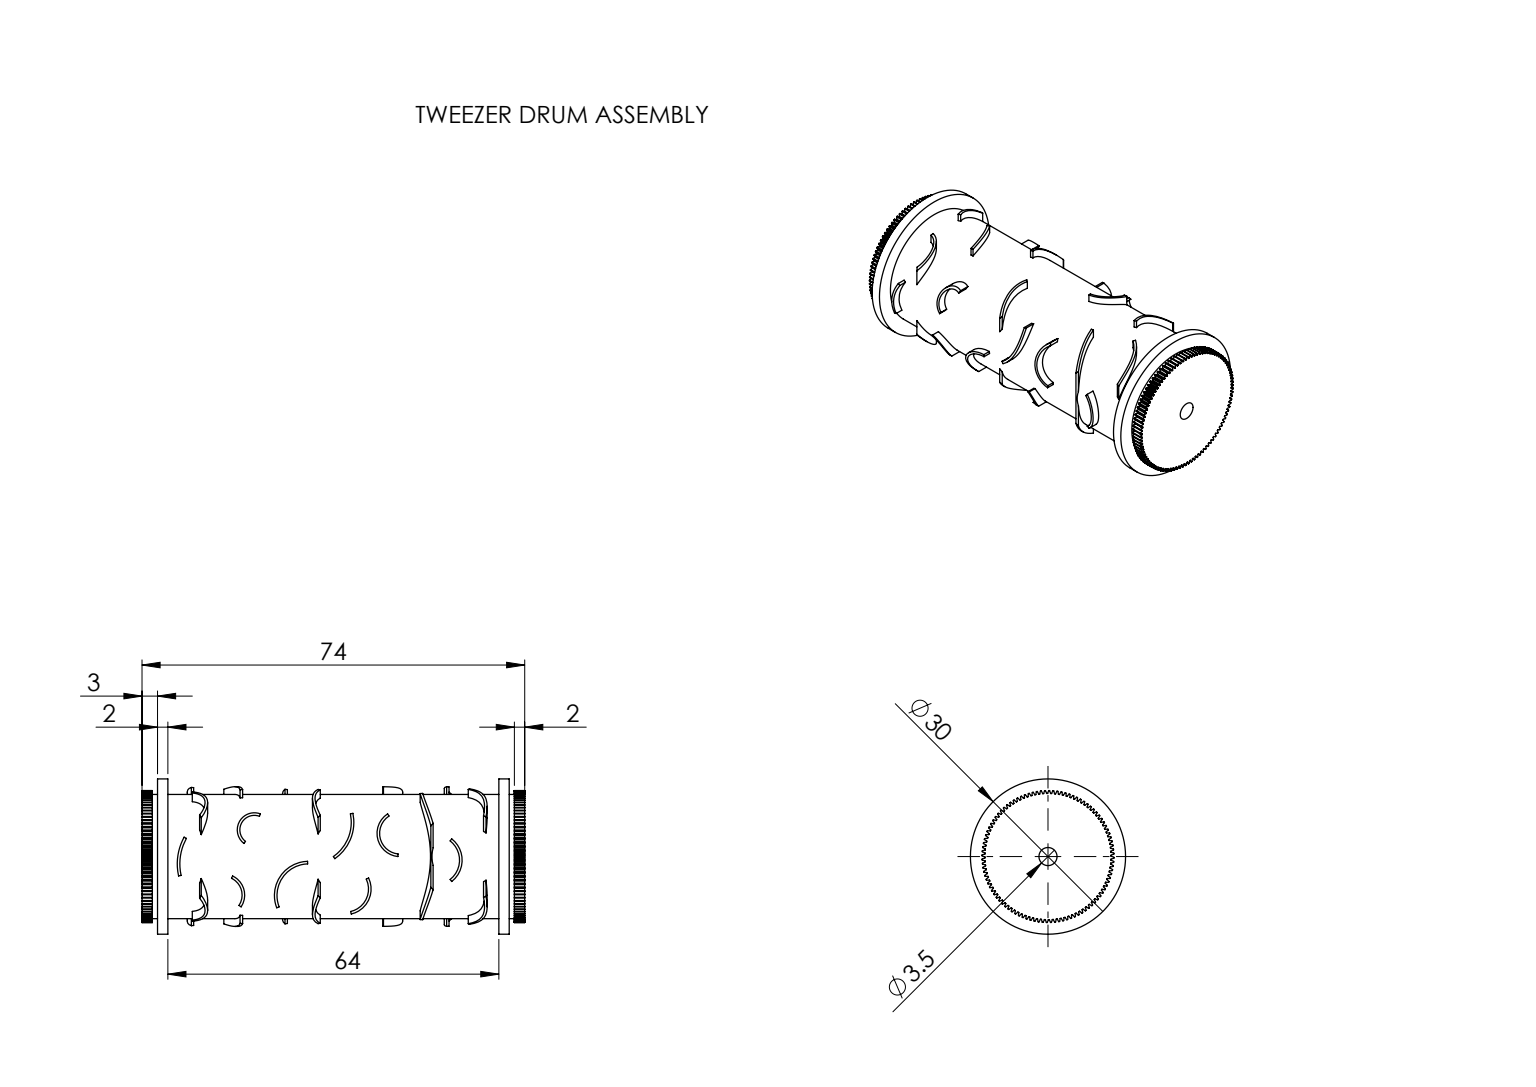
ISO-10303-21;
HEADER;
FILE_DESCRIPTION (('STEP AP214'),
    '1' );
FILE_NAME ('tweezer drum assembly.step',
    '2026-10-09T15:17:24',
    ( '' ),
    ( '' ),
    'SwSTEP 2.0',
    'SolidWorks 2026',
    '' );
FILE_SCHEMA (( 'AUTOMOTIVE_DESIGN' ));
ENDSEC;

DATA;
#1=ORIENTED_EDGE ( 'NONE', *, *, #54093, .F. ) ;
#2=( BOUNDED_CURVE ( )  B_SPLINE_CURVE ( 3, ( #3306, #62815, #58857, #63152 ),
 .UNSPECIFIED., .F., .T. ) 
 B_SPLINE_CURVE_WITH_KNOTS ( ( 4, 4 ),
 ( 1.289274629942206873, 1.307832622343243267 ),
 .UNSPECIFIED. ) 
 CURVE ( )  GEOMETRIC_REPRESENTATION_ITEM ( )  RATIONAL_B_SPLINE_CURVE ( ( 1.000000000000000000, 0.9999713002824244246, 0.9999713002824244246, 1.000000000000000000 ) ) 
 REPRESENTATION_ITEM ( '' )  );
#3=DIRECTION ( 'NONE',  ( 1.000000000000000000, 0.000000000000000000, -0.000000000000000000 ) ) ;
#4=CARTESIAN_POINT ( 'NONE',  ( 34.00000000000000000, 1.267509437117510519E-14, 0.000000000000000000 ) ) ;
#5=EDGE_CURVE ( 'NONE', #33980, #40116, #8200, .T. ) ;
#6=ORIENTED_EDGE ( 'NONE', *, *, #26203, .T. ) ;
#7=CARTESIAN_POINT ( 'NONE',  ( -27.64865282621882869, 11.88308961669896746, -6.412759754742364926 ) ) ;
#8=CARTESIAN_POINT ( 'NONE',  ( 29.22757921152195948, 7.948027597311009274, 9.002217460645077551 ) ) ;
#10=AXIS2_PLACEMENT_3D ( 'NONE', #51106, #21495, #16509 ) ;
#13=EDGE_CURVE ( 'NONE', #20288, #62523, #39030, .T. ) ;
#14=CIRCLE ( 'NONE', #45668, 4.999999999999999112 ) ;
#15=ORIENTED_EDGE ( 'NONE', *, *, #45352, .F. ) ;
#16=CARTESIAN_POINT ( 'NONE',  ( -2.532614230583026593, 25.00000000000000000, 10.89930238848911337 ) ) ;
#17=CARTESIAN_POINT ( 'NONE',  ( -20.31445708845316389, -13.09484702705360704, -3.338600914039887346 ) ) ;
#22=CARTESIAN_POINT ( 'NONE',  ( 37.00000000000000711, -6.303578524887017309, -10.42955799785317872 ) ) ;
#23=CARTESIAN_POINT ( 'NONE',  ( 3.459614771489464946, -11.09853614738469396, 25.00000000000000000 ) ) ;
#24=AXIS2_PLACEMENT_3D ( 'NONE', #425, #35953, #14688 ) ;
#26=CARTESIAN_POINT ( 'NONE',  ( 35.00000000000000000, 4.705694406421931860E-17, -3.469127814946512892E-15 ) ) ;
#27=CIRCLE ( 'NONE', #62657, 12.18649999999999878 ) ;
#29=CARTESIAN_POINT ( 'NONE',  ( 47.00000000000000711, 4.705694406421931860E-17, -3.469127814946512892E-15 ) ) ;
#30=DIRECTION ( 'NONE',  ( 1.000000000000000000, -0.000000000000000000, 0.000000000000000000 ) ) ;
#32=CARTESIAN_POINT ( 'NONE',  ( -36.00000000000000711, -2.527899948230555083, -12.49688848680887077 ) ) ;
#36=CIRCLE ( 'NONE', #39342, 5.000000000000000000 ) ;
#38=ORIENTED_EDGE ( 'NONE', *, *, #32481, .T. ) ;
#39=DIRECTION ( 'NONE',  ( 0.2227494284590502138, 0.000000000000000000, 0.9748757316300199482 ) ) ;
#41=DIRECTION ( 'NONE',  ( -1.000000000000000000, 0.000000000000000000, 0.000000000000000000 ) ) ;
#42=DIRECTION ( 'NONE',  ( -0.000000000000000000, -0.000000000000000000, -1.000000000000000000 ) ) ;
#43=ORIENTED_EDGE ( 'NONE', *, *, #16886, .F. ) ;
#44=VERTEX_POINT ( 'NONE', #43427 ) ;
#45=ORIENTED_EDGE ( 'NONE', *, *, #528, .T. ) ;
#47=AXIS2_PLACEMENT_3D ( 'NONE', #35700, #25750, #46038 ) ;
#48=CARTESIAN_POINT ( 'NONE',  ( -20.92008205012189848, -11.37744109147143590, -3.816568647652266222 ) ) ;
#49=EDGE_CURVE ( 'NONE', #39147, #50867, #8852, .T. ) ;
#52=CARTESIAN_POINT ( 'NONE',  ( 35.00000000000000000, 3.511814412392283646, 11.66953048682395355 ) ) ;
#54=ORIENTED_EDGE ( 'NONE', *, *, #43453, .T. ) ;
#56=EDGE_CURVE ( 'NONE', #31963, #46746, #12133, .T. ) ;
#58=DIRECTION ( 'NONE',  ( -0.000000000000000000, -0.000000000000000000, -1.000000000000000000 ) ) ;
#62=EDGE_LOOP ( 'NONE', ( #29288, #23107, #41719, #50661 ) ) ;
#64=VECTOR ( 'NONE', #37546, 1000.000000000000000 ) ;
#65=ORIENTED_EDGE ( 'NONE', *, *, #16176, .T. ) ;
#66=CARTESIAN_POINT ( 'NONE',  ( -28.82521652700830117, 2.770713649382011923, -11.70126355471820467 ) ) ;
#68=CARTESIAN_POINT ( 'NONE',  ( 37.00000000000000711, -11.24036214326524608, -6.018036132182126963 ) ) ;
#72=FACE_OUTER_BOUND ( 'NONE', #21763, .T. ) ;
#73=ADVANCED_FACE ( 'NONE', ( #28468 ), #28161, .T. ) ;
#76=CARTESIAN_POINT ( 'NONE',  ( -37.00000000000000711, 0.7536123767500182424, -11.72195762423409171 ) ) ;
#77=ORIENTED_EDGE ( 'NONE', *, *, #43041, .T. ) ;
#79=AXIS2_PLACEMENT_3D ( 'NONE', #49490, #64734, #28522 ) ;
#80=ORIENTED_EDGE ( 'NONE', *, *, #29710, .F. ) ;
#82=VERTEX_POINT ( 'NONE', #8514 ) ;
#83=EDGE_CURVE ( 'NONE', #13628, #12164, #48775, .T. ) ;
#85=VECTOR ( 'NONE', #37422, 1000.000000000000000 ) ;
#86=ORIENTED_EDGE ( 'NONE', *, *, #15250, .T. ) ;
#87=DIRECTION ( 'NONE',  ( 1.000000000000000000, -0.000000000000000000, -0.000000000000000000 ) ) ;
#88=LINE ( 'NONE', #34354, #47498 ) ;
#91=DIRECTION ( 'NONE',  ( 1.000000000000000000, 0.000000000000000000, 0.000000000000000000 ) ) ;
#92=CIRCLE ( 'NONE', #17079, 4.999999999999999112 ) ;
#93=AXIS2_PLACEMENT_3D ( 'NONE', #46470, #925, #21193 ) ;
#94=AXIS2_PLACEMENT_3D ( 'NONE', #16809, #31133, #22127 ) ;
#95=VERTEX_POINT ( 'NONE', #49115 ) ;
#96=CARTESIAN_POINT ( 'NONE',  ( -37.00000000000000711, 7.474872387601008583, 9.060822531526074641 ) ) ;
#97=EDGE_CURVE ( 'NONE', #10033, #43796, #33778, .T. ) ;
#98=AXIS2_PLACEMENT_3D ( 'NONE', #57341, #58008, #7118 ) ;
#99=ORIENTED_EDGE ( 'NONE', *, *, #2192, .T. ) ;
#102=FACE_OUTER_BOUND ( 'NONE', #65679, .T. ) ;
#105=CARTESIAN_POINT ( 'NONE',  ( -35.00000000000000000, 0.000000000000000000, 0.000000000000000000 ) ) ;
#107=AXIS2_PLACEMENT_3D ( 'NONE', #48295, #12020, #32299 ) ;
#108=CIRCLE ( 'NONE', #63839, 12.18649999999999700 ) ;
#109=AXIS2_PLACEMENT_3D ( 'NONE', #42573, #46294, #734 ) ;
#112=AXIS2_PLACEMENT_3D ( 'NONE', #43314, #33991, #53653 ) ;
#113=CARTESIAN_POINT ( 'NONE',  ( -10.71713000802667359, -9.043952695441483058, -10.03432938415238951 ) ) ;
#115=ORIENTED_EDGE ( 'NONE', *, *, #54584, .T. ) ;
#119=AXIS2_PLACEMENT_3D ( 'NONE', #1581, #5588, #900 ) ;
#120=ADVANCED_FACE ( 'NONE', ( #39097 ), #54424, .T. ) ;
#122=CARTESIAN_POINT ( 'NONE',  ( -37.00000000000000711, 12.02534193257726969, -4.237174932027097718 ) ) ;
#123=DIRECTION ( 'NONE',  ( 1.000000000000000000, -0.000000000000000000, 0.000000000000000000 ) ) ;
#124=CIRCLE ( 'NONE', #37284, 5.000000000000000000 ) ;
#127=CARTESIAN_POINT ( 'NONE',  ( 2.096166925314653984, 2.110369137379828786, -11.81794094722716260 ) ) ;
#129=EDGE_LOOP ( 'NONE', ( #26089, #45979, #28221, #53129 ) ) ;
#130=CARTESIAN_POINT ( 'NONE',  ( -35.00000000000000000, 11.56998259273177787, 3.827046518385122553 ) ) ;
#131=AXIS2_PLACEMENT_3D ( 'NONE', #9769, #50367, #4141 ) ;
#132=CARTESIAN_POINT ( 'NONE',  ( 37.00000000000000711, 4.705694406421931860E-17, -3.469127814946512892E-15 ) ) ;
#133=ORIENTED_EDGE ( 'NONE', *, *, #30675, .T. ) ;
#134=EDGE_CURVE ( 'NONE', #53943, #37151, #49390, .T. ) ;
#136=VERTEX_POINT ( 'NONE', #26116 ) ;
#137=AXIS2_PLACEMENT_3D ( 'NONE', #15886, #35532, #47176 ) ;
#139=VECTOR ( 'NONE', #13828, 1000.000000000000000 ) ;
#140=EDGE_CURVE ( 'NONE', #38995, #49368, #10066, .T. ) ;
#141=ORIENTED_EDGE ( 'NONE', *, *, #6255, .F. ) ;
#142=FACE_OUTER_BOUND ( 'NONE', #36024, .T. ) ;
#143=DIRECTION ( 'NONE',  ( 0.000000000000000000, -0.01356324068817999114, 0.9999080150203989437 ) ) ;
#144=DIRECTION ( 'NONE',  ( 1.000000000000000000, 0.000000000000000000, 0.000000000000000000 ) ) ;
#145=DIRECTION ( 'NONE',  ( 0.000000000000000000, -0.9796553971857763221, -0.2006870767258792099 ) ) ;
#148=CARTESIAN_POINT ( 'NONE',  ( -17.73782175230979874, 11.72754298194778677, 2.564785682591074867 ) ) ;
#149=CARTESIAN_POINT ( 'NONE',  ( 3.780834652287974773, 8.352030633203074927, 25.00000000000000000 ) ) ;
#150=ORIENTED_EDGE ( 'NONE', *, *, #41675, .F. ) ;
#151=DIRECTION ( 'NONE',  ( 0.1024315404614497965, 0.9947400562552481951, 0.000000000000000000 ) ) ;
#152=EDGE_CURVE ( 'NONE', #21897, #44042, #18588, .T. ) ;
#153=VERTEX_POINT ( 'NONE', #21105 ) ;
#154=CARTESIAN_POINT ( 'NONE',  ( 35.00000000000000000, 5.015831474386306610, -10.62137734850269943 ) ) ;
#155=EDGE_LOOP ( 'NONE', ( #12731, #28986, #56785, #59281 ) ) ;
#156=ORIENTED_EDGE ( 'NONE', *, *, #22157, .F. ) ;
#158=AXIS2_PLACEMENT_3D ( 'NONE', #49089, #24435, #29743 ) ;
#160=DIRECTION ( 'NONE',  ( 0.9318405276259970060, 0.3628680629012471237, 0.000000000000000000 ) ) ;
#161=AXIS2_PLACEMENT_3D ( 'NONE', #36598, #16644, #2007 ) ;
#163=CARTESIAN_POINT ( 'NONE',  ( 37.00000000000000711, -4.426194442447322075, -11.35427606708804937 ) ) ;
#167=VERTEX_POINT ( 'NONE', #45398 ) ;
#168=CARTESIAN_POINT ( 'NONE',  ( -36.00000000000000711, -10.59380114696474884, 7.094637218249319588 ) ) ;
#169=EDGE_LOOP ( 'NONE', ( #2246, #11811, #65657, #252 ) ) ;
#170=EDGE_CURVE ( 'NONE', #3983, #20113, #56362, .T. ) ;
#171=AXIS2_PLACEMENT_3D ( 'NONE', #20760, #45365, #40362 ) ;
#172=EDGE_CURVE ( 'NONE', #21730, #4780, #9821, .T. ) ;
#173=VERTEX_POINT ( 'NONE', #29764 ) ;
#174=FACE_OUTER_BOUND ( 'NONE', #28123, .T. ) ;
#176=DIRECTION ( 'NONE',  ( 0.000000000000000000, -0.4380125133594036657, 0.8989688749565127868 ) ) ;
#182=AXIS2_PLACEMENT_3D ( 'NONE', #6884, #41786, #7187 ) ;
#184=ORIENTED_EDGE ( 'NONE', *, *, #58820, .T. ) ;
#185=ADVANCED_FACE ( 'NONE', ( #61669 ), #5522, .T. ) ;
#187=VECTOR ( 'NONE', #61611, 1000.000000000000000 ) ;
#188=CARTESIAN_POINT ( 'NONE',  ( -19.47984447937493613, -3.750539801530005768, -12.96855624952674724 ) ) ;
#189=CARTESIAN_POINT ( 'NONE',  ( 36.00000000000000711, 4.983891302653744582, 11.73555825188270596 ) ) ;
#190=CARTESIAN_POINT ( 'NONE',  ( 6.361445718264521432, -4.355102044641763648, -12.77822703589027320 ) ) ;
#192=AXIS2_PLACEMENT_3D ( 'NONE', #53124, #17228, #57806 ) ;
#196=( BOUNDED_CURVE ( )  B_SPLINE_CURVE ( 3, ( #42557, #43227, #37603, #11661 ),
 .UNSPECIFIED., .F., .F. ) 
 B_SPLINE_CURVE_WITH_KNOTS ( ( 4, 4 ),
 ( 1.718692970945833176, 1.736025308729231442 ),
 .UNSPECIFIED. ) 
 CURVE ( )  GEOMETRIC_REPRESENTATION_ITEM ( )  RATIONAL_B_SPLINE_CURVE ( ( 1.000000000000000000, 0.9999749659955903258, 0.9999749659955903258, 1.000000000000000000 ) ) 
 REPRESENTATION_ITEM ( '' )  );
#197=CYLINDRICAL_SURFACE ( 'NONE', #36249, 12.18650000000000055 ) ;
#200=ORIENTED_EDGE ( 'NONE', *, *, #42042, .T. ) ;
#202=CARTESIAN_POINT ( 'NONE',  ( -35.00000000000000000, 10.14433819232434253, 6.753013023069750709 ) ) ;
#203=FACE_OUTER_BOUND ( 'NONE', #44719, .T. ) ;
#204=CIRCLE ( 'NONE', #54373, 12.74999999999999822 ) ;
#205=AXIS2_PLACEMENT_3D ( 'NONE', #46819, #52490, #27194 ) ;
#207=AXIS2_PLACEMENT_3D ( 'NONE', #6492, #31105, #57702 ) ;
#209=EDGE_CURVE ( 'NONE', #63155, #63467, #60591, .T. ) ;
#211=ORIENTED_EDGE ( 'NONE', *, *, #16595, .T. ) ;
#212=CARTESIAN_POINT ( 'NONE',  ( -37.00000000000000711, -12.18632975068353019, -0.06441628369849204672 ) ) ;
#217=VERTEX_POINT ( 'NONE', #15781 ) ;
#218=CARTESIAN_POINT ( 'NONE',  ( -35.00000000000000000, 8.839356091080043498, 8.389074212634319849 ) ) ;
#219=DIRECTION ( 'NONE',  ( -1.000000000000000000, 0.000000000000000000, 0.000000000000000000 ) ) ;
#221=AXIS2_PLACEMENT_3D ( 'NONE', #54414, #54070, #45388 ) ;
#222=EDGE_CURVE ( 'NONE', #29075, #15867, #7943, .T. ) ;
#229=CIRCLE ( 'NONE', #27843, 5.000000000000000888 ) ;
#230=CARTESIAN_POINT ( 'NONE',  ( -9.317410475120057711, 12.33400277018097313, -5.499978468384917996 ) ) ;
#231=CARTESIAN_POINT ( 'NONE',  ( -18.58686583997218378, 5.413436517372335111, -12.37033473226556701 ) ) ;
#232=DIRECTION ( 'NONE',  ( 0.000000000000000000, 0.9105187689795939399, -0.4134677391718545314 ) ) ;
#234=DIRECTION ( 'NONE',  ( 0.000000000000000000, -0.9718671068226485410, 0.2355298848897412756 ) ) ;
#237=ORIENTED_EDGE ( 'NONE', *, *, #59193, .T. ) ;
#238=DIRECTION ( 'NONE',  ( 0.000000000000000000, -0.01356324068817999114, 0.9999080150203989437 ) ) ;
#240=CIRCLE ( 'NONE', #37383, 5.000000000000000000 ) ;
#242=CARTESIAN_POINT ( 'NONE',  ( 35.00000000000000000, 1.771820996347156507, -11.61175578952786935 ) ) ;
#243=VECTOR ( 'NONE', #9924, 1000.000000000000000 ) ;
#245=AXIS2_PLACEMENT_3D ( 'NONE', #20192, #25505, #24868 ) ;
#246=AXIS2_PLACEMENT_3D ( 'NONE', #24663, #44940, #65220 ) ;
#250=CARTESIAN_POINT ( 'NONE',  ( 11.97679899998448683, 9.005363106165312104, -7.938319193498352355 ) ) ;
#252=ORIENTED_EDGE ( 'NONE', *, *, #20641, .T. ) ;
#253=ORIENTED_EDGE ( 'NONE', *, *, #48209, .T. ) ;
#254=FACE_OUTER_BOUND ( 'NONE', #27919, .T. ) ;
#255=ORIENTED_EDGE ( 'NONE', *, *, #44339, .F. ) ;
#256=CARTESIAN_POINT ( 'NONE',  ( 25.05309951391468459, -8.823569016628452388, -8.132934882857099979 ) ) ;
#259=ADVANCED_FACE ( 'NONE', ( #62326 ), #1174, .T. ) ;
#260=CARTESIAN_POINT ( 'NONE',  ( -35.00000000000000000, 9.752226076388895493, 6.547236723514054724 ) ) ;
#261=AXIS2_PLACEMENT_3D ( 'NONE', #65222, #29972, #35280 ) ;
#265=DIRECTION ( 'NONE',  ( -1.000000000000000000, -0.000000000000000000, 0.000000000000000000 ) ) ;
#266=VERTEX_POINT ( 'NONE', #11780 ) ;
#269=EDGE_CURVE ( 'NONE', #27971, #17610, #57880, .T. ) ;
#270=DIRECTION ( 'NONE',  ( 1.000000000000000000, 0.000000000000000000, 0.000000000000000000 ) ) ;
#271=DIRECTION ( 'NONE',  ( 0.000000000000000000, -0.01356324068817999114, 0.9999080150203989437 ) ) ;
#272=LINE ( 'NONE', #49512, #53068 ) ;
#273=LINE ( 'NONE', #15537, #61542 ) ;
#274=FACE_OUTER_BOUND ( 'NONE', #61383, .T. ) ;
#275=CARTESIAN_POINT ( 'NONE',  ( -37.00000000000000711, 1.591260454995410578, -12.08216339958899077 ) ) ;
#276=DIRECTION ( 'NONE',  ( 1.000000000000000000, 0.000000000000000000, 0.000000000000000000 ) ) ;
#278=CARTESIAN_POINT ( 'NONE',  ( 35.00000000000000000, -4.545979934229326780, 11.30684963584393543 ) ) ;
#279=EDGE_CURVE ( 'NONE', #31543, #49222, #7578, .T. ) ;
#280=AXIS2_PLACEMENT_3D ( 'NONE', #4610, #53838, #9548 ) ;
#282=CARTESIAN_POINT ( 'NONE',  ( -3.473816564737393087, -10.12352008167872164, 6.455743956261353667 ) ) ;
#283=CARTESIAN_POINT ( 'NONE',  ( -37.00000000000000711, 5.246972444134173408, -10.99909370905151995 ) ) ;
#286=CARTESIAN_POINT ( 'NONE',  ( 10.75853767213705225, 7.830989516993144051, 25.00000000000000000 ) ) ;
#287=ORIENTED_EDGE ( 'NONE', *, *, #23022, .F. ) ;
#288=AXIS2_PLACEMENT_3D ( 'NONE', #38389, #39045, #58707 ) ;
#301=CYLINDRICAL_SURFACE ( 'NONE', #23785, 4.999999999999999112 ) ;
#302=CARTESIAN_POINT ( 'NONE',  ( 36.00000000000000711, 1.457575200925544934, -12.66641127287626567 ) ) ;
#308=ORIENTED_EDGE ( 'NONE', *, *, #52732, .F. ) ;
#309=ORIENTED_EDGE ( 'NONE', *, *, #45374, .F. ) ;
#310=CARTESIAN_POINT ( 'NONE',  ( -30.12760453383368286, -0.2822123306220293837, 11.99877405949625242 ) ) ;
#311=VERTEX_POINT ( 'NONE', #11457 ) ;
#312=CARTESIAN_POINT ( 'NONE',  ( -27.45775109278351067, -10.51123867646838050, -8.471355351200609007 ) ) ;
#316=CARTESIAN_POINT ( 'NONE',  ( -11.40165637463000259, -7.955952249420155553, 10.91980268859785141 ) ) ;
#317=CARTESIAN_POINT ( 'NONE',  ( -11.37368538729251277, -6.793519583034608011, 9.901714675131643162 ) ) ;
#318=ORIENTED_EDGE ( 'NONE', *, *, #52044, .T. ) ;
#322=CARTESIAN_POINT ( 'NONE',  ( -35.00000000000000000, 1.039216533673073206, -11.70009620280410445 ) ) ;
#324=FACE_OUTER_BOUND ( 'NONE', #21670, .T. ) ;
#325=VERTEX_POINT ( 'NONE', #18102 ) ;
#327=ORIENTED_EDGE ( 'NONE', *, *, #30537, .F. ) ;
#329=CARTESIAN_POINT ( 'NONE',  ( -37.00000000000000711, -10.54834585426215732, -6.102719229070786788 ) ) ;
#330=CARTESIAN_POINT ( 'NONE',  ( 35.00000000000000000, 1.285879139104720949E-14, 0.000000000000000000 ) ) ;
#333=ORIENTED_EDGE ( 'NONE', *, *, #41127, .T. ) ;
#337=ORIENTED_EDGE ( 'NONE', *, *, #61367, .T. ) ;
#338=VECTOR ( 'NONE', #37910, 1000.000000000000000 ) ;
#339=AXIS2_PLACEMENT_3D ( 'NONE', #1310, #57489, #57162 ) ;
#341=EDGE_LOOP ( 'NONE', ( #2410, #23856, #26253, #58156 ) ) ;
#342=FACE_OUTER_BOUND ( 'NONE', #65268, .T. ) ;
#347=FACE_OUTER_BOUND ( 'NONE', #44647, .T. ) ;
#350=DIRECTION ( 'NONE',  ( 1.000000000000000000, 0.000000000000000000, 0.000000000000000000 ) ) ;
#351=ORIENTED_EDGE ( 'NONE', *, *, #15803, .T. ) ;
#352=CARTESIAN_POINT ( 'NONE',  ( -17.29244623348158783, 2.525873743887551814, 13.26159725786978960 ) ) ;
#354=CARTESIAN_POINT ( 'NONE',  ( -27.59804998575971169, 11.74707290664110637, -6.658303971331236859 ) ) ;
#355=VECTOR ( 'NONE', #27928, 1000.000000000000000 ) ;
#356=CARTESIAN_POINT ( 'NONE',  ( 29.03457606387295087, 4.854210015632069997, 10.97436308512422265 ) ) ;
#358=EDGE_CURVE ( 'NONE', #57018, #62845, #48344, .T. ) ;
#359=VECTOR ( 'NONE', #61792, 1000.000000000000000 ) ;
#360=ORIENTED_EDGE ( 'NONE', *, *, #31909, .T. ) ;
#361=LINE ( 'NONE', #6019, #33319 ) ;
#363=ORIENTED_EDGE ( 'NONE', *, *, #32286, .F. ) ;
#364=CARTESIAN_POINT ( 'NONE',  ( 12.47628546223243617, 0.000000000000000000, 13.50000000000000178 ) ) ;
#365=DIRECTION ( 'NONE',  ( -1.000000000000000000, 0.000000000000000000, 0.000000000000000000 ) ) ;
#368=CARTESIAN_POINT ( 'NONE',  ( -10.90165637462999904, -7.508992741355383416, -9.360289953322597611 ) ) ;
#369=CARTESIAN_POINT ( 'NONE',  ( -35.00000000000000000, 0.000000000000000000, 0.000000000000000000 ) ) ;
#371=DIRECTION ( 'NONE',  ( -1.000000000000000000, 0.000000000000000000, 0.000000000000000000 ) ) ;
#372=CARTESIAN_POINT ( 'NONE',  ( 36.00000000000000711, 0.3137578094511053184, 12.74613886779084204 ) ) ;
#373=CARTESIAN_POINT ( 'NONE',  ( 21.64884475953936160, 11.05386968847107454, -4.688304422177896669 ) ) ;
#374=CARTESIAN_POINT ( 'NONE',  ( 35.00000000000000000, 8.854740511458958352, 7.717887834988148121 ) ) ;
#376=EDGE_CURVE ( 'NONE', #58777, #10202, #63172, .T. ) ;
#377=CARTESIAN_POINT ( 'NONE',  ( -21.04919400413958286, 12.98042452237757516, -3.710884547572586900 ) ) ;
#379=EDGE_CURVE ( 'NONE', #7202, #39390, #41905, .T. ) ;
#380=CARTESIAN_POINT ( 'NONE',  ( -37.00000000000000711, 10.80478261802190154, -5.636262487437199376 ) ) ;
#381=CARTESIAN_POINT ( 'NONE',  ( -37.00000000000000711, -6.280308599560071592, -9.926225166347094842 ) ) ;
#382=DIRECTION ( 'NONE',  ( 0.000000000000000000, 0.1740410799127543318, 0.9847383929261630531 ) ) ;
#385=VECTOR ( 'NONE', #46411, 1000.000000000000000 ) ;
#386=CIRCLE ( 'NONE', #53354, 12.74999999999999822 ) ;
#387=EDGE_CURVE ( 'NONE', #44901, #11376, #34493, .T. ) ;
#388=ORIENTED_EDGE ( 'NONE', *, *, #52425, .T. ) ;
#389=ORIENTED_EDGE ( 'NONE', *, *, #15138, .T. ) ;
#395=VERTEX_POINT ( 'NONE', #38712 ) ;
#396=EDGE_CURVE ( 'NONE', #8331, #58552, #45570, .T. ) ;
#397=AXIS2_PLACEMENT_3D ( 'NONE', #55947, #25689, #45980 ) ;
#398=ORIENTED_EDGE ( 'NONE', *, *, #32115, .T. ) ;
#400=DIRECTION ( 'NONE',  ( 1.000000000000000000, 0.000000000000000000, -0.000000000000000000 ) ) ;
#402=CARTESIAN_POINT ( 'NONE',  ( 35.00000000000000000, 1.488153103996963100, -11.65150730582935523 ) ) ;
#403=EDGE_LOOP ( 'NONE', ( #55251, #13058, #53258, #22516 ) ) ;
#405=CARTESIAN_POINT ( 'NONE',  ( 35.00000000000000000, -9.076753354953932984, 8.954052073409695112 ) ) ;
#406=DIRECTION ( 'NONE',  ( 0.000000000000000000, 0.01356324068817998940, -0.9999080150203989437 ) ) ;
#411=VECTOR ( 'NONE', #62714, 1000.000000000000000 ) ;
#415=CARTESIAN_POINT ( 'NONE',  ( 35.00000000000000000, 10.80631716521673447, 4.603882218679430594 ) ) ;
#416=VERTEX_POINT ( 'NONE', #33391 ) ;
#417=CARTESIAN_POINT ( 'NONE',  ( -29.92777678363736626, -3.750539801530011985, -11.39883551934752681 ) ) ;
#418=ORIENTED_EDGE ( 'NONE', *, *, #52411, .F. ) ;
#422=CARTESIAN_POINT ( 'NONE',  ( 26.08439714455133185, 25.00000000000000000, 3.743551691817327942 ) ) ;
#425=CARTESIAN_POINT ( 'NONE',  ( 37.00000000000000711, 4.705694406421931860E-17, -3.469127814946512892E-15 ) ) ;
#427=CARTESIAN_POINT ( 'NONE',  ( 35.00000000000000000, -6.475373545682373333, -10.32377448871666026 ) ) ;
#428=CARTESIAN_POINT ( 'NONE',  ( 35.00000000000000000, 3.704519465651471499, 11.60979404548630178 ) ) ;
#429=VERTEX_POINT ( 'NONE', #22 ) ;
#430=DIRECTION ( 'NONE',  ( 1.000000000000000000, 0.000000000000000000, -0.000000000000000000 ) ) ;
#431=ORIENTED_EDGE ( 'NONE', *, *, #26732, .T. ) ;
#432=CARTESIAN_POINT ( 'NONE',  ( 12.60173367434126490, -10.92909900068726792, -7.935196926251238736 ) ) ;
#433=VERTEX_POINT ( 'NONE', #2833 ) ;
#434=DIRECTION ( 'NONE',  ( 1.000000000000000000, 0.000000000000000000, 0.000000000000000000 ) ) ;
#435=VECTOR ( 'NONE', #47244, 1000.000000000000000 ) ;
#437=DIRECTION ( 'NONE',  ( 0.000000000000000000, 0.3554799084908900619, 0.9346839223284567622 ) ) ;
#438=CIRCLE ( 'NONE', #2582, 12.18650000000000055 ) ;
#442=EDGE_CURVE ( 'NONE', #3284, #31374, #16898, .T. ) ;
#443=CARTESIAN_POINT ( 'NONE',  ( -37.00000000000000711, -11.71932350927023414, 3.511386971104904386 ) ) ;
#444=EDGE_LOOP ( 'NONE', ( #60169, #14313, #42330, #32413 ) ) ;
#445=CARTESIAN_POINT ( 'NONE',  ( 35.00000000000000000, 10.30098186818249673, -5.644643009979106729 ) ) ;
#446=VECTOR ( 'NONE', #37071, 1000.000000000000000 ) ;
#448=FACE_BOUND ( 'NONE', #52190, .T. ) ;
#449=CARTESIAN_POINT ( 'NONE',  ( 35.00000000000000000, 11.02904044024202967, -4.041347439436060007 ) ) ;
#450=CARTESIAN_POINT ( 'NONE',  ( -35.00000000000000000, 4.426194442447240363, 11.35427606708807957 ) ) ;
#452=DIRECTION ( 'NONE',  ( -1.000000000000000000, 0.000000000000000000, 0.000000000000000000 ) ) ;
#453=AXIS2_PLACEMENT_3D ( 'NONE', #38158, #23546, #33523 ) ;
#454=ADVANCED_FACE ( 'NONE', ( #53690 ), #60537, .T. ) ;
#457=DIRECTION ( 'NONE',  ( 0.000000000000000000, 0.01356324068818000848, -0.9999080150203990547 ) ) ;
#458=ADVANCED_FACE ( 'NONE', ( #18456 ), #8446, .T. ) ;
#459=AXIS2_PLACEMENT_3D ( 'NONE', #21770, #46690, #52988 ) ;
#460=CARTESIAN_POINT ( 'NONE',  ( 36.00000000000000711, -12.21925492305364713, -3.640372113593510761 ) ) ;
#462=EDGE_CURVE ( 'NONE', #46347, #21361, #20738, .T. ) ;
#463=ORIENTED_EDGE ( 'NONE', *, *, #54480, .T. ) ;
#464=DIRECTION ( 'NONE',  ( 1.000000000000000000, 0.000000000000000000, 0.000000000000000000 ) ) ;
#468=EDGE_CURVE ( 'NONE', #3878, #65629, #14971, .T. ) ;
#470=CARTESIAN_POINT ( 'NONE',  ( -14.11589373245165469, 8.250315036047107142, -10.68561190601526256 ) ) ;
#471=ORIENTED_EDGE ( 'NONE', *, *, #2353, .F. ) ;
#473=EDGE_CURVE ( 'NONE', #55881, #65529, #14365, .T. ) ;
#474=CYLINDRICAL_SURFACE ( 'NONE', #40618, 12.74999999999999822 ) ;
#476=VERTEX_POINT ( 'NONE', #20306 ) ;
#477=CARTESIAN_POINT ( 'NONE',  ( 35.00000000000000000, -11.80185301892977279, 4.824807283154242121 ) ) ;
#478=CARTESIAN_POINT ( 'NONE',  ( 35.00000000000000000, 11.73808581813437080, -0.4353888892050498116 ) ) ;
#480=AXIS2_PLACEMENT_3D ( 'NONE', #59042, #13770, #54378 ) ;
#481=AXIS2_PLACEMENT_3D ( 'NONE', #42373, #6510, #550 ) ;
#484=EDGE_LOOP ( 'NONE', ( #30253, #3866, #979, #57703 ) ) ;
#485=EDGE_CURVE ( 'NONE', #64690, #35052, #56203, .T. ) ;
#487=DIRECTION ( 'NONE',  ( 0.000000000000000000, -0.7381862504171878836, 0.6745969609292743474 ) ) ;
#488=CARTESIAN_POINT ( 'NONE',  ( -35.00000000000000000, 0.000000000000000000, 0.000000000000000000 ) ) ;
#489=CARTESIAN_POINT ( 'NONE',  ( 6.812204945636112896, -4.138731716409435712, 11.26369831714195335 ) ) ;
#490=CARTESIAN_POINT ( 'NONE',  ( -4.989057617119008192, -0.9162120371760335003, 13.46887357958837406 ) ) ;
#492=CARTESIAN_POINT ( 'NONE',  ( 24.83805482081016791, -1.521295006216393908, -13.41549933947825224 ) ) ;
#493=CARTESIAN_POINT ( 'NONE',  ( 35.00000000000000000, 10.42955799785319648, -6.303578524886984447 ) ) ;
#494=ORIENTED_EDGE ( 'NONE', *, *, #26778, .F. ) ;
#495=PLANE ( 'NONE',  #171 ) ;
#496=ORIENTED_EDGE ( 'NONE', *, *, #1465, .F. ) ;
#498=EDGE_LOOP ( 'NONE', ( #38392, #765, #24138, #47981 ) ) ;
#502=AXIS2_PLACEMENT_3D ( 'NONE', #24845, #9864, #15502 ) ;
#503=DIRECTION ( 'NONE',  ( -1.000000000000000000, -0.000000000000000000, 0.000000000000000000 ) ) ;
#504=CYLINDRICAL_SURFACE ( 'NONE', #54627, 5.000000000000000888 ) ;
#505=CYLINDRICAL_SURFACE ( 'NONE', #15469, 5.000000000000000888 ) ;
#508=ORIENTED_EDGE ( 'NONE', *, *, #5192, .T. ) ;
#510=ORIENTED_EDGE ( 'NONE', *, *, #14071, .T. ) ;
#511=ORIENTED_EDGE ( 'NONE', *, *, #46854, .F. ) ;
#513=CARTESIAN_POINT ( 'NONE',  ( -35.00000000000000000, -10.99909370905153594, -5.246972444134134328 ) ) ;
#515=CARTESIAN_POINT ( 'NONE',  ( 17.41455116976016981, 8.220693008476809283, 8.757759849264344254 ) ) ;
#517=ADVANCED_FACE ( 'NONE', ( #51579 ), #45917, .T. ) ;
#518=CARTESIAN_POINT ( 'NONE',  ( -5.884299113211928223, -0.9870258725403491251, -11.95978215124650923 ) ) ;
#519=AXIS2_PLACEMENT_3D ( 'NONE', #15215, #29220, #49515 ) ;
#521=ORIENTED_EDGE ( 'NONE', *, *, #24511, .T. ) ;
#523=VECTOR ( 'NONE', #9694, 1000.000000000000000 ) ;
#524=LINE ( 'NONE', #25127, #20210 ) ;
#525=EDGE_CURVE ( 'NONE', #52168, #55868, #30598, .T. ) ;
#526=CARTESIAN_POINT ( 'NONE',  ( -3.378459980749651148, -10.08685364769616299, 9.001353960567275436 ) ) ;
#527=DIRECTION ( 'NONE',  ( -1.000000000000000000, -0.000000000000000000, 0.000000000000000000 ) ) ;
#528=EDGE_CURVE ( 'NONE', #9921, #51290, #11199, .T. ) ;
#529=CARTESIAN_POINT ( 'NONE',  ( 35.00000000000000000, 11.42599468261429152, -4.237620530777845396 ) ) ;
#533=CARTESIAN_POINT ( 'NONE',  ( 37.00000000000000711, 2.696588552979229725, 12.46157735505186004 ) ) ;
#535=EDGE_CURVE ( 'NONE', #13015, #47412, #20651, .T. ) ;
#536=ORIENTED_EDGE ( 'NONE', *, *, #57948, .T. ) ;
#537=AXIS2_PLACEMENT_3D ( 'NONE', #40562, #25944, #41206 ) ;
#539=DIRECTION ( 'NONE',  ( 0.000000000000000000, -0.6745969609292555846, -0.7381862504172049810 ) ) ;
#540=LINE ( 'NONE', #61351, #50346 ) ;
#541=AXIS2_PLACEMENT_3D ( 'NONE', #51689, #37348, #57984 ) ;
#543=CYLINDRICAL_SURFACE ( 'NONE', #45743, 12.75000000000000178 ) ;
#544=ORIENTED_EDGE ( 'NONE', *, *, #30185, .F. ) ;
#545=CARTESIAN_POINT ( 'NONE',  ( -19.17721427606680251, -3.894607805094318032, -12.92689141258588847 ) ) ;
#547=ADVANCED_FACE ( 'NONE', ( #26942 ), #6028, .T. ) ;
#549=ORIENTED_EDGE ( 'NONE', *, *, #20317, .T. ) ;
#550=DIRECTION ( 'NONE',  ( 0.000000000000000000, -0.01356324068817998940, 0.9999080150203990547 ) ) ;
#552=CYLINDRICAL_SURFACE ( 'NONE', #25924, 4.999999999999999112 ) ;
#553=EDGE_CURVE ( 'NONE', #5802, #65741, #4808, .T. ) ;
#555=ORIENTED_EDGE ( 'NONE', *, *, #41297, .F. ) ;
#558=EDGE_CURVE ( 'NONE', #56170, #24551, #58977, .T. ) ;
#560=ORIENTED_EDGE ( 'NONE', *, *, #56639, .F. ) ;
#561=EDGE_CURVE ( 'NONE', #2301, #2844, #15412, .T. ) ;
#562=DIRECTION ( 'NONE',  ( -0.4327406564646559262, 0.9015184547431841500, 0.000000000000000000 ) ) ;
#564=CARTESIAN_POINT ( 'NONE',  ( 24.06146064158421538, -2.489685948191276310, -11.74338419841854098 ) ) ;
#565=CARTESIAN_POINT ( 'NONE',  ( 8.449549814414584858, 4.860417429574915182, -12.59635262386618137 ) ) ;
#566=DIRECTION ( 'NONE',  ( 0.000000000000000000, 0.4935949184179201366, -0.8696919319575217022 ) ) ;
#567=ADVANCED_FACE ( 'NONE', ( #41231 ), #60880, .T. ) ;
#568=CARTESIAN_POINT ( 'NONE',  ( 37.00000000000000711, 1.113475361586665491, 12.70128625845191195 ) ) ;
#571=ORIENTED_EDGE ( 'NONE', *, *, #34753, .T. ) ;
#573=ORIENTED_EDGE ( 'NONE', *, *, #35161, .T. ) ;
#575=DIRECTION ( 'NONE',  ( 1.000000000000000000, 0.000000000000000000, -0.000000000000000000 ) ) ;
#577=LINE ( 'NONE', #31779, #44701 ) ;
#578=ORIENTED_EDGE ( 'NONE', *, *, #49298, .F. ) ;
#579=CARTESIAN_POINT ( 'NONE',  ( -35.00000000000000000, 4.309077947445652867, 10.92721691015457708 ) ) ;
#582=DIRECTION ( 'NONE',  ( 0.000000000000000000, 0.7381862504171926576, -0.6745969609292691294 ) ) ;
#583=ORIENTED_EDGE ( 'NONE', *, *, #15533, .F. ) ;
#584=ORIENTED_EDGE ( 'NONE', *, *, #3130, .T. ) ;
#585=CARTESIAN_POINT ( 'NONE',  ( -35.00000000000000000, 0.000000000000000000, 0.000000000000000000 ) ) ;
#586=EDGE_LOOP ( 'NONE', ( #58558, #49260, #9799, #51354 ) ) ;
#587=DIRECTION ( 'NONE',  ( 0.000000000000000000, 0.01356324068817998940, -0.9999080150203990547 ) ) ;
#590=AXIS2_PLACEMENT_3D ( 'NONE', #54056, #34078, #29119 ) ;
#592=EDGE_CURVE ( 'NONE', #6726, #39576, #27098, .T. ) ;
#593=DIRECTION ( 'NONE',  ( 1.000000000000000000, 0.000000000000000000, -0.000000000000000000 ) ) ;
#595=DIRECTION ( 'NONE',  ( -0.000000000000000000, -0.000000000000000000, -1.000000000000000000 ) ) ;
#598=CARTESIAN_POINT ( 'NONE',  ( 35.00000000000000000, 11.53507381115583108, 2.216820770815121744 ) ) ;
#599=DIRECTION ( 'NONE',  ( 0.000000000000000000, -0.01356324068817998940, 0.9999080150203990547 ) ) ;
#600=CARTESIAN_POINT ( 'NONE',  ( 37.00000000000000711, -4.732539170486179891, 11.23004253107769301 ) ) ;
#601=CARTESIAN_POINT ( 'NONE',  ( 35.00000000000000000, 11.50504120060948487, 4.018060380616274685 ) ) ;
#602=DIRECTION ( 'NONE',  ( -1.000000000000000000, 0.000000000000000000, -0.000000000000000000 ) ) ;
#605=ADVANCED_FACE ( 'NONE', ( #31279 ), #16314, .T. ) ;
#607=AXIS2_PLACEMENT_3D ( 'NONE', #17941, #12282, #63161 ) ;
#612=CYLINDRICAL_SURFACE ( 'NONE', #1698, 12.75000000000000178 ) ;
#615=EDGE_CURVE ( 'NONE', #42846, #32620, #57927, .T. ) ;
#617=CARTESIAN_POINT ( 'NONE',  ( -11.08926364416224963, -9.550046432103219018, -9.555892453209455795 ) ) ;
#618=DIRECTION ( 'NONE',  ( 0.000000000000000000, 0.01356324068817998593, -0.9999080150203990547 ) ) ;
#621=CARTESIAN_POINT ( 'NONE',  ( 29.03457606387295087, -4.854210015632035358, 10.97436308512422265 ) ) ;
#624=ORIENTED_EDGE ( 'NONE', *, *, #54431, .T. ) ;
#626=ORIENTED_EDGE ( 'NONE', *, *, #10255, .T. ) ;
#630=CARTESIAN_POINT ( 'NONE',  ( -10.90165637462998660, -7.182798387602194801, 9.621968923399183637 ) ) ;
#632=CIRCLE ( 'NONE', #37787, 5.000000000000001776 ) ;
#635=CARTESIAN_POINT ( 'NONE',  ( 36.00000000000000711, 6.564808257521770329, -10.93004082984021252 ) ) ;
#636=ADVANCED_FACE ( 'NONE', ( #57208 ), #11635, .T. ) ;
#639=CYLINDRICAL_SURFACE ( 'NONE', #40636, 4.999999999999999112 ) ;
#642=CARTESIAN_POINT ( 'NONE',  ( 22.68150004936237707, 3.158880575389225065, 11.57756885178368833 ) ) ;
#643=ADVANCED_FACE ( 'NONE', ( #37224 ), #17294, .T. ) ;
#644=DIRECTION ( 'NONE',  ( 0.000000000000000000, 0.01356324068818000848, -0.9999080150203990547 ) ) ;
#649=DIRECTION ( 'NONE',  ( 0.000000000000000000, 0.000000000000000000, 1.000000000000000000 ) ) ;
#650=CARTESIAN_POINT ( 'NONE',  ( -37.00000000000000711, 7.238157050195776598, -10.49626516989263614 ) ) ;
#651=CARTESIAN_POINT ( 'NONE',  ( -35.00000000000000000, 9.040300684349693583, 7.499679039484089316 ) ) ;
#652=ORIENTED_EDGE ( 'NONE', *, *, #58820, .F. ) ;
#654=ORIENTED_EDGE ( 'NONE', *, *, #45190, .F. ) ;
#656=CYLINDRICAL_SURFACE ( 'NONE', #61527, 10.20557198542813815 ) ;
#660=ORIENTED_EDGE ( 'NONE', *, *, #35188, .F. ) ;
#661=CARTESIAN_POINT ( 'NONE',  ( 0.000000000000000000, -1.734723475976807094E-15, 13.50000000000000178 ) ) ;
#664=EDGE_LOOP ( 'NONE', ( #36440, #17580, #50368, #8037 ) ) ;
#665=VERTEX_POINT ( 'NONE', #32884 ) ;
#667=DIRECTION ( 'NONE',  ( 0.000000000000000000, 0.2960891610144510966, 0.9551603052523479631 ) ) ;
#669=EDGE_CURVE ( 'NONE', #52645, #21040, #65347, .T. ) ;
#673=ORIENTED_EDGE ( 'NONE', *, *, #65732, .F. ) ;
#674=AXIS2_PLACEMENT_3D ( 'NONE', #36714, #57996, #52358 ) ;
#675=DIRECTION ( 'NONE',  ( -1.000000000000000000, 0.000000000000000000, 0.000000000000000000 ) ) ;
#676=ADVANCED_FACE ( 'NONE', ( #21954 ), #1688, .T. ) ;
#677=CIRCLE ( 'NONE', #34620, 5.000000000000000000 ) ;
#678=ORIENTED_EDGE ( 'NONE', *, *, #14140, .T. ) ;
#679=CARTESIAN_POINT ( 'NONE',  ( -29.92777678363736626, -3.750539801530011985, -12.96855624952674724 ) ) ;
#681=DIRECTION ( 'NONE',  ( 0.000000000000000000, -0.9246979985058763063, -0.3807014730195120711 ) ) ;
#682=CARTESIAN_POINT ( 'NONE',  ( -37.00000000000000711, -10.91072401419407001, -5.428340790341820821 ) ) ;
#686=ORIENTED_EDGE ( 'NONE', *, *, #30624, .T. ) ;
#689=FACE_OUTER_BOUND ( 'NONE', #23945, .T. ) ;
#692=DIRECTION ( 'NONE',  ( 0.000000000000000000, -0.01356324068817998940, 0.9999080150203990547 ) ) ;
#694=EDGE_CURVE ( 'NONE', #57232, #43816, #50467, .T. ) ;
#695=EDGE_CURVE ( 'NONE', #22968, #32750, #36676, .T. ) ;
#696=ORIENTED_EDGE ( 'NONE', *, *, #59994, .F. ) ;
#697=CARTESIAN_POINT ( 'NONE',  ( 36.00000000000000711, 4.400442035670942609, -11.96656215839370851 ) ) ;
#698=CARTESIAN_POINT ( 'NONE',  ( 47.00000000000000711, 4.705694406421931860E-17, -3.469127814946512892E-15 ) ) ;
#699=CARTESIAN_POINT ( 'NONE',  ( 23.32362518313050614, 9.357419094640528456, -7.519995448741596533 ) ) ;
#700=CARTESIAN_POINT ( 'NONE',  ( 23.64431542999218294, -11.46495565953754792, -7.133712268643341403 ) ) ;
#701=EDGE_CURVE ( 'NONE', #12145, #21025, #36642, .T. ) ;
#707=VECTOR ( 'NONE', #33683, 1000.000000000000000 ) ;
#710=ORIENTED_EDGE ( 'NONE', *, *, #27283, .T. ) ;
#711=ADVANCED_FACE ( 'NONE', ( #43522 ), #63474, .T. ) ;
#714=CYLINDRICAL_SURFACE ( 'NONE', #28997, 4.999999999999997335 ) ;
#715=CARTESIAN_POINT ( 'NONE',  ( -35.00000000000000000, 0.000000000000000000, 0.000000000000000000 ) ) ;
#716=DIRECTION ( 'NONE',  ( 0.000000000000000000, -0.01356324068817991828, 0.9999080150203990547 ) ) ;
#717=ORIENTED_EDGE ( 'NONE', *, *, #21995, .T. ) ;
#718=ORIENTED_EDGE ( 'NONE', *, *, #61557, .T. ) ;
#720=CARTESIAN_POINT ( 'NONE',  ( 37.00000000000000711, -12.74613886779084382, 0.3137578094510532489 ) ) ;
#722=ORIENTED_EDGE ( 'NONE', *, *, #37336, .F. ) ;
#723=CARTESIAN_POINT ( 'NONE',  ( 6.361445718264521432, -4.355102044641763648, 12.77822703589027320 ) ) ;
#724=CYLINDRICAL_SURFACE ( 'NONE', #42705, 5.000000000000000888 ) ;
#728=LINE ( 'NONE', #60250, #54703 ) ;
#729=EDGE_LOOP ( 'NONE', ( #16935, #19715, #52598, #51184 ) ) ;
#730=LINE ( 'NONE', #49960, #59686 ) ;
#731=ORIENTED_EDGE ( 'NONE', *, *, #62834, .F. ) ;
#732=LINE ( 'NONE', #6711, #42192 ) ;
#733=ORIENTED_EDGE ( 'NONE', *, *, #40830, .F. ) ;
#734=DIRECTION ( 'NONE',  ( 0.000000000000000000, 0.4134677391718449280, 0.9105187689795983808 ) ) ;
#737=DIRECTION ( 'NONE',  ( 1.000000000000000000, 0.000000000000000000, 0.000000000000000000 ) ) ;
#742=CARTESIAN_POINT ( 'NONE',  ( 5.187165255848094958, -10.33573060559526446, 8.685987315626189087 ) ) ;
#743=VERTEX_POINT ( 'NONE', #12287 ) ;
#746=ORIENTED_EDGE ( 'NONE', *, *, #28329, .F. ) ;
#748=CARTESIAN_POINT ( 'NONE',  ( 35.00000000000000000, 11.60979404548634619, -3.704519465651352483 ) ) ;
#749=ORIENTED_EDGE ( 'NONE', *, *, #60715, .T. ) ;
#753=AXIS2_PLACEMENT_3D ( 'NONE', #48750, #3202, #43746 ) ;
#754=CYLINDRICAL_SURFACE ( 'NONE', #41257, 12.75000000000000178 ) ;
#757=ORIENTED_EDGE ( 'NONE', *, *, #3796, .F. ) ;
#758=VECTOR ( 'NONE', #8324, 1000.000000000000000 ) ;
#759=CARTESIAN_POINT ( 'NONE',  ( -35.00000000000000000, 0.000000000000000000, 0.000000000000000000 ) ) ;
#762=FACE_OUTER_BOUND ( 'NONE', #45586, .T. ) ;
#765=ORIENTED_EDGE ( 'NONE', *, *, #30183, .F. ) ;
#767=( BOUNDED_CURVE ( )  B_SPLINE_CURVE ( 3, ( #59079, #17840, #43417, #33125 ),
 .UNSPECIFIED., .F., .F. ) 
 B_SPLINE_CURVE_WITH_KNOTS ( ( 4, 4 ),
 ( 0.6374084671583093442, 0.6849672343075862146 ),
 .UNSPECIFIED. ) 
 CURVE ( )  GEOMETRIC_REPRESENTATION_ITEM ( )  RATIONAL_B_SPLINE_CURVE ( ( 1.000000000000000000, 0.9998115225205463918, 0.9998115225205463918, 1.000000000000000000 ) ) 
 REPRESENTATION_ITEM ( '' )  );
#768=CARTESIAN_POINT ( 'NONE',  ( 26.44191060433393048, 12.90701898410668846, 3.963759825896518763 ) ) ;
#770=CARTESIAN_POINT ( 'NONE',  ( 11.99003848479309298, 10.55797189877291054, -8.414293459742244963 ) ) ;
#774=DIRECTION ( 'NONE',  ( -1.000000000000000000, 0.000000000000000000, 0.000000000000000000 ) ) ;
#775=EDGE_CURVE ( 'NONE', #30093, #56170, #13911, .T. ) ;
#777=CARTESIAN_POINT ( 'NONE',  ( -18.06053859689077257, 5.591681739832217168, 12.28972654602461922 ) ) ;
#779=ORIENTED_EDGE ( 'NONE', *, *, #18157, .F. ) ;
#781=CARTESIAN_POINT ( 'NONE',  ( 37.00000000000000711, 7.499679039484058229, -9.040300684349723781 ) ) ;
#783=EDGE_LOOP ( 'NONE', ( #27018, #40138, #64745, #62156 ) ) ;
#785=CARTESIAN_POINT ( 'NONE',  ( -37.00000000000000711, -11.37311665002361494, -2.936739658819992549 ) ) ;
#786=VERTEX_POINT ( 'NONE', #60455 ) ;
#787=ORIENTED_EDGE ( 'NONE', *, *, #22061, .F. ) ;
#791=CIRCLE ( 'NONE', #37956, 12.18650000000000233 ) ;
#792=ORIENTED_EDGE ( 'NONE', *, *, #53491, .T. ) ;
#795=DIRECTION ( 'NONE',  ( -1.000000000000000000, 0.000000000000000000, 0.000000000000000000 ) ) ;
#796=CARTESIAN_POINT ( 'NONE',  ( 10.75853767213705225, 7.830989516993144051, 9.092612561015865680 ) ) ;
#797=VERTEX_POINT ( 'NONE', #24897 ) ;
#802=ORIENTED_EDGE ( 'NONE', *, *, #61825, .F. ) ;
#803=LINE ( 'NONE', #51023, #53281 ) ;
#804=ORIENTED_EDGE ( 'NONE', *, *, #45884, .F. ) ;
#805=CARTESIAN_POINT ( 'NONE',  ( -35.00000000000000000, 5.921969905510501064, -10.14408668126206869 ) ) ;
#809=CYLINDRICAL_SURFACE ( 'NONE', #10731, 4.999999999999998224 ) ;
#813=CYLINDRICAL_SURFACE ( 'NONE', #28256, 4.725920239717170901 ) ;
#814=LINE ( 'NONE', #56699, #25637 ) ;
#815=VERTEX_POINT ( 'NONE', #59176 ) ;
#816=EDGE_CURVE ( 'NONE', #36349, #13265, #3325, .T. ) ;
#817=VERTEX_POINT ( 'NONE', #29533 ) ;
#818=EDGE_CURVE ( 'NONE', #43621, #13249, #2936, .T. ) ;
#820=EDGE_LOOP ( 'NONE', ( #51764, #48932, #27665, #36662 ) ) ;
#823=ORIENTED_EDGE ( 'NONE', *, *, #31386, .T. ) ;
#826=DIRECTION ( 'NONE',  ( -1.000000000000000000, 0.000000000000000000, 0.000000000000000000 ) ) ;
#828=LINE ( 'NONE', #62628, #34195 ) ;
#829=LINE ( 'NONE', #56713, #27354 ) ;
#831=CARTESIAN_POINT ( 'NONE',  ( -35.00000000000000000, -11.78745411414837818, -3.093009498344053032 ) ) ;
#833=DIRECTION ( 'NONE',  ( 1.000000000000000000, 0.000000000000000000, 0.000000000000000000 ) ) ;
#834=CIRCLE ( 'NONE', #42232, 12.74999999999999822 ) ;
#835=ORIENTED_EDGE ( 'NONE', *, *, #4136, .T. ) ;
#836=FACE_OUTER_BOUND ( 'NONE', #5027, .T. ) ;
#837=ADVANCED_FACE ( 'NONE', ( #54832 ), #8614, .T. ) ;
#840=CARTESIAN_POINT ( 'NONE',  ( 4.036807064762983899, -10.39659893473963947, 5.993789462885469987 ) ) ;
#841=LINE ( 'NONE', #529, #61898 ) ;
#842=CIRCLE ( 'NONE', #43306, 5.000000000000000000 ) ;
#843=ADVANCED_FACE ( 'NONE', ( #40163 ), #38885, .T. ) ;
#844=CARTESIAN_POINT ( 'NONE',  ( 24.40033961665191953, -0.3581885377669972170, -13.50005958318994814 ) ) ;
#846=FACE_OUTER_BOUND ( 'NONE', #63936, .T. ) ;
#848=DIRECTION ( 'NONE',  ( -1.000000000000000000, 0.000000000000000000, -0.000000000000000000 ) ) ;
#849=CARTESIAN_POINT ( 'NONE',  ( 35.00000000000000000, -10.62137734850271364, -5.015831474386272859 ) ) ;
#851=CARTESIAN_POINT ( 'NONE',  ( -24.94459482683992135, 9.240370367366107729, 7.658175360001901133 ) ) ;
#853=VERTEX_POINT ( 'NONE', #39190 ) ;
#854=CARTESIAN_POINT ( 'NONE',  ( -17.83419946441818027, -9.720786832536937538, -9.367833439828872955 ) ) ;
#855=DIRECTION ( 'NONE',  ( 0.000000000000000000, 0.01356324068817998940, -0.9999080150203990547 ) ) ;
#857=ORIENTED_EDGE ( 'NONE', *, *, #24910, .T. ) ;
#860=CARTESIAN_POINT ( 'NONE',  ( 37.00000000000000711, 4.705694406421931860E-17, -3.469127814946512892E-15 ) ) ;
#861=CARTESIAN_POINT ( 'NONE',  ( 35.00000000000000000, 4.705694406421931860E-17, -3.469127814946512892E-15 ) ) ;
#864=CIRCLE ( 'NONE', #38023, 12.74999999999999822 ) ;
#865=EDGE_CURVE ( 'NONE', #65236, #8648, #45234, .T. ) ;
#867=ORIENTED_EDGE ( 'NONE', *, *, #9217, .F. ) ;
#870=CARTESIAN_POINT ( 'NONE',  ( 23.55206865562520946, -3.422725234784213200, -11.50504497094062550 ) ) ;
#872=CARTESIAN_POINT ( 'NONE',  ( -9.790055383657291443, 10.81845249703099299, -5.209507621916693587 ) ) ;
#873=CARTESIAN_POINT ( 'NONE',  ( -37.00000000000000711, 2.627174906296914525, 11.44858830469741129 ) ) ;
#876=VECTOR ( 'NONE', #40647, 1000.000000000000000 ) ;
#878=DIRECTION ( 'NONE',  ( 1.000000000000000000, 0.000000000000000000, -0.000000000000000000 ) ) ;
#879=ORIENTED_EDGE ( 'NONE', *, *, #58206, .T. ) ;
#880=AXIS2_PLACEMENT_3D ( 'NONE', #6476, #57343, #1160 ) ;
#882=CARTESIAN_POINT ( 'NONE',  ( -2.812344914800137818, -12.94091111974181452, 3.845999582511304471 ) ) ;
#884=EDGE_CURVE ( 'NONE', #59432, #13921, #39910, .T. ) ;
#885=DIRECTION ( 'NONE',  ( 1.000000000000000000, -0.000000000000000000, -0.000000000000000000 ) ) ;
#886=VERTEX_POINT ( 'NONE', #24230 ) ;
#887=CARTESIAN_POINT ( 'NONE',  ( -37.00000000000000711, 12.15823808070322798, 0.8294751490779768144 ) ) ;
#888=CARTESIAN_POINT ( 'NONE',  ( -37.00000000000000711, 7.608228585767727203, 10.23119532541075394 ) ) ;
#890=FACE_BOUND ( 'NONE', #11009, .T. ) ;
#891=EDGE_LOOP ( 'NONE', ( #65575, #20229, #17505, #23044 ) ) ;
#894=EDGE_CURVE ( 'NONE', #54998, #17169, #38397, .T. ) ;
#895=ORIENTED_EDGE ( 'NONE', *, *, #62262, .F. ) ;
#896=CARTESIAN_POINT ( 'NONE',  ( 37.00000000000000711, 12.46157735505189201, -2.696588552979104492 ) ) ;
#899=CARTESIAN_POINT ( 'NONE',  ( -37.00000000000000711, -9.733281772932221187, 8.235637554476612721 ) ) ;
#900=DIRECTION ( 'NONE',  ( 0.000000000000000000, 0.9105187689795969375, -0.4134677391718481476 ) ) ;
#902=AXIS2_PLACEMENT_3D ( 'NONE', #63159, #17287, #26597 ) ;
#905=ORIENTED_EDGE ( 'NONE', *, *, #34232, .T. ) ;
#906=CARTESIAN_POINT ( 'NONE',  ( -35.00000000000000000, -11.17622378668009020, 3.614449339633449387 ) ) ;
#908=EDGE_CURVE ( 'NONE', #45349, #45226, #9101, .T. ) ;
#909=CYLINDRICAL_SURFACE ( 'NONE', #28937, 4.999999999999999112 ) ;
#910=DIRECTION ( 'NONE',  ( 1.000000000000000000, 0.000000000000000000, 0.000000000000000000 ) ) ;
#911=CARTESIAN_POINT ( 'NONE',  ( -8.866453229254560142, 8.638462841324983543, -8.362614154885761764 ) ) ;
#912=DIRECTION ( 'NONE',  ( 0.000000000000000000, -0.3218879778916041157, 0.9467777615094549182 ) ) ;
#913=CARTESIAN_POINT ( 'NONE',  ( -18.04458733766117362, 11.34280559204706584, 3.916728392552376370 ) ) ;
#916=EDGE_CURVE ( 'NONE', #29332, #12123, #10240, .T. ) ;
#917=VECTOR ( 'NONE', #57645, 1000.000000000000000 ) ;
#919=ORIENTED_EDGE ( 'NONE', *, *, #8955, .T. ) ;
#920=DIRECTION ( 'NONE',  ( 0.000000000000000000, -0.01356324068818697166, 0.9999080150203988326 ) ) ;
#922=AXIS2_PLACEMENT_3D ( 'NONE', #48961, #13037, #52946 ) ;
#924=VERTEX_POINT ( 'NONE', #56460 ) ;
#925=DIRECTION ( 'NONE',  ( 1.000000000000000000, -0.000000000000000000, 0.000000000000000000 ) ) ;
#926=CARTESIAN_POINT ( 'NONE',  ( -14.51396536449455610, 7.857708026690540137, -10.97759357154228432 ) ) ;
#928=VECTOR ( 'NONE', #37946, 1000.000000000000000 ) ;
#931=EDGE_LOOP ( 'NONE', ( #4139, #42751, #11276, #57230 ) ) ;
#935=CIRCLE ( 'NONE', #32749, 5.000000000000000888 ) ;
#938=DIRECTION ( 'NONE',  ( -1.000000000000000000, -0.000000000000000000, 0.000000000000000000 ) ) ;
#943=FACE_OUTER_BOUND ( 'NONE', #16437, .T. ) ;
#944=CARTESIAN_POINT ( 'NONE',  ( 35.00000000000000000, -0.7214809346829402781, -11.72397916322012179 ) ) ;
#945=CARTESIAN_POINT ( 'NONE',  ( 28.71051995168708970, -9.891108990099938936, 6.797948428913199947 ) ) ;
#946=CARTESIAN_POINT ( 'NONE',  ( -5.393986094047766855, -1.427626268664394571, 11.91478156919506404 ) ) ;
#947=EDGE_CURVE ( 'NONE', #60093, #51437, #11236, .T. ) ;
#948=ADVANCED_FACE ( 'NONE', ( #65750 ), #31196, .T. ) ;
#949=ORIENTED_EDGE ( 'NONE', *, *, #54584, .F. ) ;
#950=EDGE_LOOP ( 'NONE', ( #25283, #63821, #8181, #28315 ) ) ;
#952=ORIENTED_EDGE ( 'NONE', *, *, #24463, .T. ) ;
#953=CARTESIAN_POINT ( 'NONE',  ( 35.00000000000000000, -9.430788938293991563, 7.718225330433904574 ) ) ;
#954=CARTESIAN_POINT ( 'NONE',  ( -36.00000000000000711, -12.02534193257724304, 4.237174932027182983 ) ) ;
#955=CARTESIAN_POINT ( 'NONE',  ( 2.798553295784531159, 25.00000000000000000, 7.462808788758677814 ) ) ;
#957=AXIS2_PLACEMENT_3D ( 'NONE', #6472, #26751, #47375 ) ;
#960=CARTESIAN_POINT ( 'NONE',  ( -8.908813177951650175, -2.340099471291562150, 11.77039042327342067 ) ) ;
#963=CARTESIAN_POINT ( 'NONE',  ( 37.00000000000000711, -9.913596905230170009, -8.017674001891752056 ) ) ;
#964=ORIENTED_EDGE ( 'NONE', *, *, #16319, .F. ) ;
#966=CARTESIAN_POINT ( 'NONE',  ( -37.00000000000000711, 2.772148766916116891, 11.86701198550357361 ) ) ;
#967=AXIS2_PLACEMENT_3D ( 'NONE', #4976, #11582, #20901 ) ;
#974=ORIENTED_EDGE ( 'NONE', *, *, #28534, .T. ) ;
#975=CARTESIAN_POINT ( 'NONE',  ( 35.00000000000000000, -11.07407352312215387, -3.916263239775311433 ) ) ;
#976=( BOUNDED_CURVE ( )  B_SPLINE_CURVE ( 3, ( #14907, #9952, #43298, #30235 ),
 .UNSPECIFIED., .F., .F. ) 
 B_SPLINE_CURVE_WITH_KNOTS ( ( 4, 4 ),
 ( 4.466372954730139178, 4.500313351398628647 ),
 .UNSPECIFIED. ) 
 CURVE ( )  GEOMETRIC_REPRESENTATION_ITEM ( )  RATIONAL_B_SPLINE_CURVE ( ( 1.000000000000000000, 0.9999040064266120353, 0.9999040064266120353, 1.000000000000000000 ) ) 
 REPRESENTATION_ITEM ( '' )  );
#977=LINE ( 'NONE', #51851, #49870 ) ;
#978=CARTESIAN_POINT ( 'NONE',  ( 47.00000000000000711, 4.705694406421931860E-17, -3.469127814946512892E-15 ) ) ;
#979=ORIENTED_EDGE ( 'NONE', *, *, #2691, .F. ) ;
#980=ORIENTED_EDGE ( 'NONE', *, *, #36684, .F. ) ;
#982=ADVANCED_FACE ( 'NONE', ( #30839 ), #5948, .T. ) ;
#985=ORIENTED_EDGE ( 'NONE', *, *, #43519, .T. ) ;
#986=EDGE_LOOP ( 'NONE', ( #31605, #32517, #57643, #11627 ) ) ;
#987=CIRCLE ( 'NONE', #55129, 12.18650000000000055 ) ;
#988=EDGE_LOOP ( 'NONE', ( #38920, #20606, #12540, #50252 ) ) ;
#991=CARTESIAN_POINT ( 'NONE',  ( 21.90174657591892071, -11.97747433400148864, -0.7349207973210698519 ) ) ;
#993=DIRECTION ( 'NONE',  ( 0.000000000000000000, 0.01356324068817998940, -0.9999080150203989437 ) ) ;
#994=ORIENTED_EDGE ( 'NONE', *, *, #57357, .F. ) ;
#995=DIRECTION ( 'NONE',  ( 1.000000000000000000, 0.000000000000000000, -0.000000000000000000 ) ) ;
#997=CARTESIAN_POINT ( 'NONE',  ( -37.00000000000000711, 4.339012074900111315, -10.91536515067643620 ) ) ;
#1004=FACE_OUTER_BOUND ( 'NONE', #17361, .T. ) ;
#1005=EDGE_CURVE ( 'NONE', #21005, #53943, #44133, .T. ) ;
#1009=ADVANCED_FACE ( 'NONE', ( #26854 ), #62740, .T. ) ;
#1010=AXIS2_PLACEMENT_3D ( 'NONE', #24968, #10626, #19322 ) ;
#1011=ORIENTED_EDGE ( 'NONE', *, *, #26962, .F. ) ;
#1014=CARTESIAN_POINT ( 'NONE',  ( 37.00000000000000711, 4.705694406421931860E-17, -3.469127814946512892E-15 ) ) ;
#1016=LINE ( 'NONE', #52861, #2253 ) ;
#1018=ORIENTED_EDGE ( 'NONE', *, *, #29438, .F. ) ;
#1019=DIRECTION ( 'NONE',  ( 0.000000000000000000, -0.01356324068818000848, 0.9999080150203990547 ) ) ;
#1020=FACE_OUTER_BOUND ( 'NONE', #1382, .T. ) ;
#1022=CARTESIAN_POINT ( 'NONE',  ( 22.12238245485356458, -12.73425672584572332, -4.485642937375443395 ) ) ;
#1023=B_SPLINE_CURVE_WITH_KNOTS ( 'NONE', 3,
 ( #2979, #13270, #33551, #28551, #65099, #65414, #61104, #15536, #44480, #45156, #24542, #30187 ),
 .UNSPECIFIED., .F., .F.,
 ( 4, 2, 2, 2, 2, 4 ),
 ( 1.734723475976807094E-18, 0.002074334512336499341, 0.003111501768504749445, 0.004148669024672999549, 0.006223003537009496287, 0.008297338049345992159 ),
 .UNSPECIFIED. ) ;
#1024=VECTOR ( 'NONE', #60903, 1000.000000000000000 ) ;
#1025=VECTOR ( 'NONE', #16569, 1000.000000000000000 ) ;
#1028=CARTESIAN_POINT ( 'NONE',  ( -35.00000000000000000, 11.98254675519231682, -2.220215194441768514 ) ) ;
#1029=CARTESIAN_POINT ( 'NONE',  ( 35.00000000000000000, -8.573591947375261313, 8.029056188533775895 ) ) ;
#1031=ADVANCED_FACE ( 'NONE', ( #43113 ), #42126, .T. ) ;
#1032=VERTEX_POINT ( 'NONE', #32477 ) ;
#1034=ORIENTED_EDGE ( 'NONE', *, *, #30537, .T. ) ;
#1038=DIRECTION ( 'NONE',  ( 0.000000000000000000, 0.01356324068817998940, -0.9999080150203990547 ) ) ;
#1039=ORIENTED_EDGE ( 'NONE', *, *, #46514, .F. ) ;
#1041=ORIENTED_EDGE ( 'NONE', *, *, #25305, .F. ) ;
#1045=AXIS2_PLACEMENT_3D ( 'NONE', #33482, #4199, #54087 ) ;
#1046=LINE ( 'NONE', #40617, #52317 ) ;
#1047=AXIS2_PLACEMENT_3D ( 'NONE', #27167, #17845, #32464 ) ;
#1048=ORIENTED_EDGE ( 'NONE', *, *, #11029, .T. ) ;
#1050=DIRECTION ( 'NONE',  ( 1.000000000000000000, 0.000000000000000000, 0.000000000000000000 ) ) ;
#1051=VERTEX_POINT ( 'NONE', #11553 ) ;
#1053=AXIS2_PLACEMENT_3D ( 'NONE', #55646, #61272, #35333 ) ;
#1055=CARTESIAN_POINT ( 'NONE',  ( 37.00000000000000711, 4.705694406421931860E-17, -3.469127814946512892E-15 ) ) ;
#1056=VERTEX_POINT ( 'NONE', #39108 ) ;
#1059=ORIENTED_EDGE ( 'NONE', *, *, #49853, .T. ) ;
#1063=AXIS2_PLACEMENT_3D ( 'NONE', #861, #10178, #41085 ) ;
#1066=DIRECTION ( 'NONE',  ( 1.000000000000000000, 0.000000000000000000, 0.000000000000000000 ) ) ;
#1067=CARTESIAN_POINT ( 'NONE',  ( -35.00000000000000000, -11.26103545359858060, 3.340853584269496412 ) ) ;
#1070=CARTESIAN_POINT ( 'NONE',  ( 7.309108772466194281, -6.069286178474166071, 12.06637494226818497 ) ) ;
#1071=ORIENTED_EDGE ( 'NONE', *, *, #40860, .F. ) ;
#1074=VERTEX_POINT ( 'NONE', #18846 ) ;
#1076=DIRECTION ( 'NONE',  ( 1.000000000000000000, 0.000000000000000000, 0.000000000000000000 ) ) ;
#1077=ORIENTED_EDGE ( 'NONE', *, *, #61845, .T. ) ;
#1078=FACE_OUTER_BOUND ( 'NONE', #64648, .T. ) ;
#1079=CARTESIAN_POINT ( 'NONE',  ( 37.00000000000000711, 4.705694406421931860E-17, -3.469127814946512892E-15 ) ) ;
#1080=AXIS2_PLACEMENT_3D ( 'NONE', #63758, #8253, #58147 ) ;
#1081=DIRECTION ( 'NONE',  ( 0.000000000000000000, 0.2006870767258889243, -0.9796553971857742127 ) ) ;
#1083=EDGE_CURVE ( 'NONE', #21740, #52529, #32443, .T. ) ;
#1085=ORIENTED_EDGE ( 'NONE', *, *, #1083, .F. ) ;
#1086=CARTESIAN_POINT ( 'NONE',  ( 37.00000000000000711, 6.415447294506860132, 11.01837265713066039 ) ) ;
#1090=DIRECTION ( 'NONE',  ( 0.000000000000000000, 0.5987040770935676548, -0.8009703041134167423 ) ) ;
#1094=LINE ( 'NONE', #21366, #20226 ) ;
#1095=CIRCLE ( 'NONE', #9555, 5.000000000000000000 ) ;
#1097=DIRECTION ( 'NONE',  ( -1.000000000000000000, 0.000000000000000000, 0.000000000000000000 ) ) ;
#1098=DIRECTION ( 'NONE',  ( 0.000000000000000000, 0.5472293298355214164, -0.8369827122275381726 ) ) ;
#1100=CARTESIAN_POINT ( 'NONE',  ( -27.45775109278351067, 25.00000000000000000, -8.471355351200609007 ) ) ;
#1103=VECTOR ( 'NONE', #57071, 1000.000000000000000 ) ;
#1105=ORIENTED_EDGE ( 'NONE', *, *, #29117, .F. ) ;
#1106=CARTESIAN_POINT ( 'NONE',  ( -17.13707773434846970, 7.268845792200386846, 11.37713557020030208 ) ) ;
#1107=CARTESIAN_POINT ( 'NONE',  ( -37.00000000000000711, 10.64792938439755510, 5.927257550915356887 ) ) ;
#1109=EDGE_CURVE ( 'NONE', #46540, #6959, #56926, .T. ) ;
#1112=CARTESIAN_POINT ( 'NONE',  ( -8.382709950485196515, 9.053270168017110819, -10.03930267771108475 ) ) ;
#1113=VERTEX_POINT ( 'NONE', #19502 ) ;
#1115=DIRECTION ( 'NONE',  ( 0.000000000000000000, -0.3807014730195085739, 0.9246979985058777496 ) ) ;
#1116=EDGE_LOOP ( 'NONE', ( #42630, #41333, #24812, #1836 ) ) ;
#1117=AXIS2_PLACEMENT_3D ( 'NONE', #41618, #17000, #31633 ) ;
#1120=ORIENTED_EDGE ( 'NONE', *, *, #9168, .T. ) ;
#1122=EDGE_LOOP ( 'NONE', ( #11131, #28574, #253, #22854 ) ) ;
#1125=DIRECTION ( 'NONE',  ( 1.000000000000000000, -0.000000000000000000, 0.000000000000000000 ) ) ;
#1129=DIRECTION ( 'NONE',  ( -1.000000000000000000, 0.000000000000000000, -0.000000000000000000 ) ) ;
#1132=DIRECTION ( 'NONE',  ( 1.000000000000000000, -0.000000000000000000, 0.000000000000000000 ) ) ;
#1135=CIRCLE ( 'NONE', #10652, 12.18649999999999878 ) ;
#1136=EDGE_CURVE ( 'NONE', #35622, #23170, #24469, .T. ) ;
#1138=CARTESIAN_POINT ( 'NONE',  ( 35.00000000000000000, 4.041347439436019151, 11.02904044024204211 ) ) ;
#1140=CARTESIAN_POINT ( 'NONE',  ( 24.48732188013169520, -8.567156455853016439, -8.406226182303409900 ) ) ;
#1141=CARTESIAN_POINT ( 'NONE',  ( 35.00000000000000000, -12.31350058095520339, 3.307597835713371737 ) ) ;
#1143=DIRECTION ( 'NONE',  ( 1.000000000000000000, 0.000000000000000000, -0.000000000000000000 ) ) ;
#1147=DIRECTION ( 'NONE',  ( 0.000000000000000000, 0.01356324068817998940, -0.9999080150203990547 ) ) ;
#1149=CARTESIAN_POINT ( 'NONE',  ( -19.63078887151198515, 11.93475341793434730, -1.289600524599101572 ) ) ;
#1151=ORIENTED_EDGE ( 'NONE', *, *, #37057, .T. ) ;
#1152=ORIENTED_EDGE ( 'NONE', *, *, #45461, .T. ) ;
#1153=CARTESIAN_POINT ( 'NONE',  ( 35.00000000000000000, 2.772148766916280316, 11.86701198550353098 ) ) ;
#1155=ORIENTED_EDGE ( 'NONE', *, *, #41410, .F. ) ;
#1156=CARTESIAN_POINT ( 'NONE',  ( 35.00000000000000000, -11.68758509253247091, 1.171570255487570655 ) ) ;
#1160=DIRECTION ( 'NONE',  ( 0.000000000000000000, 0.7790879021242529401, -0.6269146997507959451 ) ) ;
#1161=AXIS2_PLACEMENT_3D ( 'NONE', #49958, #33676, #43990 ) ;
#1162=EDGE_CURVE ( 'NONE', #12842, #47761, #3890, .T. ) ;
#1163=CIRCLE ( 'NONE', #38299, 4.999999999999999112 ) ;
#1165=CYLINDRICAL_SURFACE ( 'NONE', #49359, 12.74999999999999822 ) ;
#1166=CIRCLE ( 'NONE', #20287, 4.999999999999999112 ) ;
#1168=ORIENTED_EDGE ( 'NONE', *, *, #27101, .T. ) ;
#1170=B_SPLINE_CURVE_WITH_KNOTS ( 'NONE', 3,
 ( #43101, #1589, #42425, #52771, #17191, #57774, #63376, #17844, #47780, #2231, #42772, #63066, #37796, #58090, #12505, #32780 ),
 .UNSPECIFIED., .F., .F.,
 ( 4, 2, 2, 2, 2, 2, 2, 4 ),
 ( 0.000000000000000000, 0.001069476264344462095, 0.002138952528688924191, 0.003208428793033386069, 0.004277905057377848382, 0.005347381321722308525, 0.006416857586066768669, 0.008555810114755681151 ),
 .UNSPECIFIED. ) ;
#1173=EDGE_CURVE ( 'NONE', #14200, #27538, #25441, .T. ) ;
#1174=CYLINDRICAL_SURFACE ( 'NONE', #20700, 12.18650000000000055 ) ;
#1175=DIRECTION ( 'NONE',  ( -0.5551681190699946367, -0.8317381556525372810, 0.000000000000000000 ) ) ;
#1177=CARTESIAN_POINT ( 'NONE',  ( 23.98848397398876386, -2.635302845098066005, -13.24129003998613818 ) ) ;
#1184=DIRECTION ( 'NONE',  ( 0.000000000000000000, 0.01356324068817998940, -0.9999080150203990547 ) ) ;
#1187=AXIS2_PLACEMENT_3D ( 'NONE', #38821, #13847, #54458 ) ;
#1188=CYLINDRICAL_SURFACE ( 'NONE', #10759, 12.18649999999999878 ) ;
#1189=ADVANCED_FACE ( 'NONE', ( #24151 ), #60062, .T. ) ;
#1190=ORIENTED_EDGE ( 'NONE', *, *, #47667, .T. ) ;
#1191=VECTOR ( 'NONE', #8769, 1000.000000000000000 ) ;
#1192=DIRECTION ( 'NONE',  ( 0.000000000000000000, -0.01356324068817991828, 0.9999080150203990547 ) ) ;
#1193=CARTESIAN_POINT ( 'NONE',  ( 35.00000000000000000, 4.705694406421931860E-17, -3.469127814946512892E-15 ) ) ;
#1194=CARTESIAN_POINT ( 'NONE',  ( -37.00000000000000711, 9.557269938331666381, -7.561043153947866635 ) ) ;
#1196=ADVANCED_FACE ( 'NONE', ( #49754 ), #20478, .T. ) ;
#1198=DIRECTION ( 'NONE',  ( 1.000000000000000000, -0.000000000000000000, 0.000000000000000000 ) ) ;
#1199=DIRECTION ( 'NONE',  ( 0.000000000000000000, 0.01356324068817998940, -0.9999080150203990547 ) ) ;
#1204=CIRCLE ( 'NONE', #54337, 12.74999999999999822 ) ;
#1208=AXIS2_PLACEMENT_3D ( 'NONE', #4040, #59247, #13668 ) ;
#1211=FACE_OUTER_BOUND ( 'NONE', #48333, .T. ) ;
#1212=CARTESIAN_POINT ( 'NONE',  ( -3.937012649977812195, -11.99793950917781871, 6.201358434801304220 ) ) ;
#1214=AXIS2_PLACEMENT_3D ( 'NONE', #38750, #59356, #48734 ) ;
#1215=DIRECTION ( 'NONE',  ( -1.000000000000000000, 0.000000000000000000, 0.000000000000000000 ) ) ;
#1216=DIRECTION ( 'NONE',  ( 1.000000000000000000, 0.000000000000000000, -0.000000000000000000 ) ) ;
#1217=EDGE_LOOP ( 'NONE', ( #62554, #41264, #18470, #150 ) ) ;
#1219=ORIENTED_EDGE ( 'NONE', *, *, #23759, .T. ) ;
#1220=CARTESIAN_POINT ( 'NONE',  ( 36.00000000000000711, -7.379373053628790480, 10.39746860227898395 ) ) ;
#1221=AXIS2_PLACEMENT_3D ( 'NONE', #48517, #2969, #43494 ) ;
#1224=DIRECTION ( 'NONE',  ( -0.000000000000000000, -0.000000000000000000, -1.000000000000000000 ) ) ;
#1225=CARTESIAN_POINT ( 'NONE',  ( -18.08686583997241115, 5.151216734910855521, 10.83812558286605920 ) ) ;
#1226=DIRECTION ( 'NONE',  ( -1.000000000000000000, -0.000000000000000000, 0.000000000000000000 ) ) ;
#1228=DIRECTION ( 'NONE',  ( 0.000000000000000000, 0.8989688749565143411, 0.4380125133594006681 ) ) ;
#1229=CARTESIAN_POINT ( 'NONE',  ( -32.00000000000000711, -12.00000000000000000, 0.000000000000000000 ) ) ;
#1232=EDGE_LOOP ( 'NONE', ( #11511, #7631, #29856, #47653 ) ) ;
#1233=CARTESIAN_POINT ( 'NONE',  ( 27.63711073776143223, -12.51469113205075168, 5.065401719838317440 ) ) ;
#1235=AXIS2_PLACEMENT_3D ( 'NONE', #2780, #48642, #58287 ) ;
#1236=ORIENTED_EDGE ( 'NONE', *, *, #57082, .T. ) ;
#1237=CARTESIAN_POINT ( 'NONE',  ( 21.94266139820581429, -11.68884937910924293, -2.741396137623683948 ) ) ;
#1239=DIRECTION ( 'NONE',  ( 1.000000000000000000, 0.000000000000000000, 0.000000000000000000 ) ) ;
#1241=VECTOR ( 'NONE', #6426, 1000.000000000000000 ) ;
#1242=AXIS2_PLACEMENT_3D ( 'NONE', #60511, #15295, #41533 ) ;
#1244=CARTESIAN_POINT ( 'NONE',  ( 35.00000000000000000, -4.986700593229777212, -10.63508530065520219 ) ) ;
#1245=VECTOR ( 'NONE', #6917, 1000.000000000000000 ) ;
#1247=EDGE_LOOP ( 'NONE', ( #2779, #5008, #62184, #20386 ) ) ;
#1248=CARTESIAN_POINT ( 'NONE',  ( -35.00000000000000000, 0.000000000000000000, 0.000000000000000000 ) ) ;
#1249=VERTEX_POINT ( 'NONE', #5189 ) ;
#1250=DIRECTION ( 'NONE',  ( 0.000000000000000000, 0.07632122047556488820, -0.9970832820307038435 ) ) ;
#1251=LINE ( 'NONE', #62721, #48697 ) ;
#1252=CARTESIAN_POINT ( 'NONE',  ( 26.08439714455133185, -12.97057518889163674, 3.743551691817328386 ) ) ;
#1253=CARTESIAN_POINT ( 'NONE',  ( 35.00000000000000000, -5.921969905510278132, 10.14408668126219304 ) ) ;
#1254=DIRECTION ( 'NONE',  ( 1.000000000000000000, 0.000000000000000000, 0.000000000000000000 ) ) ;
#1257=AXIS2_PLACEMENT_3D ( 'NONE', #41429, #62068, #5570 ) ;
#1258=ORIENTED_EDGE ( 'NONE', *, *, #38065, .T. ) ;
#1259=EDGE_CURVE ( 'NONE', #40664, #61618, #26125, .T. ) ;
#1261=EDGE_LOOP ( 'NONE', ( #2127, #37907, #43374, #41136 ) ) ;
#1270=ORIENTED_EDGE ( 'NONE', *, *, #14859, .T. ) ;
#1272=DIRECTION ( 'NONE',  ( 0.000000000000000000, 0.01356324068817991828, -0.9999080150203990547 ) ) ;
#1273=VECTOR ( 'NONE', #55372, 1000.000000000000000 ) ;
#1277=CARTESIAN_POINT ( 'NONE',  ( 35.00000000000000000, 6.891188680298960811, 9.512294188640820991 ) ) ;
#1280=VERTEX_POINT ( 'NONE', #10480 ) ;
#1284=EDGE_CURVE ( 'NONE', #44262, #34193, #56371, .T. ) ;
#1286=CARTESIAN_POINT ( 'NONE',  ( 37.00000000000000711, 12.18359334611896294, 0.2661492558803733588 ) ) ;
#1290=CIRCLE ( 'NONE', #40516, 5.000000000000000888 ) ;
#1291=CIRCLE ( 'NONE', #35191, 12.75000000000000178 ) ;
#1293=ADVANCED_FACE ( 'NONE', ( #5868 ), #46400, .T. ) ;
#1294=VERTEX_POINT ( 'NONE', #16138 ) ;
#1295=LINE ( 'NONE', #635, #38213 ) ;
#1296=ORIENTED_EDGE ( 'NONE', *, *, #64814, .F. ) ;
#1297=CARTESIAN_POINT ( 'NONE',  ( -35.00000000000000000, -3.916263239775430005, 11.07407352312211302 ) ) ;
#1298=CARTESIAN_POINT ( 'NONE',  ( 2.311395794103597190, 2.385532211604124431, -13.30448733390617200 ) ) ;
#1299=DIRECTION ( 'NONE',  ( 0.000000000000000000, 0.9651210252299786685, 0.2618041379715667083 ) ) ;
#1303=CARTESIAN_POINT ( 'NONE',  ( -34.00000000000000000, 1.836970198721035357E-16, 0.000000000000000000 ) ) ;
#1305=ORIENTED_EDGE ( 'NONE', *, *, #43787, .F. ) ;
#1307=ORIENTED_EDGE ( 'NONE', *, *, #42679, .F. ) ;
#1308=CARTESIAN_POINT ( 'NONE',  ( 35.00000000000000000, 11.30684963584395675, 4.545979934229284147 ) ) ;
#1309=AXIS2_PLACEMENT_3D ( 'NONE', #24829, #20155, #14812 ) ;
#1310=CARTESIAN_POINT ( 'NONE',  ( 37.00000000000000711, -11.68758509253247091, 1.171570255487570655 ) ) ;
#1313=CARTESIAN_POINT ( 'NONE',  ( 37.00000000000000711, -11.23004253107767880, -4.732539170486222524 ) ) ;
#1315=CARTESIAN_POINT ( 'NONE',  ( 37.00000000000000711, -12.18632975068352664, -0.06441628369832411161 ) ) ;
#1320=EDGE_LOOP ( 'NONE', ( #39520, #12299, #58562, #58515 ) ) ;
#1321=ADVANCED_FACE ( 'NONE', ( #63314 ), #37395, .T. ) ;
#1322=CARTESIAN_POINT ( 'NONE',  ( 1.557635548354367794, 1.399767314629970505, 13.43135513698036299 ) ) ;
#1326=VERTEX_POINT ( 'NONE', #28096 ) ;
#1330=CARTESIAN_POINT ( 'NONE',  ( -20.34666746044321073, -11.74305062490097029, -2.487411478320596725 ) ) ;
#1331=CARTESIAN_POINT ( 'NONE',  ( -25.86628395826706850, 8.041618865309581921, 10.84354029019568522 ) ) ;
#1332=FACE_OUTER_BOUND ( 'NONE', #7494, .T. ) ;
#1333=ORIENTED_EDGE ( 'NONE', *, *, #46244, .T. ) ;
#1335=AXIS2_PLACEMENT_3D ( 'NONE', #32137, #48122, #7196 ) ;
#1336=VERTEX_POINT ( 'NONE', #43038 ) ;
#1337=DIRECTION ( 'NONE',  ( -1.000000000000000000, 0.000000000000000000, 0.000000000000000000 ) ) ;
#1339=DIRECTION ( 'NONE',  ( 0.000000000000000000, -0.01356324068817999114, 0.9999080150203989437 ) ) ;
#1342=CIRCLE ( 'NONE', #7733, 5.000000000000000000 ) ;
#1343=CIRCLE ( 'NONE', #26811, 4.999999999999999112 ) ;
#1344=ADVANCED_FACE ( 'NONE', ( #48392 ), #32400, .T. ) ;
#1345=AXIS2_PLACEMENT_3D ( 'NONE', #49197, #64138, #59165 ) ;
#1348=VERTEX_POINT ( 'NONE', #6497 ) ;
#1349=FACE_OUTER_BOUND ( 'NONE', #63831, .T. ) ;
#1353=CARTESIAN_POINT ( 'NONE',  ( -37.00000000000000711, 12.31350058095527977, -3.307597835713114609 ) ) ;
#1354=ORIENTED_EDGE ( 'NONE', *, *, #49116, .T. ) ;
#1355=EDGE_CURVE ( 'NONE', #63364, #34567, #51610, .T. ) ;
#1356=CARTESIAN_POINT ( 'NONE',  ( 36.00000000000000711, -12.02534193257717732, 4.237174932027350849 ) ) ;
#1358=CARTESIAN_POINT ( 'NONE',  ( -37.00000000000000711, 0.000000000000000000, 0.000000000000000000 ) ) ;
#1360=AXIS2_PLACEMENT_3D ( 'NONE', #14903, #24921, #60155 ) ;
#1362=CARTESIAN_POINT ( 'NONE',  ( -37.00000000000000711, 9.063649021439076137, -8.146229107149299153 ) ) ;
#1363=CIRCLE ( 'NONE', #62902, 4.999999999999999112 ) ;
#1364=CARTESIAN_POINT ( 'NONE',  ( -35.00000000000000000, 3.645068577060182946, -11.16627499335651130 ) ) ;
#1365=EDGE_CURVE ( 'NONE', #54583, #6133, #31419, .T. ) ;
#1367=DIRECTION ( 'NONE',  ( 1.000000000000000000, -0.000000000000000000, 0.000000000000000000 ) ) ;
#1370=AXIS2_PLACEMENT_3D ( 'NONE', #58301, #28044, #48656 ) ;
#1372=( BOUNDED_CURVE ( )  B_SPLINE_CURVE ( 3, ( #42728, #17809, #52740, #7164 ),
 .UNSPECIFIED., .F., .F. ) 
 B_SPLINE_CURVE_WITH_KNOTS ( ( 4, 4 ),
 ( 4.409534938676864968, 4.430491180286858288 ),
 .UNSPECIFIED. ) 
 CURVE ( )  GEOMETRIC_REPRESENTATION_ITEM ( )  RATIONAL_B_SPLINE_CURVE ( ( 1.000000000000000000, 0.9999634033296326274, 0.9999634033296326274, 1.000000000000000000 ) ) 
 REPRESENTATION_ITEM ( '' )  );
#1376=ADVANCED_FACE ( 'NONE', ( #27415 ), #62998, .T. ) ;
#1378=ORIENTED_EDGE ( 'NONE', *, *, #20910, .F. ) ;
#1381=ORIENTED_EDGE ( 'NONE', *, *, #64814, .T. ) ;
#1382=EDGE_LOOP ( 'NONE', ( #26703, #19641, #8896, #19929 ) ) ;
#1383=DIRECTION ( 'NONE',  ( -1.000000000000000000, -0.000000000000000000, 0.000000000000000000 ) ) ;
#1386=CARTESIAN_POINT ( 'NONE',  ( -35.00000000000000000, 11.68758509253248334, -1.171570255487489609 ) ) ;
#1387=AXIS2_PLACEMENT_3D ( 'NONE', #21736, #33335, #27348 ) ;
#1388=EDGE_LOOP ( 'NONE', ( #16752, #1462, #26249, #1120 ) ) ;
#1389=EDGE_CURVE ( 'NONE', #56717, #10498, #42052, .T. ) ;
#1390=LINE ( 'NONE', #6701, #43213 ) ;
#1391=ADVANCED_FACE ( 'NONE', ( #57364 ), #22783, .T. ) ;
#1392=DIRECTION ( 'NONE',  ( -1.000000000000000000, 0.000000000000000000, 0.000000000000000000 ) ) ;
#1393=VERTEX_POINT ( 'NONE', #52389 ) ;
#1394=DIRECTION ( 'NONE',  ( -1.000000000000000000, 0.000000000000000000, 0.000000000000000000 ) ) ;
#1396=CARTESIAN_POINT ( 'NONE',  ( 22.88594695219327235, -4.822122601967141264, 10.98850006195556261 ) ) ;
#1398=EDGE_CURVE ( 'NONE', #41624, #60517, #38382, .T. ) ;
#1402=CIRCLE ( 'NONE', #65067, 12.18650000000000055 ) ;
#1403=CARTESIAN_POINT ( 'NONE',  ( -17.99580626142726913, -9.062273765671413628, 10.02044534816332444 ) ) ;
#1404=FACE_OUTER_BOUND ( 'NONE', #7670, .T. ) ;
#1407=DIRECTION ( 'NONE',  ( 1.000000000000000000, 0.000000000000000000, 0.000000000000000000 ) ) ;
#1408=CARTESIAN_POINT ( 'NONE',  ( 9.378405691591813920, 1.708243947577828603, 11.87965240138111334 ) ) ;
#1410=CARTESIAN_POINT ( 'NONE',  ( -37.00000000000000711, 4.074242145636005397, 12.08151691381191917 ) ) ;
#1412=LINE ( 'NONE', #16368, #43875 ) ;
#1413=ORIENTED_EDGE ( 'NONE', *, *, #32374, .T. ) ;
#1414=DIRECTION ( 'NONE',  ( -1.000000000000000000, 0.000000000000000000, 0.000000000000000000 ) ) ;
#1415=AXIS2_PLACEMENT_3D ( 'NONE', #34083, #430, #18818 ) ;
#1420=DIRECTION ( 'NONE',  ( -0.000000000000000000, -0.000000000000000000, -1.000000000000000000 ) ) ;
#1421=DIRECTION ( 'NONE',  ( 0.000000000000000000, -0.2355298848897586506, -0.9718671068226442111 ) ) ;
#1424=EDGE_CURVE ( 'NONE', #59191, #52452, #53699, .T. ) ;
#1425=VECTOR ( 'NONE', #15661, 1000.000000000000000 ) ;
#1427=CARTESIAN_POINT ( 'NONE',  ( -17.22487315615078529, -6.630673841149409498, -10.00324445667050632 ) ) ;
#1428=ORIENTED_EDGE ( 'NONE', *, *, #17508, .T. ) ;
#1430=DIRECTION ( 'NONE',  ( 0.000000000000000000, 0.01356324068817991828, -0.9999080150203990547 ) ) ;
#1431=DIRECTION ( 'NONE',  ( -1.000000000000000000, 0.000000000000000000, 0.000000000000000000 ) ) ;
#1432=ORIENTED_EDGE ( 'NONE', *, *, #31378, .F. ) ;
#1433=AXIS2_PLACEMENT_3D ( 'NONE', #57152, #60822, #5639 ) ;
#1435=AXIS2_PLACEMENT_3D ( 'NONE', #4838, #49720, #160 ) ;
#1437=AXIS2_PLACEMENT_3D ( 'NONE', #13118, #38721, #7136 ) ;
#1438=AXIS2_PLACEMENT_3D ( 'NONE', #54853, #24588, #58891 ) ;
#1439=CARTESIAN_POINT ( 'NONE',  ( 25.05309951391468459, -8.823569016628452388, -8.132934882857099979 ) ) ;
#1440=FACE_OUTER_BOUND ( 'NONE', #7234, .T. ) ;
#1441=CIRCLE ( 'NONE', #47057, 12.74999999999999822 ) ;
#1442=CARTESIAN_POINT ( 'NONE',  ( -47.00000000000000711, 0.000000000000000000, 0.000000000000000000 ) ) ;
#1443=DIRECTION ( 'NONE',  ( 0.000000000000000000, 0.01356324068817998593, -0.9999080150203990547 ) ) ;
#1445=CARTESIAN_POINT ( 'NONE',  ( -35.00000000000000000, 8.029056188533687077, 8.573591947375351907 ) ) ;
#1446=CARTESIAN_POINT ( 'NONE',  ( 3.459614771489464946, -11.09853614738469396, -4.563167253695070258 ) ) ;
#1448=AXIS2_PLACEMENT_3D ( 'NONE', #48467, #3236, #53776 ) ;
#1449=EDGE_CURVE ( 'NONE', #61567, #28743, #13368, .T. ) ;
#1450=AXIS2_PLACEMENT_3D ( 'NONE', #48727, #3181, #23447 ) ;
#1451=ORIENTED_EDGE ( 'NONE', *, *, #30996, .F. ) ;
#1452=CARTESIAN_POINT ( 'NONE',  ( -17.69390680376402258, 6.600471761193754894, 11.77845348364601996 ) ) ;
#1453=DIRECTION ( 'NONE',  ( -1.000000000000000000, 0.000000000000000000, -0.000000000000000000 ) ) ;
#1454=ORIENTED_EDGE ( 'NONE', *, *, #58874, .T. ) ;
#1458=ORIENTED_EDGE ( 'NONE', *, *, #55303, .T. ) ;
#1459=CARTESIAN_POINT ( 'NONE',  ( -35.00000000000000000, 12.00000000000000000, 1.469576158976823947E-15 ) ) ;
#1461=CARTESIAN_POINT ( 'NONE',  ( -35.00000000000000000, -12.63095688309030251, 1.738225594539951180 ) ) ;
#1462=ORIENTED_EDGE ( 'NONE', *, *, #37652, .F. ) ;
#1463=ORIENTED_EDGE ( 'NONE', *, *, #41590, .T. ) ;
#1465=EDGE_CURVE ( 'NONE', #23780, #54185, #42038, .T. ) ;
#1467=AXIS2_PLACEMENT_3D ( 'NONE', #21914, #47200, #23554 ) ;
#1468=ORIENTED_EDGE ( 'NONE', *, *, #58715, .T. ) ;
#1469=EDGE_CURVE ( 'NONE', #55989, #47412, #52698, .T. ) ;
#1470=CARTESIAN_POINT ( 'NONE',  ( -24.82451523953541894, -8.749778939910779485, 8.214417963206811280 ) ) ;
#1472=CYLINDRICAL_SURFACE ( 'NONE', #36511, 12.18650000000000055 ) ;
#1473=DIRECTION ( 'NONE',  ( -0.000000000000000000, -1.000000000000000000, -0.000000000000000000 ) ) ;
#1474=VERTEX_POINT ( 'NONE', #29386 ) ;
#1478=CARTESIAN_POINT ( 'NONE',  ( -24.30326519513172912, 8.383402268046477701, 8.588829520052238209 ) ) ;
#1484=DIRECTION ( 'NONE',  ( 1.000000000000000000, 0.000000000000000000, 0.000000000000000000 ) ) ;
#1485=AXIS2_PLACEMENT_3D ( 'NONE', #4253, #44462, #34500 ) ;
#1487=EDGE_LOOP ( 'NONE', ( #40463, #44615, #58905, #31420 ) ) ;
#1488=CARTESIAN_POINT ( 'NONE',  ( 23.33049619018955312, -9.351986643931601506, -7.526857238819390616 ) ) ;
#1492=DIRECTION ( 'NONE',  ( 0.000000000000000000, 0.01356324068817998940, -0.9999080150203990547 ) ) ;
#1493=EDGE_CURVE ( 'NONE', #46522, #8559, #53740, .T. ) ;
#1494=DIRECTION ( 'NONE',  ( 0.000000000000000000, -0.01356324068817998940, 0.9999080150203990547 ) ) ;
#1496=ORIENTED_EDGE ( 'NONE', *, *, #9929, .F. ) ;
#1497=AXIS2_PLACEMENT_3D ( 'NONE', #59919, #25635, #9334 ) ;
#1501=AXIS2_PLACEMENT_3D ( 'NONE', #3959, #28890, #49202 ) ;
#1502=VERTEX_POINT ( 'NONE', #59660 ) ;
#1503=AXIS2_PLACEMENT_3D ( 'NONE', #7546, #12863, #16874 ) ;
#1504=DIRECTION ( 'NONE',  ( 1.000000000000000000, 0.000000000000000000, 0.000000000000000000 ) ) ;
#1507=DIRECTION ( 'NONE',  ( 1.000000000000000000, 0.000000000000000000, 0.000000000000000000 ) ) ;
#1508=LINE ( 'NONE', #21785, #38033 ) ;
#1509=CIRCLE ( 'NONE', #9928, 5.000000000000000888 ) ;
#1510=CARTESIAN_POINT ( 'NONE',  ( -9.424604252909290381, -2.780242171103320725, -11.67835095153480651 ) ) ;
#1512=EDGE_CURVE ( 'NONE', #38977, #43321, #21885, .T. ) ;
#1513=ORIENTED_EDGE ( 'NONE', *, *, #62573, .T. ) ;
#1514=VECTOR ( 'NONE', #11526, 1000.000000000000000 ) ;
#1515=DIRECTION ( 'NONE',  ( 0.000000000000000000, 0.01356324068817992175, -0.9999080150203990547 ) ) ;
#1516=CARTESIAN_POINT ( 'NONE',  ( -3.700366998126892071, -10.78403306819907037, 5.280571526603965005 ) ) ;
#1520=CARTESIAN_POINT ( 'NONE',  ( 35.00000000000000000, -11.60979404548631777, 3.704519465651427534 ) ) ;
#1521=DIRECTION ( 'NONE',  ( -1.000000000000000000, -0.000000000000000000, 0.000000000000000000 ) ) ;
#1522=CARTESIAN_POINT ( 'NONE',  ( 8.459345231580508440, 3.955827861842277748, -11.33263784498325322 ) ) ;
#1524=VERTEX_POINT ( 'NONE', #24080 ) ;
#1527=AXIS2_PLACEMENT_3D ( 'NONE', #57874, #11963, #21638 ) ;
#1528=DIRECTION ( 'NONE',  ( -1.000000000000000000, 0.000000000000000000, 0.000000000000000000 ) ) ;
#1532=CARTESIAN_POINT ( 'NONE',  ( 12.03570575446059365, 0.5714357744993003863, -13.48808386659669090 ) ) ;
#1533=DIRECTION ( 'NONE',  ( 0.000000000000000000, 0.9987865678893278476, -0.04924826701374234589 ) ) ;
#1535=ORIENTED_EDGE ( 'NONE', *, *, #11385, .T. ) ;
#1537=DIRECTION ( 'NONE',  ( -1.000000000000000000, 0.000000000000000000, 0.000000000000000000 ) ) ;
#1539=VERTEX_POINT ( 'NONE', #34687 ) ;
#1540=CARTESIAN_POINT ( 'NONE',  ( -8.891032880924175430, -12.93614229090407974, -3.860857758255645589 ) ) ;
#1543=CIRCLE ( 'NONE', #56749, 4.999999999999999112 ) ;
#1545=ORIENTED_EDGE ( 'NONE', *, *, #49357, .T. ) ;
#1546=CARTESIAN_POINT ( 'NONE',  ( -37.00000000000000711, 0.000000000000000000, 0.000000000000000000 ) ) ;
#1548=DIRECTION ( 'NONE',  ( 0.000000000000000000, 0.1740410799127544150, 0.9847383929261631641 ) ) ;
#1549=EDGE_LOOP ( 'NONE', ( #57812, #3118, #14716, #20448, #33194, #50371 ) ) ;
#1552=DIRECTION ( 'NONE',  ( 0.000000000000000000, -0.8515178078024812081, 0.5243256840888652626 ) ) ;
#1559=ORIENTED_EDGE ( 'NONE', *, *, #44651, .T. ) ;
#1560=VERTEX_POINT ( 'NONE', #36338 ) ;
#1561=CARTESIAN_POINT ( 'NONE',  ( -37.00000000000000711, 11.26103545359856106, -3.340853584269573684 ) ) ;
#1566=AXIS2_PLACEMENT_3D ( 'NONE', #49824, #8597, #40146 ) ;
#1567=CARTESIAN_POINT ( 'NONE',  ( 35.00000000000000000, -10.70999494708488520, 5.814360711498399503 ) ) ;
#1568=ORIENTED_EDGE ( 'NONE', *, *, #10098, .T. ) ;
#1571=CARTESIAN_POINT ( 'NONE',  ( -37.00000000000000711, 0.000000000000000000, 0.000000000000000000 ) ) ;
#1572=ORIENTED_EDGE ( 'NONE', *, *, #64314, .T. ) ;
#1573=ORIENTED_EDGE ( 'NONE', *, *, #28751, .T. ) ;
#1575=AXIS2_PLACEMENT_3D ( 'NONE', #57977, #37341, #41999 ) ;
#1576=ORIENTED_EDGE ( 'NONE', *, *, #65162, .F. ) ;
#1579=DIRECTION ( 'NONE',  ( 0.000000000000000000, 0.5243256840888563808, 0.8515178078024868702 ) ) ;
#1581=CARTESIAN_POINT ( 'NONE',  ( -35.00000000000000000, 8.854740511458851770, 7.717887834988275131 ) ) ;
#1582=CARTESIAN_POINT ( 'NONE',  ( 37.00000000000000711, -0.3025107581130382917, 11.74226168163341022 ) ) ;
#1584=ADVANCED_FACE ( 'NONE', ( #50355 ), #16049, .T. ) ;
#1585=VERTEX_POINT ( 'NONE', #30683 ) ;
#1587=VERTEX_POINT ( 'NONE', #41315 ) ;
#1588=CARTESIAN_POINT ( 'NONE',  ( 145.1370849898475797, 3.309064568108273190E-14, 0.000000000000000000 ) ) ;
#1589=CARTESIAN_POINT ( 'NONE',  ( -9.027317351555117497, -12.84017734719011727, -4.182396712693398300 ) ) ;
#1590=AXIS2_PLACEMENT_3D ( 'NONE', #52840, #62468, #52200 ) ;
#1591=CARTESIAN_POINT ( 'NONE',  ( -7.181456785175555524, 5.890186129966279438, -10.45493698471458188 ) ) ;
#1595=VECTOR ( 'NONE', #34066, 1000.000000000000000 ) ;
#1596=ORIENTED_EDGE ( 'NONE', *, *, #24861, .F. ) ;
#1597=VERTEX_POINT ( 'NONE', #55314 ) ;
#1600=ORIENTED_EDGE ( 'NONE', *, *, #54426, .F. ) ;
#1601=CYLINDRICAL_SURFACE ( 'NONE', #4382, 4.999999999999999112 ) ;
#1602=CARTESIAN_POINT ( 'NONE',  ( -15.22041587299536580, 7.970357817492780939, -10.89607067939092921 ) ) ;
#1603=CARTESIAN_POINT ( 'NONE',  ( 35.00000000000000000, -8.295159312811920316, -8.927548052240867449 ) ) ;
#1605=EDGE_CURVE ( 'NONE', #5918, #64188, #25380, .T. ) ;
#1606=ORIENTED_EDGE ( 'NONE', *, *, #38771, .T. ) ;
#1608=CYLINDRICAL_SURFACE ( 'NONE', #8785, 4.999999999999999112 ) ;
#1611=CIRCLE ( 'NONE', #16463, 12.74999999999999822 ) ;
#1612=CARTESIAN_POINT ( 'NONE',  ( -19.69476066079020171, -4.201994156881551312, 12.82938989607585789 ) ) ;
#1613=DIRECTION ( 'NONE',  ( 0.000000000000000000, 0.4935949184179201366, -0.8696919319575218132 ) ) ;
#1615=DIRECTION ( 'NONE',  ( 0.000000000000000000, 0.01356324068817998940, -0.9999080150203990547 ) ) ;
#1616=EDGE_LOOP ( 'NONE', ( #3027, #44782, #54567, #22064 ) ) ;
#1617=LINE ( 'NONE', #46492, #47192 ) ;
#1618=DIRECTION ( 'NONE',  ( -1.000000000000000000, -0.000000000000000000, 0.000000000000000000 ) ) ;
#1621=CARTESIAN_POINT ( 'NONE',  ( -10.41597200609069596, -5.095536857955488941, 10.87159232434287048 ) ) ;
#1622=ORIENTED_EDGE ( 'NONE', *, *, #18904, .T. ) ;
#1623=VERTEX_POINT ( 'NONE', #20397 ) ;
#1626=FACE_OUTER_BOUND ( 'NONE', #59385, .T. ) ;
#1627=CARTESIAN_POINT ( 'NONE',  ( 3.221585903514446514, 4.631497350863631901, -12.68724791558186737 ) ) ;
#1628=AXIS2_PLACEMENT_3D ( 'NONE', #62830, #62492, #53855 ) ;
#1629=CARTESIAN_POINT ( 'NONE',  ( 35.00000000000000000, 0.4871980014161481631, -12.74068829017554272 ) ) ;
#1632=FACE_OUTER_BOUND ( 'NONE', #13235, .T. ) ;
#1635=EDGE_CURVE ( 'NONE', #18994, #21897, #55971, .T. ) ;
#1637=EDGE_LOOP ( 'NONE', ( #29744, #46586, #63482, #8654 ) ) ;
#1639=CARTESIAN_POINT ( 'NONE',  ( 35.00000000000000000, 4.705694406421931860E-17, -3.469127814946512892E-15 ) ) ;
#1640=AXIS2_PLACEMENT_3D ( 'NONE', #55925, #40284, #5392 ) ;
#1641=CYLINDRICAL_SURFACE ( 'NONE', #30194, 12.18649999999999878 ) ;
#1645=ORIENTED_EDGE ( 'NONE', *, *, #22512, .F. ) ;
#1646=CARTESIAN_POINT ( 'NONE',  ( 35.00000000000000000, -12.16632754454236043, 0.7008968033240018380 ) ) ;
#1647=CARTESIAN_POINT ( 'NONE',  ( -35.00000000000000000, -3.473736367725171359, -12.26766708251995475 ) ) ;
#1648=CARTESIAN_POINT ( 'NONE',  ( 35.00000000000000000, 6.946017217730082294, 10.01317267707878500 ) ) ;
#1650=VERTEX_POINT ( 'NONE', #65597 ) ;
#1651=CARTESIAN_POINT ( 'NONE',  ( 2.676981048097610394, 3.126245636041473652, 13.13819726198281401 ) ) ;
#1652=ORIENTED_EDGE ( 'NONE', *, *, #36627, .F. ) ;
#1656=ORIENTED_EDGE ( 'NONE', *, *, #24245, .F. ) ;
#1657=FACE_OUTER_BOUND ( 'NONE', #27220, .T. ) ;
#1659=CIRCLE ( 'NONE', #59005, 12.74999999999999822 ) ;
#1660=ADVANCED_FACE ( 'NONE', ( #46334 ), #20072, .T. ) ;
#1661=DIRECTION ( 'NONE',  ( 0.000000000000000000, -0.01356324068817991828, 0.9999080150203990547 ) ) ;
#1663=DIRECTION ( 'NONE',  ( 1.000000000000000000, 0.000000000000000000, 0.000000000000000000 ) ) ;
#1664=EDGE_LOOP ( 'NONE', ( #38738, #24437, #29499, #200 ) ) ;
#1667=ORIENTED_EDGE ( 'NONE', *, *, #21231, .F. ) ;
#1669=B_SPLINE_CURVE_WITH_KNOTS ( 'NONE', 3,
 ( #31136, #6861, #61708, #872, #27441, #2186, #26800, #51446, #5894, #37091, #10848, #26155, #51760, #12155, #22465, #46752, #21144, #16814 ),
 .UNSPECIFIED., .F., .F.,
 ( 4, 2, 2, 2, 2, 2, 2, 2, 4 ),
 ( 3.127317220692751144E-18, 0.001286103680247937435, 0.002572207360495871835, 0.003858311040743806018, 0.004501362880867774627, 0.005144414720991742802, 0.006430518401239680021, 0.007716622081487616372, 0.01028882944198348734 ),
 .UNSPECIFIED. ) ;
#1670=DIRECTION ( 'NONE',  ( 0.000000000000000000, 0.01356324068817998940, -0.9999080150203990547 ) ) ;
#1671=EDGE_CURVE ( 'NONE', #3168, #52651, #38877, .T. ) ;
#1674=DIRECTION ( 'NONE',  ( 1.000000000000000000, -0.000000000000000000, 0.000000000000000000 ) ) ;
#1675=DIRECTION ( 'NONE',  ( -1.000000000000000000, -1.836970198721029688E-16, -0.000000000000000000 ) ) ;
#1677=ADVANCED_FACE ( 'NONE', ( #17384 ), #47633, .T. ) ;
#1678=DIRECTION ( 'NONE',  ( -1.000000000000000000, 0.000000000000000000, 0.000000000000000000 ) ) ;
#1682=DIRECTION ( 'NONE',  ( -1.000000000000000000, 0.000000000000000000, 0.000000000000000000 ) ) ;
#1688=CYLINDRICAL_SURFACE ( 'NONE', #32395, 12.18650000000000055 ) ;
#1690=DIRECTION ( 'NONE',  ( -1.000000000000000000, 0.000000000000000000, -0.000000000000000000 ) ) ;
#1692=AXIS2_PLACEMENT_3D ( 'NONE', #2032, #7331, #31944 ) ;
#1693=ADVANCED_FACE ( 'NONE', ( #32327 ), #21378, .T. ) ;
#1695=ORIENTED_EDGE ( 'NONE', *, *, #38371, .T. ) ;
#1697=DIRECTION ( 'NONE',  ( 0.000000000000000000, 0.01356324068817992522, -0.9999080150203990547 ) ) ;
#1698=AXIS2_PLACEMENT_3D ( 'NONE', #20873, #11872, #61116 ) ;
#1700=ORIENTED_EDGE ( 'NONE', *, *, #12834, .F. ) ;
#1703=DIRECTION ( 'NONE',  ( 0.000000000000000000, 0.01356324068817998940, -0.9999080150203990547 ) ) ;
#1705=ORIENTED_EDGE ( 'NONE', *, *, #15911, .F. ) ;
#1706=ORIENTED_EDGE ( 'NONE', *, *, #28656, .F. ) ;
#1708=FACE_OUTER_BOUND ( 'NONE', #2461, .T. ) ;
#1710=FACE_OUTER_BOUND ( 'NONE', #53273, .T. ) ;
#1712=AXIS2_PLACEMENT_3D ( 'NONE', #44240, #23311, #59541 ) ;
#1713=DIRECTION ( 'NONE',  ( -0.000000000000000000, -1.000000000000000000, -0.000000000000000000 ) ) ;
#1715=ORIENTED_EDGE ( 'NONE', *, *, #65265, .F. ) ;
#1722=ORIENTED_EDGE ( 'NONE', *, *, #16385, .T. ) ;
#1723=CARTESIAN_POINT ( 'NONE',  ( 12.19644689801851811, 0.02881586504203031279, -13.50000000000000000 ) ) ;
#1724=CARTESIAN_POINT ( 'NONE',  ( -18.06844711592810526, -5.734463224907465850, 12.22455983143679781 ) ) ;
#1726=CARTESIAN_POINT ( 'NONE',  ( 36.00000000000000711, 11.01837265713073144, -6.415447294506746445 ) ) ;
#1727=DIRECTION ( 'NONE',  ( -1.000000000000000000, -1.836970198721029688E-16, 0.000000000000000000 ) ) ;
#1728=EDGE_CURVE ( 'NONE', #28136, #25112, #677, .T. ) ;
#1734=ORIENTED_EDGE ( 'NONE', *, *, #29161, .F. ) ;
#1735=CARTESIAN_POINT ( 'NONE',  ( -47.00000000000000711, 0.000000000000000000, 0.000000000000000000 ) ) ;
#1737=DIRECTION ( 'NONE',  ( 0.000000000000000000, -0.01356324068817998940, 0.9999080150203990547 ) ) ;
#1738=EDGE_CURVE ( 'NONE', #35815, #16693, #51652, .T. ) ;
#1740=DIRECTION ( 'NONE',  ( 0.000000000000000000, -0.01356324068818000848, 0.9999080150203990547 ) ) ;
#1742=DIRECTION ( 'NONE',  ( -1.000000000000000000, 0.000000000000000000, 0.000000000000000000 ) ) ;
#1743=EDGE_LOOP ( 'NONE', ( #40308, #678, #33809, #1774 ) ) ;
#1744=ORIENTED_EDGE ( 'NONE', *, *, #5, .T. ) ;
#1746=FACE_OUTER_BOUND ( 'NONE', #56468, .T. ) ;
#1747=ORIENTED_EDGE ( 'NONE', *, *, #45104, .F. ) ;
#1748=EDGE_CURVE ( 'NONE', #34943, #52755, #41980, .T. ) ;
#1749=DIRECTION ( 'NONE',  ( -1.000000000000000000, -1.836970198721029688E-16, 0.000000000000000000 ) ) ;
#1752=CARTESIAN_POINT ( 'NONE',  ( -3.167879205347148286, -12.42824319244124531, 5.282660448253479579 ) ) ;
#1753=CYLINDRICAL_SURFACE ( 'NONE', #48787, 5.000000000000000888 ) ;
#1755=EDGE_CURVE ( 'NONE', #35942, #13458, #26717, .T. ) ;
#1756=EDGE_LOOP ( 'NONE', ( #52914, #46976, #29109, #49555 ) ) ;
#1761=EDGE_CURVE ( 'NONE', #38782, #40551, #43282, .T. ) ;
#1763=( BOUNDED_CURVE ( )  B_SPLINE_CURVE ( 3, ( #62574, #31355, #37317, #22346 ),
 .UNSPECIFIED., .F., .F. ) 
 B_SPLINE_CURVE_WITH_KNOTS ( ( 4, 4 ),
 ( 1.881236687097070925, 1.898360998982701053 ),
 .UNSPECIFIED. ) 
 CURVE ( )  GEOMETRIC_REPRESENTATION_ITEM ( )  RATIONAL_B_SPLINE_CURVE ( ( 1.000000000000000000, 0.9999755633111596653, 0.9999755633111596653, 1.000000000000000000 ) ) 
 REPRESENTATION_ITEM ( '' )  );
#1764=DIRECTION ( 'NONE',  ( 0.000000000000000000, -0.8989688749565204473, -0.4380125133593880671 ) ) ;
#1765=ADVANCED_FACE ( 'NONE', ( #32972 ), #59258, .T. ) ;
#1769=DIRECTION ( 'NONE',  ( 0.000000000000000000, -0.01356324068817998940, 0.9999080150203990547 ) ) ;
#1770=DIRECTION ( 'NONE',  ( 1.000000000000000000, -0.000000000000000000, -0.000000000000000000 ) ) ;
#1771=ORIENTED_EDGE ( 'NONE', *, *, #21808, .T. ) ;
#1774=ORIENTED_EDGE ( 'NONE', *, *, #61825, .T. ) ;
#1775=DIRECTION ( 'NONE',  ( 1.000000000000000000, 0.000000000000000000, 0.000000000000000000 ) ) ;
#1779=ORIENTED_EDGE ( 'NONE', *, *, #28548, .F. ) ;
#1781=ORIENTED_EDGE ( 'NONE', *, *, #64674, .F. ) ;
#1782=ORIENTED_EDGE ( 'NONE', *, *, #35275, .F. ) ;
#1783=DIRECTION ( 'NONE',  ( 0.000000000000000000, -0.6269146997508042718, -0.7790879021242460567 ) ) ;
#1786=DIRECTION ( 'NONE',  ( 0.000000000000000000, 0.01356324068817992522, -0.9999080150203990547 ) ) ;
#1790=EDGE_LOOP ( 'NONE', ( #47577, #39844, #6297, #333 ) ) ;
#1794=CARTESIAN_POINT ( 'NONE',  ( -25.77840011361687189, 10.55150440484683294, 5.716830058840185025 ) ) ;
#1795=VERTEX_POINT ( 'NONE', #64870 ) ;
#1796=CARTESIAN_POINT ( 'NONE',  ( -27.86543437857248762, 9.320859823866943117, -7.583027560034842018 ) ) ;
#1798=DIRECTION ( 'NONE',  ( 0.000000000000000000, -0.8009703041134103030, -0.5987040770935764256 ) ) ;
#1801=CIRCLE ( 'NONE', #44264, 12.75000000000000178 ) ;
#1806=FACE_BOUND ( 'NONE', #38250, .T. ) ;
#1808=VECTOR ( 'NONE', #48269, 1000.000000000000000 ) ;
#1809=DIRECTION ( 'NONE',  ( 0.000000000000000000, 0.01356324068817992175, -0.9999080150203990547 ) ) ;
#1811=ORIENTED_EDGE ( 'NONE', *, *, #58271, .F. ) ;
#1812=ORIENTED_EDGE ( 'NONE', *, *, #41245, .T. ) ;
#1814=VERTEX_POINT ( 'NONE', #13683 ) ;
#1815=EDGE_CURVE ( 'NONE', #7231, #19321, #55904, .T. ) ;
#1816=VERTEX_POINT ( 'NONE', #54275 ) ;
#1817=LINE ( 'NONE', #12101, #62500 ) ;
#1818=DIRECTION ( 'NONE',  ( 0.000000000000000000, -0.9551603052523447435, 0.2960891610144610886 ) ) ;
#1819=FACE_OUTER_BOUND ( 'NONE', #27952, .T. ) ;
#1821=DIRECTION ( 'NONE',  ( -1.000000000000000000, 0.000000000000000000, 0.000000000000000000 ) ) ;
#1822=LINE ( 'NONE', #48030, #35229 ) ;
#1826=CARTESIAN_POINT ( 'NONE',  ( -37.00000000000000711, -11.39945968423475264, 5.710938531231672499 ) ) ;
#1828=DIRECTION ( 'NONE',  ( 0.000000000000000000, 0.01356324068817998940, -0.9999080150203990547 ) ) ;
#1829=CARTESIAN_POINT ( 'NONE',  ( -36.00000000000000711, 12.26766708251996363, -3.473736367725129615 ) ) ;
#1831=EDGE_CURVE ( 'NONE', #15972, #44370, #64383, .T. ) ;
#1832=VECTOR ( 'NONE', #59971, 1000.000000000000000 ) ;
#1833=CYLINDRICAL_SURFACE ( 'NONE', #33063, 5.000000000000002665 ) ;
#1834=ADVANCED_FACE ( 'NONE', ( #44583 ), #4050, .T. ) ;
#1835=CARTESIAN_POINT ( 'NONE',  ( 11.92129028673735647, 0.08362343793122377356, -11.99997311782909115 ) ) ;
#1836=ORIENTED_EDGE ( 'NONE', *, *, #35408, .T. ) ;
#1838=CARTESIAN_POINT ( 'NONE',  ( -35.00000000000000000, 0.000000000000000000, 0.000000000000000000 ) ) ;
#1841=AXIS2_PLACEMENT_3D ( 'NONE', #48515, #54145, #34174 ) ;
#1842=CARTESIAN_POINT ( 'NONE',  ( -24.81237754203414170, 8.088796810898713829, 8.871815844506174997 ) ) ;
#1843=DIRECTION ( 'NONE',  ( 0.000000000000000000, -0.01356324068817991828, 0.9999080150203990547 ) ) ;
#1844=ORIENTED_EDGE ( 'NONE', *, *, #16176, .F. ) ;
#1845=CARTESIAN_POINT ( 'NONE',  ( 18.54132159498832166, -6.065857072570194575, 10.36437726158596639 ) ) ;
#1846=CARTESIAN_POINT ( 'NONE',  ( 37.00000000000000711, 10.68873102412842258, -6.950793414699834472 ) ) ;
#1849=ORIENTED_EDGE ( 'NONE', *, *, #57670, .T. ) ;
#1851=CARTESIAN_POINT ( 'NONE',  ( -25.54417658651491863, 7.498517398407837931, 11.22596262356930197 ) ) ;
#1852=DIRECTION ( 'NONE',  ( 0.000000000000000000, 0.01356324068817998940, -0.9999080150203989437 ) ) ;
#1854=DIRECTION ( 'NONE',  ( 1.000000000000000000, -0.000000000000000000, -0.000000000000000000 ) ) ;
#1855=EDGE_CURVE ( 'NONE', #51673, #20923, #59103, .T. ) ;
#1857=ORIENTED_EDGE ( 'NONE', *, *, #50684, .F. ) ;
#1859=EDGE_CURVE ( 'NONE', #22430, #41989, #61215, .T. ) ;
#1860=CARTESIAN_POINT ( 'NONE',  ( 16.78263030916553689, 12.17295508002146320, 5.836879698929895888 ) ) ;
#1861=CARTESIAN_POINT ( 'NONE',  ( 23.76574300270097595, 1.690451441203562055, -11.88488507406290218 ) ) ;
#1862=CARTESIAN_POINT ( 'NONE',  ( 37.00000000000000711, -11.81949347079744506, 2.968224442958526943 ) ) ;
#1866=ORIENTED_EDGE ( 'NONE', *, *, #24512, .T. ) ;
#1868=ORIENTED_EDGE ( 'NONE', *, *, #60167, .F. ) ;
#1869=CARTESIAN_POINT ( 'NONE',  ( 24.83517902727939841, -1.538878142198703225, -11.90257845377566248 ) ) ;
#1870=ORIENTED_EDGE ( 'NONE', *, *, #60748, .F. ) ;
#1871=EDGE_CURVE ( 'NONE', #25468, #16649, #27987, .T. ) ;
#1873=AXIS2_PLACEMENT_3D ( 'NONE', #18740, #13079, #53659 ) ;
#1876=CARTESIAN_POINT ( 'NONE',  ( 22.68139259647346861, 3.158742727684422213, 13.12595410559641529 ) ) ;
#1878=AXIS2_PLACEMENT_3D ( 'NONE', #1248, #41449, #20858 ) ;
#1881=ORIENTED_EDGE ( 'NONE', *, *, #7064, .T. ) ;
#1882=ORIENTED_EDGE ( 'NONE', *, *, #60352, .F. ) ;
#1884=EDGE_CURVE ( 'NONE', #16592, #38075, #50271, .T. ) ;
#1885=EDGE_LOOP ( 'NONE', ( #14299, #23165, #55326, #62263 ) ) ;
#1887=CARTESIAN_POINT ( 'NONE',  ( 12.93723047338301058, 4.476360154859203355, 25.00000000000000000 ) ) ;
#1888=DIRECTION ( 'NONE',  ( -1.000000000000000000, -0.000000000000000000, -0.000000000000000000 ) ) ;
#1889=ADVANCED_FACE ( 'NONE', ( #10654 ), #14645, .T. ) ;
#1891=LINE ( 'NONE', #13483, #39409 ) ;
#1893=AXIS2_PLACEMENT_3D ( 'NONE', #48503, #64107, #53151 ) ;
#1894=B_SPLINE_CURVE_WITH_KNOTS ( 'NONE', 3,
 ( #256, #56088, #21170, #25179, #10527, #41440, #9884, #61399, #61731, #20531, #45453, #51124, #11206, #31483, #51780, #1237, #25851, #46142, #21516, #65719 ),
 .UNSPECIFIED., .F., .F.,
 ( 4, 2, 2, 2, 2, 2, 2, 2, 2, 4 ),
 ( 8.498374721940737388E-18, 0.001129263999270209906, 0.002258527998540411572, 0.003387791997810613454, 0.004517055997080814470, 0.005646319996351015919, 0.006210951995986116643, 0.006775583995621218235, 0.007904847994891418816, 0.009034111994161618531 ),
 .UNSPECIFIED. ) ;
#1895=DIRECTION ( 'NONE',  ( -1.000000000000000000, 0.000000000000000000, 0.000000000000000000 ) ) ;
#1898=ORIENTED_EDGE ( 'NONE', *, *, #59724, .T. ) ;
#1900=DIRECTION ( 'NONE',  ( -0.000000000000000000, -0.000000000000000000, -1.000000000000000000 ) ) ;
#1904=EDGE_CURVE ( 'NONE', #63443, #65388, #61219, .T. ) ;
#1905=ORIENTED_EDGE ( 'NONE', *, *, #19527, .F. ) ;
#1906=ORIENTED_EDGE ( 'NONE', *, *, #49929, .T. ) ;
#1908=ADVANCED_FACE ( 'NONE', ( #30945 ), #45928, .T. ) ;
#1910=CARTESIAN_POINT ( 'NONE',  ( 35.00000000000000000, 4.705694406421931860E-17, -3.469127814946512892E-15 ) ) ;
#1911=CARTESIAN_POINT ( 'NONE',  ( 37.00000000000000711, 4.705694406421931860E-17, -3.469127814946512892E-15 ) ) ;
#1912=ORIENTED_EDGE ( 'NONE', *, *, #9583, .T. ) ;
#1914=DIRECTION ( 'NONE',  ( -1.000000000000000000, 0.000000000000000000, 0.000000000000000000 ) ) ;
#1915=CARTESIAN_POINT ( 'NONE',  ( -29.25399988568289444, 1.550971944432816718, -13.41706731610524450 ) ) ;
#1916=CYLINDRICAL_SURFACE ( 'NONE', #55027, 5.000000000000000888 ) ;
#1917=AXIS2_PLACEMENT_3D ( 'NONE', #3547, #23819, #64352 ) ;
#1919=CARTESIAN_POINT ( 'NONE',  ( 37.00000000000000711, 12.60630747491662973, -1.908798535168425792 ) ) ;
#1920=CARTESIAN_POINT ( 'NONE',  ( -47.00000000000000711, 0.000000000000000000, 0.000000000000000000 ) ) ;
#1921=VECTOR ( 'NONE', #32346, 1000.000000000000000 ) ;
#1922=ORIENTED_EDGE ( 'NONE', *, *, #61949, .F. ) ;
#1925=CIRCLE ( 'NONE', #13586, 4.999999999999999112 ) ;
#1927=FACE_OUTER_BOUND ( 'NONE', #51480, .T. ) ;
#1928=CARTESIAN_POINT ( 'NONE',  ( -35.00000000000000000, 9.896810808925495806, -7.110831038798170134 ) ) ;
#1929=VECTOR ( 'NONE', #21014, 1000.000000000000000 ) ;
#1930=CARTESIAN_POINT ( 'NONE',  ( 37.00000000000000711, 4.705694406421931860E-17, -3.469127814946512892E-15 ) ) ;
#1931=DIRECTION ( 'NONE',  ( 0.000000000000000000, 0.000000000000000000, -1.000000000000000000 ) ) ;
#1932=ORIENTED_EDGE ( 'NONE', *, *, #16739, .T. ) ;
#1933=ORIENTED_EDGE ( 'NONE', *, *, #24025, .T. ) ;
#1937=LINE ( 'NONE', #63105, #47894 ) ;
#1945=EDGE_LOOP ( 'NONE', ( #24408, #51110, #63276, #20739 ) ) ;
#1946=VERTEX_POINT ( 'NONE', #15642 ) ;
#1949=ORIENTED_EDGE ( 'NONE', *, *, #12500, .T. ) ;
#1950=CARTESIAN_POINT ( 'NONE',  ( -9.351388602708162523, 11.42638970207765681, -3.665735721005252135 ) ) ;
#1951=DIRECTION ( 'NONE',  ( 1.000000000000000000, 0.000000000000000000, -0.000000000000000000 ) ) ;
#1952=EDGE_CURVE ( 'NONE', #1056, #33980, #27239, .T. ) ;
#1954=ORIENTED_EDGE ( 'NONE', *, *, #62247, .F. ) ;
#1957=AXIS2_PLACEMENT_3D ( 'NONE', #7343, #42932, #58578 ) ;
#1959=VERTEX_POINT ( 'NONE', #4388 ) ;
#1960=ORIENTED_EDGE ( 'NONE', *, *, #22683, .F. ) ;
#1962=ORIENTED_EDGE ( 'NONE', *, *, #44115, .T. ) ;
#1964=ORIENTED_EDGE ( 'NONE', *, *, #3810, .F. ) ;
#1965=DIRECTION ( 'NONE',  ( -1.000000000000000000, 0.000000000000000000, 0.000000000000000000 ) ) ;
#1966=ORIENTED_EDGE ( 'NONE', *, *, #19244, .F. ) ;
#1967=ORIENTED_EDGE ( 'NONE', *, *, #3399, .F. ) ;
#1969=EDGE_CURVE ( 'NONE', #23644, #35611, #24068, .T. ) ;
#1971=CIRCLE ( 'NONE', #5193, 4.999999999999999112 ) ;
#1972=FACE_OUTER_BOUND ( 'NONE', #43844, .T. ) ;
#1974=CARTESIAN_POINT ( 'NONE',  ( -37.00000000000000711, -9.821084925794515641, -7.215058775251366185 ) ) ;
#1975=CARTESIAN_POINT ( 'NONE',  ( -35.00000000000000000, -8.389074212634351824, 8.839356091080015076 ) ) ;
#1976=VECTOR ( 'NONE', #45259, 1000.000000000000000 ) ;
#1977=VECTOR ( 'NONE', #16746, 1000.000000000000000 ) ;
#1978=ORIENTED_EDGE ( 'NONE', *, *, #49712, .T. ) ;
#1979=FACE_OUTER_BOUND ( 'NONE', #46224, .T. ) ;
#1980=DIRECTION ( 'NONE',  ( 0.000000000000000000, 0.8369827122275325104, 0.5472293298355301872 ) ) ;
#1981=CIRCLE ( 'NONE', #20001, 12.74999999999999822 ) ;
#1982=DIRECTION ( 'NONE',  ( 0.000000000000000000, -0.5243256840888623760, -0.8515178078024829844 ) ) ;
#1984=CARTESIAN_POINT ( 'NONE',  ( -35.00000000000000000, 0.000000000000000000, 0.000000000000000000 ) ) ;
#1986=AXIS2_PLACEMENT_3D ( 'NONE', #50488, #910, #46153 ) ;
#1987=EDGE_CURVE ( 'NONE', #13432, #21858, #51426, .T. ) ;
#1988=ORIENTED_EDGE ( 'NONE', *, *, #28623, .F. ) ;
#1989=CARTESIAN_POINT ( 'NONE',  ( -37.00000000000000711, -1.488153103997047033, 11.65150730582934102 ) ) ;
#1990=ORIENTED_EDGE ( 'NONE', *, *, #27825, .F. ) ;
#1996=ORIENTED_EDGE ( 'NONE', *, *, #57073, .F. ) ;
#1997=DIRECTION ( 'NONE',  ( 0.000000000000000000, -0.01356324068818000848, 0.9999080150203990547 ) ) ;
#1998=DIRECTION ( 'NONE',  ( 1.000000000000000000, 0.000000000000000000, 0.000000000000000000 ) ) ;
#1999=LINE ( 'NONE', #38210, #3599 ) ;
#2000=CYLINDRICAL_SURFACE ( 'NONE', #44416, 12.18650000000000055 ) ;
#2001=EDGE_CURVE ( 'NONE', #40032, #38215, #40767, .T. ) ;
#2002=CARTESIAN_POINT ( 'NONE',  ( -37.00000000000000711, -4.018060380616481631, 11.50504120060941915 ) ) ;
#2003=ORIENTED_EDGE ( 'NONE', *, *, #41792, .T. ) ;
#2004=AXIS2_PLACEMENT_3D ( 'NONE', #64591, #39333, #49661 ) ;
#2007=DIRECTION ( 'NONE',  ( 0.000000000000000000, -0.01356324068817992001, 0.9999080150203990547 ) ) ;
#2008=CIRCLE ( 'NONE', #26402, 4.999999999999999112 ) ;
#2009=EDGE_LOOP ( 'NONE', ( #41662, #43468, #25227, #43967 ) ) ;
#2010=VECTOR ( 'NONE', #19988, 1000.000000000000000 ) ;
#2012=ORIENTED_EDGE ( 'NONE', *, *, #5105, .T. ) ;
#2015=CARTESIAN_POINT ( 'NONE',  ( -34.00000000000000000, 1.836970198721036590E-16, 0.000000000000000000 ) ) ;
#2016=VECTOR ( 'NONE', #25948, 1000.000000000000000 ) ;
#2018=EDGE_CURVE ( 'NONE', #8029, #9770, #16324, .T. ) ;
#2019=VERTEX_POINT ( 'NONE', #56903 ) ;
#2020=ORIENTED_EDGE ( 'NONE', *, *, #24564, .T. ) ;
#2021=CIRCLE ( 'NONE', #27500, 12.18649999999999878 ) ;
#2024=DIRECTION ( 'NONE',  ( 0.000000000000000000, 0.01356324068817998940, -0.9999080150203989437 ) ) ;
#2025=EDGE_CURVE ( 'NONE', #49629, #4304, #26614, .T. ) ;
#2026=VERTEX_POINT ( 'NONE', #21647 ) ;
#2027=CARTESIAN_POINT ( 'NONE',  ( 35.00000000000000000, 6.018036132182163378, -11.24036214326522654 ) ) ;
#2029=VERTEX_POINT ( 'NONE', #48150 ) ;
#2030=DIRECTION ( 'NONE',  ( 1.000000000000000000, -0.000000000000000000, 0.000000000000000000 ) ) ;
#2032=CARTESIAN_POINT ( 'NONE',  ( 35.00000000000000000, 11.72397916322012179, -0.7214809346829029746 ) ) ;
#2034=ORIENTED_EDGE ( 'NONE', *, *, #18654, .F. ) ;
#2038=DIRECTION ( 'NONE',  ( 1.000000000000000000, 0.000000000000000000, -0.000000000000000000 ) ) ;
#2039=CARTESIAN_POINT ( 'NONE',  ( -19.47984447937493613, -3.750539801530005768, 11.39883551934753925 ) ) ;
#2040=CARTESIAN_POINT ( 'NONE',  ( 35.00000000000000000, 5.143145423404279271, -11.66664283989681827 ) ) ;
#2043=DIRECTION ( 'NONE',  ( -1.000000000000000000, -0.000000000000000000, -0.000000000000000000 ) ) ;
#2045=DIRECTION ( 'NONE',  ( 0.000000000000000000, 0.01356324068817991828, -0.9999080150203990547 ) ) ;
#2050=AXIS2_PLACEMENT_3D ( 'NONE', #58930, #64215, #44560 ) ;
#2051=DIRECTION ( 'NONE',  ( 1.000000000000000000, 0.000000000000000000, 0.000000000000000000 ) ) ;
#2056=DIRECTION ( 'NONE',  ( 0.000000000000000000, -0.5472293298355331848, 0.8369827122275305120 ) ) ;
#2057=AXIS2_PLACEMENT_3D ( 'NONE', #13838, #8880, #29172 ) ;
#2058=VERTEX_POINT ( 'NONE', #31287 ) ;
#2059=ORIENTED_EDGE ( 'NONE', *, *, #5404, .T. ) ;
#2060=DIRECTION ( 'NONE',  ( -1.000000000000000000, -0.000000000000000000, -0.000000000000000000 ) ) ;
#2062=ORIENTED_EDGE ( 'NONE', *, *, #6020, .T. ) ;
#2063=CARTESIAN_POINT ( 'NONE',  ( -35.00000000000000000, -6.657191900728257394, -9.677500615117970995 ) ) ;
#2066=DIRECTION ( 'NONE',  ( -1.000000000000000000, -0.000000000000000000, 0.000000000000000000 ) ) ;
#2069=AXIS2_PLACEMENT_3D ( 'NONE', #61587, #41642, #16388 ) ;
#2071=EDGE_CURVE ( 'NONE', #47315, #28963, #61561, .T. ) ;
#2073=DIRECTION ( 'NONE',  ( -1.000000000000000000, 0.000000000000000000, 0.000000000000000000 ) ) ;
#2074=CARTESIAN_POINT ( 'NONE',  ( 6.361445718264521432, -4.355102044641763648, 25.00000000000000000 ) ) ;
#2076=FACE_OUTER_BOUND ( 'NONE', #5382, .T. ) ;
#2079=AXIS2_PLACEMENT_3D ( 'NONE', #1911, #22182, #57787 ) ;
#2080=EDGE_CURVE ( 'NONE', #32174, #47999, #22752, .T. ) ;
#2081=ORIENTED_EDGE ( 'NONE', *, *, #2651, .F. ) ;
#2082=DIRECTION ( 'NONE',  ( 1.000000000000000000, 0.000000000000000000, 0.000000000000000000 ) ) ;
#2083=CARTESIAN_POINT ( 'NONE',  ( 37.00000000000000711, 10.43555801961475282, -5.391785509271000087 ) ) ;
#2084=ORIENTED_EDGE ( 'NONE', *, *, #42682, .T. ) ;
#2085=VECTOR ( 'NONE', #49994, 1000.000000000000000 ) ;
#2087=CARTESIAN_POINT ( 'NONE',  ( 36.00000000000000711, -2.250029553613672295, 12.54989509947652770 ) ) ;
#2088=CARTESIAN_POINT ( 'NONE',  ( -35.00000000000000000, -11.56998259273174945, -3.827046518385204266 ) ) ;
#2089=ORIENTED_EDGE ( 'NONE', *, *, #34398, .T. ) ;
#2090=DIRECTION ( 'NONE',  ( -1.000000000000000000, 0.000000000000000000, 0.000000000000000000 ) ) ;
#2092=ORIENTED_EDGE ( 'NONE', *, *, #36645, .T. ) ;
#2093=DIRECTION ( 'NONE',  ( -1.000000000000000000, 0.000000000000000000, 0.000000000000000000 ) ) ;
#2096=AXIS2_PLACEMENT_3D ( 'NONE', #30955, #20971, #1038 ) ;
#2098=EDGE_CURVE ( 'NONE', #21166, #60814, #11002, .T. ) ;
#2099=ORIENTED_EDGE ( 'NONE', *, *, #13165, .T. ) ;
#2101=CARTESIAN_POINT ( 'NONE',  ( 3.709656308118471912, 4.519821899412372446, 12.72824511710198792 ) ) ;
#2102=AXIS2_PLACEMENT_3D ( 'NONE', #59192, #59504, #34226 ) ;
#2103=CARTESIAN_POINT ( 'NONE',  ( -36.00000000000000711, -4.824807283154036064, -11.80185301892985983 ) ) ;
#2106=CYLINDRICAL_SURFACE ( 'NONE', #45841, 12.18649999999999878 ) ;
#2107=ADVANCED_FACE ( 'NONE', ( #28182 ), #48472, .T. ) ;
#2111=VERTEX_POINT ( 'NONE', #2920 ) ;
#2112=CARTESIAN_POINT ( 'NONE',  ( 35.00000000000000000, -5.927257550915237871, 10.64792938439761549 ) ) ;
#2113=VERTEX_POINT ( 'NONE', #45105 ) ;
#2114=CARTESIAN_POINT ( 'NONE',  ( -37.00000000000000711, 0.000000000000000000, 0.000000000000000000 ) ) ;
#2115=AXIS2_PLACEMENT_3D ( 'NONE', #55523, #34569, #4003 ) ;
#2116=ORIENTED_EDGE ( 'NONE', *, *, #16294, .T. ) ;
#2118=DIRECTION ( 'NONE',  ( 0.000000000000000000, -0.01356324068817998940, 0.9999080150203990547 ) ) ;
#2119=CARTESIAN_POINT ( 'NONE',  ( 35.00000000000000000, 6.917234959366825642, -9.493370459201726064 ) ) ;
#2120=ORIENTED_EDGE ( 'NONE', *, *, #57931, .F. ) ;
#2124=EDGE_CURVE ( 'NONE', #33360, #15413, #64127, .T. ) ;
#2125=ORIENTED_EDGE ( 'NONE', *, *, #13653, .F. ) ;
#2127=ORIENTED_EDGE ( 'NONE', *, *, #26732, .F. ) ;
#2130=EDGE_CURVE ( 'NONE', #20972, #23800, #14807, .T. ) ;
#2133=CARTESIAN_POINT ( 'NONE',  ( 145.1370849898475797, 3.309064568108273190E-14, 0.000000000000000000 ) ) ;
#2134=DIRECTION ( 'NONE',  ( 0.000000000000000000, -0.2006870767258747135, 0.9796553971857772103 ) ) ;
#2139=AXIS2_PLACEMENT_3D ( 'NONE', #1984, #38191, #22252 ) ;
#2142=VERTEX_POINT ( 'NONE', #4209 ) ;
#2143=CARTESIAN_POINT ( 'NONE',  ( -35.00000000000000000, -12.01765980939843281, 2.021542716731355771 ) ) ;
#2144=DIRECTION ( 'NONE',  ( 0.000000000000000000, -0.9551603052523509607, 0.2960891610144411601 ) ) ;
#2145=AXIS2_PLACEMENT_3D ( 'NONE', #15184, #25163, #54118 ) ;
#2148=CARTESIAN_POINT ( 'NONE',  ( 35.00000000000000000, 4.705694406421931860E-17, -3.469127814946512892E-15 ) ) ;
#2149=CARTESIAN_POINT ( 'NONE',  ( -35.00000000000000000, 0.000000000000000000, 0.000000000000000000 ) ) ;
#2151=CARTESIAN_POINT ( 'NONE',  ( 35.00000000000000000, 11.05394794832829497, -5.130401251914769922 ) ) ;
#2152=CARTESIAN_POINT ( 'NONE',  ( 9.625472734749340731, 2.219514715007567141, -11.79494074077256904 ) ) ;
#2153=ORIENTED_EDGE ( 'NONE', *, *, #52516, .T. ) ;
#2154=DIRECTION ( 'NONE',  ( 0.000000000000000000, -0.6943713148249691658, 0.7196168960969744344 ) ) ;
#2155=DIRECTION ( 'NONE',  ( 0.000000000000000000, -0.01356324068817999114, 0.9999080150203989437 ) ) ;
#2159=ADVANCED_FACE ( 'NONE', ( #59408 ), #9498, .T. ) ;
#2160=CARTESIAN_POINT ( 'NONE',  ( 12.93723047338301058, 4.476360154859203355, 25.00000000000000000 ) ) ;
#2161=DIRECTION ( 'NONE',  ( -1.000000000000000000, 0.000000000000000000, -0.000000000000000000 ) ) ;
#2162=VECTOR ( 'NONE', #8756, 1000.000000000000000 ) ;
#2163=ORIENTED_EDGE ( 'NONE', *, *, #21823, .T. ) ;
#2164=DIRECTION ( 'NONE',  ( -0.000000000000000000, -1.000000000000000000, -0.000000000000000000 ) ) ;
#2168=ORIENTED_EDGE ( 'NONE', *, *, #39019, .F. ) ;
#2169=DIRECTION ( 'NONE',  ( 0.000000000000000000, -0.01356324068817998940, 0.9999080150203990547 ) ) ;
#2170=AXIS2_PLACEMENT_3D ( 'NONE', #48812, #60085, #56399 ) ;
#2171=LINE ( 'NONE', #61362, #7840 ) ;
#2177=AXIS2_PLACEMENT_3D ( 'NONE', #50583, #33950, #34604 ) ;
#2180=CARTESIAN_POINT ( 'NONE',  ( -37.00000000000000711, 0.000000000000000000, 0.000000000000000000 ) ) ;
#2181=VERTEX_POINT ( 'NONE', #24823 ) ;
#2183=DIRECTION ( 'NONE',  ( 0.000000000000000000, 0.1118654143051617117, 0.9937233664769761221 ) ) ;
#2185=CARTESIAN_POINT ( 'NONE',  ( -35.00000000000000000, 11.29812557209476864, 3.213188559034282132 ) ) ;
#2186=CARTESIAN_POINT ( 'NONE',  ( -9.838546225284394708, 10.19292628221959518, -6.347466807329325000 ) ) ;
#2188=CARTESIAN_POINT ( 'NONE',  ( -10.79842706929647278, -9.842369975612381694, 9.240427863961670596 ) ) ;
#2189=CARTESIAN_POINT ( 'NONE',  ( -35.00000000000000000, 10.62137734850268345, 5.015831474386344802 ) ) ;
#2190=VERTEX_POINT ( 'NONE', #49764 ) ;
#2192=EDGE_CURVE ( 'NONE', #46377, #63634, #59915, .T. ) ;
#2193=ORIENTED_EDGE ( 'NONE', *, *, #20768, .T. ) ;
#2195=ORIENTED_EDGE ( 'NONE', *, *, #39656, .F. ) ;
#2196=ORIENTED_EDGE ( 'NONE', *, *, #14629, .T. ) ;
#2200=CIRCLE ( 'NONE', #15984, 12.74999999999999822 ) ;
#2202=LINE ( 'NONE', #32439, #39618 ) ;
#2204=EDGE_CURVE ( 'NONE', #16590, #54151, #60955, .T. ) ;
#2205=DIRECTION ( 'NONE',  ( 1.000000000000000000, 0.000000000000000000, 0.000000000000000000 ) ) ;
#2206=VECTOR ( 'NONE', #46791, 1000.000000000000000 ) ;
#2207=ORIENTED_EDGE ( 'NONE', *, *, #64392, .F. ) ;
#2208=AXIS2_PLACEMENT_3D ( 'NONE', #47807, #57803, #36840 ) ;
#2211=ORIENTED_EDGE ( 'NONE', *, *, #33043, .F. ) ;
#2212=ORIENTED_EDGE ( 'NONE', *, *, #49357, .F. ) ;
#2216=ORIENTED_EDGE ( 'NONE', *, *, #20034, .F. ) ;
#2217=AXIS2_PLACEMENT_3D ( 'NONE', #18678, #9303, #9630 ) ;
#2218=CYLINDRICAL_SURFACE ( 'NONE', #31691, 12.75000000000000178 ) ;
#2219=DIRECTION ( 'NONE',  ( 1.000000000000000000, 0.000000000000000000, -0.000000000000000000 ) ) ;
#2220=CARTESIAN_POINT ( 'NONE',  ( -37.00000000000000711, -11.74614673114904129, -0.01609748574457297438 ) ) ;
#2222=DIRECTION ( 'NONE',  ( 1.000000000000000000, 0.000000000000000000, 0.000000000000000000 ) ) ;
#2227=DIRECTION ( 'NONE',  ( 1.000000000000000000, -0.000000000000000000, -0.000000000000000000 ) ) ;
#2228=ORIENTED_EDGE ( 'NONE', *, *, #7230, .F. ) ;
#2231=CARTESIAN_POINT ( 'NONE',  ( -9.010009660721790326, -10.91952191215454526, -7.945783354247663688 ) ) ;
#2233=DIRECTION ( 'NONE',  ( -1.000000000000000000, -0.000000000000000000, 0.000000000000000000 ) ) ;
#2234=VERTEX_POINT ( 'NONE', #25144 ) ;
#2235=CIRCLE ( 'NONE', #41508, 4.999999999999999112 ) ;
#2238=ORIENTED_EDGE ( 'NONE', *, *, #18675, .T. ) ;
#2239=VECTOR ( 'NONE', #46424, 1000.000000000000000 ) ;
#2240=CYLINDRICAL_SURFACE ( 'NONE', #64129, 4.999999999999997335 ) ;
#2241=VERTEX_POINT ( 'NONE', #212 ) ;
#2243=CARTESIAN_POINT ( 'NONE',  ( 8.437200413559441614, 4.868584981346780971, 10.97613720874745269 ) ) ;
#2245=DIRECTION ( 'NONE',  ( 0.000000000000000000, -0.9903235168508566222, -0.1387779952735712363 ) ) ;
#2246=ORIENTED_EDGE ( 'NONE', *, *, #64741, .T. ) ;
#2249=EDGE_CURVE ( 'NONE', #23975, #51925, #11474, .T. ) ;
#2251=CARTESIAN_POINT ( 'NONE',  ( -35.00000000000000000, 9.321877890560440250, 7.146664589317944127 ) ) ;
#2253=VECTOR ( 'NONE', #26938, 1000.000000000000000 ) ;
#2254=CARTESIAN_POINT ( 'NONE',  ( -37.00000000000000711, 12.71517666308949579, -0.9416912585473031783 ) ) ;
#2255=VECTOR ( 'NONE', #41696, 1000.000000000000000 ) ;
#2257=EDGE_LOOP ( 'NONE', ( #19542, #2542, #30218, #9068 ) ) ;
#2258=CIRCLE ( 'NONE', #62750, 4.999999999999999112 ) ;
#2260=ORIENTED_EDGE ( 'NONE', *, *, #47857, .T. ) ;
#2261=CARTESIAN_POINT ( 'NONE',  ( 35.00000000000000000, 4.705694406421931860E-17, -3.469127814946512892E-15 ) ) ;
#2262=DIRECTION ( 'NONE',  ( -1.000000000000000000, -0.000000000000000000, -0.000000000000000000 ) ) ;
#2263=DIRECTION ( 'NONE',  ( 0.000000000000000000, 0.01356324068817991481, -0.9999080150203990547 ) ) ;
#2266=DIRECTION ( 'NONE',  ( 0.9364047569793457759, -0.3509218304786018705, 0.000000000000000000 ) ) ;
#2267=EDGE_CURVE ( 'NONE', #47648, #28210, #63924, .T. ) ;
#2272=ORIENTED_EDGE ( 'NONE', *, *, #56146, .T. ) ;
#2274=CARTESIAN_POINT ( 'NONE',  ( 2.872766899732817958, 3.568102790788560963, 11.46450991852135637 ) ) ;
#2280=DIRECTION ( 'NONE',  ( 0.000000000000000000, 0.01356324068817998940, -0.9999080150203990547 ) ) ;
#2281=ORIENTED_EDGE ( 'NONE', *, *, #44975, .F. ) ;
#2282=AXIS2_PLACEMENT_3D ( 'NONE', #17570, #57151, #6936 ) ;
#2283=ORIENTED_EDGE ( 'NONE', *, *, #18854, .F. ) ;
#2284=DIRECTION ( 'NONE',  ( 0.000000000000000000, -0.01356324068817999114, 0.9999080150203989437 ) ) ;
#2286=( NAMED_UNIT ( * ) SI_UNIT ( $, .STERADIAN. ) SOLID_ANGLE_UNIT ( ) );
#2287=EDGE_CURVE ( 'NONE', #58825, #45959, #61688, .T. ) ;
#2288=DIRECTION ( 'NONE',  ( 1.000000000000000000, 0.000000000000000000, 0.000000000000000000 ) ) ;
#2290=DIRECTION ( 'NONE',  ( -1.000000000000000000, -0.000000000000000000, 0.000000000000000000 ) ) ;
#2291=ADVANCED_FACE ( 'NONE', ( #11166 ), #31441, .T. ) ;
#2293=VERTEX_POINT ( 'NONE', #33068 ) ;
#2294=DIRECTION ( 'NONE',  ( 1.000000000000000000, 0.000000000000000000, -0.000000000000000000 ) ) ;
#2296=CARTESIAN_POINT ( 'NONE',  ( -37.00000000000000711, 0.000000000000000000, 0.000000000000000000 ) ) ;
#2297=VERTEX_POINT ( 'NONE', #53375 ) ;
#2299=EDGE_CURVE ( 'NONE', #49715, #11584, #43045, .T. ) ;
#2301=VERTEX_POINT ( 'NONE', #32079 ) ;
#2302=ORIENTED_EDGE ( 'NONE', *, *, #37993, .T. ) ;
#2303=DIRECTION ( 'NONE',  ( 0.000000000000000000, 0.6478160128811893959, -0.7617968321374923857 ) ) ;
#2304=VERTEX_POINT ( 'NONE', #62341 ) ;
#2305=ORIENTED_EDGE ( 'NONE', *, *, #52599, .T. ) ;
#2306=CIRCLE ( 'NONE', #40486, 4.999999999999999112 ) ;
#2308=CARTESIAN_POINT ( 'NONE',  ( 37.00000000000000711, 4.705694406421931860E-17, -3.469127814946512892E-15 ) ) ;
#2309=CIRCLE ( 'NONE', #50049, 12.74999999999999822 ) ;
#2311=DIRECTION ( 'NONE',  ( 0.000000000000000000, 0.9937233664769765662, -0.1118654143051580896 ) ) ;
#2312=DIRECTION ( 'NONE',  ( -1.000000000000000000, 0.000000000000000000, 0.000000000000000000 ) ) ;
#2313=ADVANCED_FACE ( 'NONE', ( #7821 ), #12135, .T. ) ;
#2315=DIRECTION ( 'NONE',  ( -1.000000000000000000, -0.000000000000000000, 0.000000000000000000 ) ) ;
#2318=CARTESIAN_POINT ( 'NONE',  ( -35.00000000000000000, 0.000000000000000000, 0.000000000000000000 ) ) ;
#2319=CIRCLE ( 'NONE', #62810, 4.999999999999998224 ) ;
#2321=CARTESIAN_POINT ( 'NONE',  ( 29.56688794281942023, 5.030830317295369447, 10.90585321954392128 ) ) ;
#2324=DIRECTION ( 'NONE',  ( 0.000000000000000000, 0.07632122047556495759, -0.9970832820307038435 ) ) ;
#2325=ORIENTED_EDGE ( 'NONE', *, *, #25207, .T. ) ;
#2327=CIRCLE ( 'NONE', #63862, 12.18650000000000055 ) ;
#2328=EDGE_CURVE ( 'NONE', #51491, #51616, #5770, .T. ) ;
#2332=CARTESIAN_POINT ( 'NONE',  ( 12.25434804473628247, -13.17050011957374878, -2.969510513515200678 ) ) ;
#2333=AXIS2_PLACEMENT_3D ( 'NONE', #2318, #52845, #48524 ) ;
#2335=AXIS2_PLACEMENT_3D ( 'NONE', #7078, #53299, #42629 ) ;
#2340=B_SPLINE_CURVE_WITH_KNOTS ( 'NONE', 3,
 ( #23938, #38893, #9258, #64784, #33887, #8624 ),
 .UNSPECIFIED., .F., .F.,
 ( 4, 2, 4 ),
 ( 0.004238702544367933985, 0.006292126001073344854, 0.008345549457778756591 ),
 .UNSPECIFIED. ) ;
#2341=CYLINDRICAL_SURFACE ( 'NONE', #29013, 12.75000000000000178 ) ;
#2342=CARTESIAN_POINT ( 'NONE',  ( -4.007992427301752869, 10.70267137441327776, 8.237965989174103498 ) ) ;
#2343=AXIS2_PLACEMENT_3D ( 'NONE', #42066, #43375, #6515 ) ;
#2350=EDGE_CURVE ( 'NONE', #55613, #65690, #32260, .T. ) ;
#2352=AXIS2_PLACEMENT_3D ( 'NONE', #46510, #35850, #16256 ) ;
#2353=EDGE_CURVE ( 'NONE', #8559, #36681, #30130, .T. ) ;
#2354=AXIS2_PLACEMENT_3D ( 'NONE', #53205, #2698, #23941 ) ;
#2355=EDGE_LOOP ( 'NONE', ( #59616, #36920, #42552, #1572 ) ) ;
#2356=VECTOR ( 'NONE', #36667, 1000.000000000000000 ) ;
#2357=CARTESIAN_POINT ( 'NONE',  ( -7.181456785175555524, 5.890186129966279438, -10.45493698471458188 ) ) ;
#2362=CARTESIAN_POINT ( 'NONE',  ( -29.52025388906147541, -3.281486406648443044, 13.10044398286176559 ) ) ;
#2363=CIRCLE ( 'NONE', #39501, 5.000000000000000000 ) ;
#2367=ORIENTED_EDGE ( 'NONE', *, *, #58785, .F. ) ;
#2368=ORIENTED_EDGE ( 'NONE', *, *, #20567, .F. ) ;
#2370=EDGE_CURVE ( 'NONE', #48435, #47727, #23795, .T. ) ;
#2372=CARTESIAN_POINT ( 'NONE',  ( 36.00000000000000711, -11.66664283989683604, -5.143145423404237526 ) ) ;
#2374=CARTESIAN_POINT ( 'NONE',  ( 35.00000000000000000, 0.4993900848169179896, 12.17626345777662600 ) ) ;
#2375=ORIENTED_EDGE ( 'NONE', *, *, #23711, .F. ) ;
#2379=EDGE_LOOP ( 'NONE', ( #45485, #48910, #61777, #48884 ) ) ;
#2380=ORIENTED_EDGE ( 'NONE', *, *, #59871, .T. ) ;
#2383=CARTESIAN_POINT ( 'NONE',  ( 8.437200413559445167, 4.214301595845684645, -12.82835998935028776 ) ) ;
#2385=AXIS2_PLACEMENT_3D ( 'NONE', #34946, #59937, #23119 ) ;
#2389=DIRECTION ( 'NONE',  ( 0.000000000000000000, -0.7196168960969868689, -0.6943713148249562872 ) ) ;
#2390=DIRECTION ( 'NONE',  ( 0.000000000000000000, -0.01356324068817998940, 0.9999080150203990547 ) ) ;
#2393=CARTESIAN_POINT ( 'NONE',  ( 3.347841273039249721, -10.61118957148187825, -5.603807266321158664 ) ) ;
#2394=ORIENTED_EDGE ( 'NONE', *, *, #41950, .T. ) ;
#2396=EDGE_LOOP ( 'NONE', ( #28433, #35547, #30639, #32533 ) ) ;
#2398=CYLINDRICAL_SURFACE ( 'NONE', #45760, 12.18650000000000055 ) ;
#2404=VERTEX_POINT ( 'NONE', #52719 ) ;
#2405=VECTOR ( 'NONE', #14019, 1000.000000000000000 ) ;
#2406=EDGE_LOOP ( 'NONE', ( #28324, #28630, #43642, #24421 ) ) ;
#2407=CARTESIAN_POINT ( 'NONE',  ( -37.00000000000000711, -5.921969905510425569, 10.14408668126211488 ) ) ;
#2408=EDGE_CURVE ( 'NONE', #63443, #41839, #57713, .T. ) ;
#2409=VECTOR ( 'NONE', #52013, 1000.000000000000000 ) ;
#2410=ORIENTED_EDGE ( 'NONE', *, *, #19134, .F. ) ;
#2411=DIRECTION ( 'NONE',  ( 0.000000000000000000, -0.01356324068817998940, 0.9999080150203990547 ) ) ;
#2412=CIRCLE ( 'NONE', #56560, 12.18649999999999878 ) ;
#2417=VERTEX_POINT ( 'NONE', #11797 ) ;
#2418=CARTESIAN_POINT ( 'NONE',  ( -35.00000000000000000, 9.926225166347114381, -6.280308599560036065 ) ) ;
#2419=EDGE_CURVE ( 'NONE', #45412, #12619, #55215, .T. ) ;
#2420=CIRCLE ( 'NONE', #19356, 4.999999999999999112 ) ;
#2422=CARTESIAN_POINT ( 'NONE',  ( 22.21243700998469350, 12.61357499758618772, -4.824052666793012811 ) ) ;
#2423=CARTESIAN_POINT ( 'NONE',  ( 37.00000000000000711, -9.060822531525994705, 7.474872387601095625 ) ) ;
#2424=CARTESIAN_POINT ( 'NONE',  ( 22.88594695219327235, -4.822122601967141264, 12.60940655271284427 ) ) ;
#2426=DIRECTION ( 'NONE',  ( -1.000000000000000000, 0.000000000000000000, -0.000000000000000000 ) ) ;
#2428=CIRCLE ( 'NONE', #53399, 12.75000000000000178 ) ;
#2429=CIRCLE ( 'NONE', #26809, 4.999999999999999112 ) ;
#2430=AXIS2_PLACEMENT_3D ( 'NONE', #53108, #39109, #3235 ) ;
#2432=ORIENTED_EDGE ( 'NONE', *, *, #10252, .T. ) ;
#2433=CARTESIAN_POINT ( 'NONE',  ( -2.952869152607106251, 25.00000000000000000, 3.755417052241485365 ) ) ;
#2435=ORIENTED_EDGE ( 'NONE', *, *, #47857, .F. ) ;
#2438=ORIENTED_EDGE ( 'NONE', *, *, #28088, .F. ) ;
#2440=CARTESIAN_POINT ( 'NONE',  ( -35.00000000000000000, 4.603882218679707705, -10.80631716521661900 ) ) ;
#2442=AXIS2_PLACEMENT_3D ( 'NONE', #13497, #39763, #55052 ) ;
#2443=CARTESIAN_POINT ( 'NONE',  ( 37.00000000000000711, 4.074242145636174151, 12.08151691381185167 ) ) ;
#2444=VERTEX_POINT ( 'NONE', #45112 ) ;
#2445=VERTEX_POINT ( 'NONE', #25811 ) ;
#2446=AXIS2_PLACEMENT_3D ( 'NONE', #8640, #54538, #58545 ) ;
#2448=VERTEX_POINT ( 'NONE', #55747 ) ;
#2449=CARTESIAN_POINT ( 'NONE',  ( -35.00000000000000000, -9.926225166347071749, 6.280308599560108007 ) ) ;
#2450=CARTESIAN_POINT ( 'NONE',  ( 3.598314112554458877, 4.116749633316167944, 12.86379551159408230 ) ) ;
#2451=CARTESIAN_POINT ( 'NONE',  ( 22.57855258442564761, -4.427776684447072952, 25.00000000000000000 ) ) ;
#2455=AXIS2_PLACEMENT_3D ( 'NONE', #53253, #11362, #7700 ) ;
#2458=CARTESIAN_POINT ( 'NONE',  ( 12.51043607184429796, 0.3316456940255356201, -13.49694458083817672 ) ) ;
#2459=ORIENTED_EDGE ( 'NONE', *, *, #57575, .F. ) ;
#2460=DIRECTION ( 'NONE',  ( -1.000000000000000000, 0.000000000000000000, 0.000000000000000000 ) ) ;
#2461=EDGE_LOOP ( 'NONE', ( #41703, #13045, #49058, #56258 ) ) ;
#2462=CARTESIAN_POINT ( 'NONE',  ( 37.00000000000000711, 11.39945968423471534, -5.710938531231753323 ) ) ;
#2466=FACE_OUTER_BOUND ( 'NONE', #17509, .T. ) ;
#2471=DIRECTION ( 'NONE',  ( 0.000000000000000000, 0.01356324068817998940, -0.9999080150203990547 ) ) ;
#2472=DIRECTION ( 'NONE',  ( -1.000000000000000000, 0.000000000000000000, -0.000000000000000000 ) ) ;
#2473=CARTESIAN_POINT ( 'NONE',  ( 13.41517466982755558, 12.56449639282538833, -4.957758779083538236 ) ) ;
#2475=ORIENTED_EDGE ( 'NONE', *, *, #36230, .F. ) ;
#2479=VERTEX_POINT ( 'NONE', #50440 ) ;
#2480=CARTESIAN_POINT ( 'NONE',  ( 19.13486214123186357, -6.258902428715801491, 11.96274114462062421 ) ) ;
#2481=CIRCLE ( 'NONE', #60848, 12.18650000000000233 ) ;
#2483=DIRECTION ( 'NONE',  ( 1.000000000000000000, 0.000000000000000000, -0.000000000000000000 ) ) ;
#2487=CARTESIAN_POINT ( 'NONE',  ( -37.00000000000000711, -0.4353888892047496628, -11.73808581813438501 ) ) ;
#2488=AXIS2_PLACEMENT_3D ( 'NONE', #35844, #4974, #31221 ) ;
#2489=EDGE_CURVE ( 'NONE', #52527, #15712, #57782, .T. ) ;
#2491=ADVANCED_FACE ( 'NONE', ( #35448 ), #552, .T. ) ;
#2492=EDGE_CURVE ( 'NONE', #7978, #11644, #55076, .T. ) ;
#2493=EDGE_LOOP ( 'NONE', ( #46842, #4376, #48635, #47775 ) ) ;
#2494=CIRCLE ( 'NONE', #9917, 5.000000000000000000 ) ;
#2495=DIRECTION ( 'NONE',  ( -1.000000000000000000, 0.000000000000000000, 0.000000000000000000 ) ) ;
#2497=CARTESIAN_POINT ( 'NONE',  ( -35.00000000000000000, 0.000000000000000000, 0.000000000000000000 ) ) ;
#2501=FACE_OUTER_BOUND ( 'NONE', #39729, .T. ) ;
#2504=CIRCLE ( 'NONE', #57753, 5.000000000000000000 ) ;
#2505=DIRECTION ( 'NONE',  ( -1.000000000000000000, 0.000000000000000000, 0.000000000000000000 ) ) ;
#2506=EDGE_CURVE ( 'NONE', #21166, #40181, #46097, .T. ) ;
#2507=VECTOR ( 'NONE', #995, 1000.000000000000000 ) ;
#2510=DIRECTION ( 'NONE',  ( 1.000000000000000000, 0.000000000000000000, 0.000000000000000000 ) ) ;
#2511=DIRECTION ( 'NONE',  ( 0.000000000000000000, 0.01356324068817998940, -0.9999080150203990547 ) ) ;
#2512=CARTESIAN_POINT ( 'NONE',  ( 32.00000000000000000, 1.230770033143089974E-14, 0.000000000000000000 ) ) ;
#2514=CIRCLE ( 'NONE', #39659, 5.000000000000000000 ) ;
#2516=DIRECTION ( 'NONE',  ( -1.000000000000000000, 0.000000000000000000, -0.000000000000000000 ) ) ;
#2519=CARTESIAN_POINT ( 'NONE',  ( 17.54630545878690739, -9.526853237520755968, 7.355185947339629493 ) ) ;
#2520=CARTESIAN_POINT ( 'NONE',  ( -35.00000000000000000, 0.000000000000000000, 0.000000000000000000 ) ) ;
#2523=ORIENTED_EDGE ( 'NONE', *, *, #45730, .F. ) ;
#2524=DIRECTION ( 'NONE',  ( 0.000000000000000000, -1.000000000000000000, 0.000000000000000000 ) ) ;
#2525=DIRECTION ( 'NONE',  ( 0.000000000000000000, 0.1387779952735747058, -0.9903235168508560671 ) ) ;
#2526=ORIENTED_EDGE ( 'NONE', *, *, #49622, .T. ) ;
#2527=AXIS2_PLACEMENT_3D ( 'NONE', #64911, #15366, #45966 ) ;
#2528=VERTEX_POINT ( 'NONE', #51433 ) ;
#2530=CIRCLE ( 'NONE', #56693, 5.000000000000000000 ) ;
#2531=CARTESIAN_POINT ( 'NONE',  ( -35.00000000000000000, 3.093009498344089447, -11.78745411414836930 ) ) ;
#2532=VERTEX_POINT ( 'NONE', #15806 ) ;
#2533=DIRECTION ( 'NONE',  ( 0.000000000000000000, -0.01356324068817999114, 0.9999080150203989437 ) ) ;
#2534=DIRECTION ( 'NONE',  ( 0.000000000000000000, -0.01356324068817991828, 0.9999080150203990547 ) ) ;
#2535=( BOUNDED_CURVE ( )  B_SPLINE_CURVE ( 3, ( #49702, #64636, #34062, #34402 ),
 .UNSPECIFIED., .F., .F. ) 
 B_SPLINE_CURVE_WITH_KNOTS ( ( 4, 4 ),
 ( 0.4559373747858286308, 0.4950834085599552514 ),
 .UNSPECIFIED. ) 
 CURVE ( )  GEOMETRIC_REPRESENTATION_ITEM ( )  RATIONAL_B_SPLINE_CURVE ( ( 1.000000000000000000, 0.9998723030801468514, 0.9998723030801468514, 1.000000000000000000 ) ) 
 REPRESENTATION_ITEM ( '' )  );
#2538=CARTESIAN_POINT ( 'NONE',  ( -27.65886887683002726, 11.28192300254632663, -4.098983338605609816 ) ) ;
#2539=VECTOR ( 'NONE', #28558, 1000.000000000000000 ) ;
#2540=CARTESIAN_POINT ( 'NONE',  ( -37.00000000000000711, 0.000000000000000000, 0.000000000000000000 ) ) ;
#2541=DIRECTION ( 'NONE',  ( 0.000000000000000000, 0.01356324068817992522, -0.9999080150203990547 ) ) ;
#2542=ORIENTED_EDGE ( 'NONE', *, *, #25059, .F. ) ;
#2543=CARTESIAN_POINT ( 'NONE',  ( 9.269227953188480029, 6.105058365070425097, 12.04509100434534652 ) ) ;
#2545=CARTESIAN_POINT ( 'NONE',  ( 37.00000000000000711, 7.817492529713852889, -9.348667969174437431 ) ) ;
#2547=VERTEX_POINT ( 'NONE', #17137 ) ;
#2548=EDGE_LOOP ( 'NONE', ( #555, #42906, #60473, #53029 ) ) ;
#2549=CARTESIAN_POINT ( 'NONE',  ( -16.05148112979938091, 8.371939882860468529, 10.59070107784759962 ) ) ;
#2551=CARTESIAN_POINT ( 'NONE',  ( -27.19357181888462094, 12.48377454417557253, 5.138615876886901468 ) ) ;
#2552=EDGE_CURVE ( 'NONE', #42135, #11634, #2171, .T. ) ;
#2554=DIRECTION ( 'NONE',  ( 1.000000000000000000, -0.000000000000000000, 0.000000000000000000 ) ) ;
#2556=CARTESIAN_POINT ( 'NONE',  ( 37.00000000000000711, 6.711949091238143872, -10.84030624090609152 ) ) ;
#2558=DIRECTION ( 'NONE',  ( 1.000000000000000000, 0.000000000000000000, -0.000000000000000000 ) ) ;
#2562=ORIENTED_EDGE ( 'NONE', *, *, #48987, .T. ) ;
#2565=DIRECTION ( 'NONE',  ( -1.000000000000000000, 0.000000000000000000, 0.000000000000000000 ) ) ;
#2569=CARTESIAN_POINT ( 'NONE',  ( 37.00000000000000711, -6.280308599560208371, -9.926225166347007800 ) ) ;
#2570=CARTESIAN_POINT ( 'NONE',  ( -28.41827485489077532, 3.509237424706436403, 13.03592162821792222 ) ) ;
#2571=AXIS2_PLACEMENT_3D ( 'NONE', #975, #61164, #56161 ) ;
#2572=ADVANCED_FACE ( 'NONE', ( #62043 ), #10836, .T. ) ;
#2573=LINE ( 'NONE', #50725, #18514 ) ;
#2576=ADVANCED_FACE ( 'NONE', ( #42063 ), #52725, .T. ) ;
#2579=EDGE_CURVE ( 'NONE', #14758, #35654, #35134, .T. ) ;
#2580=DIRECTION ( 'NONE',  ( 0.000000000000000000, 0.01356324068818000848, -0.9999080150203990547 ) ) ;
#2582=AXIS2_PLACEMENT_3D ( 'NONE', #22580, #42842, #37862 ) ;
#2584=VERTEX_POINT ( 'NONE', #1851 ) ;
#2585=AXIS2_PLACEMENT_3D ( 'NONE', #57639, #36678, #56977 ) ;
#2586=ORIENTED_EDGE ( 'NONE', *, *, #36253, .F. ) ;
#2587=DIRECTION ( 'NONE',  ( -1.000000000000000000, 0.000000000000000000, -0.000000000000000000 ) ) ;
#2588=AXIS2_PLACEMENT_3D ( 'NONE', #1029, #15966, #21296 ) ;
#2589=EDGE_LOOP ( 'NONE', ( #35933, #7040, #52957, #50640 ) ) ;
#2590=CARTESIAN_POINT ( 'NONE',  ( -35.00000000000000000, -9.621072037177055947, 8.366449238204328509 ) ) ;
#2592=DIRECTION ( 'NONE',  ( -1.000000000000000000, -0.000000000000000000, 0.000000000000000000 ) ) ;
#2594=CARTESIAN_POINT ( 'NONE',  ( 35.00000000000000000, 4.705694406421931860E-17, -3.469127814946512892E-15 ) ) ;
#2595=EDGE_CURVE ( 'NONE', #35057, #40781, #8626, .T. ) ;
#2596=ORIENTED_EDGE ( 'NONE', *, *, #4064, .F. ) ;
#2597=CIRCLE ( 'NONE', #19571, 12.74999999999999822 ) ;
#2601=CARTESIAN_POINT ( 'NONE',  ( -35.00000000000000000, 11.26103545359856106, -3.340853584269573684 ) ) ;
#2602=EDGE_CURVE ( 'NONE', #51996, #19892, #7527, .T. ) ;
#2603=CIRCLE ( 'NONE', #52479, 12.74999999999999822 ) ;
#2604=EDGE_CURVE ( 'NONE', #3374, #31862, #32415, .T. ) ;
#2607=ORIENTED_EDGE ( 'NONE', *, *, #908, .T. ) ;
#2609=CARTESIAN_POINT ( 'NONE',  ( 29.29356854117942177, 11.61667008512750598, 6.891473480132332519 ) ) ;
#2610=VECTOR ( 'NONE', #61883, 1000.000000000000000 ) ;
#2612=EDGE_CURVE ( 'NONE', #39541, #30999, #6493, .T. ) ;
#2613=ORIENTED_EDGE ( 'NONE', *, *, #45161, .T. ) ;
#2614=CARTESIAN_POINT ( 'NONE',  ( -11.40165637462999548, -7.140361382672671731, -11.46568811481329320 ) ) ;
#2616=DIRECTION ( 'NONE',  ( 1.000000000000000000, 0.000000000000000000, 0.000000000000000000 ) ) ;
#2622=ORIENTED_EDGE ( 'NONE', *, *, #56044, .F. ) ;
#2623=CARTESIAN_POINT ( 'NONE',  ( 34.00000000000000000, 1.267509437117510519E-14, 0.000000000000000000 ) ) ;
#2626=CARTESIAN_POINT ( 'NONE',  ( -19.47984447937493613, -1.416020129149132334, 25.00000000000000000 ) ) ;
#2630=EDGE_LOOP ( 'NONE', ( #53656, #57220, #39139, #9933 ) ) ;
#2631=CIRCLE ( 'NONE', #4763, 12.75000000000000178 ) ;
#2632=VERTEX_POINT ( 'NONE', #52403 ) ;
#2635=ORIENTED_EDGE ( 'NONE', *, *, #54269, .T. ) ;
#2637=SURFACE_STYLE_FILL_AREA ( #47829 ) ;
#2639=DIRECTION ( 'NONE',  ( 0.000000000000000000, 0.000000000000000000, -1.000000000000000000 ) ) ;
#2640=EDGE_CURVE ( 'NONE', #57837, #60506, #33011, .T. ) ;
#2642=ORIENTED_EDGE ( 'NONE', *, *, #31297, .F. ) ;
#2643=DIRECTION ( 'NONE',  ( 1.000000000000000000, 0.000000000000000000, -0.000000000000000000 ) ) ;
#2644=CARTESIAN_POINT ( 'NONE',  ( -29.43980975494970309, -3.641506875706030488, 12.99959336572439561 ) ) ;
#2650=DIRECTION ( 'NONE',  ( 0.000000000000000000, -1.000000000000000000, 0.000000000000000000 ) ) ;
#2651=EDGE_CURVE ( 'NONE', #28214, #62051, #55328, .T. ) ;
#2655=AXIS2_PLACEMENT_3D ( 'NONE', #36098, #10849, #41096 ) ;
#2657=DIRECTION ( 'NONE',  ( -1.000000000000000000, 0.000000000000000000, 0.000000000000000000 ) ) ;
#2659=CARTESIAN_POINT ( 'NONE',  ( 35.00000000000000000, 9.060822531526046220, -7.474872387601039669 ) ) ;
#2660=EDGE_CURVE ( 'NONE', #41862, #6306, #7153, .T. ) ;
#2665=DIRECTION ( 'NONE',  ( -1.000000000000000000, 0.000000000000000000, 0.000000000000000000 ) ) ;
#2669=CARTESIAN_POINT ( 'NONE',  ( 35.00000000000000000, -0.7008968033239626472, -12.16632754454236576 ) ) ;
#2671=DIRECTION ( 'NONE',  ( 1.000000000000000000, 0.000000000000000000, -0.000000000000000000 ) ) ;
#2672=CARTESIAN_POINT ( 'NONE',  ( -27.31123137524929589, -10.57279367158372452, -8.394978051634900851 ) ) ;
#2673=VECTOR ( 'NONE', #38869, 1000.000000000000000 ) ;
#2674=EDGE_LOOP ( 'NONE', ( #5927, #12896, #37205, #6932 ) ) ;
#2676=DIRECTION ( 'NONE',  ( 0.000000000000000000, 0.9847383929261624980, -0.1740410799127578012 ) ) ;
#2678=CARTESIAN_POINT ( 'NONE',  ( -11.40165637463000436, -7.977372332587114201, 8.984547431638254977 ) ) ;
#2680=DIRECTION ( 'NONE',  ( -1.000000000000000000, 0.000000000000000000, 0.000000000000000000 ) ) ;
#2683=ORIENTED_EDGE ( 'NONE', *, *, #3424, .T. ) ;
#2686=CARTESIAN_POINT ( 'NONE',  ( -35.00000000000000000, 0.000000000000000000, 0.000000000000000000 ) ) ;
#2687=LINE ( 'NONE', #43870, #355 ) ;
#2691=EDGE_CURVE ( 'NONE', #29107, #17242, #13445, .T. ) ;
#2692=DIRECTION ( 'NONE',  ( 0.000000000000000000, -0.01356324068817998940, 0.9999080150203990547 ) ) ;
#2694=ORIENTED_EDGE ( 'NONE', *, *, #462, .T. ) ;
#2697=DIRECTION ( 'NONE',  ( -1.000000000000000000, 0.000000000000000000, 0.000000000000000000 ) ) ;
#2698=DIRECTION ( 'NONE',  ( 1.000000000000000000, 0.000000000000000000, 0.000000000000000000 ) ) ;
#2699=AXIS2_PLACEMENT_3D ( 'NONE', #64569, #33007, #39647 ) ;
#2700=ORIENTED_EDGE ( 'NONE', *, *, #12386, .F. ) ;
#2701=DIRECTION ( 'NONE',  ( 0.000000000000000000, -0.9467777615094604693, -0.3218879778915876289 ) ) ;
#2702=ORIENTED_EDGE ( 'NONE', *, *, #47798, .T. ) ;
#2703=CARTESIAN_POINT ( 'NONE',  ( -18.01337138201670030, 3.271325267346269161, 11.54736685641333160 ) ) ;
#2705=CARTESIAN_POINT ( 'NONE',  ( 36.00000000000000711, 7.882940143791775434, -10.02106554660711701 ) ) ;
#2710=ORIENTED_EDGE ( 'NONE', *, *, #39070, .T. ) ;
#2712=AXIS2_PLACEMENT_3D ( 'NONE', #43683, #48380, #14076 ) ;
#2713=CYLINDRICAL_SURFACE ( 'NONE', #41655, 12.74999999999999822 ) ;
#2716=CARTESIAN_POINT ( 'NONE',  ( 35.00000000000000000, 4.705694406421931860E-17, -3.469127814946512892E-15 ) ) ;
#2718=EDGE_CURVE ( 'NONE', #29384, #11130, #33416, .T. ) ;
#2719=EDGE_LOOP ( 'NONE', ( #32378, #45023, #65484, #60596 ) ) ;
#2720=FACE_OUTER_BOUND ( 'NONE', #7014, .T. ) ;
#2722=DIRECTION ( 'NONE',  ( 1.000000000000000000, 0.000000000000000000, -0.000000000000000000 ) ) ;
#2724=ORIENTED_EDGE ( 'NONE', *, *, #48916, .T. ) ;
#2725=CARTESIAN_POINT ( 'NONE',  ( 35.00000000000000000, 11.07407352312218052, 3.916263239775223504 ) ) ;
#2726=ORIENTED_EDGE ( 'NONE', *, *, #3503, .T. ) ;
#2728=CARTESIAN_POINT ( 'NONE',  ( 9.222597103870787905, 1.921402420396019828, -13.36471210326569725 ) ) ;
#2729=EDGE_LOOP ( 'NONE', ( #58236, #27164, #39804, #57675 ) ) ;
#2730=EDGE_CURVE ( 'NONE', #9320, #16904, #18178, .T. ) ;
#2732=CARTESIAN_POINT ( 'NONE',  ( 35.00000000000000000, 4.705694406421931860E-17, -3.469127814946512892E-15 ) ) ;
#2733=FACE_OUTER_BOUND ( 'NONE', #18156, .T. ) ;
#2736=CARTESIAN_POINT ( 'NONE',  ( -27.28559572956275758, -11.69480911083762642, -2.740757448209772740 ) ) ;
#2739=VECTOR ( 'NONE', #36907, 1000.000000000000000 ) ;
#2740=ORIENTED_EDGE ( 'NONE', *, *, #51926, .T. ) ;
#2744=ADVANCED_FACE ( 'NONE', ( #8145 ), #49397, .T. ) ;
#2745=ORIENTED_EDGE ( 'NONE', *, *, #1284, .T. ) ;
#2746=CYLINDRICAL_SURFACE ( 'NONE', #2050, 12.74999999999999822 ) ;
#2749=ADVANCED_FACE ( 'NONE', ( #44048 ), #13130, .T. ) ;
#2750=CIRCLE ( 'NONE', #50521, 12.75000000000000178 ) ;
#2751=ORIENTED_EDGE ( 'NONE', *, *, #20214, .T. ) ;
#2755=VERTEX_POINT ( 'NONE', #38057 ) ;
#2757=CARTESIAN_POINT ( 'NONE',  ( -3.191454007415039040, -11.27527210208590347, 4.125543110481471487 ) ) ;
#2759=CARTESIAN_POINT ( 'NONE',  ( -35.00000000000000000, -8.352657516904613999, -8.258652103341526995 ) ) ;
#2760=CARTESIAN_POINT ( 'NONE',  ( -18.01369897008283161, -9.089080147352223804, 7.856079936729432056 ) ) ;
#2761=ORIENTED_EDGE ( 'NONE', *, *, #12161, .F. ) ;
#2762=CARTESIAN_POINT ( 'NONE',  ( -47.00000000000000711, 0.000000000000000000, 0.000000000000000000 ) ) ;
#2764=AXIS2_PLACEMENT_3D ( 'NONE', #12947, #33874, #28247 ) ;
#2765=EDGE_CURVE ( 'NONE', #49572, #57602, #26663, .T. ) ;
#2767=CARTESIAN_POINT ( 'NONE',  ( 22.36482863261543486, 13.46837713145128923, -0.9234811557364158707 ) ) ;
#2774=AXIS2_PLACEMENT_3D ( 'NONE', #11467, #1528, #12126 ) ;
#2775=ORIENTED_EDGE ( 'NONE', *, *, #59116, .T. ) ;
#2776=LINE ( 'NONE', #64550, #2405 ) ;
#2779=ORIENTED_EDGE ( 'NONE', *, *, #24683, .T. ) ;
#2780=CARTESIAN_POINT ( 'NONE',  ( -35.00000000000000000, -11.16627499335652374, -3.645068577060142978 ) ) ;
#2781=ORIENTED_EDGE ( 'NONE', *, *, #56167, .F. ) ;
#2783=ORIENTED_EDGE ( 'NONE', *, *, #473, .F. ) ;
#2784=ORIENTED_EDGE ( 'NONE', *, *, #15216, .T. ) ;
#2785=CARTESIAN_POINT ( 'NONE',  ( 29.52102924165219378, -11.15227936632555483, 7.620086186309502629 ) ) ;
#2788=VERTEX_POINT ( 'NONE', #13764 ) ;
#2790=CARTESIAN_POINT ( 'NONE',  ( -27.45775109278351067, 8.499184579339635448, -8.471355351200609007 ) ) ;
#2792=CARTESIAN_POINT ( 'NONE',  ( 37.00000000000000711, -5.636262487437393887, -10.80478261802180207 ) ) ;
#2793=EDGE_CURVE ( 'NONE', #56080, #29748, #47889, .T. ) ;
#2795=DIRECTION ( 'NONE',  ( -1.000000000000000000, -0.000000000000000000, 0.000000000000000000 ) ) ;
#2796=DIRECTION ( 'NONE',  ( 1.000000000000000000, 0.000000000000000000, -0.000000000000000000 ) ) ;
#2798=CARTESIAN_POINT ( 'NONE',  ( -25.29775422704755172, 10.32001691524481402, 6.125646727044483875 ) ) ;
#2799=ORIENTED_EDGE ( 'NONE', *, *, #59038, .T. ) ;
#2800=DIRECTION ( 'NONE',  ( -0.000000000000000000, -1.000000000000000000, -0.000000000000000000 ) ) ;
#2802=DIRECTION ( 'NONE',  ( 1.000000000000000000, 0.000000000000000000, 0.000000000000000000 ) ) ;
#2804=CARTESIAN_POINT ( 'NONE',  ( 37.00000000000000711, 11.10408318471059452, -6.265926637539536159 ) ) ;
#2806=DIRECTION ( 'NONE',  ( -1.000000000000000000, 0.000000000000000000, 0.000000000000000000 ) ) ;
#2807=CARTESIAN_POINT ( 'NONE',  ( 35.00000000000000000, -1.171570255487531131, -11.68758509253248157 ) ) ;
#2808=EDGE_CURVE ( 'NONE', #39817, #40383, #60643, .T. ) ;
#2813=FACE_OUTER_BOUND ( 'NONE', #29033, .T. ) ;
#2814=ORIENTED_EDGE ( 'NONE', *, *, #43181, .T. ) ;
#2815=EDGE_CURVE ( 'NONE', #14551, #6535, #14968, .T. ) ;
#2817=CARTESIAN_POINT ( 'NONE',  ( 35.00000000000000000, 11.74226168163341377, 0.3025107581129941048 ) ) ;
#2819=CARTESIAN_POINT ( 'NONE',  ( -18.25240752046768833, -11.98742856354572339, 0.6375846530299378312 ) ) ;
#2825=AXIS2_PLACEMENT_3D ( 'NONE', #6144, #26405, #1147 ) ;
#2826=LINE ( 'NONE', #39017, #65216 ) ;
#2827=AXIS2_PLACEMENT_3D ( 'NONE', #48964, #53285, #3085 ) ;
#2828=ORIENTED_EDGE ( 'NONE', *, *, #34295, .T. ) ;
#2831=FACE_OUTER_BOUND ( 'NONE', #40202, .T. ) ;
#2832=EDGE_CURVE ( 'NONE', #2026, #5091, #45792, .T. ) ;
#2833=CARTESIAN_POINT ( 'NONE',  ( -37.00000000000000711, 1.908798535168378274, 12.60630747491664039 ) ) ;
#2835=LINE ( 'NONE', #2151, #4428 ) ;
#2836=CARTESIAN_POINT ( 'NONE',  ( -10.90165637462999548, -7.338442233538555293, 11.33311006114865016 ) ) ;
#2837=ORIENTED_EDGE ( 'NONE', *, *, #58030, .F. ) ;
#2841=EDGE_CURVE ( 'NONE', #10202, #44435, #31966, .T. ) ;
#2842=DIRECTION ( 'NONE',  ( 1.000000000000000000, 0.000000000000000000, 0.000000000000000000 ) ) ;
#2843=CARTESIAN_POINT ( 'NONE',  ( -24.79843077534458118, -10.56684401205973067, 8.408718480432709086 ) ) ;
#2844=VERTEX_POINT ( 'NONE', #30054 ) ;
#2845=CYLINDRICAL_SURFACE ( 'NONE', #288, 2.809571291727933851 ) ;
#2848=EDGE_LOOP ( 'NONE', ( #49569, #20665, #41019, #53208 ) ) ;
#2849=CARTESIAN_POINT ( 'NONE',  ( -37.00000000000000711, 0.000000000000000000, 0.000000000000000000 ) ) ;
#2850=CARTESIAN_POINT ( 'NONE',  ( -37.00000000000000711, 10.91536515067641844, 4.339012074900148619 ) ) ;
#2852=ORIENTED_EDGE ( 'NONE', *, *, #39819, .F. ) ;
#2853=VECTOR ( 'NONE', #40637, 1000.000000000000000 ) ;
#2854=CARTESIAN_POINT ( 'NONE',  ( -10.48620311856347875, -9.720786832536937538, 25.00000000000000000 ) ) ;
#2855=AXIS2_PLACEMENT_3D ( 'NONE', #34707, #49703, #39720 ) ;
#2856=ORIENTED_EDGE ( 'NONE', *, *, #10380, .F. ) ;
#2857=CARTESIAN_POINT ( 'NONE',  ( 35.00000000000000000, 8.352657516904789858, 8.258652103341336925 ) ) ;
#2858=DIRECTION ( 'NONE',  ( 0.000000000000000000, -0.01356324068817998940, 0.9999080150203990547 ) ) ;
#2859=CARTESIAN_POINT ( 'NONE',  ( -35.00000000000000000, -7.474872387600942858, -9.060822531526127932 ) ) ;
#2862=DIRECTION ( 'NONE',  ( 0.000000000000000000, 0.6745969609292664648, 0.7381862504171951000 ) ) ;
#2866=VERTEX_POINT ( 'NONE', #29398 ) ;
#2867=EDGE_CURVE ( 'NONE', #17595, #52959, #27700, .T. ) ;
#2868=CARTESIAN_POINT ( 'NONE',  ( 9.582000644489843566, 6.678480302218151365, 11.73685885562068698 ) ) ;
#2869=VERTEX_POINT ( 'NONE', #30695 ) ;
#2870=CARTESIAN_POINT ( 'NONE',  ( 0.2851083653049504285, -0.4107471485392698018, -11.99296822225284131 ) ) ;
#2872=ORIENTED_EDGE ( 'NONE', *, *, #6828, .T. ) ;
#2874=CARTESIAN_POINT ( 'NONE',  ( -24.92192216651048042, 9.674054327626246064, 9.421735467875462788 ) ) ;
#2876=FACE_OUTER_BOUND ( 'NONE', #28107, .T. ) ;
#2877=ADVANCED_FACE ( 'NONE', ( #49695 ), #14738, .T. ) ;
#2880=CARTESIAN_POINT ( 'NONE',  ( -18.08686583997218733, 5.151216734910788908, 12.47858029384653733 ) ) ;
#2881=EDGE_LOOP ( 'NONE', ( #38268, #60198, #62102, #14492 ) ) ;
#2882=CARTESIAN_POINT ( 'NONE',  ( 37.00000000000000711, -0.06441628369827803735, 12.18632975068352309 ) ) ;
#2883=CARTESIAN_POINT ( 'NONE',  ( -36.00000000000000711, -3.640372113593638659, 12.21925492305361161 ) ) ;
#2884=DIRECTION ( 'NONE',  ( -1.000000000000000000, 0.000000000000000000, -0.000000000000000000 ) ) ;
#2885=ORIENTED_EDGE ( 'NONE', *, *, #57234, .T. ) ;
#2887=ORIENTED_EDGE ( 'NONE', *, *, #65660, .F. ) ;
#2888=CARTESIAN_POINT ( 'NONE',  ( 37.00000000000000711, 4.705694406421931860E-17, -3.469127814946512892E-15 ) ) ;
#2891=DIRECTION ( 'NONE',  ( -1.000000000000000000, -0.000000000000000000, 0.000000000000000000 ) ) ;
#2892=CARTESIAN_POINT ( 'NONE',  ( -35.00000000000000000, -6.917234959366895808, 9.493370459201672773 ) ) ;
#2893=CARTESIAN_POINT ( 'NONE',  ( 22.88594695219327235, 3.421158645304719137, 25.00000000000000000 ) ) ;
#2894=EDGE_CURVE ( 'NONE', #58474, #4846, #34698, .T. ) ;
#2895=EDGE_LOOP ( 'NONE', ( #56832, #21515, #23366, #1932 ) ) ;
#2896=CARTESIAN_POINT ( 'NONE',  ( -36.00000000000000711, -2.865935305911713638, 12.42372387097881514 ) ) ;
#2897=CIRCLE ( 'NONE', #40021, 5.000000000000000888 ) ;
#2898=ORIENTED_EDGE ( 'NONE', *, *, #18521, .F. ) ;
#2900=CARTESIAN_POINT ( 'NONE',  ( -35.00000000000000000, 8.766823244862097297, -7.817610399097422835 ) ) ;
#2901=CIRCLE ( 'NONE', #1841, 4.999999999999999112 ) ;
#2902=CARTESIAN_POINT ( 'NONE',  ( 36.00000000000000711, -6.564808257521689505, 10.93004082984025160 ) ) ;
#2903=CARTESIAN_POINT ( 'NONE',  ( -35.00000000000000000, -11.71932350927023414, 3.511386971104906163 ) ) ;
#2904=LINE ( 'NONE', #42778, #6808 ) ;
#2907=CARTESIAN_POINT ( 'NONE',  ( -28.85619398320021745, 3.750539801530000439, -11.39883551934754280 ) ) ;
#2909=FACE_OUTER_BOUND ( 'NONE', #53583, .T. ) ;
#2915=EDGE_CURVE ( 'NONE', #23899, #52056, #51122, .T. ) ;
#2918=( BOUNDED_CURVE ( )  B_SPLINE_CURVE ( 3, ( #43238, #17986, #38247, #53582 ),
 .UNSPECIFIED., .F., .F. ) 
 B_SPLINE_CURVE_WITH_KNOTS ( ( 4, 4 ),
 ( 4.678153363932756825, 4.712388980384688786 ),
 .UNSPECIFIED. ) 
 CURVE ( )  GEOMETRIC_REPRESENTATION_ITEM ( )  RATIONAL_B_SPLINE_CURVE ( ( 1.000000000000000000, 0.9999023292654991568, 0.9999023292654991568, 1.000000000000000000 ) ) 
 REPRESENTATION_ITEM ( '' )  );
#2920=CARTESIAN_POINT ( 'NONE',  ( 37.00000000000000711, -10.93004082984022851, -6.564808257521734802 ) ) ;
#2921=CARTESIAN_POINT ( 'NONE',  ( 35.00000000000000000, 4.705694406421931860E-17, -3.469127814946512892E-15 ) ) ;
#2923=ORIENTED_EDGE ( 'NONE', *, *, #38317, .T. ) ;
#2925=CARTESIAN_POINT ( 'NONE',  ( 37.00000000000000711, -10.91072401419414462, -5.428340790341669830 ) ) ;
#2926=CARTESIAN_POINT ( 'NONE',  ( 35.00000000000000000, 11.23004253107771078, 4.732539170486136371 ) ) ;
#2927=CARTESIAN_POINT ( 'NONE',  ( 37.00000000000000711, 4.705694406421931860E-17, -3.469127814946512892E-15 ) ) ;
#2929=EDGE_CURVE ( 'NONE', #19851, #45626, #57484, .T. ) ;
#2931=CARTESIAN_POINT ( 'NONE',  ( -35.00000000000000000, 9.557269938331666381, -7.561043153947866635 ) ) ;
#2933=DIRECTION ( 'NONE',  ( -1.000000000000000000, -1.836970198721029688E-16, -0.000000000000000000 ) ) ;
#2936=( BOUNDED_CURVE ( )  B_SPLINE_CURVE ( 3, ( #23598, #43868, #14253, #49837 ),
 .UNSPECIFIED., .F., .F. ) 
 B_SPLINE_CURVE_WITH_KNOTS ( ( 4, 4 ),
 ( 0.7870380171267665759, 0.8138757160357118492 ),
 .UNSPECIFIED. ) 
 CURVE ( )  GEOMETRIC_REPRESENTATION_ITEM ( )  RATIONAL_B_SPLINE_CURVE ( ( 1.000000000000000000, 0.9999399790604226457, 0.9999399790604226457, 1.000000000000000000 ) ) 
 REPRESENTATION_ITEM ( '' )  );
#2937=DIRECTION ( 'NONE',  ( 1.000000000000000000, -0.000000000000000000, 0.000000000000000000 ) ) ;
#2938=CARTESIAN_POINT ( 'NONE',  ( -36.00000000000000711, -11.10408318471063893, 6.265926637539455335 ) ) ;
#2943=ADVANCED_FACE ( 'NONE', ( #40346 ), #60644, .T. ) ;
#2944=VERTEX_POINT ( 'NONE', #64966 ) ;
#2946=ORIENTED_EDGE ( 'NONE', *, *, #22340, .T. ) ;
#2947=VECTOR ( 'NONE', #29132, 1000.000000000000000 ) ;
#2951=ADVANCED_FACE ( 'NONE', ( #14425 ), #64629, .T. ) ;
#2953=ORIENTED_EDGE ( 'NONE', *, *, #22959, .F. ) ;
#2954=DIRECTION ( 'NONE',  ( 0.000000000000000000, 0.01356324068818000848, -0.9999080150203990547 ) ) ;
#2955=LINE ( 'NONE', #34164, #34793 ) ;
#2958=ORIENTED_EDGE ( 'NONE', *, *, #53017, .F. ) ;
#2959=ORIENTED_EDGE ( 'NONE', *, *, #35908, .T. ) ;
#2961=ORIENTED_EDGE ( 'NONE', *, *, #7551, .T. ) ;
#2962=DIRECTION ( 'NONE',  ( -0.000000000000000000, -0.000000000000000000, -1.000000000000000000 ) ) ;
#2967=CARTESIAN_POINT ( 'NONE',  ( -35.00000000000000000, 0.000000000000000000, 0.000000000000000000 ) ) ;
#2969=DIRECTION ( 'NONE',  ( -1.000000000000000000, 0.000000000000000000, -0.000000000000000000 ) ) ;
#2971=ADVANCED_FACE ( 'NONE', ( #27040 ), #47002, .T. ) ;
#2972=DIRECTION ( 'NONE',  ( 0.000000000000000000, -0.01356324068817991828, 0.9999080150203990547 ) ) ;
#2973=ORIENTED_EDGE ( 'NONE', *, *, #32600, .F. ) ;
#2974=LINE ( 'NONE', #8269, #30672 ) ;
#2976=EDGE_CURVE ( 'NONE', #6394, #47785, #29876, .T. ) ;
#2979=CARTESIAN_POINT ( 'NONE',  ( -18.04458733766117362, 12.91933584589294703, 3.916728392552376370 ) ) ;
#2980=DIRECTION ( 'NONE',  ( 1.000000000000000000, 0.000000000000000000, 0.000000000000000000 ) ) ;
#2984=AXIS2_PLACEMENT_3D ( 'NONE', #13475, #8495, #59372 ) ;
#2985=ORIENTED_EDGE ( 'NONE', *, *, #22245, .F. ) ;
#2988=ORIENTED_EDGE ( 'NONE', *, *, #46326, .F. ) ;
#2989=CARTESIAN_POINT ( 'NONE',  ( -35.00000000000000000, 0.000000000000000000, 0.000000000000000000 ) ) ;
#2991=CARTESIAN_POINT ( 'NONE',  ( 12.73187067999545263, -12.88776733229570759, -4.024014788385745334 ) ) ;
#2992=CIRCLE ( 'NONE', #10402, 12.75000000000000178 ) ;
#2993=DIRECTION ( 'NONE',  ( -1.000000000000000000, 0.000000000000000000, 0.000000000000000000 ) ) ;
#2997=CARTESIAN_POINT ( 'NONE',  ( -35.00000000000000000, 0.000000000000000000, 0.000000000000000000 ) ) ;
#2999=AXIS2_PLACEMENT_3D ( 'NONE', #45318, #35327, #55639 ) ;
#3002=EDGE_CURVE ( 'NONE', #14430, #37563, #32339, .T. ) ;
#3003=DIRECTION ( 'NONE',  ( 1.000000000000000000, 0.000000000000000000, -0.000000000000000000 ) ) ;
#3005=CARTESIAN_POINT ( 'NONE',  ( -35.00000000000000000, -8.551552972817024312, -8.052525312709976291 ) ) ;
#3006=FACE_OUTER_BOUND ( 'NONE', #47177, .T. ) ;
#3007=CARTESIAN_POINT ( 'NONE',  ( -35.00000000000000000, 10.01317267707896441, -6.946017217729827387 ) ) ;
#3008=ADVANCED_FACE ( 'NONE', ( #56663 ), #15727, .T. ) ;
#3009=EDGE_CURVE ( 'NONE', #46698, #18117, #54352, .T. ) ;
#3010=VERTEX_POINT ( 'NONE', #46023 ) ;
#3012=CARTESIAN_POINT ( 'NONE',  ( 36.00000000000000711, 4.824807283154290971, 11.80185301892974969 ) ) ;
#3013=ORIENTED_EDGE ( 'NONE', *, *, #11270, .F. ) ;
#3016=CARTESIAN_POINT ( 'NONE',  ( 35.00000000000000000, 11.95840593935204765, 2.346765782874299155 ) ) ;
#3017=VECTOR ( 'NONE', #2565, 1000.000000000000000 ) ;
#3018=CARTESIAN_POINT ( 'NONE',  ( 35.00000000000000000, 11.61175578952788356, 1.771820996347031940 ) ) ;
#3019=DIRECTION ( 'NONE',  ( 0.000000000000000000, 0.01356324068817991828, -0.9999080150203990547 ) ) ;
#3021=EDGE_CURVE ( 'NONE', #40781, #57018, #62826, .T. ) ;
#3022=ORIENTED_EDGE ( 'NONE', *, *, #52424, .T. ) ;
#3025=AXIS2_PLACEMENT_3D ( 'NONE', #40471, #10534, #49813 ) ;
#3026=DIRECTION ( 'NONE',  ( -1.000000000000000000, 0.000000000000000000, 0.000000000000000000 ) ) ;
#3027=ORIENTED_EDGE ( 'NONE', *, *, #51591, .F. ) ;
#3028=FACE_OUTER_BOUND ( 'NONE', #17338, .T. ) ;
#3031=AXIS2_PLACEMENT_3D ( 'NONE', #11825, #32108, #47434 ) ;
#3033=LINE ( 'NONE', #63198, #22237 ) ;
#3034=EDGE_CURVE ( 'NONE', #58117, #10303, #51351, .T. ) ;
#3036=VERTEX_POINT ( 'NONE', #16065 ) ;
#3037=VERTEX_POINT ( 'NONE', #11406 ) ;
#3041=CYLINDRICAL_SURFACE ( 'NONE', #52851, 12.75000000000000178 ) ;
#3042=VERTEX_POINT ( 'NONE', #42295 ) ;
#3043=AXIS2_PLACEMENT_3D ( 'NONE', #50798, #20542, #31175 ) ;
#3045=EDGE_CURVE ( 'NONE', #35492, #37945, #26709, .T. ) ;
#3049=DIRECTION ( 'NONE',  ( 0.3902440745007897949, -0.000000000000000000, 0.9207114435679737419 ) ) ;
#3051=VERTEX_POINT ( 'NONE', #21739 ) ;
#3053=CARTESIAN_POINT ( 'NONE',  ( 37.00000000000000711, -1.457575200925456560, 12.66641127287626745 ) ) ;
#3054=ORIENTED_EDGE ( 'NONE', *, *, #47180, .F. ) ;
#3055=CARTESIAN_POINT ( 'NONE',  ( 35.00000000000000000, -9.557269938331497627, 7.561043153948066475 ) ) ;
#3057=EDGE_CURVE ( 'NONE', #62587, #11696, #27743, .T. ) ;
#3058=ORIENTED_EDGE ( 'NONE', *, *, #18484, .T. ) ;
#3059=CARTESIAN_POINT ( 'NONE',  ( 24.97632970311353162, 10.66122974065908657, -8.283959357202872908 ) ) ;
#3061=DIRECTION ( 'NONE',  ( 1.000000000000000000, 0.000000000000000000, 0.000000000000000000 ) ) ;
#3063=AXIS2_PLACEMENT_3D ( 'NONE', #16, #19667, #20946 ) ;
#3064=VERTEX_POINT ( 'NONE', #23358 ) ;
#3065=CARTESIAN_POINT ( 'NONE',  ( -35.00000000000000000, 11.53507381115580444, 2.216820770815288721 ) ) ;
#3066=AXIS2_PLACEMENT_3D ( 'NONE', #32125, #42413, #7513 ) ;
#3067=VERTEX_POINT ( 'NONE', #27677 ) ;
#3068=DIRECTION ( 'NONE',  ( -0.000000000000000000, -1.000000000000000000, -0.000000000000000000 ) ) ;
#3069=CARTESIAN_POINT ( 'NONE',  ( 26.34661844826604593, -11.53221627053866527, 3.317828791472333005 ) ) ;
#3070=CARTESIAN_POINT ( 'NONE',  ( -35.00000000000000000, -3.805206332242558886, 12.16893194857548721 ) ) ;
#3071=CARTESIAN_POINT ( 'NONE',  ( -3.543971956890883401, 9.152513797769646686, 7.771635824158136252 ) ) ;
#3072=CARTESIAN_POINT ( 'NONE',  ( -17.63957941232862225, -7.319940456796631523, 9.513823268653226251 ) ) ;
#3076=VECTOR ( 'NONE', #18172, 1000.000000000000000 ) ;
#3077=EDGE_CURVE ( 'NONE', #3342, #1280, #55378, .T. ) ;
#3079=AXIS2_PLACEMENT_3D ( 'NONE', #33922, #3713, #64199 ) ;
#3083=VECTOR ( 'NONE', #21615, 1000.000000000000000 ) ;
#3084=DIRECTION ( 'NONE',  ( -0.4298323628305344979, -0.9029087107030918657, 0.000000000000000000 ) ) ;
#3085=DIRECTION ( 'NONE',  ( 0.000000000000000000, -0.01356324068817991828, 0.9999080150203990547 ) ) ;
#3087=ADVANCED_FACE ( 'NONE', ( #60156 ), #47984, .T. ) ;
#3088=ORIENTED_EDGE ( 'NONE', *, *, #10282, .F. ) ;
#3089=CARTESIAN_POINT ( 'NONE',  ( 12.70099391640234465, -11.34186981777373759, -3.924130698594886280 ) ) ;
#3090=ORIENTED_EDGE ( 'NONE', *, *, #18942, .F. ) ;
#3092=CARTESIAN_POINT ( 'NONE',  ( 8.937200413559443390, 4.476360154859203355, -11.13383131558893346 ) ) ;
#3093=CARTESIAN_POINT ( 'NONE',  ( 35.00000000000000000, 4.705694406421931860E-17, -3.469127814946512892E-15 ) ) ;
#3094=ORIENTED_EDGE ( 'NONE', *, *, #21650, .F. ) ;
#3095=CARTESIAN_POINT ( 'NONE',  ( 22.68139259647346861, 3.158742727684421769, -13.12595410559641529 ) ) ;
#3096=LINE ( 'NONE', #43630, #12897 ) ;
#3097=EDGE_LOOP ( 'NONE', ( #52112, #62138, #26968, #41318 ) ) ;
#3098=ADVANCED_FACE ( 'NONE', ( #38658 ), #32988, .T. ) ;
#3099=ORIENTED_EDGE ( 'NONE', *, *, #9674, .F. ) ;
#3100=ORIENTED_EDGE ( 'NONE', *, *, #31329, .T. ) ;
#3102=ADVANCED_FACE ( 'NONE', ( #28346 ), #14275, .T. ) ;
#3104=AXIS2_PLACEMENT_3D ( 'NONE', #48862, #3317, #23591 ) ;
#3106=DIRECTION ( 'NONE',  ( 0.000000000000000000, -0.01356324068817998940, 0.9999080150203990547 ) ) ;
#3110=ORIENTED_EDGE ( 'NONE', *, *, #36810, .T. ) ;
#3112=AXIS2_PLACEMENT_3D ( 'NONE', #57338, #36724, #37711 ) ;
#3113=CARTESIAN_POINT ( 'NONE',  ( 37.00000000000000711, -11.61175578952786758, -1.771820996347120092 ) ) ;
#3114=FACE_OUTER_BOUND ( 'NONE', #20761, .T. ) ;
#3116=ORIENTED_EDGE ( 'NONE', *, *, #64620, .F. ) ;
#3118=ORIENTED_EDGE ( 'NONE', *, *, #39032, .F. ) ;
#3119=DIRECTION ( 'NONE',  ( -1.000000000000000000, 0.000000000000000000, -0.000000000000000000 ) ) ;
#3122=CARTESIAN_POINT ( 'NONE',  ( -37.00000000000000711, -2.021542716731318912, -12.01765980939844169 ) ) ;
#3127=FACE_OUTER_BOUND ( 'NONE', #29561, .T. ) ;
#3128=CARTESIAN_POINT ( 'NONE',  ( -10.65303786363494964, -5.744948954241079875, -12.22272377441934665 ) ) ;
#3130=EDGE_CURVE ( 'NONE', #24709, #29997, #23039, .T. ) ;
#3131=AXIS2_PLACEMENT_3D ( 'NONE', #63324, #26783, #16797 ) ;
#3133=ORIENTED_EDGE ( 'NONE', *, *, #13676, .T. ) ;
#3134=DIRECTION ( 'NONE',  ( -1.000000000000000000, 0.000000000000000000, -0.000000000000000000 ) ) ;
#3135=ORIENTED_EDGE ( 'NONE', *, *, #16718, .F. ) ;
#3136=EDGE_CURVE ( 'NONE', #3037, #23216, #36240, .T. ) ;
#3137=ORIENTED_EDGE ( 'NONE', *, *, #29275, .F. ) ;
#3143=DIRECTION ( 'NONE',  ( -1.000000000000000000, -0.000000000000000000, 0.000000000000000000 ) ) ;
#3144=EDGE_CURVE ( 'NONE', #46242, #60760, #3096, .T. ) ;
#3145=CYLINDRICAL_SURFACE ( 'NONE', #48263, 12.74999999999999822 ) ;
#3148=DIRECTION ( 'NONE',  ( -1.000000000000000000, 0.000000000000000000, 0.000000000000000000 ) ) ;
#3149=CARTESIAN_POINT ( 'NONE',  ( 35.00000000000000000, -5.710938531231789739, -11.39945968423469402 ) ) ;
#3151=FACE_OUTER_BOUND ( 'NONE', #10072, .T. ) ;
#3152=AXIS2_PLACEMENT_3D ( 'NONE', #48782, #28811, #49123 ) ;
#3153=EDGE_CURVE ( 'NONE', #18713, #38075, #19265, .T. ) ;
#3154=VECTOR ( 'NONE', #21270, 1000.000000000000000 ) ;
#3155=CARTESIAN_POINT ( 'NONE',  ( -35.00000000000000000, -2.346765782874520312, 11.95840593935200680 ) ) ;
#3156=CARTESIAN_POINT ( 'NONE',  ( -10.86457796283016997, -6.815227495106873867, 11.65522549784055073 ) ) ;
#3162=DIRECTION ( 'NONE',  ( -0.000000000000000000, -0.000000000000000000, -1.000000000000000000 ) ) ;
#3163=CIRCLE ( 'NONE', #29707, 4.999999999999999112 ) ;
#3167=CARTESIAN_POINT ( 'NONE',  ( -17.68998094701642643, 2.870745959822725624, -11.65346102617277602 ) ) ;
#3168=VERTEX_POINT ( 'NONE', #40525 ) ;
#3170=CARTESIAN_POINT ( 'NONE',  ( -35.00000000000000000, -0.7536123767499333104, 11.72195762423409704 ) ) ;
#3172=ADVANCED_FACE ( 'NONE', ( #15259 ), #60821, .T. ) ;
#3176=CARTESIAN_POINT ( 'NONE',  ( -35.00000000000000000, 0.000000000000000000, 0.000000000000000000 ) ) ;
#3177=ADVANCED_FACE ( 'NONE', ( #25563 ), #61793, .T. ) ;
#3179=DIRECTION ( 'NONE',  ( 0.000000000000000000, 0.3554799084908970563, 0.9346839223284539866 ) ) ;
#3180=CARTESIAN_POINT ( 'NONE',  ( -35.00000000000000000, 7.717887834988368390, -8.854740511458771834 ) ) ;
#3181=DIRECTION ( 'NONE',  ( -1.000000000000000000, 0.000000000000000000, 0.000000000000000000 ) ) ;
#3186=DIRECTION ( 'NONE',  ( -1.000000000000000000, 0.000000000000000000, -0.000000000000000000 ) ) ;
#3190=ORIENTED_EDGE ( 'NONE', *, *, #42347, .F. ) ;
#3191=ORIENTED_EDGE ( 'NONE', *, *, #8600, .T. ) ;
#3192=CARTESIAN_POINT ( 'NONE',  ( -2.532614230583023041, -12.88560382747352584, 4.026315189028235153 ) ) ;
#3195=CARTESIAN_POINT ( 'NONE',  ( -25.54417658651491863, 7.498517398407837931, 11.22596262356930197 ) ) ;
#3196=CIRCLE ( 'NONE', #34021, 5.000000000000000000 ) ;
#3198=CARTESIAN_POINT ( 'NONE',  ( 22.57855258442565116, 3.026812727784649493, -11.61199400236326973 ) ) ;
#3200=LINE ( 'NONE', #63040, #44751 ) ;
#3202=DIRECTION ( 'NONE',  ( -1.000000000000000000, 0.000000000000000000, 0.000000000000000000 ) ) ;
#3204=CYLINDRICAL_SURFACE ( 'NONE', #24218, 12.18650000000000055 ) ;
#3205=ORIENTED_EDGE ( 'NONE', *, *, #39463, .F. ) ;
#3210=CARTESIAN_POINT ( 'NONE',  ( 10.75853767213705225, 7.830989516993144051, 25.00000000000000000 ) ) ;
#3211=CARTESIAN_POINT ( 'NONE',  ( 29.03457606387295087, 7.862146963512124387, 10.97436308512422265 ) ) ;
#3212=ADVANCED_FACE ( 'NONE', ( #26228 ), #55837, .T. ) ;
#3213=CARTESIAN_POINT ( 'NONE',  ( -47.00000000000000711, 0.000000000000000000, 0.000000000000000000 ) ) ;
#3215=LINE ( 'NONE', #28793, #9992 ) ;
#3217=ORIENTED_EDGE ( 'NONE', *, *, #46388, .T. ) ;
#3219=ORIENTED_EDGE ( 'NONE', *, *, #48908, .T. ) ;
#3220=CARTESIAN_POINT ( 'NONE',  ( -37.00000000000000711, -10.32377448871672598, 6.475373545682264975 ) ) ;
#3221=CARTESIAN_POINT ( 'NONE',  ( -37.00000000000000711, -6.018036132182241538, 11.24036214326518390 ) ) ;
#3222=AXIS2_PLACEMENT_3D ( 'NONE', #31865, #52185, #57498 ) ;
#3224=DIRECTION ( 'NONE',  ( 1.000000000000000000, 0.000000000000000000, 0.000000000000000000 ) ) ;
#3225=CARTESIAN_POINT ( 'NONE',  ( -28.14458306582303848, 12.90557762884671433, -3.973285507432364305 ) ) ;
#3226=EDGE_CURVE ( 'NONE', #61808, #25415, #11841, .T. ) ;
#3228=CYLINDRICAL_SURFACE ( 'NONE', #51129, 12.75000000000000178 ) ;
#3229=CARTESIAN_POINT ( 'NONE',  ( 10.16774168188999816, 8.043487525566618501, 8.909738100526366722 ) ) ;
#3233=ORIENTED_EDGE ( 'NONE', *, *, #37897, .F. ) ;
#3234=DIRECTION ( 'NONE',  ( -1.000000000000000000, 0.000000000000000000, 0.000000000000000000 ) ) ;
#3235=DIRECTION ( 'NONE',  ( 0.000000000000000000, -0.01356324068817998940, 0.9999080150203990547 ) ) ;
#3236=DIRECTION ( 'NONE',  ( 1.000000000000000000, 0.000000000000000000, 0.000000000000000000 ) ) ;
#3237=DIRECTION ( 'NONE',  ( -1.000000000000000000, 0.000000000000000000, 0.000000000000000000 ) ) ;
#3238=VECTOR ( 'NONE', #61130, 1000.000000000000000 ) ;
#3239=AXIS2_PLACEMENT_3D ( 'NONE', #19149, #34442, #54744 ) ;
#3240=AXIS2_PLACEMENT_3D ( 'NONE', #42259, #17358, #63872 ) ;
#3241=EDGE_CURVE ( 'NONE', #32833, #3673, #51525, .T. ) ;
#3242=AXIS2_PLACEMENT_3D ( 'NONE', #44208, #18947, #30229 ) ;
#3244=CARTESIAN_POINT ( 'NONE',  ( -28.23740090307966355, -10.53170506870664624, -5.760529898918337111 ) ) ;
#3245=ORIENTED_EDGE ( 'NONE', *, *, #47251, .F. ) ;
#3254=DIRECTION ( 'NONE',  ( 0.000000000000000000, 0.01356324068817998940, -0.9999080150203990547 ) ) ;
#3258=ORIENTED_EDGE ( 'NONE', *, *, #51060, .T. ) ;
#3259=AXIS2_PLACEMENT_3D ( 'NONE', #105, #16702, #45996 ) ;
#3265=DIRECTION ( 'NONE',  ( 0.000000000000000000, 0.9847383929261610547, -0.1740410799127650732 ) ) ;
#3266=DIRECTION ( 'NONE',  ( 0.000000000000000000, 0.01356324068817992175, -0.9999080150203990547 ) ) ;
#3268=EDGE_LOOP ( 'NONE', ( #2961, #42320, #27202, #45516 ) ) ;
#3269=EDGE_LOOP ( 'NONE', ( #12065, #2099, #53228, #46921 ) ) ;
#3270=CARTESIAN_POINT ( 'NONE',  ( -19.69476066079020171, -4.201994156881551312, -11.24025111398909615 ) ) ;
#3271=VECTOR ( 'NONE', #52281, 1000.000000000000000 ) ;
#3275=CARTESIAN_POINT ( 'NONE',  ( -20.79170840334646542, -12.91784323155722269, -3.921648409140116698 ) ) ;
#3276=ORIENTED_EDGE ( 'NONE', *, *, #14531, .F. ) ;
#3277=CIRCLE ( 'NONE', #21291, 12.75000000000000178 ) ;
#3284=VERTEX_POINT ( 'NONE', #5972 ) ;
#3287=ORIENTED_EDGE ( 'NONE', *, *, #52505, .T. ) ;
#3288=FACE_OUTER_BOUND ( 'NONE', #38240, .T. ) ;
#3293=CARTESIAN_POINT ( 'NONE',  ( 37.00000000000000711, -1.030638227056475120, 12.14284015767850811 ) ) ;
#3295=VECTOR ( 'NONE', #47182, 1000.000000000000000 ) ;
#3296=CARTESIAN_POINT ( 'NONE',  ( -35.00000000000000000, 0.000000000000000000, 0.000000000000000000 ) ) ;
#3297=VERTEX_POINT ( 'NONE', #1629 ) ;
#3304=CARTESIAN_POINT ( 'NONE',  ( 22.86336934118476805, 2.804796819963978560, 13.20738486019996927 ) ) ;
#3305=CARTESIAN_POINT ( 'NONE',  ( 35.00000000000000000, 4.705694406421931860E-17, -3.469127814946512892E-15 ) ) ;
#3306=CARTESIAN_POINT ( 'NONE',  ( -28.85619398320021745, 3.750539801530000439, -12.96855624952673836 ) ) ;
#3307=CARTESIAN_POINT ( 'NONE',  ( 35.00000000000000000, 10.01317267707886671, -6.946017217729977489 ) ) ;
#3308=AXIS2_PLACEMENT_3D ( 'NONE', #41002, #30040, #61283 ) ;
#3310=VERTEX_POINT ( 'NONE', #21902 ) ;
#3311=CARTESIAN_POINT ( 'NONE',  ( -18.58686583997219799, 5.411564556385481062, -10.71438573093091051 ) ) ;
#3312=AXIS2_PLACEMENT_3D ( 'NONE', #60212, #20949, #61511 ) ;
#3313=AXIS2_PLACEMENT_3D ( 'NONE', #65255, #60586, #10055 ) ;
#3315=VERTEX_POINT ( 'NONE', #26544 ) ;
#3316=EDGE_CURVE ( 'NONE', #41887, #25967, #30106, .T. ) ;
#3317=DIRECTION ( 'NONE',  ( 1.000000000000000000, 0.000000000000000000, 0.000000000000000000 ) ) ;
#3319=CARTESIAN_POINT ( 'NONE',  ( 12.85737776239257357, -12.70266831868442736, -4.575077721476746184 ) ) ;
#3322=EDGE_CURVE ( 'NONE', #62589, #14872, #24572, .T. ) ;
#3324=ORIENTED_EDGE ( 'NONE', *, *, #32858, .T. ) ;
#3325=LINE ( 'NONE', #23930, #30325 ) ;
#3328=DIRECTION ( 'NONE',  ( 0.000000000000000000, -0.01356324068817998940, 0.9999080150203990547 ) ) ;
#3332=CIRCLE ( 'NONE', #12839, 12.18649999999999878 ) ;
#3334=ORIENTED_EDGE ( 'NONE', *, *, #17797, .T. ) ;
#3335=EDGE_CURVE ( 'NONE', #48435, #15604, #60700, .T. ) ;
#3337=AXIS2_PLACEMENT_3D ( 'NONE', #10418, #25395, #9425 ) ;
#3339=CARTESIAN_POINT ( 'NONE',  ( -35.00000000000000000, 12.46157735505192932, -2.696588552978924636 ) ) ;
#3340=CIRCLE ( 'NONE', #40469, 12.75000000000000178 ) ;
#3341=CIRCLE ( 'NONE', #16074, 12.18649999999999878 ) ;
#3342=VERTEX_POINT ( 'NONE', #62435 ) ;
#3343=ORIENTED_EDGE ( 'NONE', *, *, #39453, .F. ) ;
#3345=ADVANCED_FACE ( 'NONE', ( #31848 ), #16897, .T. ) ;
#3346=EDGE_LOOP ( 'NONE', ( #32467, #58061, #4704, #33924 ) ) ;
#3347=LINE ( 'NONE', #43886, #62674 ) ;
#3349=DIRECTION ( 'NONE',  ( 0.000000000000000000, -0.9105187689795998240, 0.4134677391718418193 ) ) ;
#3353=ORIENTED_EDGE ( 'NONE', *, *, #44055, .F. ) ;
#3354=ORIENTED_EDGE ( 'NONE', *, *, #10018, .T. ) ;
#3355=ORIENTED_EDGE ( 'NONE', *, *, #16756, .T. ) ;
#3360=ORIENTED_EDGE ( 'NONE', *, *, #23685, .F. ) ;
#3362=CIRCLE ( 'NONE', #6579, 12.18650000000000055 ) ;
#3365=DIRECTION ( 'NONE',  ( 1.000000000000000000, -0.000000000000000000, -0.000000000000000000 ) ) ;
#3367=CARTESIAN_POINT ( 'NONE',  ( -14.11589373245165469, 8.250315036047107142, 25.00000000000000000 ) ) ;
#3369=CIRCLE ( 'NONE', #24608, 12.18650000000000055 ) ;
#3370=ORIENTED_EDGE ( 'NONE', *, *, #14006, .F. ) ;
#3371=DIRECTION ( 'NONE',  ( -1.000000000000000000, 0.000000000000000000, 0.000000000000000000 ) ) ;
#3372=ORIENTED_EDGE ( 'NONE', *, *, #60318, .T. ) ;
#3373=CYLINDRICAL_SURFACE ( 'NONE', #3079, 4.999999999999999112 ) ;
#3374=VERTEX_POINT ( 'NONE', #11903 ) ;
#3375=CIRCLE ( 'NONE', #53244, 5.000000000000000888 ) ;
#3376=ORIENTED_EDGE ( 'NONE', *, *, #57570, .F. ) ;
#3378=FACE_OUTER_BOUND ( 'NONE', #10579, .T. ) ;
#3379=CARTESIAN_POINT ( 'NONE',  ( 37.00000000000000711, 4.983891302653743693, 11.73555825188270596 ) ) ;
#3380=ADVANCED_FACE ( 'NONE', ( #41842 ), #47184, .T. ) ;
#3385=DIRECTION ( 'NONE',  ( 1.000000000000000000, 0.000000000000000000, -0.000000000000000000 ) ) ;
#3389=DIRECTION ( 'NONE',  ( 0.000000000000000000, 0.2618041379715563277, -0.9651210252299812220 ) ) ;
#3390=VERTEX_POINT ( 'NONE', #22207 ) ;
#3392=DIRECTION ( 'NONE',  ( -1.000000000000000000, 0.000000000000000000, 0.000000000000000000 ) ) ;
#3396=AXIS2_PLACEMENT_3D ( 'NONE', #63332, #17799, #38060 ) ;
#3398=CIRCLE ( 'NONE', #63877, 12.18649999999999878 ) ;
#3399=EDGE_CURVE ( 'NONE', #20070, #49500, #8684, .T. ) ;
#3400=VERTEX_POINT ( 'NONE', #22556 ) ;
#3401=DIRECTION ( 'NONE',  ( 0.000000000000000000, -0.2355298848897378061, -0.9718671068226493182 ) ) ;
#3402=VERTEX_POINT ( 'NONE', #37510 ) ;
#3403=CARTESIAN_POINT ( 'NONE',  ( 35.00000000000000000, -12.08216339958901564, -1.591260454995201412 ) ) ;
#3404=DIRECTION ( 'NONE',  ( 1.000000000000000000, 0.000000000000000000, 0.000000000000000000 ) ) ;
#3405=DIRECTION ( 'NONE',  ( 1.000000000000000000, -0.000000000000000000, 0.000000000000000000 ) ) ;
#3406=PLANE ( 'NONE',  #52142 ) ;
#3407=ADVANCED_FACE ( 'NONE', ( #16585 ), #57815, .T. ) ;
#3409=VERTEX_POINT ( 'NONE', #42818 ) ;
#3410=CARTESIAN_POINT ( 'NONE',  ( -14.11589373245165469, 8.250315036047107142, 25.00000000000000000 ) ) ;
#3411=CIRCLE ( 'NONE', #41632, 5.000000000000000888 ) ;
#3412=CIRCLE ( 'NONE', #38400, 5.000000000000000888 ) ;
#3413=CIRCLE ( 'NONE', #59681, 5.000000000000000888 ) ;
#3415=ADVANCED_FACE ( 'NONE', ( #37839 ), #36532, .T. ) ;
#3416=AXIS2_PLACEMENT_3D ( 'NONE', #39568, #10606, #14294 ) ;
#3421=CARTESIAN_POINT ( 'NONE',  ( 5.650264051100599261, -9.979872282089162994, -6.674586346603469167 ) ) ;
#3422=DIRECTION ( 'NONE',  ( -1.000000000000000000, -0.000000000000000000, -0.000000000000000000 ) ) ;
#3423=AXIS2_PLACEMENT_3D ( 'NONE', #18091, #16769, #58011 ) ;
#3424=EDGE_CURVE ( 'NONE', #82, #12941, #13849, .T. ) ;
#3427=CARTESIAN_POINT ( 'NONE',  ( 12.18694916440639631, -11.65410571009191365, -2.865109251948741775 ) ) ;
#3429=CIRCLE ( 'NONE', #46930, 12.74999999999999822 ) ;
#3430=EDGE_LOOP ( 'NONE', ( #56406, #32269, #624, #3471 ) ) ;
#3431=DIRECTION ( 'NONE',  ( 0.000000000000000000, 0.01356324068817998940, -0.9999080150203989437 ) ) ;
#3436=ORIENTED_EDGE ( 'NONE', *, *, #53366, .F. ) ;
#3438=ORIENTED_EDGE ( 'NONE', *, *, #40843, .F. ) ;
#3441=AXIS2_PLACEMENT_3D ( 'NONE', #3176, #63999, #54702 ) ;
#3442=DIRECTION ( 'NONE',  ( 0.000000000000000000, -0.01356324068817998940, 0.9999080150203990547 ) ) ;
#3443=CIRCLE ( 'NONE', #37385, 5.000000000000000000 ) ;
#3445=ORIENTED_EDGE ( 'NONE', *, *, #61614, .T. ) ;
#3446=DIRECTION ( 'NONE',  ( 1.000000000000000000, 0.000000000000000000, 0.000000000000000000 ) ) ;
#3451=DIRECTION ( 'NONE',  ( -1.000000000000000000, 0.000000000000000000, 0.000000000000000000 ) ) ;
#3452=CYLINDRICAL_SURFACE ( 'NONE', #50059, 12.18649999999999878 ) ;
#3453=DIRECTION ( 'NONE',  ( 0.000000000000000000, 0.000000000000000000, -1.000000000000000000 ) ) ;
#3456=DIRECTION ( 'NONE',  ( 0.000000000000000000, 0.000000000000000000, -1.000000000000000000 ) ) ;
#3459=DIRECTION ( 'NONE',  ( 0.000000000000000000, -0.9987865678893282917, 0.04924826701373502535 ) ) ;
#3460=ORIENTED_EDGE ( 'NONE', *, *, #14689, .F. ) ;
#3461=CYLINDRICAL_SURFACE ( 'NONE', #29492, 12.18650000000000055 ) ;
#3462=VECTOR ( 'NONE', #61075, 1000.000000000000000 ) ;
#3464=DIRECTION ( 'NONE',  ( 0.000000000000000000, -0.01356324068817991828, 0.9999080150203990547 ) ) ;
#3469=DIRECTION ( 'NONE',  ( 0.000000000000000000, 0.4935949184179262983, -0.8696919319575183716 ) ) ;
#3470=CARTESIAN_POINT ( 'NONE',  ( 9.687175622948609899, 13.48729812737144940, -0.5854820436212360146 ) ) ;
#3471=ORIENTED_EDGE ( 'NONE', *, *, #11070, .T. ) ;
#3472=CARTESIAN_POINT ( 'NONE',  ( -35.00000000000000000, 0.000000000000000000, 0.000000000000000000 ) ) ;
#3477=CARTESIAN_POINT ( 'NONE',  ( -37.00000000000000711, 11.24036214326520700, 6.018036132182202458 ) ) ;
#3478=CARTESIAN_POINT ( 'NONE',  ( 35.00000000000000000, 4.705694406421931860E-17, -3.469127814946512892E-15 ) ) ;
#3479=CARTESIAN_POINT ( 'NONE',  ( -37.00000000000000711, 11.96656215839369253, 4.400442035670988794 ) ) ;
#3481=FACE_OUTER_BOUND ( 'NONE', #62582, .T. ) ;
#3482=LINE ( 'NONE', #44999, #17210 ) ;
#3483=CARTESIAN_POINT ( 'NONE',  ( -34.00000000000000000, -11.99999999999999822, 0.000000000000000000 ) ) ;
#3486=PLANE ( 'NONE',  #58248 ) ;
#3488=CARTESIAN_POINT ( 'NONE',  ( -17.83419946441818027, -9.720786832536937538, 9.367833439828872955 ) ) ;
#3491=AXIS2_PLACEMENT_3D ( 'NONE', #38739, #49700, #4145 ) ;
#3492=DIRECTION ( 'NONE',  ( 0.000000000000000000, 0.1387779952735747335, -0.9903235168508560671 ) ) ;
#3493=AXIS2_PLACEMENT_3D ( 'NONE', #781, #35999, #10748 ) ;
#3494=CARTESIAN_POINT ( 'NONE',  ( -8.333162451619710254, -1.931509586269193113, 13.36158470235419493 ) ) ;
#3495=CARTESIAN_POINT ( 'NONE',  ( -10.39029797936073862, -5.035631434083518876, 12.53173546626830692 ) ) ;
#3497=DIRECTION ( 'NONE',  ( 0.000000000000000000, 0.01356324068817998940, -0.9999080150203990547 ) ) ;
#3499=DIRECTION ( 'NONE',  ( 1.000000000000000000, -0.000000000000000000, 0.000000000000000000 ) ) ;
#3502=AXIS2_PLACEMENT_3D ( 'NONE', #4655, #16584, #37168 ) ;
#3503=EDGE_CURVE ( 'NONE', #48169, #32449, #28197, .T. ) ;
#3505=DIRECTION ( 'NONE',  ( 1.000000000000000000, 0.000000000000000000, 0.000000000000000000 ) ) ;
#3506=VERTEX_POINT ( 'NONE', #43462 ) ;
#3510=CARTESIAN_POINT ( 'NONE',  ( -18.58686583997219799, 4.913588802969568903, -10.95106697391550021 ) ) ;
#3511=ORIENTED_EDGE ( 'NONE', *, *, #35759, .T. ) ;
#3512=EDGE_CURVE ( 'NONE', #29524, #25246, #13872, .T. ) ;
#3513=CARTESIAN_POINT ( 'NONE',  ( 22.80793912684299229, 11.57402466465492097, -6.956843576774104143 ) ) ;
#3515=ORIENTED_EDGE ( 'NONE', *, *, #40168, .F. ) ;
#3516=ORIENTED_EDGE ( 'NONE', *, *, #14940, .T. ) ;
#3518=VERTEX_POINT ( 'NONE', #63742 ) ;
#3520=CARTESIAN_POINT ( 'NONE',  ( -35.00000000000000000, 11.65150730582932503, 1.488153103997165605 ) ) ;
#3522=DIRECTION ( 'NONE',  ( 1.000000000000000000, 0.000000000000000000, 0.000000000000000000 ) ) ;
#3523=( BOUNDED_CURVE ( )  B_SPLINE_CURVE ( 3, ( #52338, #6779, #52663, #7088 ),
 .UNSPECIFIED., .F., .F. ) 
 B_SPLINE_CURVE_WITH_KNOTS ( ( 4, 4 ),
 ( 4.347126718975509618, 4.378220820213373443 ),
 .UNSPECIFIED. ) 
 CURVE ( )  GEOMETRIC_REPRESENTATION_ITEM ( )  RATIONAL_B_SPLINE_CURVE ( ( 1.000000000000000000, 0.9999194313618959828, 0.9999194313618959828, 1.000000000000000000 ) ) 
 REPRESENTATION_ITEM ( '' )  );
#3526=FACE_OUTER_BOUND ( 'NONE', #40539, .T. ) ;
#3527=ORIENTED_EDGE ( 'NONE', *, *, #24110, .F. ) ;
#3528=DIRECTION ( 'NONE',  ( 1.000000000000000000, 0.000000000000000000, 0.000000000000000000 ) ) ;
#3530=AXIS2_PLACEMENT_3D ( 'NONE', #42470, #2937, #27206 ) ;
#3531=CARTESIAN_POINT ( 'NONE',  ( 35.00000000000000000, -1.771820996347075017, 11.61175578952787113 ) ) ;
#3534=ORIENTED_EDGE ( 'NONE', *, *, #37135, .F. ) ;
#3535=CARTESIAN_POINT ( 'NONE',  ( -17.47216009470839282, 7.641999522472164408, 11.13043964233116334 ) ) ;
#3537=AXIS2_PLACEMENT_3D ( 'NONE', #37145, #1914, #62408 ) ;
#3538=CARTESIAN_POINT ( 'NONE',  ( -37.00000000000000711, 6.584150480049697940, -10.25474254703946109 ) ) ;
#3541=CARTESIAN_POINT ( 'NONE',  ( -37.00000000000000711, 8.366449238204365813, 9.621072037177027525 ) ) ;
#3543=ORIENTED_EDGE ( 'NONE', *, *, #61845, .F. ) ;
#3545=LINE ( 'NONE', #18815, #65467 ) ;
#3546=EDGE_LOOP ( 'NONE', ( #7831, #26719, #1155, #24190 ) ) ;
#3547=CARTESIAN_POINT ( 'NONE',  ( 35.00000000000000000, 4.705694406421931860E-17, -3.469127814946512892E-15 ) ) ;
#3548=VECTOR ( 'NONE', #27012, 1000.000000000000000 ) ;
#3550=ORIENTED_EDGE ( 'NONE', *, *, #58564, .T. ) ;
#3552=EDGE_CURVE ( 'NONE', #36795, #34842, #51024, .T. ) ;
#3553=DIRECTION ( 'NONE',  ( 0.000000000000000000, -0.9718671068226434340, 0.2355298848897617037 ) ) ;
#3556=CARTESIAN_POINT ( 'NONE',  ( 29.51976981715666781, 7.690765383426390045, 11.09513982864076276 ) ) ;
#3557=AXIS2_PLACEMENT_3D ( 'NONE', #51444, #57389, #11816 ) ;
#3558=CYLINDRICAL_SURFACE ( 'NONE', #45832, 5.000000000000000888 ) ;
#3560=ORIENTED_EDGE ( 'NONE', *, *, #15162, .T. ) ;
#3561=EDGE_LOOP ( 'NONE', ( #1606, #2702, #10604, #22563 ) ) ;
#3562=VECTOR ( 'NONE', #15614, 1000.000000000000000 ) ;
#3563=EDGE_CURVE ( 'NONE', #39575, #47639, #22456, .T. ) ;
#3564=DIRECTION ( 'NONE',  ( 1.000000000000000000, 0.000000000000000000, 0.000000000000000000 ) ) ;
#3565=EDGE_CURVE ( 'NONE', #52756, #35052, #34053, .T. ) ;
#3566=DIRECTION ( 'NONE',  ( -1.000000000000000000, 0.000000000000000000, 0.000000000000000000 ) ) ;
#3567=DIRECTION ( 'NONE',  ( 1.000000000000000000, 0.000000000000000000, -0.000000000000000000 ) ) ;
#3570=CIRCLE ( 'NONE', #48129, 5.000000000000000888 ) ;
#3571=CARTESIAN_POINT ( 'NONE',  ( -27.69104391824479805, 10.87192706255359909, -8.023814012560558595 ) ) ;
#3572=CARTESIAN_POINT ( 'NONE',  ( -47.00000000000000711, 0.000000000000000000, 0.000000000000000000 ) ) ;
#3574=B_SPLINE_CURVE_WITH_KNOTS ( 'NONE', 3,
 ( #63001, #56378, #10825, #42055, #36426, #62338, #31110, #37066, #5873, #46406, #11794, #851, #17128, #52392, #6839, #47405, #1842, #38386, #23774, #44039, #17464, #54360, #43362, #13755 ),
 .UNSPECIFIED., .F., .F.,
 ( 4, 2, 2, 2, 2, 2, 2, 2, 2, 2, 2, 4 ),
 ( 0.000000000000000000, 0.0005610479560808320819, 0.001122095912161664164, 0.001683143868242496137, 0.002244191824323328328, 0.003366287736484988805, 0.003927335692565820345, 0.004488383648646649716, 0.005610479560808312796, 0.006732575472969976743, 0.007854671385131640690, 0.008976767297293304637 ),
 .UNSPECIFIED. ) ;
#3578=ORIENTED_EDGE ( 'NONE', *, *, #18077, .F. ) ;
#3579=AXIS2_PLACEMENT_3D ( 'NONE', #43688, #13112, #47703 ) ;
#3580=CARTESIAN_POINT ( 'NONE',  ( -20.79170840334646542, 11.34110549087207076, -3.921648409140116698 ) ) ;
#3582=CIRCLE ( 'NONE', #36490, 12.18649999999999700 ) ;
#3583=DIRECTION ( 'NONE',  ( 0.000000000000000000, 0.01356324068817998940, -0.9999080150203990547 ) ) ;
#3584=EDGE_CURVE ( 'NONE', #1539, #36570, #21294, .T. ) ;
#3585=CIRCLE ( 'NONE', #36442, 12.74999999999999822 ) ;
#3586=AXIS2_PLACEMENT_3D ( 'NONE', #43141, #7928, #3265 ) ;
#3587=EDGE_CURVE ( 'NONE', #12178, #60093, #52113, .T. ) ;
#3590=EDGE_LOOP ( 'NONE', ( #62897, #38164, #17334, #15130 ) ) ;
#3592=CARTESIAN_POINT ( 'NONE',  ( 29.69944545120181090, 10.33295084604707448, 8.690866588745604915 ) ) ;
#3595=ORIENTED_EDGE ( 'NONE', *, *, #2287, .T. ) ;
#3596=CARTESIAN_POINT ( 'NONE',  ( -11.13234721864718679, -5.599044822695524282, -12.29123017578099208 ) ) ;
#3597=FACE_OUTER_BOUND ( 'NONE', #50287, .T. ) ;
#3598=CARTESIAN_POINT ( 'NONE',  ( 17.30586438374871250, -10.58231581927869058, 8.416062268768557786 ) ) ;
#3599=VECTOR ( 'NONE', #53857, 1000.000000000000000 ) ;
#3601=CARTESIAN_POINT ( 'NONE',  ( -9.368646887739329188, -10.53974709387553865, -8.470498924738002700 ) ) ;
#3602=AXIS2_PLACEMENT_3D ( 'NONE', #33086, #57732, #52735 ) ;
#3603=B_SPLINE_CURVE_WITH_KNOTS ( 'NONE', 3,
 ( #13066, #53313, #33350, #28354, #53960, #57978, #18057, #2101, #2450, #38321, #48340, #23369, #43638, #63928, #12388, #47655, #47996, #18729 ),
 .UNSPECIFIED., .F., .F.,
 ( 4, 2, 2, 2, 2, 2, 2, 2, 4 ),
 ( 0.000000000000000000, 0.002646377093913540243, 0.003307971367391926605, 0.003969565640870312967, 0.005292754187827087425, 0.006615942734783859282, 0.007939131281740631138, 0.009262319828697403862, 0.01058550837565417659 ),
 .UNSPECIFIED. ) ;
#3604=DIRECTION ( 'NONE',  ( -1.000000000000000000, 0.000000000000000000, 0.000000000000000000 ) ) ;
#3607=DIRECTION ( 'NONE',  ( 0.000000000000000000, -0.01356324068817992522, 0.9999080150203990547 ) ) ;
#3610=CARTESIAN_POINT ( 'NONE',  ( 35.00000000000000000, -1.463443770872862482, -12.09831040184923978 ) ) ;
#3612=VECTOR ( 'NONE', #350, 1000.000000000000000 ) ;
#3613=DIRECTION ( 'NONE',  ( -1.000000000000000000, 0.000000000000000000, 0.000000000000000000 ) ) ;
#3614=CARTESIAN_POINT ( 'NONE',  ( -27.16408673750832747, -8.649729821182791767, -8.318274995791206550 ) ) ;
#3616=ORIENTED_EDGE ( 'NONE', *, *, #38696, .F. ) ;
#3617=CARTESIAN_POINT ( 'NONE',  ( -19.42173080018139331, -4.342950793773034057, -11.18689537328631012 ) ) ;
#3619=CYLINDRICAL_SURFACE ( 'NONE', #39737, 12.74999999999999822 ) ;
#3620=CARTESIAN_POINT ( 'NONE',  ( 35.00000000000000000, -10.30098186818245409, 5.644643009979177783 ) ) ;
#3621=AXIS2_PLACEMENT_3D ( 'NONE', #13550, #48502, #2954 ) ;
#3625=EDGE_CURVE ( 'NONE', #29278, #19802, #1135, .T. ) ;
#3627=CARTESIAN_POINT ( 'NONE',  ( 24.84806924723610067, -1.530817552018350014, 13.41866073552183103 ) ) ;
#3628=ORIENTED_EDGE ( 'NONE', *, *, #25198, .F. ) ;
#3629=ORIENTED_EDGE ( 'NONE', *, *, #55805, .T. ) ;
#3630=DIRECTION ( 'NONE',  ( -1.000000000000000000, 0.000000000000000000, 0.000000000000000000 ) ) ;
#3631=AXIS2_PLACEMENT_3D ( 'NONE', #25626, #40927, #3492 ) ;
#3632=CARTESIAN_POINT ( 'NONE',  ( 37.00000000000000711, 12.38385022362086119, 3.033604067594442899 ) ) ;
#3633=CIRCLE ( 'NONE', #18480, 4.999999999999998224 ) ;
#3634=EDGE_LOOP ( 'NONE', ( #21382, #38910, #34269, #39006 ) ) ;
#3635=VERTEX_POINT ( 'NONE', #46118 ) ;
#3636=CARTESIAN_POINT ( 'NONE',  ( -35.00000000000000000, 0.000000000000000000, 0.000000000000000000 ) ) ;
#3637=DIRECTION ( 'NONE',  ( 0.000000000000000000, -0.6745969609292555846, -0.7381862504172050921 ) ) ;
#3638=AXIS2_PLACEMENT_3D ( 'NONE', #48796, #38133, #58443 ) ;
#3639=CARTESIAN_POINT ( 'NONE',  ( 35.00000000000000000, 4.705694406421931860E-17, -3.469127814946512892E-15 ) ) ;
#3641=EDGE_CURVE ( 'NONE', #46339, #56916, #40441, .T. ) ;
#3643=LINE ( 'NONE', #23908, #59888 ) ;
#3644=ORIENTED_EDGE ( 'NONE', *, *, #18240, .T. ) ;
#3645=CARTESIAN_POINT ( 'NONE',  ( 37.00000000000000711, -10.80631716521670427, -4.603882218679513194 ) ) ;
#3646=VECTOR ( 'NONE', #54082, 1000.000000000000000 ) ;
#3647=CARTESIAN_POINT ( 'NONE',  ( -15.47692202957099461, 7.964177873487604309, 8.976325883789177951 ) ) ;
#3654=CARTESIAN_POINT ( 'NONE',  ( 22.36482863261543486, -11.96441317219524514, -0.9234811557364158707 ) ) ;
#3656=AXIS2_PLACEMENT_3D ( 'NONE', #63929, #33351, #58644 ) ;
#3657=ORIENTED_EDGE ( 'NONE', *, *, #19108, .F. ) ;
#3658=CARTESIAN_POINT ( 'NONE',  ( -16.86326112465461335, 8.068804307413738997, -8.883526352222181899 ) ) ;
#3659=ORIENTED_EDGE ( 'NONE', *, *, #17187, .T. ) ;
#3660=CYLINDRICAL_SURFACE ( 'NONE', #9377, 5.000000000000000888 ) ;
#3661=CARTESIAN_POINT ( 'NONE',  ( 35.00000000000000000, -8.052525312709825300, 8.551552972817161091 ) ) ;
#3663=LINE ( 'NONE', #38204, #33489 ) ;
#3664=CARTESIAN_POINT ( 'NONE',  ( -25.64778288570172649, -7.682669607182212701, 11.10295593026794592 ) ) ;
#3666=ORIENTED_EDGE ( 'NONE', *, *, #6794, .F. ) ;
#3669=CARTESIAN_POINT ( 'NONE',  ( -37.00000000000000711, 0.000000000000000000, 0.000000000000000000 ) ) ;
#3670=ADVANCED_FACE ( 'NONE', ( #5558 ), #45121, .T. ) ;
#3673=VERTEX_POINT ( 'NONE', #19533 ) ;
#3677=CARTESIAN_POINT ( 'NONE',  ( 35.00000000000000000, -10.25474254703957477, -6.584150480049516752 ) ) ;
#3678=AXIS2_PLACEMENT_3D ( 'NONE', #13140, #29722, #24759 ) ;
#3680=CARTESIAN_POINT ( 'NONE',  ( 35.00000000000000000, 4.705694406421931860E-17, -3.469127814946512892E-15 ) ) ;
#3682=ADVANCED_FACE ( 'NONE', ( #40791 ), #19847, .T. ) ;
#3683=ORIENTED_EDGE ( 'NONE', *, *, #32481, .F. ) ;
#3687=CARTESIAN_POINT ( 'NONE',  ( 35.00000000000000000, 10.42955799785319648, -6.303578524886984447 ) ) ;
#3688=VECTOR ( 'NONE', #23494, 1000.000000000000000 ) ;
#3692=ORIENTED_EDGE ( 'NONE', *, *, #5414, .F. ) ;
#3693=ORIENTED_EDGE ( 'NONE', *, *, #63432, .T. ) ;
#3696=CIRCLE ( 'NONE', #40832, 12.75000000000000178 ) ;
#3697=CARTESIAN_POINT ( 'NONE',  ( 35.00000000000000000, -11.73555825188272728, 4.983891302653700173 ) ) ;
#3698=EDGE_CURVE ( 'NONE', #50756, #18994, #31917, .T. ) ;
#3699=ORIENTED_EDGE ( 'NONE', *, *, #37989, .T. ) ;
#3701=CARTESIAN_POINT ( 'NONE',  ( 35.00000000000000000, 4.705694406421931860E-17, -3.469127814946512892E-15 ) ) ;
#3704=ADVANCED_FACE ( 'NONE', ( #10505 ), #31766, .T. ) ;
#3705=AXIS2_PLACEMENT_3D ( 'NONE', #45704, #51383, #2471 ) ;
#3706=CARTESIAN_POINT ( 'NONE',  ( 37.00000000000000711, 3.473736367725426266, 12.26766708251987836 ) ) ;
#3713=DIRECTION ( 'NONE',  ( 1.000000000000000000, 0.000000000000000000, 0.000000000000000000 ) ) ;
#3714=ORIENTED_EDGE ( 'NONE', *, *, #50463, .T. ) ;
#3715=ORIENTED_EDGE ( 'NONE', *, *, #33858, .T. ) ;
#3716=EDGE_LOOP ( 'NONE', ( #26940, #57656, #59420, #63941 ) ) ;
#3717=CARTESIAN_POINT ( 'NONE',  ( 35.00000000000000000, -0.01609748574436820068, 11.74614673114903596 ) ) ;
#3719=AXIS2_PLACEMENT_3D ( 'NONE', #13896, #20206, #44177 ) ;
#3724=ORIENTED_EDGE ( 'NONE', *, *, #20601, .F. ) ;
#3727=ORIENTED_EDGE ( 'NONE', *, *, #57185, .T. ) ;
#3728=FACE_OUTER_BOUND ( 'NONE', #24247, .T. ) ;
#3729=EDGE_CURVE ( 'NONE', #58346, #32993, #57067, .T. ) ;
#3732=EDGE_LOOP ( 'NONE', ( #4401, #20527, #60849, #45202 ) ) ;
#3733=CARTESIAN_POINT ( 'NONE',  ( 24.82652845881425208, 10.42385221765396608, -8.578654028722157321 ) ) ;
#3734=CARTESIAN_POINT ( 'NONE',  ( 27.76606509001456047, 10.82004123774806104, 5.203714701047107205 ) ) ;
#3736=ORIENTED_EDGE ( 'NONE', *, *, #30183, .T. ) ;
#3741=ORIENTED_EDGE ( 'NONE', *, *, #65425, .F. ) ;
#3742=CARTESIAN_POINT ( 'NONE',  ( 35.00000000000000000, 7.817610399097634222, 8.766823244861901898 ) ) ;
#3743=FACE_OUTER_BOUND ( 'NONE', #27761, .T. ) ;
#3746=CARTESIAN_POINT ( 'NONE',  ( 12.10998784662220729, 8.443435280036798218, -8.526922110106905706 ) ) ;
#3748=CARTESIAN_POINT ( 'NONE',  ( -37.00000000000000711, 11.73555825188283741, -4.983891302653459476 ) ) ;
#3751=CARTESIAN_POINT ( 'NONE',  ( -17.37639885904427217, -8.896818990903957669, 8.082699191722323206 ) ) ;
#3754=CARTESIAN_POINT ( 'NONE',  ( -35.00000000000000000, 0.000000000000000000, 0.000000000000000000 ) ) ;
#3755=LINE ( 'NONE', #45266, #20498 ) ;
#3756=B_SPLINE_CURVE_WITH_KNOTS ( 'NONE', 3,
 ( #16101, #41361, #46691, #45375, #1149, #4841, #30414, #50395 ),
 .UNSPECIFIED., .F., .F.,
 ( 4, 2, 2, 4 ),
 ( 8.673617379884035472E-19, 0.002119351272183964390, 0.003179026908275949404, 0.004238702544367933985 ),
 .UNSPECIFIED. ) ;
#3758=AXIS2_PLACEMENT_3D ( 'NONE', #10391, #45326, #34991 ) ;
#3760=DIRECTION ( 'NONE',  ( -1.000000000000000000, 0.000000000000000000, 0.000000000000000000 ) ) ;
#3761=ORIENTED_EDGE ( 'NONE', *, *, #40239, .T. ) ;
#3762=DIRECTION ( 'NONE',  ( 0.000000000000000000, 0.01356324068817998940, -0.9999080150203989437 ) ) ;
#3763=CARTESIAN_POINT ( 'NONE',  ( 36.00000000000000711, 12.71517666308947980, -0.9416912585474879194 ) ) ;
#3765=CARTESIAN_POINT ( 'NONE',  ( -36.00000000000000711, -8.235637554476577193, -9.733281772932251386 ) ) ;
#3766=ORIENTED_EDGE ( 'NONE', *, *, #26056, .F. ) ;
#3769=ORIENTED_EDGE ( 'NONE', *, *, #55650, .T. ) ;
#3770=CARTESIAN_POINT ( 'NONE',  ( 29.72939054355411770, -10.04502241635329618, 9.030387493296032630 ) ) ;
#3771=EDGE_CURVE ( 'NONE', #42318, #41624, #9601, .T. ) ;
#3777=EDGE_LOOP ( 'NONE', ( #65203, #65443, #9866, #50058 ) ) ;
#3778=AXIS2_PLACEMENT_3D ( 'NONE', #57873, #7295, #47878 ) ;
#3779=CARTESIAN_POINT ( 'NONE',  ( 35.00000000000000000, 3.213188559034240832, -11.29812557209478285 ) ) ;
#3780=ADVANCED_FACE ( 'NONE', ( #47099 ), #42725, .T. ) ;
#3782=DIRECTION ( 'NONE',  ( 0.000000000000000000, -0.01356324068818000848, 0.9999080150203990547 ) ) ;
#3784=EDGE_LOOP ( 'NONE', ( #18917, #35647, #59782, #31930 ) ) ;
#3787=ORIENTED_EDGE ( 'NONE', *, *, #20519, .T. ) ;
#3788=DIRECTION ( 'NONE',  ( -1.000000000000000000, 0.000000000000000000, 0.000000000000000000 ) ) ;
#3789=ORIENTED_EDGE ( 'NONE', *, *, #32404, .F. ) ;
#3790=DIRECTION ( 'NONE',  ( -1.000000000000000000, -0.000000000000000000, 0.000000000000000000 ) ) ;
#3792=CIRCLE ( 'NONE', #9071, 12.74999999999999822 ) ;
#3793=FACE_OUTER_BOUND ( 'NONE', #15978, .T. ) ;
#3794=DIRECTION ( 'NONE',  ( -1.000000000000000000, -1.836970198721029688E-16, -0.000000000000000000 ) ) ;
#3796=EDGE_CURVE ( 'NONE', #8191, #32188, #23289, .T. ) ;
#3797=DIRECTION ( 'NONE',  ( 0.000000000000000000, -0.01356324068817991828, 0.9999080150203990547 ) ) ;
#3800=ORIENTED_EDGE ( 'NONE', *, *, #53495, .T. ) ;
#3801=VERTEX_POINT ( 'NONE', #1862 ) ;
#3803=ORIENTED_EDGE ( 'NONE', *, *, #57741, .F. ) ;
#3808=FACE_OUTER_BOUND ( 'NONE', #56333, .T. ) ;
#3810=EDGE_CURVE ( 'NONE', #40981, #64820, #53048, .T. ) ;
#3813=AXIS2_PLACEMENT_3D ( 'NONE', #63470, #49206, #53851 ) ;
#3814=CARTESIAN_POINT ( 'NONE',  ( -35.00000000000000000, 0.000000000000000000, 0.000000000000000000 ) ) ;
#3816=ORIENTED_EDGE ( 'NONE', *, *, #62229, .F. ) ;
#3817=DIRECTION ( 'NONE',  ( -1.000000000000000000, 0.000000000000000000, 0.000000000000000000 ) ) ;
#3818=ADVANCED_FACE ( 'NONE', ( #28425 ), #13143, .T. ) ;
#3820=CARTESIAN_POINT ( 'NONE',  ( -17.34810147968408955, -8.828308823152831053, 10.23480574679286548 ) ) ;
#3824=CARTESIAN_POINT ( 'NONE',  ( -37.00000000000000711, -0.1414404973751262617, -12.74921544981111410 ) ) ;
#3826=CYLINDRICAL_SURFACE ( 'NONE', #63790, 4.999999999999999112 ) ;
#3828=DIRECTION ( 'NONE',  ( 1.000000000000000000, 0.000000000000000000, 0.000000000000000000 ) ) ;
#3829=ADVANCED_FACE ( 'NONE', ( #38745 ), #19113, .T. ) ;
#3830=CARTESIAN_POINT ( 'NONE',  ( -47.00000000000000711, 0.000000000000000000, 0.000000000000000000 ) ) ;
#3831=DIRECTION ( 'NONE',  ( -1.000000000000000000, -0.000000000000000000, 0.000000000000000000 ) ) ;
#3832=ORIENTED_EDGE ( 'NONE', *, *, #46902, .F. ) ;
#3833=DIRECTION ( 'NONE',  ( -1.000000000000000000, -0.000000000000000000, 0.000000000000000000 ) ) ;
#3834=CARTESIAN_POINT ( 'NONE',  ( -9.792688973508125727, -10.81058943113889015, -5.226288967600182467 ) ) ;
#3841=ORIENTED_EDGE ( 'NONE', *, *, #37598, .F. ) ;
#3842=DIRECTION ( 'NONE',  ( 0.000000000000000000, -0.01356324068818000328, 0.9999080150203990547 ) ) ;
#3846=CARTESIAN_POINT ( 'NONE',  ( 37.00000000000000711, 0.9416912585476251429, 12.71517666308946382 ) ) ;
#3848=CARTESIAN_POINT ( 'NONE',  ( 35.00000000000000000, 4.705694406421931860E-17, -3.469127814946512892E-15 ) ) ;
#3850=DIRECTION ( 'NONE',  ( 0.000000000000000000, -0.2960891610144378849, -0.9551603052523520709 ) ) ;
#3852=CYLINDRICAL_SURFACE ( 'NONE', #59649, 12.75000000000000178 ) ;
#3854=ORIENTED_EDGE ( 'NONE', *, *, #3002, .F. ) ;
#3855=DIRECTION ( 'NONE',  ( 1.000000000000000000, 0.000000000000000000, 0.000000000000000000 ) ) ;
#3856=ORIENTED_EDGE ( 'NONE', *, *, #59311, .F. ) ;
#3857=ORIENTED_EDGE ( 'NONE', *, *, #39106, .F. ) ;
#3858=LINE ( 'NONE', #13465, #33688 ) ;
#3860=CARTESIAN_POINT ( 'NONE',  ( -3.762642749413128485, 7.436900049367464405, 9.428156105167504464 ) ) ;
#3861=CARTESIAN_POINT ( 'NONE',  ( 24.05602761403608270, -2.477051208052090558, 11.74280428119080355 ) ) ;
#3862=AXIS2_PLACEMENT_3D ( 'NONE', #16676, #54232, #64206 ) ;
#3863=CARTESIAN_POINT ( 'NONE',  ( 35.00000000000000000, -5.672855678558609505, 10.28547182238013669 ) ) ;
#3866=ORIENTED_EDGE ( 'NONE', *, *, #48987, .F. ) ;
#3868=ORIENTED_EDGE ( 'NONE', *, *, #11142, .T. ) ;
#3869=DIRECTION ( 'NONE',  ( 0.000000000000000000, 0.4380125133593913422, -0.8989688749565187820 ) ) ;
#3872=EDGE_CURVE ( 'NONE', #9460, #815, #53390, .T. ) ;
#3873=CARTESIAN_POINT ( 'NONE',  ( 35.00000000000000000, 9.926225166347027340, -6.280308599560179061 ) ) ;
#3874=FACE_OUTER_BOUND ( 'NONE', #25209, .T. ) ;
#3875=EDGE_CURVE ( 'NONE', #30274, #48764, #26612, .T. ) ;
#3876=CARTESIAN_POINT ( 'NONE',  ( 22.36482863261543486, 25.00000000000000000, -0.9234811557364158707 ) ) ;
#3877=VERTEX_POINT ( 'NONE', #23118 ) ;
#3878=VERTEX_POINT ( 'NONE', #18797 ) ;
#3882=CARTESIAN_POINT ( 'NONE',  ( -34.00000000000000000, 11.99999999999999822, 1.469576158976823750E-15 ) ) ;
#3884=CARTESIAN_POINT ( 'NONE',  ( -28.21800245578230815, 12.11161220946422290, -5.971072691807515653 ) ) ;
#3885=CARTESIAN_POINT ( 'NONE',  ( -8.782159582855564750, -2.870306520432511554, -11.65443128345066626 ) ) ;
#3886=CARTESIAN_POINT ( 'NONE',  ( -37.00000000000000711, 0.000000000000000000, 0.000000000000000000 ) ) ;
#3888=DIRECTION ( 'NONE',  ( -1.000000000000000000, 0.000000000000000000, -0.000000000000000000 ) ) ;
#3890=LINE ( 'NONE', #59735, #16567 ) ;
#3894=EDGE_CURVE ( 'NONE', #12199, #11505, #11743, .T. ) ;
#3895=AXIS2_PLACEMENT_3D ( 'NONE', #44058, #64326, #29100 ) ;
#3897=EDGE_CURVE ( 'NONE', #7867, #29014, #23794, .T. ) ;
#3900=ORIENTED_EDGE ( 'NONE', *, *, #53832, .T. ) ;
#3906=CARTESIAN_POINT ( 'NONE',  ( 16.78263030916553333, -12.17295508002144011, 5.836879698929882565 ) ) ;
#3908=CARTESIAN_POINT ( 'NONE',  ( -47.00000000000000711, 0.000000000000000000, 0.000000000000000000 ) ) ;
#3909=CARTESIAN_POINT ( 'NONE',  ( -37.00000000000000711, -2.216820770815165265, 11.53507381115582575 ) ) ;
#3910=DIRECTION ( 'NONE',  ( 0.000000000000000000, -0.8515178078024812081, 0.5243256840888652626 ) ) ;
#3911=ORIENTED_EDGE ( 'NONE', *, *, #24453, .F. ) ;
#3914=DIRECTION ( 'NONE',  ( -1.000000000000000000, 0.000000000000000000, -0.000000000000000000 ) ) ;
#3917=DIRECTION ( 'NONE',  ( 0.000000000000000000, -0.9847383929261599445, 0.1740410799127720953 ) ) ;
#3918=CARTESIAN_POINT ( 'NONE',  ( -29.28143770085004505, 2.978801202832155326, -11.65275938077009066 ) ) ;
#3919=DIRECTION ( 'NONE',  ( 0.000000000000000000, -1.000000000000000000, 0.000000000000000000 ) ) ;
#3920=ORIENTED_EDGE ( 'NONE', *, *, #25974, .F. ) ;
#3922=ORIENTED_EDGE ( 'NONE', *, *, #54696, .F. ) ;
#3923=LINE ( 'NONE', #58818, #22566 ) ;
#3924=VERTEX_POINT ( 'NONE', #55008 ) ;
#3925=EDGE_CURVE ( 'NONE', #14535, #41991, #42536, .T. ) ;
#3926=DIRECTION ( 'NONE',  ( -1.000000000000000000, 0.000000000000000000, 0.000000000000000000 ) ) ;
#3930=DIRECTION ( 'NONE',  ( -1.000000000000000000, -0.000000000000000000, 0.000000000000000000 ) ) ;
#3932=ORIENTED_EDGE ( 'NONE', *, *, #11915, .T. ) ;
#3933=LINE ( 'NONE', #20187, #7717 ) ;
#3934=DIRECTION ( 'NONE',  ( 1.000000000000000000, 0.000000000000000000, 0.000000000000000000 ) ) ;
#3936=CIRCLE ( 'NONE', #753, 5.000000000000001776 ) ;
#3937=CARTESIAN_POINT ( 'NONE',  ( -35.00000000000000000, -12.66641127287624968, -1.457575200925677494 ) ) ;
#3938=ORIENTED_EDGE ( 'NONE', *, *, #2595, .T. ) ;
#3940=ADVANCED_FACE ( 'NONE', ( #20094 ), #54708, .F. ) ;
#3943=CARTESIAN_POINT ( 'NONE',  ( 37.00000000000000711, -10.01317267707881342, 6.946017217730045878 ) ) ;
#3944=CIRCLE ( 'NONE', #26241, 12.74999999999999822 ) ;
#3947=ORIENTED_EDGE ( 'NONE', *, *, #28526, .T. ) ;
#3949=CARTESIAN_POINT ( 'NONE',  ( -15.95528719064657075, 7.880328173109766965, 9.049993051904070995 ) ) ;
#3950=ADVANCED_FACE ( 'NONE', ( #10429 ), #4153, .T. ) ;
#3951=CARTESIAN_POINT ( 'NONE',  ( 37.00000000000000711, -8.366449238204431538, -9.621072037176967129 ) ) ;
#3952=DIRECTION ( 'NONE',  ( 0.000000000000000000, -0.01356324068817998940, 0.9999080150203990547 ) ) ;
#3954=CARTESIAN_POINT ( 'NONE',  ( 23.55545670043567341, -3.418074724591041669, 13.06318810598877356 ) ) ;
#3957=FACE_OUTER_BOUND ( 'NONE', #17320, .T. ) ;
#3959=CARTESIAN_POINT ( 'NONE',  ( 35.00000000000000000, 4.705694406421931860E-17, -3.469127814946512892E-15 ) ) ;
#3960=VERTEX_POINT ( 'NONE', #9780 ) ;
#3962=DIRECTION ( 'NONE',  ( 0.000000000000000000, 0.01356324068817998940, -0.9999080150203989437 ) ) ;
#3964=DIRECTION ( 'NONE',  ( -1.000000000000000000, 0.000000000000000000, 0.000000000000000000 ) ) ;
#3966=EDGE_LOOP ( 'NONE', ( #4762, #13373, #52001, #43164 ) ) ;
#3967=CARTESIAN_POINT ( 'NONE',  ( -35.00000000000000000, -6.280308599560071592, -9.926225166347094842 ) ) ;
#3968=LINE ( 'NONE', #32885, #35289 ) ;
#3969=LINE ( 'NONE', #24233, #43918 ) ;
#3973=CIRCLE ( 'NONE', #36851, 12.18649999999999878 ) ;
#3974=VERTEX_POINT ( 'NONE', #19780 ) ;
#3976=ORIENTED_EDGE ( 'NONE', *, *, #63079, .F. ) ;
#3979=CIRCLE ( 'NONE', #28369, 12.18650000000000055 ) ;
#3980=CARTESIAN_POINT ( 'NONE',  ( 37.00000000000000711, -12.63095688309027764, 1.738225594540123708 ) ) ;
#3982=EDGE_CURVE ( 'NONE', #30390, #46189, #44689, .T. ) ;
#3983=VERTEX_POINT ( 'NONE', #30065 ) ;
#3987=CARTESIAN_POINT ( 'NONE',  ( -35.00000000000000000, 9.677500615117999416, -6.657191900728212985 ) ) ;
#3989=FACE_OUTER_BOUND ( 'NONE', #14522, .T. ) ;
#3991=CARTESIAN_POINT ( 'NONE',  ( -18.11249319439446737, -11.56825399538298882, 3.263832109282014393 ) ) ;
#3992=EDGE_LOOP ( 'NONE', ( #30418, #17987, #62430, #32757 ) ) ;
#3994=ORIENTED_EDGE ( 'NONE', *, *, #15090, .F. ) ;
#3995=ORIENTED_EDGE ( 'NONE', *, *, #61519, .F. ) ;
#4000=CARTESIAN_POINT ( 'NONE',  ( -35.00000000000000000, 0.000000000000000000, 0.000000000000000000 ) ) ;
#4001=ORIENTED_EDGE ( 'NONE', *, *, #52857, .F. ) ;
#4003=DIRECTION ( 'NONE',  ( 0.000000000000000000, -0.01356324068817998940, 0.9999080150203990547 ) ) ;
#4005=ORIENTED_EDGE ( 'NONE', *, *, #64620, .T. ) ;
#4006=ORIENTED_EDGE ( 'NONE', *, *, #51893, .T. ) ;
#4009=ORIENTED_EDGE ( 'NONE', *, *, #28726, .F. ) ;
#4010=CARTESIAN_POINT ( 'NONE',  ( 36.00000000000000711, -0.4871980014160596784, 12.74068829017554094 ) ) ;
#4013=ORIENTED_EDGE ( 'NONE', *, *, #41975, .F. ) ;
#4015=DIRECTION ( 'NONE',  ( -1.000000000000000000, -1.836970198721029688E-16, -0.000000000000000000 ) ) ;
#4016=EDGE_CURVE ( 'NONE', #45368, #8244, #2504, .T. ) ;
#4017=DIRECTION ( 'NONE',  ( 1.000000000000000000, 0.000000000000000000, -0.000000000000000000 ) ) ;
#4018=FACE_OUTER_BOUND ( 'NONE', #19946, .T. ) ;
#4021=DIRECTION ( 'NONE',  ( 0.000000000000000000, -0.01356324068818000848, 0.9999080150203990547 ) ) ;
#4022=AXIS2_PLACEMENT_3D ( 'NONE', #62808, #16939, #52540 ) ;
#4025=CARTESIAN_POINT ( 'NONE',  ( -17.83717122027472612, -8.628852110296120870, -10.38608613287006044 ) ) ;
#4026=ORIENTED_EDGE ( 'NONE', *, *, #24613, .F. ) ;
#4027=CARTESIAN_POINT ( 'NONE',  ( -16.48583967416821494, 8.235227529897704457, 8.728494452408142479 ) ) ;
#4028=CYLINDRICAL_SURFACE ( 'NONE', #13826, 12.18650000000000055 ) ;
#4030=CIRCLE ( 'NONE', #43262, 4.999999999999999112 ) ;
#4031=VERTEX_POINT ( 'NONE', #40037 ) ;
#4032=EDGE_CURVE ( 'NONE', #63155, #33997, #44094, .T. ) ;
#4033=ORIENTED_EDGE ( 'NONE', *, *, #4631, .F. ) ;
#4034=VECTOR ( 'NONE', #25844, 1000.000000000000000 ) ;
#4036=ORIENTED_EDGE ( 'NONE', *, *, #33420, .T. ) ;
#4037=DIRECTION ( 'NONE',  ( 0.000000000000000000, 0.01356324068817998940, -0.9999080150203990547 ) ) ;
#4038=CARTESIAN_POINT ( 'NONE',  ( -25.54417658651491863, 25.00000000000000000, 11.22596262356930197 ) ) ;
#4040=CARTESIAN_POINT ( 'NONE',  ( -37.00000000000000711, 1.039216533673073206, -11.70009620280410445 ) ) ;
#4041=CARTESIAN_POINT ( 'NONE',  ( 35.00000000000000000, 4.705694406421931860E-17, -3.469127814946512892E-15 ) ) ;
#4045=EDGE_CURVE ( 'NONE', #3673, #52526, #29625, .T. ) ;
#4046=FACE_OUTER_BOUND ( 'NONE', #63130, .T. ) ;
#4050=CYLINDRICAL_SURFACE ( 'NONE', #21934, 12.18650000000000055 ) ;
#4051=DIRECTION ( 'NONE',  ( 1.000000000000000000, -0.000000000000000000, 0.000000000000000000 ) ) ;
#4053=EDGE_CURVE ( 'NONE', #6027, #3315, #27985, .T. ) ;
#4055=CARTESIAN_POINT ( 'NONE',  ( -30.18541646480307250, -1.416020129149132112, 11.91616074890920096 ) ) ;
#4058=FACE_OUTER_BOUND ( 'NONE', #41489, .T. ) ;
#4061=VECTOR ( 'NONE', #54326, 1000.000000000000000 ) ;
#4063=VERTEX_POINT ( 'NONE', #51685 ) ;
#4064=EDGE_CURVE ( 'NONE', #28784, #29441, #32234, .T. ) ;
#4065=ORIENTED_EDGE ( 'NONE', *, *, #42941, .F. ) ;
#4066=ORIENTED_EDGE ( 'NONE', *, *, #43284, .F. ) ;
#4067=DIRECTION ( 'NONE',  ( -1.000000000000000000, 0.000000000000000000, 0.000000000000000000 ) ) ;
#4068=CARTESIAN_POINT ( 'NONE',  ( -27.75688124897997966, 10.82714900795144253, -5.182596736677783866 ) ) ;
#4071=DIRECTION ( 'NONE',  ( 0.000000000000000000, -0.01356324068817991828, 0.9999080150203990547 ) ) ;
#4072=CARTESIAN_POINT ( 'NONE',  ( 37.00000000000000711, -9.430788938293991563, 7.718225330433904574 ) ) ;
#4073=DIRECTION ( 'NONE',  ( -1.000000000000000000, -0.000000000000000000, -0.000000000000000000 ) ) ;
#4075=( BOUNDED_CURVE ( )  B_SPLINE_CURVE ( 3, ( #1540, #5880, #26137, #46415 ),
 .UNSPECIFIED., .F., .F. ) 
 B_SPLINE_CURVE_WITH_KNOTS ( ( 4, 4 ),
 ( 4.422350118998207513, 4.437400365793983781 ),
 .UNSPECIFIED. ) 
 CURVE ( )  GEOMETRIC_REPRESENTATION_ITEM ( )  RATIONAL_B_SPLINE_CURVE ( ( 1.000000000000000000, 0.9999811242616895024, 0.9999811242616895024, 1.000000000000000000 ) ) 
 REPRESENTATION_ITEM ( '' )  );
#4078=CARTESIAN_POINT ( 'NONE',  ( -29.58114640908272364, -2.918339774162580280, -11.64592837444328666 ) ) ;
#4079=DIRECTION ( 'NONE',  ( 1.000000000000000000, -0.000000000000000000, 0.000000000000000000 ) ) ;
#4081=CARTESIAN_POINT ( 'NONE',  ( 22.61491127797214062, 25.00000000000000000, 9.376349503825034404 ) ) ;
#4085=PLANE ( 'NONE',  #41034 ) ;
#4086=CARTESIAN_POINT ( 'NONE',  ( 32.00000000000000000, 1.230770033143089974E-14, 0.000000000000000000 ) ) ;
#4087=DIRECTION ( 'NONE',  ( -1.000000000000000000, 0.000000000000000000, 0.000000000000000000 ) ) ;
#4089=VECTOR ( 'NONE', #6896, 1000.000000000000000 ) ;
#4093=DIRECTION ( 'NONE',  ( 0.000000000000000000, 0.7196168960969817618, 0.6943713148249613942 ) ) ;
#4095=ORIENTED_EDGE ( 'NONE', *, *, #44938, .T. ) ;
#4096=AXIS2_PLACEMENT_3D ( 'NONE', #42756, #52444, #12492 ) ;
#4098=EDGE_LOOP ( 'NONE', ( #8112, #51549, #52752, #49493 ) ) ;
#4104=CYLINDRICAL_SURFACE ( 'NONE', #29932, 4.999999999999999112 ) ;
#4106=ADVANCED_FACE ( 'NONE', ( #16428 ), #56993, .T. ) ;
#4107=DIRECTION ( 'NONE',  ( -1.000000000000000000, 0.000000000000000000, 0.000000000000000000 ) ) ;
#4108=CARTESIAN_POINT ( 'NONE',  ( 35.00000000000000000, -11.05394794832825767, 5.130401251914841865 ) ) ;
#4109=VECTOR ( 'NONE', #22187, 1000.000000000000000 ) ;
#4110=CIRCLE ( 'NONE', #12579, 12.75000000000000178 ) ;
#4111=ORIENTED_EDGE ( 'NONE', *, *, #53102, .T. ) ;
#4112=DIRECTION ( 'NONE',  ( 0.000000000000000000, 0.2960891610144510966, 0.9551603052523478521 ) ) ;
#4114=AXIS2_PLACEMENT_3D ( 'NONE', #54241, #53911, #23986 ) ;
#4116=ORIENTED_EDGE ( 'NONE', *, *, #55631, .F. ) ;
#4117=VECTOR ( 'NONE', #3564, 1000.000000000000000 ) ;
#4118=ADVANCED_FACE ( 'NONE', ( #31688 ), #27363, .T. ) ;
#4120=CARTESIAN_POINT ( 'NONE',  ( -5.873305616363168724, -0.9854497472355991938, 13.46436504529688349 ) ) ;
#4121=EDGE_CURVE ( 'NONE', #48838, #42404, #43930, .T. ) ;
#4122=CARTESIAN_POINT ( 'NONE',  ( 35.00000000000000000, 11.66664283989686979, 5.143145423404150485 ) ) ;
#4124=ORIENTED_EDGE ( 'NONE', *, *, #43841, .T. ) ;
#4126=DIRECTION ( 'NONE',  ( 0.000000000000000000, -0.9999080150203988326, -0.01356324068819046366 ) ) ;
#4127=CARTESIAN_POINT ( 'NONE',  ( 3.153349365415208716, 2.981698431668006410, 11.62552590921464990 ) ) ;
#4129=AXIS2_PLACEMENT_3D ( 'NONE', #65505, #50582, #50898 ) ;
#4131=LINE ( 'NONE', #35679, #5523 ) ;
#4132=LINE ( 'NONE', #50014, #61681 ) ;
#4133=EDGE_LOOP ( 'NONE', ( #52201, #31547, #59214, #35250 ) ) ;
#4134=CIRCLE ( 'NONE', #63588, 12.18650000000000055 ) ;
#4135=DIRECTION ( 'NONE',  ( 1.000000000000000000, 0.000000000000000000, 0.000000000000000000 ) ) ;
#4136=EDGE_CURVE ( 'NONE', #39957, #29408, #4640, .T. ) ;
#4138=CARTESIAN_POINT ( 'NONE',  ( 35.00000000000000000, -3.511814412392203266, -11.66953048682398730 ) ) ;
#4139=ORIENTED_EDGE ( 'NONE', *, *, #28623, .T. ) ;
#4140=CARTESIAN_POINT ( 'NONE',  ( 8.437200413559441614, 4.476360154859203355, 12.73625532737111143 ) ) ;
#4141=DIRECTION ( 'NONE',  ( 0.000000000000000000, -0.01356324068817998940, 0.9999080150203990547 ) ) ;
#4142=EDGE_LOOP ( 'NONE', ( #48265, #50609, #32135, #63906 ) ) ;
#4143=VERTEX_POINT ( 'NONE', #31051 ) ;
#4145=DIRECTION ( 'NONE',  ( 0.000000000000000000, 0.01356324068817998940, -0.9999080150203989437 ) ) ;
#4147=ORIENTED_EDGE ( 'NONE', *, *, #33585, .T. ) ;
#4149=CARTESIAN_POINT ( 'NONE',  ( -36.00000000000000711, 10.93004082984018588, 6.564808257521810297 ) ) ;
#4150=CYLINDRICAL_SURFACE ( 'NONE', #2855, 10.20557198542813815 ) ;
#4151=AXIS2_PLACEMENT_3D ( 'NONE', #4799, #25064, #25714 ) ;
#4152=FACE_OUTER_BOUND ( 'NONE', #54205, .T. ) ;
#4153=CYLINDRICAL_SURFACE ( 'NONE', #35411, 12.18650000000000055 ) ;
#4159=CARTESIAN_POINT ( 'NONE',  ( -47.00000000000000711, 0.000000000000000000, 0.000000000000000000 ) ) ;
#4161=FACE_OUTER_BOUND ( 'NONE', #60835, .T. ) ;
#4163=AXIS2_PLACEMENT_3D ( 'NONE', #61032, #19814, #4858 ) ;
#4167=CARTESIAN_POINT ( 'NONE',  ( -35.00000000000000000, 2.905556151562625811, 11.38112321385051651 ) ) ;
#4169=B_SPLINE_CURVE_WITH_KNOTS ( 'NONE', 3,
 ( #8974, #3991, #20248, #64801, #25240, #24590, #44524, #65462 ),
 .UNSPECIFIED., .F., .F.,
 ( 4, 2, 2, 4 ),
 ( 8.673617379884035472E-19, 0.002049566690290811118, 0.003074350035436216894, 0.004099133380581623104 ),
 .UNSPECIFIED. ) ;
#4170=CARTESIAN_POINT ( 'NONE',  ( -37.00000000000000711, -12.18359334611896472, -0.2661492558804631203 ) ) ;
#4172=ORIENTED_EDGE ( 'NONE', *, *, #11777, .T. ) ;
#4175=ORIENTED_EDGE ( 'NONE', *, *, #21479, .T. ) ;
#4178=DIRECTION ( 'NONE',  ( -1.000000000000000000, 0.000000000000000000, 0.000000000000000000 ) ) ;
#4180=EDGE_CURVE ( 'NONE', #45226, #58319, #38610, .T. ) ;
#4181=PLANE ( 'NONE',  #27785 ) ;
#4182=AXIS2_PLACEMENT_3D ( 'NONE', #9656, #4373, #4719 ) ;
#4183=CARTESIAN_POINT ( 'NONE',  ( -36.00000000000000711, 8.366449238204365813, 9.621072037177027525 ) ) ;
#4184=ORIENTED_EDGE ( 'NONE', *, *, #30714, .T. ) ;
#4185=AXIS2_PLACEMENT_3D ( 'NONE', #62549, #41954, #37635 ) ;
#4189=ADVANCED_FACE ( 'NONE', ( #17407 ), #33002, .T. ) ;
#4190=DIRECTION ( 'NONE',  ( 0.000000000000000000, 0.3554799084908899509, 0.9346839223284567622 ) ) ;
#4191=VECTOR ( 'NONE', #36169, 1000.000000000000000 ) ;
#4193=EDGE_CURVE ( 'NONE', #59561, #50772, #14145, .T. ) ;
#4194=DIRECTION ( 'NONE',  ( 1.000000000000000000, -0.000000000000000000, 0.000000000000000000 ) ) ;
#4195=CIRCLE ( 'NONE', #45578, 12.74999999999999822 ) ;
#4196=CARTESIAN_POINT ( 'NONE',  ( 6.992580758904643368, -4.514504415418986838, -12.72890816843052697 ) ) ;
#4197=CARTESIAN_POINT ( 'NONE',  ( 37.00000000000000711, 11.78745411414844035, 3.093009498343795460 ) ) ;
#4199=DIRECTION ( 'NONE',  ( 1.000000000000000000, -0.000000000000000000, 0.000000000000000000 ) ) ;
#4200=ADVANCED_FACE ( 'NONE', ( #23051 ), #33988, .T. ) ;
#4204=CARTESIAN_POINT ( 'NONE',  ( 21.90174657591892071, 13.47998113580524659, -0.7349207973210680755 ) ) ;
#4207=CARTESIAN_POINT ( 'NONE',  ( -27.75187954703365634, -11.73910552422975861, -2.553580313601046203 ) ) ;
#4208=EDGE_LOOP ( 'NONE', ( #64650, #65545, #55244, #61218 ) ) ;
#4209=CARTESIAN_POINT ( 'NONE',  ( 35.00000000000000000, -11.66664283989683426, -5.143145423404237526 ) ) ;
#4211=EDGE_CURVE ( 'NONE', #24405, #2547, #22673, .T. ) ;
#4213=ORIENTED_EDGE ( 'NONE', *, *, #6171, .F. ) ;
#4214=CARTESIAN_POINT ( 'NONE',  ( -37.00000000000000711, 1.488153103997124971, -11.65150730582933036 ) ) ;
#4215=CARTESIAN_POINT ( 'NONE',  ( -35.00000000000000000, 7.608228585767725427, 10.23119532541075216 ) ) ;
#4219=CARTESIAN_POINT ( 'NONE',  ( 35.00000000000000000, -9.060822531525994705, 7.474872387601095625 ) ) ;
#4220=DIRECTION ( 'NONE',  ( 1.000000000000000000, 0.000000000000000000, 0.000000000000000000 ) ) ;
#4222=CIRCLE ( 'NONE', #5273, 4.999999999999999112 ) ;
#4223=AXIS2_PLACEMENT_3D ( 'NONE', #55461, #25519, #46155 ) ;
#4225=ADVANCED_FACE ( 'NONE', ( #7403 ), #27691, .T. ) ;
#4226=VERTEX_POINT ( 'NONE', #2792 ) ;
#4228=CARTESIAN_POINT ( 'NONE',  ( -2.532614230583026593, -5.020478806276874373, 10.89930238848911337 ) ) ;
#4229=CARTESIAN_POINT ( 'NONE',  ( -47.00000000000000711, 0.000000000000000000, 0.000000000000000000 ) ) ;
#4232=VECTOR ( 'NONE', #49031, 1000.000000000000000 ) ;
#4235=DIRECTION ( 'NONE',  ( 0.000000000000000000, -0.01356324068817998940, 0.9999080150203990547 ) ) ;
#4236=CARTESIAN_POINT ( 'NONE',  ( -27.01437459610461644, -8.723448335974111956, -8.240233560378637634 ) ) ;
#4237=ORIENTED_EDGE ( 'NONE', *, *, #56944, .F. ) ;
#4238=ORIENTED_EDGE ( 'NONE', *, *, #21607, .T. ) ;
#4239=CARTESIAN_POINT ( 'NONE',  ( -17.83857753042823902, -8.695343837413979315, -8.292117721727052526 ) ) ;
#4240=EDGE_LOOP ( 'NONE', ( #2745, #13939, #33885, #15924 ) ) ;
#4241=CIRCLE ( 'NONE', #19092, 4.999999999999999112 ) ;
#4242=CARTESIAN_POINT ( 'NONE',  ( -35.00000000000000000, -12.00000000000000000, 0.000000000000000000 ) ) ;
#4243=DIRECTION ( 'NONE',  ( 1.000000000000000000, -0.000000000000000000, 0.000000000000000000 ) ) ;
#4248=CARTESIAN_POINT ( 'NONE',  ( 37.00000000000000711, 7.882940143791775434, -10.02106554660711701 ) ) ;
#4249=ORIENTED_EDGE ( 'NONE', *, *, #15145, .F. ) ;
#4251=ORIENTED_EDGE ( 'NONE', *, *, #12653, .T. ) ;
#4253=CARTESIAN_POINT ( 'NONE',  ( -37.00000000000000711, -1.171570255487366152, -11.68758509253249400 ) ) ;
#4256=CARTESIAN_POINT ( 'NONE',  ( -37.00000000000000711, -11.72195762423409349, -0.7536123767499773862 ) ) ;
#4257=ORIENTED_EDGE ( 'NONE', *, *, #33036, .T. ) ;
#4258=CYLINDRICAL_SURFACE ( 'NONE', #60696, 12.18650000000000055 ) ;
#4259=CARTESIAN_POINT ( 'NONE',  ( -35.00000000000000000, 11.59095880812008161, -1.903127969211228621 ) ) ;
#4260=EDGE_CURVE ( 'NONE', #10291, #40353, #59006, .T. ) ;
#4263=CYLINDRICAL_SURFACE ( 'NONE', #13170, 8.549672981451799103 ) ;
#4264=ORIENTED_EDGE ( 'NONE', *, *, #37117, .F. ) ;
#4265=DIRECTION ( 'NONE',  ( 0.000000000000000000, -0.01356324068817992175, 0.9999080150203990547 ) ) ;
#4266=CARTESIAN_POINT ( 'NONE',  ( 35.00000000000000000, 4.705694406421931860E-17, -3.469127814946512892E-15 ) ) ;
#4267=CARTESIAN_POINT ( 'NONE',  ( 37.00000000000000711, 4.705694406421931860E-17, -3.469127814946512892E-15 ) ) ;
#4269=DIRECTION ( 'NONE',  ( 1.000000000000000000, 0.000000000000000000, 0.000000000000000000 ) ) ;
#4272=DIRECTION ( 'NONE',  ( 1.000000000000000000, 0.000000000000000000, 0.000000000000000000 ) ) ;
#4275=CIRCLE ( 'NONE', #13787, 5.000000000000000000 ) ;
#4279=VERTEX_POINT ( 'NONE', #18731 ) ;
#4283=DIRECTION ( 'NONE',  ( 0.000000000000000000, -0.01356324068817998940, 0.9999080150203990547 ) ) ;
#4286=EDGE_LOOP ( 'NONE', ( #15085, #60183, #25685, #45669 ) ) ;
#4289=CARTESIAN_POINT ( 'NONE',  ( 35.00000000000000000, 2.497432891016841960, -11.47758908105695319 ) ) ;
#4290=DIRECTION ( 'NONE',  ( 0.000000000000000000, -0.9937233664769772323, 0.1118654143051511785 ) ) ;
#4291=ADVANCED_FACE ( 'NONE', ( #54931 ), #39642, .T. ) ;
#4292=CIRCLE ( 'NONE', #43526, 12.18649999999999878 ) ;
#4293=VECTOR ( 'NONE', #65377, 1000.000000000000000 ) ;
#4294=DIRECTION ( 'NONE',  ( -1.000000000000000000, 0.000000000000000000, 0.000000000000000000 ) ) ;
#4295=ORIENTED_EDGE ( 'NONE', *, *, #11269, .F. ) ;
#4296=DIRECTION ( 'NONE',  ( 1.000000000000000000, 0.000000000000000000, 0.000000000000000000 ) ) ;
#4297=ORIENTED_EDGE ( 'NONE', *, *, #64865, .F. ) ;
#4299=LINE ( 'NONE', #24574, #44807 ) ;
#4300=AXIS2_PLACEMENT_3D ( 'NONE', #26328, #42578, #6720 ) ;
#4301=CARTESIAN_POINT ( 'NONE',  ( -2.676156797222401185, -7.839276155712920691, 10.99183054655307856 ) ) ;
#4304=VERTEX_POINT ( 'NONE', #14669 ) ;
#4305=EDGE_LOOP ( 'NONE', ( #4172, #9214, #35617, #52439 ) ) ;
#4307=EDGE_CURVE ( 'NONE', #1585, #3924, #54578, .T. ) ;
#4309=AXIS2_PLACEMENT_3D ( 'NONE', #21509, #26816, #38687 ) ;
#4311=DIRECTION ( 'NONE',  ( 0.000000000000000000, 0.1118654143051615590, 0.9937233664769760111 ) ) ;
#4313=DIRECTION ( 'NONE',  ( 1.000000000000000000, 0.000000000000000000, -0.000000000000000000 ) ) ;
#4317=CARTESIAN_POINT ( 'NONE',  ( -37.00000000000000711, 2.865935305911801123, -12.42372387097879383 ) ) ;
#4318=VERTEX_POINT ( 'NONE', #64565 ) ;
#4325=CIRCLE ( 'NONE', #64809, 5.000000000000000888 ) ;
#4326=AXIS2_PLACEMENT_3D ( 'NONE', #14273, #58888, #43542 ) ;
#4328=EDGE_CURVE ( 'NONE', #14909, #59342, #39964, .T. ) ;
#4329=FACE_BOUND ( 'NONE', #40938, .T. ) ;
#4331=DIRECTION ( 'NONE',  ( 0.000000000000000000, 0.1740410799127614649, 0.9847383929261618318 ) ) ;
#4335=VERTEX_POINT ( 'NONE', #35294 ) ;
#4336=EDGE_LOOP ( 'NONE', ( #48501, #2751, #32442, #57647, #9148, #13174 ) ) ;
#4338=ORIENTED_EDGE ( 'NONE', *, *, #40602, .F. ) ;
#4342=ORIENTED_EDGE ( 'NONE', *, *, #40179, .T. ) ;
#4344=DIRECTION ( 'NONE',  ( 1.000000000000000000, -0.000000000000000000, -0.000000000000000000 ) ) ;
#4346=CIRCLE ( 'NONE', #62745, 4.999999999999997335 ) ;
#4348=CYLINDRICAL_SURFACE ( 'NONE', #13252, 5.000000000000000888 ) ;
#4352=AXIS2_PLACEMENT_3D ( 'NONE', #30337, #44974, #60927 ) ;
#4353=ADVANCED_FACE ( 'NONE', ( #9361 ), #34951, .T. ) ;
#4354=ORIENTED_EDGE ( 'NONE', *, *, #29039, .T. ) ;
#4355=DIRECTION ( 'NONE',  ( 0.000000000000000000, 0.2618041379715635442, -0.9651210252299794456 ) ) ;
#4356=DIRECTION ( 'NONE',  ( -1.000000000000000000, 0.000000000000000000, 0.000000000000000000 ) ) ;
#4360=DIRECTION ( 'NONE',  ( -1.000000000000000000, 0.000000000000000000, -0.000000000000000000 ) ) ;
#4361=VECTOR ( 'NONE', #36884, 1000.000000000000000 ) ;
#4365=CARTESIAN_POINT ( 'NONE',  ( -35.00000000000000000, 9.196955404009424129, -8.830544224262844466 ) ) ;
#4366=CIRCLE ( 'NONE', #40455, 12.74999999999999822 ) ;
#4367=ORIENTED_EDGE ( 'NONE', *, *, #42678, .T. ) ;
#4369=CARTESIAN_POINT ( 'NONE',  ( -18.49080574448724690, -13.49999999999999822, -2.827202046691532642E-15 ) ) ;
#4373=DIRECTION ( 'NONE',  ( 1.000000000000000000, 0.000000000000000000, 0.000000000000000000 ) ) ;
#4374=EDGE_CURVE ( 'NONE', #29266, #41816, #65240, .T. ) ;
#4375=EDGE_CURVE ( 'NONE', #32447, #1539, #51403, .T. ) ;
#4376=ORIENTED_EDGE ( 'NONE', *, *, #22938, .F. ) ;
#4377=DIRECTION ( 'NONE',  ( 0.000000000000000000, -0.3807014730195086849, 0.9246979985058776386 ) ) ;
#4378=CARTESIAN_POINT ( 'NONE',  ( -37.00000000000000711, 12.73293890771483383, 0.6593684648220944355 ) ) ;
#4379=DIRECTION ( 'NONE',  ( 1.000000000000000000, 0.000000000000000000, 0.000000000000000000 ) ) ;
#4380=EDGE_CURVE ( 'NONE', #50839, #65109, #44958, .T. ) ;
#4381=CIRCLE ( 'NONE', #51076, 5.000000000000000888 ) ;
#4382=AXIS2_PLACEMENT_3D ( 'NONE', #42780, #16865, #33138 ) ;
#4385=CIRCLE ( 'NONE', #25583, 12.18650000000000055 ) ;
#4388=CARTESIAN_POINT ( 'NONE',  ( -35.00000000000000000, 6.946017217729938409, 10.01317267707888981 ) ) ;
#4392=AXIS2_PLACEMENT_3D ( 'NONE', #32326, #17383, #52640 ) ;
#4393=ORIENTED_EDGE ( 'NONE', *, *, #59501, .T. ) ;
#4394=DIRECTION ( 'NONE',  ( 1.000000000000000000, 0.000000000000000000, -0.000000000000000000 ) ) ;
#4396=VERTEX_POINT ( 'NONE', #55260 ) ;
#4397=CYLINDRICAL_SURFACE ( 'NONE', #60769, 12.75000000000000178 ) ;
#4399=DIRECTION ( 'NONE',  ( -0.000000000000000000, -1.000000000000000000, -0.000000000000000000 ) ) ;
#4401=ORIENTED_EDGE ( 'NONE', *, *, #22350, .F. ) ;
#4404=ORIENTED_EDGE ( 'NONE', *, *, #2267, .F. ) ;
#4407=CARTESIAN_POINT ( 'NONE',  ( -35.00000000000000000, 8.534258022646220354, -8.699265615722891809 ) ) ;
#4408=VERTEX_POINT ( 'NONE', #40952 ) ;
#4410=CARTESIAN_POINT ( 'NONE',  ( 37.00000000000000711, -3.640372113593465464, 12.21925492305365246 ) ) ;
#4412=VECTOR ( 'NONE', #5321, 1000.000000000000000 ) ;
#4413=DIRECTION ( 'NONE',  ( 1.000000000000000000, 0.000000000000000000, 0.000000000000000000 ) ) ;
#4415=FACE_OUTER_BOUND ( 'NONE', #6021, .T. ) ;
#4418=EDGE_LOOP ( 'NONE', ( #11730, #60237, #23705, #42193 ) ) ;
#4420=ORIENTED_EDGE ( 'NONE', *, *, #48613, .F. ) ;
#4421=CARTESIAN_POINT ( 'NONE',  ( 35.00000000000000000, 4.705694406421931860E-17, -3.469127814946512892E-15 ) ) ;
#4422=ORIENTED_EDGE ( 'NONE', *, *, #32105, .T. ) ;
#4425=CARTESIAN_POINT ( 'NONE',  ( -19.69476066079020171, -4.201994156881551312, 25.00000000000000000 ) ) ;
#4426=DIRECTION ( 'NONE',  ( 0.000000000000000000, 0.01356324068817998940, -0.9999080150203990547 ) ) ;
#4428=VECTOR ( 'NONE', #37054, 1000.000000000000000 ) ;
#4429=CARTESIAN_POINT ( 'NONE',  ( -35.00000000000000000, 2.250029553613936528, -12.54989509947648862 ) ) ;
#4432=DIRECTION ( 'NONE',  ( -1.000000000000000000, -0.000000000000000000, 0.000000000000000000 ) ) ;
#4434=DIRECTION ( 'NONE',  ( -1.000000000000000000, 0.000000000000000000, 0.000000000000000000 ) ) ;
#4435=ORIENTED_EDGE ( 'NONE', *, *, #19827, .T. ) ;
#4436=ADVANCED_FACE ( 'NONE', ( #6702 ), #51608, .T. ) ;
#4438=CARTESIAN_POINT ( 'NONE',  ( -35.00000000000000000, 0.000000000000000000, 0.000000000000000000 ) ) ;
#4439=ORIENTED_EDGE ( 'NONE', *, *, #58564, .F. ) ;
#4440=EDGE_CURVE ( 'NONE', #40547, #21398, #61861, .T. ) ;
#4441=ORIENTED_EDGE ( 'NONE', *, *, #528, .F. ) ;
#4442=DIRECTION ( 'NONE',  ( 1.000000000000000000, 0.000000000000000000, 0.000000000000000000 ) ) ;
#4443=CARTESIAN_POINT ( 'NONE',  ( 35.00000000000000000, 4.705694406421931860E-17, -3.469127814946512892E-15 ) ) ;
#4445=DIRECTION ( 'NONE',  ( -1.000000000000000000, -0.000000000000000000, -0.000000000000000000 ) ) ;
#4448=CARTESIAN_POINT ( 'NONE',  ( -35.00000000000000000, -11.29812557209474733, -3.213188559034363401 ) ) ;
#4450=FACE_OUTER_BOUND ( 'NONE', #6377, .T. ) ;
#4453=FACE_OUTER_BOUND ( 'NONE', #29006, .T. ) ;
#4454=AXIS2_PLACEMENT_3D ( 'NONE', #41269, #29654, #30331 ) ;
#4455=CARTESIAN_POINT ( 'NONE',  ( -19.47984447937493613, -3.750539801530005768, 11.39883551934753925 ) ) ;
#4456=CARTESIAN_POINT ( 'NONE',  ( -18.89779455570165467, -4.072785471668618484, 12.87288005866979290 ) ) ;
#4458=EDGE_CURVE ( 'NONE', #40836, #31528, #20424, .T. ) ;
#4459=ORIENTED_EDGE ( 'NONE', *, *, #15976, .F. ) ;
#4461=CIRCLE ( 'NONE', #19315, 5.000000000000000000 ) ;
#4462=CARTESIAN_POINT ( 'NONE',  ( -4.989057617119008192, -0.9162120371760335003, 13.46887357958837406 ) ) ;
#4463=B_SPLINE_CURVE_WITH_KNOTS ( 'NONE', 3,
 ( #4140, #24406, #9768, #44674, #34052, #39706, #24752, #55327, #65302, #14424, #35363, #30386, #19769, #40027, #60313, #50680, #35686, #57892 ),
 .UNSPECIFIED., .F., .F.,
 ( 4, 2, 2, 2, 2, 2, 2, 2, 4 ),
 ( 0.004907007814975161697, 0.005737531593967190244, 0.006568055372959219658, 0.007398579151951248205, 0.008229102930943277619, 0.009059626709935306166, 0.009890150488927336447, 0.01072067426791936673, 0.01155119804691139528 ),
 .UNSPECIFIED. ) ;
#4464=CARTESIAN_POINT ( 'NONE',  ( 35.00000000000000000, -11.29812557209478996, -3.213188559034203529 ) ) ;
#4466=ORIENTED_EDGE ( 'NONE', *, *, #37652, .T. ) ;
#4470=AXIS2_PLACEMENT_3D ( 'NONE', #38398, #32089, #53385 ) ;
#4472=AXIS2_PLACEMENT_3D ( 'NONE', #53703, #8137, #7461 ) ;
#4473=CARTESIAN_POINT ( 'NONE',  ( 37.00000000000000711, 7.251710744571704836, 9.240395740215555875 ) ) ;
#4474=DIRECTION ( 'NONE',  ( -1.000000000000000000, 0.000000000000000000, -0.000000000000000000 ) ) ;
#4476=ORIENTED_EDGE ( 'NONE', *, *, #14771, .T. ) ;
#4479=LINE ( 'NONE', #60311, #15893 ) ;
#4481=CARTESIAN_POINT ( 'NONE',  ( -27.45775109278351067, 11.83395752356219077, -1.989333891161980894 ) ) ;
#4483=ORIENTED_EDGE ( 'NONE', *, *, #33472, .T. ) ;
#4484=EDGE_CURVE ( 'NONE', #44370, #29968, #21320, .T. ) ;
#4486=ORIENTED_EDGE ( 'NONE', *, *, #8419, .F. ) ;
#4487=AXIS2_PLACEMENT_3D ( 'NONE', #18748, #39005, #29357 ) ;
#4488=ADVANCED_FACE ( 'NONE', ( #31614 ), #42231, .T. ) ;
#4490=ORIENTED_EDGE ( 'NONE', *, *, #16136, .F. ) ;
#4491=AXIS2_PLACEMENT_3D ( 'NONE', #5448, #52312, #27026 ) ;
#4494=FACE_OUTER_BOUND ( 'NONE', #12581, .T. ) ;
#4495=CARTESIAN_POINT ( 'NONE',  ( 6.361445718264521432, -4.355102044641763648, 11.18181944858514498 ) ) ;
#4497=CARTESIAN_POINT ( 'NONE',  ( 11.86852745065355741, -10.64790170674533165, -8.300198448557058128 ) ) ;
#4498=CYLINDRICAL_SURFACE ( 'NONE', #19180, 5.000000000000000888 ) ;
#4499=ORIENTED_EDGE ( 'NONE', *, *, #26117, .F. ) ;
#4500=LINE ( 'NONE', #34411, #55403 ) ;
#4501=ORIENTED_EDGE ( 'NONE', *, *, #45939, .T. ) ;
#4502=DIRECTION ( 'NONE',  ( -0.000000000000000000, -1.000000000000000000, -0.000000000000000000 ) ) ;
#4503=ORIENTED_EDGE ( 'NONE', *, *, #18439, .F. ) ;
#4504=ORIENTED_EDGE ( 'NONE', *, *, #55773, .F. ) ;
#4507=CARTESIAN_POINT ( 'NONE',  ( -35.00000000000000000, -8.389074212634351824, 8.839356091080015076 ) ) ;
#4508=ADVANCED_FACE ( 'NONE', ( #41602 ), #51280, .T. ) ;
#4509=CARTESIAN_POINT ( 'NONE',  ( -47.00000000000000711, 0.000000000000000000, 0.000000000000000000 ) ) ;
#4510=FACE_OUTER_BOUND ( 'NONE', #38978, .T. ) ;
#4511=CARTESIAN_POINT ( 'NONE',  ( 35.00000000000000000, 8.839356091080166067, 8.389074212634184846 ) ) ;
#4513=AXIS2_PLACEMENT_3D ( 'NONE', #54156, #29516, #49819 ) ;
#4514=EDGE_CURVE ( 'NONE', #33155, #16289, #45924, .T. ) ;
#4516=DIRECTION ( 'NONE',  ( -1.000000000000000000, 0.000000000000000000, 0.000000000000000000 ) ) ;
#4517=ORIENTED_EDGE ( 'NONE', *, *, #18521, .T. ) ;
#4518=EDGE_CURVE ( 'NONE', #17303, #7978, #57612, .T. ) ;
#4520=DIRECTION ( 'NONE',  ( 1.000000000000000000, 0.000000000000000000, 0.000000000000000000 ) ) ;
#4521=VECTOR ( 'NONE', #54462, 1000.000000000000000 ) ;
#4523=CARTESIAN_POINT ( 'NONE',  ( 18.78313359089984402, -1.065647145831489118, 12.00131809889008316 ) ) ;
#4525=CIRCLE ( 'NONE', #15125, 5.000000000000000888 ) ;
#4526=FACE_OUTER_BOUND ( 'NONE', #52474, .T. ) ;
#4527=VECTOR ( 'NONE', #24748, 1000.000000000000000 ) ;
#4530=ORIENTED_EDGE ( 'NONE', *, *, #8419, .T. ) ;
#4531=ADVANCED_FACE ( 'NONE', ( #62210 ), #15658, .T. ) ;
#4532=VERTEX_POINT ( 'NONE', #37263 ) ;
#4533=DIRECTION ( 'NONE',  ( -1.000000000000000000, 0.000000000000000000, 0.000000000000000000 ) ) ;
#4534=DIRECTION ( 'NONE',  ( -0.5446691071471760903, 0.8386510381079236298, 0.000000000000000000 ) ) ;
#4535=DIRECTION ( 'NONE',  ( -1.000000000000000000, 0.000000000000000000, 0.000000000000000000 ) ) ;
#4538=CARTESIAN_POINT ( 'NONE',  ( -35.00000000000000000, 0.000000000000000000, 0.000000000000000000 ) ) ;
#4539=CARTESIAN_POINT ( 'NONE',  ( -28.08328025583519860, 11.67727086453252028, -6.780915823467608128 ) ) ;
#4541=VECTOR ( 'NONE', #11345, 1000.000000000000000 ) ;
#4542=CARTESIAN_POINT ( 'NONE',  ( 7.298320481653675529, -6.062943420091013280, -12.06387388335232735 ) ) ;
#4543=LINE ( 'NONE', #18841, #9890 ) ;
#4544=AXIS2_PLACEMENT_3D ( 'NONE', #51548, #15920, #17259 ) ;
#4545=DIRECTION ( 'NONE',  ( 0.000000000000000000, 0.9903235168508555120, 0.1387779952735782862 ) ) ;
#4546=CARTESIAN_POINT ( 'NONE',  ( 3.455388140186490986, 8.284410676190358203, 8.681632586536974117 ) ) ;
#4549=CARTESIAN_POINT ( 'NONE',  ( 22.78424990826529495, -4.691658877507584258, -11.04575192261954264 ) ) ;
#4550=CARTESIAN_POINT ( 'NONE',  ( 22.36482863261543486, 11.96441317219527889, -0.9234811557364158707 ) ) ;
#4554=ORIENTED_EDGE ( 'NONE', *, *, #34292, .T. ) ;
#4555=CARTESIAN_POINT ( 'NONE',  ( 35.00000000000000000, 4.705694406421931860E-17, -3.469127814946512892E-15 ) ) ;
#4558=EDGE_LOOP ( 'NONE', ( #23336, #42826, #32160, #14044 ) ) ;
#4559=CARTESIAN_POINT ( 'NONE',  ( -27.01437459610461644, -11.79277645698183186, -2.220455681983952267 ) ) ;
#4560=CARTESIAN_POINT ( 'NONE',  ( -35.00000000000000000, -10.63508530065525370, 4.986700593229667078 ) ) ;
#4561=AXIS2_PLACEMENT_3D ( 'NONE', #35012, #4135, #14419 ) ;
#4565=VECTOR ( 'NONE', #57791, 1000.000000000000000 ) ;
#4566=ADVANCED_FACE ( 'NONE', ( #57574 ), #724, .T. ) ;
#4570=FACE_OUTER_BOUND ( 'NONE', #20764, .T. ) ;
#4572=CARTESIAN_POINT ( 'NONE',  ( -14.24546914926061625, 8.298873997449982554, -10.64811974057628952 ) ) ;
#4574=DIRECTION ( 'NONE',  ( 1.000000000000000000, 0.000000000000000000, 0.000000000000000000 ) ) ;
#4575=CYLINDRICAL_SURFACE ( 'NONE', #502, 12.18649999999999878 ) ;
#4576=DIRECTION ( 'NONE',  ( 1.000000000000000000, 0.000000000000000000, -0.000000000000000000 ) ) ;
#4578=ORIENTED_EDGE ( 'NONE', *, *, #54969, .T. ) ;
#4580=VECTOR ( 'NONE', #46393, 1000.000000000000000 ) ;
#4581=ORIENTED_EDGE ( 'NONE', *, *, #45464, .F. ) ;
#4582=VECTOR ( 'NONE', #58203, 1000.000000000000000 ) ;
#4583=CARTESIAN_POINT ( 'NONE',  ( -37.00000000000000711, 0.000000000000000000, 0.000000000000000000 ) ) ;
#4584=ADVANCED_FACE ( 'NONE', ( #11665 ), #31939, .T. ) ;
#4585=CARTESIAN_POINT ( 'NONE',  ( -37.00000000000000711, 5.710938531231712467, 11.39945968423473666 ) ) ;
#4588=CARTESIAN_POINT ( 'NONE',  ( 11.05611852032334319, 11.87696910296720532, -1.718393329984558626 ) ) ;
#4590=CARTESIAN_POINT ( 'NONE',  ( 29.51976981715666781, 7.690765383426390045, 11.09513982864076276 ) ) ;
#4592=ORIENTED_EDGE ( 'NONE', *, *, #9241, .T. ) ;
#4593=AXIS2_PLACEMENT_3D ( 'NONE', #54405, #40644, #50642 ) ;
#4594=ORIENTED_EDGE ( 'NONE', *, *, #38046, .T. ) ;
#4595=CYLINDRICAL_SURFACE ( 'NONE', #36371, 12.18650000000000055 ) ;
#4596=EDGE_CURVE ( 'NONE', #2241, #43998, #40645, .T. ) ;
#4597=ORIENTED_EDGE ( 'NONE', *, *, #62553, .T. ) ;
#4599=ORIENTED_EDGE ( 'NONE', *, *, #16761, .F. ) ;
#4604=VECTOR ( 'NONE', #36065, 1000.000000000000000 ) ;
#4606=ORIENTED_EDGE ( 'NONE', *, *, #27251, .T. ) ;
#4608=EDGE_CURVE ( 'NONE', #52575, #33456, #43904, .T. ) ;
#4609=DIRECTION ( 'NONE',  ( 1.000000000000000000, 0.000000000000000000, 0.000000000000000000 ) ) ;
#4610=CARTESIAN_POINT ( 'NONE',  ( 35.00000000000000000, 4.705694406421931860E-17, -3.469127814946512892E-15 ) ) ;
#4611=EDGE_CURVE ( 'NONE', #56955, #27835, #33912, .T. ) ;
#4612=DIRECTION ( 'NONE',  ( 0.000000000000000000, 0.01356324068817992175, -0.9999080150203990547 ) ) ;
#4613=CIRCLE ( 'NONE', #23691, 4.999999999999999112 ) ;
#4617=CARTESIAN_POINT ( 'NONE',  ( 35.00000000000000000, 4.705694406421931860E-17, -3.469127814946512892E-15 ) ) ;
#4619=CARTESIAN_POINT ( 'NONE',  ( 37.00000000000000711, -9.821084925794620446, -7.215058775251224077 ) ) ;
#4622=AXIS2_PLACEMENT_3D ( 'NONE', #25238, #65776, #55839 ) ;
#4626=ORIENTED_EDGE ( 'NONE', *, *, #58715, .F. ) ;
#4627=CARTESIAN_POINT ( 'NONE',  ( -2.532614230583022152, -11.30437021680553222, 4.026315189028233377 ) ) ;
#4630=AXIS2_PLACEMENT_3D ( 'NONE', #7361, #18694, #43266 ) ;
#4631=EDGE_CURVE ( 'NONE', #7848, #53238, #47914, .T. ) ;
#4634=ORIENTED_EDGE ( 'NONE', *, *, #47403, .T. ) ;
#4637=CARTESIAN_POINT ( 'NONE',  ( 10.09892164510067580, 1.646990700008696518, 11.88792003737877145 ) ) ;
#4638=CARTESIAN_POINT ( 'NONE',  ( 35.00000000000000000, -11.60979404548631777, 3.704519465651427534 ) ) ;
#4639=CARTESIAN_POINT ( 'NONE',  ( 35.00000000000000000, -8.352657516904727686, -8.258652103341406203 ) ) ;
#4640=CIRCLE ( 'NONE', #20573, 12.18650000000000055 ) ;
#4643=ORIENTED_EDGE ( 'NONE', *, *, #11728, .F. ) ;
#4644=DIRECTION ( 'NONE',  ( 1.000000000000000000, 0.000000000000000000, -0.000000000000000000 ) ) ;
#4645=CYLINDRICAL_SURFACE ( 'NONE', #28870, 12.74999999999999822 ) ;
#4646=CARTESIAN_POINT ( 'NONE',  ( 10.75853767213705225, 7.830989516993144051, -9.092612561015865680 ) ) ;
#4647=DIRECTION ( 'NONE',  ( 1.000000000000000000, 0.000000000000000000, 0.000000000000000000 ) ) ;
#4648=EDGE_CURVE ( 'NONE', #63364, #64117, #22649, .T. ) ;
#4649=CIRCLE ( 'NONE', #57767, 4.999999999999999112 ) ;
#4650=ORIENTED_EDGE ( 'NONE', *, *, #10647, .T. ) ;
#4651=VERTEX_POINT ( 'NONE', #4674 ) ;
#4653=ORIENTED_EDGE ( 'NONE', *, *, #44835, .T. ) ;
#4654=DIRECTION ( 'NONE',  ( 0.000000000000000000, 0.01356324068817998940, -0.9999080150203989437 ) ) ;
#4655=CARTESIAN_POINT ( 'NONE',  ( 35.00000000000000000, -7.717887834988180984, 8.854740511458926377 ) ) ;
#4660=CARTESIAN_POINT ( 'NONE',  ( 12.93723047338301058, 4.476360154859203355, 25.00000000000000000 ) ) ;
#4661=VERTEX_POINT ( 'NONE', #64813 ) ;
#4662=AXIS2_PLACEMENT_3D ( 'NONE', #49038, #24983, #61205 ) ;
#4663=ADVANCED_FACE ( 'NONE', ( #35553 ), #64494, .T. ) ;
#4664=AXIS2_PLACEMENT_3D ( 'NONE', #50708, #62614, #17423 ) ;
#4666=ORIENTED_EDGE ( 'NONE', *, *, #6181, .T. ) ;
#4667=ORIENTED_EDGE ( 'NONE', *, *, #13485, .F. ) ;
#4668=B_SPLINE_CURVE_WITH_KNOTS ( 'NONE', 3,
 ( #59740, #59102, #33491, #24821, #50097, #54762, #3244, #19510, #53782, #23515, #13829, #8216, #4207, #39779 ),
 .UNSPECIFIED., .F., .F.,
 ( 4, 2, 2, 2, 2, 2, 4 ),
 ( 2.453269466693398698E-18, 0.001897844907058980971, 0.002846767360588470155, 0.003795689814117958905, 0.004744612267647447222, 0.005693534721176935973, 0.007591379628235916943 ),
 .UNSPECIFIED. ) ;
#4669=CYLINDRICAL_SURFACE ( 'NONE', #43627, 5.000000000000000888 ) ;
#4670=VECTOR ( 'NONE', #9499, 1000.000000000000000 ) ;
#4673=ORIENTED_EDGE ( 'NONE', *, *, #2867, .F. ) ;
#4674=CARTESIAN_POINT ( 'NONE',  ( 35.00000000000000000, -10.64792938439759595, -5.927257550915285833 ) ) ;
#4675=ORIENTED_EDGE ( 'NONE', *, *, #44741, .T. ) ;
#4677=DIRECTION ( 'NONE',  ( 0.000000000000000000, 0.01356324068817998940, -0.9999080150203990547 ) ) ;
#4679=CARTESIAN_POINT ( 'NONE',  ( 37.00000000000000711, -10.42955799785315563, 6.303578524887051948 ) ) ;
#4682=CIRCLE ( 'NONE', #25879, 12.18650000000000055 ) ;
#4683=ORIENTED_EDGE ( 'NONE', *, *, #28314, .T. ) ;
#4684=DIRECTION ( 'NONE',  ( 1.000000000000000000, -0.000000000000000000, -0.000000000000000000 ) ) ;
#4686=VERTEX_POINT ( 'NONE', #18963 ) ;
#4689=AXIS2_PLACEMENT_3D ( 'NONE', #5191, #25458, #10482 ) ;
#4691=ORIENTED_EDGE ( 'NONE', *, *, #26416, .F. ) ;
#4692=DIRECTION ( 'NONE',  ( 0.000000000000000000, 0.1740410799127614649, 0.9847383929261618318 ) ) ;
#4693=AXIS2_PLACEMENT_3D ( 'NONE', #9779, #45040, #8814 ) ;
#4695=CYLINDRICAL_SURFACE ( 'NONE', #56360, 4.999999999999999112 ) ;
#4699=VERTEX_POINT ( 'NONE', #59524 ) ;
#4700=( BOUNDED_CURVE ( )  B_SPLINE_CURVE ( 3, ( #4204, #54757, #49455, #64694 ),
 .UNSPECIFIED., .F., .F. ) 
 B_SPLINE_CURVE_WITH_KNOTS ( ( 4, 4 ),
 ( 1.625261828949994269, 1.639255800632265947 ),
 .UNSPECIFIED. ) 
 CURVE ( )  GEOMETRIC_REPRESENTATION_ITEM ( )  RATIONAL_B_SPLINE_CURVE ( ( 1.000000000000000000, 0.9999836807962925178, 0.9999836807962925178, 1.000000000000000000 ) ) 
 REPRESENTATION_ITEM ( '' )  );
#4701=CARTESIAN_POINT ( 'NONE',  ( -17.54726996257253191, -11.36053454945672136, 3.865003848717349033 ) ) ;
#4702=AXIS2_PLACEMENT_3D ( 'NONE', #25511, #25188, #19565 ) ;
#4704=ORIENTED_EDGE ( 'NONE', *, *, #37989, .F. ) ;
#4705=FACE_OUTER_BOUND ( 'NONE', #19790, .T. ) ;
#4708=EDGE_CURVE ( 'NONE', #50294, #34584, #15140, .T. ) ;
#4710=VERTEX_POINT ( 'NONE', #60171 ) ;
#4711=DIRECTION ( 'NONE',  ( 0.000000000000000000, -0.07632122047555053856, 0.9970832820307050648 ) ) ;
#4712=EDGE_CURVE ( 'NONE', #9845, #13243, #33189, .T. ) ;
#4717=EDGE_CURVE ( 'NONE', #49616, #16668, #23671, .T. ) ;
#4719=DIRECTION ( 'NONE',  ( 0.000000000000000000, 0.01356324068817998940, -0.9999080150203989437 ) ) ;
#4720=ORIENTED_EDGE ( 'NONE', *, *, #65519, .F. ) ;
#4721=AXIS2_PLACEMENT_3D ( 'NONE', #63337, #53387, #36771 ) ;
#4724=CARTESIAN_POINT ( 'NONE',  ( 35.00000000000000000, -5.300372733891561161, 11.59605747147791632 ) ) ;
#4725=CARTESIAN_POINT ( 'NONE',  ( -37.00000000000000711, 0.000000000000000000, 0.000000000000000000 ) ) ;
#4726=DIRECTION ( 'NONE',  ( 0.000000000000000000, 0.01356324068817998940, -0.9999080150203989437 ) ) ;
#4730=DIRECTION ( 'NONE',  ( 1.000000000000000000, 0.000000000000000000, 0.000000000000000000 ) ) ;
#4733=CIRCLE ( 'NONE', #25940, 12.18649999999999878 ) ;
#4734=ADVANCED_FACE ( 'NONE', ( #34566, #44534, #40200, #54863, #60834, #44223, #9286, #49878, #19292, #55181, #4329, #54554, #39560, #24601, #8984, #44879, #4988 ), #59863, .T. ) ;
#4735=ORIENTED_EDGE ( 'NONE', *, *, #43142, .T. ) ;
#4737=ADVANCED_FACE ( 'NONE', ( #14593 ), #45522, .T. ) ;
#4739=CYLINDRICAL_SURFACE ( 'NONE', #14051, 4.999999999999999112 ) ;
#4740=DIRECTION ( 'NONE',  ( 0.000000000000000000, 0.9987865678893278476, -0.04924826701374234589 ) ) ;
#4742=VECTOR ( 'NONE', #46053, 1000.000000000000000 ) ;
#4744=EDGE_CURVE ( 'NONE', #58586, #47206, #35216, .T. ) ;
#4745=ORIENTED_EDGE ( 'NONE', *, *, #49036, .T. ) ;
#4746=ORIENTED_EDGE ( 'NONE', *, *, #52842, .F. ) ;
#4747=CARTESIAN_POINT ( 'NONE',  ( -35.00000000000000000, -1.262958560998674429, -12.12087942037211086 ) ) ;
#4749=ORIENTED_EDGE ( 'NONE', *, *, #36121, .T. ) ;
#4751=DIRECTION ( 'NONE',  ( 1.000000000000000000, 0.000000000000000000, -0.000000000000000000 ) ) ;
#4756=DIRECTION ( 'NONE',  ( 1.000000000000000000, 0.000000000000000000, -0.000000000000000000 ) ) ;
#4758=ORIENTED_EDGE ( 'NONE', *, *, #29791, .F. ) ;
#4759=DIRECTION ( 'NONE',  ( 0.000000000000000000, -0.01356324068817998940, 0.9999080150203990547 ) ) ;
#4762=ORIENTED_EDGE ( 'NONE', *, *, #32702, .F. ) ;
#4763=AXIS2_PLACEMENT_3D ( 'NONE', #46667, #17735, #16425 ) ;
#4766=DIRECTION ( 'NONE',  ( -1.000000000000000000, 0.000000000000000000, -0.000000000000000000 ) ) ;
#4768=ADVANCED_FACE ( 'NONE', ( #30556, #50859 ), #27791, .F. ) ;
#4771=CARTESIAN_POINT ( 'NONE',  ( -26.97057981164311968, -10.82588076752199768, 5.177076099659926989 ) ) ;
#4773=LINE ( 'NONE', #30988, #26606 ) ;
#4775=CYLINDRICAL_SURFACE ( 'NONE', #41738, 8.049672981451799103 ) ;
#4776=CARTESIAN_POINT ( 'NONE',  ( 12.90763733317001538, 13.13803547055557175, -3.111388515484440731 ) ) ;
#4779=CARTESIAN_POINT ( 'NONE',  ( 13.40087876459804050, -12.56852956566119239, -4.932660016159226224 ) ) ;
#4780=VERTEX_POINT ( 'NONE', #32437 ) ;
#4781=ORIENTED_EDGE ( 'NONE', *, *, #60447, .T. ) ;
#4782=DIRECTION ( 'NONE',  ( 0.000000000000000000, 0.9551603052523468529, -0.2960891610144544828 ) ) ;
#4783=DIRECTION ( 'NONE',  ( -1.000000000000000000, -0.000000000000000000, 0.000000000000000000 ) ) ;
#4785=CARTESIAN_POINT ( 'NONE',  ( 35.00000000000000000, -1.791059740004336875, 12.05416472667166694 ) ) ;
#4787=CIRCLE ( 'NONE', #56804, 5.000000000000001776 ) ;
#4788=CARTESIAN_POINT ( 'NONE',  ( -17.29244623348158783, 2.525873743887551814, 25.00000000000000000 ) ) ;
#4789=FACE_OUTER_BOUND ( 'NONE', #36677, .T. ) ;
#4791=ORIENTED_EDGE ( 'NONE', *, *, #65136, .T. ) ;
#4793=CARTESIAN_POINT ( 'NONE',  ( 35.00000000000000000, -0.8294751490778421443, 12.15823808070322976 ) ) ;
#4796=CIRCLE ( 'NONE', #52587, 5.000000000000002665 ) ;
#4798=LINE ( 'NONE', #45332, #37363 ) ;
#4799=CARTESIAN_POINT ( 'NONE',  ( -35.00000000000000000, 1.456211999474342766, 11.65554240571057854 ) ) ;
#4800=EDGE_LOOP ( 'NONE', ( #40724, #32651, #1782, #54523 ) ) ;
#4802=CIRCLE ( 'NONE', #29186, 5.000000000000000000 ) ;
#4804=CARTESIAN_POINT ( 'NONE',  ( 35.00000000000000000, 4.705694406421931860E-17, -3.469127814946512892E-15 ) ) ;
#4805=FACE_OUTER_BOUND ( 'NONE', #17669, .T. ) ;
#4808=CIRCLE ( 'NONE', #29239, 4.999999999999999112 ) ;
#4809=ORIENTED_EDGE ( 'NONE', *, *, #29158, .T. ) ;
#4812=ORIENTED_EDGE ( 'NONE', *, *, #41396, .F. ) ;
#4813=CARTESIAN_POINT ( 'NONE',  ( 21.48709468929590827, 12.93615662171536584, -3.881105879424552985 ) ) ;
#4818=AXIS2_PLACEMENT_3D ( 'NONE', #18735, #59609, #38327 ) ;
#4819=ADVANCED_FACE ( 'NONE', ( #32035 ), #47360, .T. ) ;
#4821=CARTESIAN_POINT ( 'NONE',  ( 37.00000000000000711, -7.215058775251181444, 9.821084925794645315 ) ) ;
#4823=CARTESIAN_POINT ( 'NONE',  ( -37.00000000000000711, -2.865935305911713638, 12.42372387097881514 ) ) ;
#4824=CARTESIAN_POINT ( 'NONE',  ( -35.00000000000000000, 1.456211999474342766, 11.65554240571057854 ) ) ;
#4828=ORIENTED_EDGE ( 'NONE', *, *, #18900, .T. ) ;
#4829=CARTESIAN_POINT ( 'NONE',  ( 12.52750123246316072, 0.4973700281276248192, 25.00000000000000000 ) ) ;
#4831=ORIENTED_EDGE ( 'NONE', *, *, #65276, .F. ) ;
#4832=LINE ( 'NONE', #25098, #11495 ) ;
#4835=DIRECTION ( 'NONE',  ( 0.000000000000000000, -0.8515178078024923103, 0.5243256840888473880 ) ) ;
#4838=CARTESIAN_POINT ( 'NONE',  ( -10.48620311856347875, -9.720786832536937538, 25.00000000000000000 ) ) ;
#4839=AXIS2_PLACEMENT_3D ( 'NONE', #60211, #15628, #50584 ) ;
#4840=CARTESIAN_POINT ( 'NONE',  ( -37.00000000000000711, -10.84030624090602046, -6.711949091238257559 ) ) ;
#4841=CARTESIAN_POINT ( 'NONE',  ( -19.31276997470573775, 11.98635249372530254, -0.6547996305031958952 ) ) ;
#4844=ORIENTED_EDGE ( 'NONE', *, *, #28406, .T. ) ;
#4845=CARTESIAN_POINT ( 'NONE',  ( -37.00000000000000711, -1.456211999474261054, -11.65554240571058742 ) ) ;
#4846=VERTEX_POINT ( 'NONE', #1141 ) ;
#4848=CARTESIAN_POINT ( 'NONE',  ( 35.00000000000000000, 4.705694406421931860E-17, -3.469127814946512892E-15 ) ) ;
#4851=CARTESIAN_POINT ( 'NONE',  ( -37.00000000000000711, 11.72397916322013600, -0.7214809346827312231 ) ) ;
#4852=DIRECTION ( 'NONE',  ( 0.000000000000000000, -0.01356324068818000848, 0.9999080150203990547 ) ) ;
#4853=EDGE_CURVE ( 'NONE', #36886, #17119, #18361, .T. ) ;
#4854=CARTESIAN_POINT ( 'NONE',  ( -10.70196691523763732, -4.522197807754633203, -11.12215661015785884 ) ) ;
#4855=CARTESIAN_POINT ( 'NONE',  ( -37.00000000000000711, 0.7214809346828596759, 11.72397916322012712 ) ) ;
#4856=ORIENTED_EDGE ( 'NONE', *, *, #16070, .F. ) ;
#4857=ORIENTED_EDGE ( 'NONE', *, *, #16047, .T. ) ;
#4858=DIRECTION ( 'NONE',  ( 0.000000000000000000, -0.01356324068817999114, 0.9999080150203989437 ) ) ;
#4861=AXIS2_PLACEMENT_3D ( 'NONE', #50051, #14448, #49088 ) ;
#4862=ADVANCED_FACE ( 'NONE', ( #62613 ), #57326, .T. ) ;
#4863=DIRECTION ( 'NONE',  ( 0.000000000000000000, 0.2960891610144510966, 0.9551603052523478521 ) ) ;
#4866=DIRECTION ( 'NONE',  ( 1.000000000000000000, 0.000000000000000000, -0.000000000000000000 ) ) ;
#4867=CARTESIAN_POINT ( 'NONE',  ( -36.00000000000000711, -12.74921544981111055, 0.1414404973751696992 ) ) ;
#4869=ORIENTED_EDGE ( 'NONE', *, *, #14006, .T. ) ;
#4871=DIRECTION ( 'NONE',  ( 1.000000000000000000, 0.000000000000000000, 0.000000000000000000 ) ) ;
#4873=AXIS2_PLACEMENT_3D ( 'NONE', #15864, #6582, #56811 ) ;
#4876=EDGE_CURVE ( 'NONE', #20288, #27619, #52984, .T. ) ;
#4877=ORIENTED_EDGE ( 'NONE', *, *, #46840, .F. ) ;
#4878=CARTESIAN_POINT ( 'NONE',  ( 36.00000000000000711, -3.033604067594489528, 12.38385022362084698 ) ) ;
#4881=ORIENTED_EDGE ( 'NONE', *, *, #44741, .F. ) ;
#4882=EDGE_CURVE ( 'NONE', #36323, #56883, #55504, .T. ) ;
#4886=DIRECTION ( 'NONE',  ( -1.000000000000000000, 0.000000000000000000, 0.000000000000000000 ) ) ;
#4888=CYLINDRICAL_SURFACE ( 'NONE', #61784, 4.999999999999999112 ) ;
#4891=AXIS2_PLACEMENT_3D ( 'NONE', #24051, #23735, #33368 ) ;
#4892=DIRECTION ( 'NONE',  ( 0.000000000000000000, -0.5987040770935562195, 0.8009703041134254020 ) ) ;
#4893=VERTEX_POINT ( 'NONE', #17421 ) ;
#4894=CARTESIAN_POINT ( 'NONE',  ( -47.00000000000000711, 0.000000000000000000, 0.000000000000000000 ) ) ;
#4898=DIRECTION ( 'NONE',  ( 1.000000000000000000, 0.000000000000000000, 0.000000000000000000 ) ) ;
#4899=CARTESIAN_POINT ( 'NONE',  ( -35.00000000000000000, 9.493370459201697642, 6.917234959366862057 ) ) ;
#4900=CARTESIAN_POINT ( 'NONE',  ( -18.58686583997218378, 5.151216734910788908, 12.47858029384653555 ) ) ;
#4901=CARTESIAN_POINT ( 'NONE',  ( 27.62838931380291996, 25.00000000000000000, -3.066727421130092779 ) ) ;
#4902=EDGE_CURVE ( 'NONE', #29799, #21899, #44711, .T. ) ;
#4904=FACE_OUTER_BOUND ( 'NONE', #63253, .T. ) ;
#4906=B_SPLINE_CURVE_WITH_KNOTS ( 'NONE', 3,
 ( #10234, #40837, #55470, #55136, #30511, #44832, #4942, #5262, #25203, #14552, #282, #61113, #29857, #30200, #15548, #4627 ),
 .UNSPECIFIED., .F., .F.,
 ( 4, 2, 2, 2, 2, 2, 2, 4 ),
 ( 0.000000000000000000, 0.002440323270129363641, 0.003660484905194043726, 0.004880646540258723812, 0.006100808175323402596, 0.007320969810388081381, 0.008541131445452760165, 0.009761293080517437215 ),
 .UNSPECIFIED. ) ;
#4907=VECTOR ( 'NONE', #23737, 1000.000000000000000 ) ;
#4909=EDGE_CURVE ( 'NONE', #52455, #23780, #36220, .T. ) ;
#4910=CYLINDRICAL_SURFACE ( 'NONE', #62744, 7.011478057721953761 ) ;
#4911=VERTEX_POINT ( 'NONE', #37698 ) ;
#4912=FACE_OUTER_BOUND ( 'NONE', #11363, .T. ) ;
#4913=DIRECTION ( 'NONE',  ( 0.000000000000000000, -0.01356324068818000848, 0.9999080150203990547 ) ) ;
#4914=LINE ( 'NONE', #45448, #25503 ) ;
#4915=VERTEX_POINT ( 'NONE', #27705 ) ;
#4918=ORIENTED_EDGE ( 'NONE', *, *, #10334, .T. ) ;
#4924=DIRECTION ( 'NONE',  ( -1.000000000000000000, 0.000000000000000000, 0.000000000000000000 ) ) ;
#4928=CARTESIAN_POINT ( 'NONE',  ( -35.00000000000000000, 10.70999494708501132, -5.814360711498173018 ) ) ;
#4931=CARTESIAN_POINT ( 'NONE',  ( -2.532614230583026593, 7.965877694534055031, 10.89930238848911337 ) ) ;
#4932=DIRECTION ( 'NONE',  ( -1.000000000000000000, 0.000000000000000000, 0.000000000000000000 ) ) ;
#4933=CYLINDRICAL_SURFACE ( 'NONE', #3719, 5.000000000000000888 ) ;
#4936=ADVANCED_FACE ( 'NONE', ( #21421 ), #809, .T. ) ;
#4939=AXIS2_PLACEMENT_3D ( 'NONE', #9435, #64976, #143 ) ;
#4940=AXIS2_PLACEMENT_3D ( 'NONE', #29965, #50918, #5363 ) ;
#4942=CARTESIAN_POINT ( 'NONE',  ( -3.484441229472478252, -8.595929743150758640, 8.383143565561299582 ) ) ;
#4944=CARTESIAN_POINT ( 'NONE',  ( -17.69233425103264423, 6.603005964784629533, -11.77702021843230007 ) ) ;
#4945=CARTESIAN_POINT ( 'NONE',  ( -37.00000000000000711, 1.030638227056741574, -12.14284015767849034 ) ) ;
#4946=DIRECTION ( 'NONE',  ( -1.000000000000000000, 0.000000000000000000, 0.000000000000000000 ) ) ;
#4948=CARTESIAN_POINT ( 'NONE',  ( 35.00000000000000000, 8.766823244861988940, -7.817610399097547180 ) ) ;
#4951=CARTESIAN_POINT ( 'NONE',  ( -25.86628395826706850, -8.041618865309574815, 10.84354029019568522 ) ) ;
#4952=EDGE_CURVE ( 'NONE', #34891, #20989, #56692, .T. ) ;
#4956=EDGE_CURVE ( 'NONE', #38662, #27609, #30907, .T. ) ;
#4960=CARTESIAN_POINT ( 'NONE',  ( 35.00000000000000000, -4.603882218679472338, 10.80631716521671493 ) ) ;
#4961=CARTESIAN_POINT ( 'NONE',  ( 35.00000000000000000, -11.73808581813437613, 0.4353888892049613824 ) ) ;
#4964=CARTESIAN_POINT ( 'NONE',  ( 6.361445718264521432, -4.355102044641763648, 12.77822703589027320 ) ) ;
#4965=EDGE_LOOP ( 'NONE', ( #18528, #35963, #37243, #8002 ) ) ;
#4966=ADVANCED_FACE ( 'NONE', ( #2466 ), #49006, .T. ) ;
#4969=ORIENTED_EDGE ( 'NONE', *, *, #46621, .T. ) ;
#4973=CARTESIAN_POINT ( 'NONE',  ( -37.00000000000000711, -7.971186206369537786, 9.217970097227697224 ) ) ;
#4974=DIRECTION ( 'NONE',  ( 1.000000000000000000, 0.000000000000000000, -0.000000000000000000 ) ) ;
#4975=EDGE_CURVE ( 'NONE', #15890, #7338, #59586, .T. ) ;
#4976=CARTESIAN_POINT ( 'NONE',  ( 37.00000000000000711, 6.917234959366825642, -9.493370459201726064 ) ) ;
#4978=ORIENTED_EDGE ( 'NONE', *, *, #54572, .T. ) ;
#4981=AXIS2_PLACEMENT_3D ( 'NONE', #37938, #17677, #26992 ) ;
#4982=CYLINDRICAL_SURFACE ( 'NONE', #45772, 5.000000000000000888 ) ;
#4984=CARTESIAN_POINT ( 'NONE',  ( 37.00000000000000711, 11.01837265713073144, -6.415447294506746445 ) ) ;
#4986=VECTOR ( 'NONE', #9054, 1000.000000000000000 ) ;
#4987=ADVANCED_FACE ( 'NONE', ( #17750 ), #33684, .T. ) ;
#4988=FACE_BOUND ( 'NONE', #41732, .T. ) ;
#4989=ORIENTED_EDGE ( 'NONE', *, *, #27853, .T. ) ;
#4990=DIRECTION ( 'NONE',  ( -0.9748757316300199482, 0.000000000000000000, 0.2227494284590502138 ) ) ;
#4991=DIRECTION ( 'NONE',  ( 1.000000000000000000, 0.000000000000000000, 0.000000000000000000 ) ) ;
#4992=CARTESIAN_POINT ( 'NONE',  ( 16.78263030916553333, 10.48479066935627202, 5.836879698929882565 ) ) ;
#4993=CARTESIAN_POINT ( 'NONE',  ( 4.833640382554417414, -10.56051903602595132, 5.701708524974907988 ) ) ;
#4994=VERTEX_POINT ( 'NONE', #58659 ) ;
#4995=ORIENTED_EDGE ( 'NONE', *, *, #22585, .F. ) ;
#4996=ADVANCED_FACE ( 'NONE', ( #53329 ), #48668, .T. ) ;
#4997=CARTESIAN_POINT ( 'NONE',  ( -35.00000000000000000, 11.23004253107764505, 4.732539170486304236 ) ) ;
#4998=ORIENTED_EDGE ( 'NONE', *, *, #11770, .F. ) ;
#5002=VERTEX_POINT ( 'NONE', #3122 ) ;
#5006=CARTESIAN_POINT ( 'NONE',  ( 35.00000000000000000, 9.908974237959730758, 6.307491713048920090 ) ) ;
#5008=ORIENTED_EDGE ( 'NONE', *, *, #53074, .T. ) ;
#5010=VERTEX_POINT ( 'NONE', #28692 ) ;
#5011=CARTESIAN_POINT ( 'NONE',  ( 35.00000000000000000, 2.220215194442072271, 11.98254675519225287 ) ) ;
#5013=ORIENTED_EDGE ( 'NONE', *, *, #45355, .F. ) ;
#5016=ADVANCED_FACE ( 'NONE', ( #28057 ), #44000, .T. ) ;
#5018=ORIENTED_EDGE ( 'NONE', *, *, #31461, .F. ) ;
#5020=AXIS2_PLACEMENT_3D ( 'NONE', #4443, #9729, #24714 ) ;
#5026=DIRECTION ( 'NONE',  ( 0.000000000000000000, -0.01356324068817998940, 0.9999080150203990547 ) ) ;
#5027=EDGE_LOOP ( 'NONE', ( #48748, #32294, #20041, #549 ) ) ;
#5028=EDGE_CURVE ( 'NONE', #6695, #16592, #21319, .T. ) ;
#5029=CARTESIAN_POINT ( 'NONE',  ( 37.00000000000000711, -11.65150730582935523, -1.488153103996925797 ) ) ;
#5030=LINE ( 'NONE', #60538, #41798 ) ;
#5031=DIRECTION ( 'NONE',  ( 0.000000000000000000, 0.01356324068817998940, -0.9999080150203990547 ) ) ;
#5032=VECTOR ( 'NONE', #57919, 1000.000000000000000 ) ;
#5034=EDGE_CURVE ( 'NONE', #25959, #40797, #64836, .T. ) ;
#5035=AXIS2_PLACEMENT_3D ( 'NONE', #64812, #29264, #55765 ) ;
#5038=ADVANCED_FACE ( 'NONE', ( #35306 ), #50630, .T. ) ;
#5039=DIRECTION ( 'NONE',  ( -1.000000000000000000, -0.000000000000000000, 0.000000000000000000 ) ) ;
#5041=ORIENTED_EDGE ( 'NONE', *, *, #26778, .T. ) ;
#5042=( BOUNDED_CURVE ( )  B_SPLINE_CURVE ( 3, ( #27197, #62758, #58123, #47489 ),
 .UNSPECIFIED., .F., .F. ) 
 B_SPLINE_CURVE_WITH_KNOTS ( ( 4, 4 ),
 ( 2.475131039105764152, 2.535910263743374582 ),
 .UNSPECIFIED. ) 
 CURVE ( )  GEOMETRIC_REPRESENTATION_ITEM ( )  RATIONAL_B_SPLINE_CURVE ( ( 1.000000000000000000, 0.9996921808454459768, 0.9996921808454459768, 1.000000000000000000 ) ) 
 REPRESENTATION_ITEM ( '' )  );
#5043=ORIENTED_EDGE ( 'NONE', *, *, #9364, .T. ) ;
#5044=CARTESIAN_POINT ( 'NONE',  ( -18.25006854224444908, -9.443202773001939221, -7.404452808139720510 ) ) ;
#5046=DIRECTION ( 'NONE',  ( -1.000000000000000000, -0.000000000000000000, 0.000000000000000000 ) ) ;
#5049=ORIENTED_EDGE ( 'NONE', *, *, #10407, .T. ) ;
#5051=VERTEX_POINT ( 'NONE', #25671 ) ;
#5053=CARTESIAN_POINT ( 'NONE',  ( 28.56560408307198884, -10.68382391369774709, 5.468123827008506410 ) ) ;
#5056=AXIS2_PLACEMENT_3D ( 'NONE', #45296, #65553, #31317 ) ;
#5057=DIRECTION ( 'NONE',  ( -1.000000000000000000, 0.000000000000000000, -0.000000000000000000 ) ) ;
#5058=ORIENTED_EDGE ( 'NONE', *, *, #57463, .F. ) ;
#5060=DIRECTION ( 'NONE',  ( -1.000000000000000000, 0.000000000000000000, 0.000000000000000000 ) ) ;
#5061=CARTESIAN_POINT ( 'NONE',  ( -37.00000000000000711, 2.080187960898737476, -12.57916205664479214 ) ) ;
#5063=AXIS2_PLACEMENT_3D ( 'NONE', #6652, #46235, #61833 ) ;
#5065=DIRECTION ( 'NONE',  ( 0.000000000000000000, 0.01356324068817992175, -0.9999080150203990547 ) ) ;
#5067=CARTESIAN_POINT ( 'NONE',  ( 35.00000000000000000, -10.63508530065518443, 4.986700593229810963 ) ) ;
#5068=ORIENTED_EDGE ( 'NONE', *, *, #14772, .T. ) ;
#5070=CARTESIAN_POINT ( 'NONE',  ( -25.86628395826706850, 8.041618865309581921, 10.84354029019568522 ) ) ;
#5074=CIRCLE ( 'NONE', #42205, 4.999999999999999112 ) ;
#5078=DIRECTION ( 'NONE',  ( 1.000000000000000000, 0.000000000000000000, 0.000000000000000000 ) ) ;
#5080=LINE ( 'NONE', #25676, #31452 ) ;
#5081=AXIS2_PLACEMENT_3D ( 'NONE', #11122, #17075, #6139 ) ;
#5082=CARTESIAN_POINT ( 'NONE',  ( 35.00000000000000000, -11.23004253107767880, -4.732539170486222524 ) ) ;
#5085=CARTESIAN_POINT ( 'NONE',  ( -36.00000000000000711, 9.733281772932279807, -8.235637554476541666 ) ) ;
#5088=EDGE_LOOP ( 'NONE', ( #2988, #24299, #37985, #56306 ) ) ;
#5089=FACE_OUTER_BOUND ( 'NONE', #403, .T. ) ;
#5090=ORIENTED_EDGE ( 'NONE', *, *, #40336, .T. ) ;
#5091=VERTEX_POINT ( 'NONE', #20688 ) ;
#5095=DIRECTION ( 'NONE',  ( 0.000000000000000000, -0.7790879021242441693, 0.6269146997508066033 ) ) ;
#5096=CARTESIAN_POINT ( 'NONE',  ( 11.74548640120467979, 8.775604215601129354, -8.184666801472349817 ) ) ;
#5098=CARTESIAN_POINT ( 'NONE',  ( -36.00000000000000711, -11.73555825188280011, 4.983891302653541189 ) ) ;
#5099=EDGE_CURVE ( 'NONE', #37413, #38593, #55305, .T. ) ;
#5105=EDGE_CURVE ( 'NONE', #37124, #49993, #52019, .T. ) ;
#5106=CARTESIAN_POINT ( 'NONE',  ( 37.00000000000000711, -12.02534193257717732, 4.237174932027349961 ) ) ;
#5112=AXIS2_PLACEMENT_3D ( 'NONE', #24058, #23074, #58996 ) ;
#5113=EDGE_CURVE ( 'NONE', #49413, #51431, #6482, .T. ) ;
#5115=CARTESIAN_POINT ( 'NONE',  ( 35.00000000000000000, -6.102719229070595830, 10.54834585426226390 ) ) ;
#5116=DIRECTION ( 'NONE',  ( 0.000000000000000000, -0.01356324068817998940, 0.9999080150203990547 ) ) ;
#5117=CARTESIAN_POINT ( 'NONE',  ( -37.00000000000000711, -9.913596905230058098, -8.017674001891892388 ) ) ;
#5119=DIRECTION ( 'NONE',  ( -1.000000000000000000, 0.000000000000000000, 0.000000000000000000 ) ) ;
#5120=DIRECTION ( 'NONE',  ( 0.000000000000000000, -1.000000000000000000, 0.000000000000000000 ) ) ;
#5121=EDGE_LOOP ( 'NONE', ( #11839, #19611, #16092, #17241 ) ) ;
#5123=CARTESIAN_POINT ( 'NONE',  ( 2.879519832977797567, 3.585229973219939748, -11.45904250108715416 ) ) ;
#5124=DIRECTION ( 'NONE',  ( -0.000000000000000000, -1.000000000000000000, -0.000000000000000000 ) ) ;
#5126=CARTESIAN_POINT ( 'NONE',  ( 21.63147231831337791, 13.42138622850559138, -1.508105519309493658 ) ) ;
#5127=DIRECTION ( 'NONE',  ( 0.000000000000000000, 0.01356324068817998940, -0.9999080150203990547 ) ) ;
#5128=ORIENTED_EDGE ( 'NONE', *, *, #6637, .F. ) ;
#5129=ORIENTED_EDGE ( 'NONE', *, *, #18926, .F. ) ;
#5134=ADVANCED_FACE ( 'NONE', ( #16005 ), #10691, .T. ) ;
#5135=DIRECTION ( 'NONE',  ( 0.000000000000000000, -0.8989688749565111214, -0.4380125133594070519 ) ) ;
#5136=FACE_OUTER_BOUND ( 'NONE', #25904, .T. ) ;
#5137=DIRECTION ( 'NONE',  ( -1.000000000000000000, 0.000000000000000000, 0.000000000000000000 ) ) ;
#5140=CIRCLE ( 'NONE', #4096, 12.18649999999999878 ) ;
#5142=CARTESIAN_POINT ( 'NONE',  ( 11.99003848479309831, -10.55797189877288922, -8.414293459742250292 ) ) ;
#5144=VERTEX_POINT ( 'NONE', #21331 ) ;
#5146=DIRECTION ( 'NONE',  ( 1.000000000000000000, 0.000000000000000000, 0.000000000000000000 ) ) ;
#5147=ORIENTED_EDGE ( 'NONE', *, *, #2815, .T. ) ;
#5150=ORIENTED_EDGE ( 'NONE', *, *, #56497, .F. ) ;
#5153=VECTOR ( 'NONE', #45804, 1000.000000000000000 ) ;
#5155=DIRECTION ( 'NONE',  ( 0.000000000000000000, -0.01356324068817991828, 0.9999080150203990547 ) ) ;
#5156=EDGE_CURVE ( 'NONE', #6304, #39733, #56936, .T. ) ;
#5157=CARTESIAN_POINT ( 'NONE',  ( 10.66583743953261809, 7.973724152180643010, 8.969682718315048930 ) ) ;
#5158=CARTESIAN_POINT ( 'NONE',  ( 37.00000000000000711, -2.696588552979144460, -12.46157735505188491 ) ) ;
#5160=AXIS2_PLACEMENT_3D ( 'NONE', #23259, #54518, #64777 ) ;
#5161=AXIS2_PLACEMENT_3D ( 'NONE', #18143, #3855, #44067 ) ;
#5165=AXIS2_PLACEMENT_3D ( 'NONE', #1735, #22002, #37288 ) ;
#5166=ORIENTED_EDGE ( 'NONE', *, *, #35744, .T. ) ;
#5168=CARTESIAN_POINT ( 'NONE',  ( -37.00000000000000711, 6.917234959366964198, -9.493370459201624811 ) ) ;
#5169=AXIS2_PLACEMENT_3D ( 'NONE', #43848, #23914, #60120 ) ;
#5170=CARTESIAN_POINT ( 'NONE',  ( -35.00000000000000000, -4.018060380616481631, 11.50504120060941915 ) ) ;
#5171=CARTESIAN_POINT ( 'NONE',  ( 16.90635187068963319, 9.959026633630651659, 6.781309966538392686 ) ) ;
#5173=LINE ( 'NONE', #41374, #49081 ) ;
#5174=PLANE ( 'NONE',  #52485 ) ;
#5176=ORIENTED_EDGE ( 'NONE', *, *, #52274, .F. ) ;
#5177=ORIENTED_EDGE ( 'NONE', *, *, #29490, .T. ) ;
#5179=CARTESIAN_POINT ( 'NONE',  ( -37.00000000000000711, -3.640372113593639547, 12.21925492305360983 ) ) ;
#5182=AXIS2_PLACEMENT_3D ( 'NONE', #53849, #64452, #23924 ) ;
#5184=CYLINDRICAL_SURFACE ( 'NONE', #50079, 4.999999999999999112 ) ;
#5187=EDGE_CURVE ( 'NONE', #35366, #30999, #17341, .T. ) ;
#5189=CARTESIAN_POINT ( 'NONE',  ( -18.08686583997275221, 5.151216734910927464, -12.47858029384662970 ) ) ;
#5190=CARTESIAN_POINT ( 'NONE',  ( 22.57855258442564761, -4.427776684447072952, -11.15324139578564910 ) ) ;
#5191=CARTESIAN_POINT ( 'NONE',  ( -35.00000000000000000, 0.000000000000000000, 0.000000000000000000 ) ) ;
#5192=EDGE_CURVE ( 'NONE', #39732, #37109, #21020, .T. ) ;
#5193=AXIS2_PLACEMENT_3D ( 'NONE', #1582, #10880, #31169 ) ;
#5194=CARTESIAN_POINT ( 'NONE',  ( 37.00000000000000711, 4.705694406421931860E-17, -3.469127814946512892E-15 ) ) ;
#5196=EDGE_LOOP ( 'NONE', ( #57397, #60145, #55905, #60991 ) ) ;
#5197=CARTESIAN_POINT ( 'NONE',  ( -35.00000000000000000, 0.000000000000000000, 0.000000000000000000 ) ) ;
#5200=EDGE_LOOP ( 'NONE', ( #36657, #4393, #31789, #12330 ) ) ;
#5203=CARTESIAN_POINT ( 'NONE',  ( -36.00000000000000711, -0.6593684648221369571, 12.73293890771483383 ) ) ;
#5206=CYLINDRICAL_SURFACE ( 'NONE', #1063, 12.18649999999999878 ) ;
#5207=ORIENTED_EDGE ( 'NONE', *, *, #23845, .F. ) ;
#5209=EDGE_CURVE ( 'NONE', #9622, #64587, #8605, .T. ) ;
#5212=CARTESIAN_POINT ( 'NONE',  ( -1.734723475976807094E-15, -3.469446951953614189E-15, -11.99999999999998934 ) ) ;
#5213=CARTESIAN_POINT ( 'NONE',  ( -9.027418811960407297, 12.84010590367175020, -4.182636090463161871 ) ) ;
#5214=CARTESIAN_POINT ( 'NONE',  ( -16.82774105938391429, 8.087890278022925372, -10.80991447578766973 ) ) ;
#5215=CARTESIAN_POINT ( 'NONE',  ( 8.813543937826676000, 6.315452948875024397, -11.93749476812985222 ) ) ;
#5216=CYLINDRICAL_SURFACE ( 'NONE', #54551, 5.000000000000001776 ) ;
#5217=CARTESIAN_POINT ( 'NONE',  ( 37.00000000000000711, 0.3137578094511062066, 12.74613886779084204 ) ) ;
#5218=CARTESIAN_POINT ( 'NONE',  ( 37.00000000000000711, -7.238157050195554554, 10.49626516989278180 ) ) ;
#5222=DIRECTION ( 'NONE',  ( 0.000000000000000000, 0.04924826701373895277, 0.9987865678893280696 ) ) ;
#5225=CIRCLE ( 'NONE', #24335, 5.000000000000000000 ) ;
#5226=CARTESIAN_POINT ( 'NONE',  ( -36.00000000000000711, 9.506317355798369562, 8.496612874013196759 ) ) ;
#5227=ORIENTED_EDGE ( 'NONE', *, *, #5414, .T. ) ;
#5229=CARTESIAN_POINT ( 'NONE',  ( 12.17720086923866951, 9.239009060064711676, -7.666669395372703200 ) ) ;
#5232=VERTEX_POINT ( 'NONE', #6065 ) ;
#5233=ORIENTED_EDGE ( 'NONE', *, *, #42679, .T. ) ;
#5234=DIRECTION ( 'NONE',  ( 0.000000000000000000, -0.01356324068817999114, 0.9999080150203989437 ) ) ;
#5236=CYLINDRICAL_SURFACE ( 'NONE', #29557, 12.18649999999999878 ) ;
#5237=DIRECTION ( 'NONE',  ( 0.000000000000000000, -0.01356324068817991828, 0.9999080150203990547 ) ) ;
#5238=CARTESIAN_POINT ( 'NONE',  ( 37.00000000000000711, 4.018060380616396365, -11.50504120060944757 ) ) ;
#5239=VECTOR ( 'NONE', #59750, 1000.000000000000000 ) ;
#5240=DIRECTION ( 'NONE',  ( -1.000000000000000000, 0.000000000000000000, 0.000000000000000000 ) ) ;
#5242=LINE ( 'NONE', #25510, #5153 ) ;
#5243=CARTESIAN_POINT ( 'NONE',  ( -35.00000000000000000, 6.303578524886947143, 10.42955799785322490 ) ) ;
#5244=VECTOR ( 'NONE', #44505, 1000.000000000000000 ) ;
#5246=ORIENTED_EDGE ( 'NONE', *, *, #31498, .F. ) ;
#5249=EDGE_CURVE ( 'NONE', #56247, #50602, #63207, .T. ) ;
#5250=CARTESIAN_POINT ( 'NONE',  ( 35.00000000000000000, -11.35427606708803161, 4.426194442447358490 ) ) ;
#5252=CARTESIAN_POINT ( 'NONE',  ( 12.67839809834435805, 12.93864317191487778, -3.856941399089210076 ) ) ;
#5253=LINE ( 'NONE', #21534, #20162 ) ;
#5256=CIRCLE ( 'NONE', #50920, 12.74999999999999822 ) ;
#5257=CARTESIAN_POINT ( 'NONE',  ( 35.00000000000000000, 5.015831474386306610, -10.62137734850269943 ) ) ;
#5258=ORIENTED_EDGE ( 'NONE', *, *, #43132, .T. ) ;
#5262=CARTESIAN_POINT ( 'NONE',  ( -3.543624739456839645, -9.146489499550646940, 7.778742444933206102 ) ) ;
#5265=DIRECTION ( 'NONE',  ( 0.000000000000000000, -0.9105187689795911643, 0.4134677391718609707 ) ) ;
#5266=CYLINDRICAL_SURFACE ( 'NONE', #27569, 15.00000000000000000 ) ;
#5270=LINE ( 'NONE', #51160, #8733 ) ;
#5271=CARTESIAN_POINT ( 'NONE',  ( 35.00000000000000000, 11.61175578952788356, 1.771820996347031940 ) ) ;
#5273=AXIS2_PLACEMENT_3D ( 'NONE', #24557, #64149, #18625 ) ;
#5274=FACE_OUTER_BOUND ( 'NONE', #49786, .T. ) ;
#5279=ORIENTED_EDGE ( 'NONE', *, *, #29490, .F. ) ;
#5281=CARTESIAN_POINT ( 'NONE',  ( 47.00000000000000711, 4.705694406421931860E-17, -3.469127814946512892E-15 ) ) ;
#5282=FACE_OUTER_BOUND ( 'NONE', #16550, .T. ) ;
#5284=CIRCLE ( 'NONE', #13753, 4.999999999999999112 ) ;
#5286=ORIENTED_EDGE ( 'NONE', *, *, #42675, .T. ) ;
#5288=CARTESIAN_POINT ( 'NONE',  ( -16.98800322446194855, 2.922502605998049674, -13.17987020110343543 ) ) ;
#5290=AXIS2_PLACEMENT_3D ( 'NONE', #22961, #53872, #53557 ) ;
#5291=CARTESIAN_POINT ( 'NONE',  ( 35.00000000000000000, 4.705694406421931860E-17, -3.469127814946512892E-15 ) ) ;
#5294=DIRECTION ( 'NONE',  ( -1.000000000000000000, -0.000000000000000000, 0.000000000000000000 ) ) ;
#5299=ORIENTED_EDGE ( 'NONE', *, *, #62647, .F. ) ;
#5301=CIRCLE ( 'NONE', #46726, 4.999999999999999112 ) ;
#5302=ORIENTED_EDGE ( 'NONE', *, *, #27879, .F. ) ;
#5303=DIRECTION ( 'NONE',  ( 1.000000000000000000, -0.000000000000000000, 0.000000000000000000 ) ) ;
#5309=DIRECTION ( 'NONE',  ( 0.000000000000000000, 0.01356324068817992175, -0.9999080150203990547 ) ) ;
#5310=CARTESIAN_POINT ( 'NONE',  ( -19.47984447937493613, -1.416020129149132334, 25.00000000000000000 ) ) ;
#5312=CARTESIAN_POINT ( 'NONE',  ( 7.253112616783349509, -5.573154064202213931, 10.62982316258792537 ) ) ;
#5314=ORIENTED_EDGE ( 'NONE', *, *, #55178, .F. ) ;
#5316=ORIENTED_EDGE ( 'NONE', *, *, #47336, .F. ) ;
#5317=CARTESIAN_POINT ( 'NONE',  ( 35.00000000000000000, 4.705694406421931860E-17, -3.469127814946512892E-15 ) ) ;
#5320=ORIENTED_EDGE ( 'NONE', *, *, #56146, .F. ) ;
#5321=DIRECTION ( 'NONE',  ( -1.000000000000000000, -0.000000000000000000, 0.000000000000000000 ) ) ;
#5323=CIRCLE ( 'NONE', #49932, 12.74999999999999822 ) ;
#5325=CARTESIAN_POINT ( 'NONE',  ( -35.00000000000000000, 0.000000000000000000, 0.000000000000000000 ) ) ;
#5329=VERTEX_POINT ( 'NONE', #5960 ) ;
#5332=DIRECTION ( 'NONE',  ( -1.000000000000000000, -0.000000000000000000, 0.000000000000000000 ) ) ;
#5333=ADVANCED_FACE ( 'NONE', ( #62755 ), #22542, .T. ) ;
#5334=CARTESIAN_POINT ( 'NONE',  ( -3.550933850019966531, 11.20544481737731068, 7.538207320140815071 ) ) ;
#5335=EDGE_CURVE ( 'NONE', #50397, #44716, #1166, .T. ) ;
#5336=B_SPLINE_CURVE_WITH_KNOTS ( 'NONE', 3,
 ( #12289, #12953, #48548, #33236, #53546, #47881 ),
 .UNSPECIFIED., .F., .F.,
 ( 4, 2, 4 ),
 ( 0.004228585846910009986, 0.006274987364148632354, 0.008321388881387255590 ),
 .UNSPECIFIED. ) ;
#5338=CARTESIAN_POINT ( 'NONE',  ( 37.00000000000000711, 6.564808257521771218, -10.93004082984021075 ) ) ;
#5339=DIRECTION ( 'NONE',  ( 0.000000000000000000, 0.01356324068817998940, -0.9999080150203990547 ) ) ;
#5344=CARTESIAN_POINT ( 'NONE',  ( -37.00000000000000711, 0.000000000000000000, 0.000000000000000000 ) ) ;
#5346=EDGE_LOOP ( 'NONE', ( #11701, #61492, #32104, #16570 ) ) ;
#5347=EDGE_CURVE ( 'NONE', #55989, #63543, #9636, .T. ) ;
#5348=CARTESIAN_POINT ( 'NONE',  ( -24.35585564769671407, -10.90390688210781356, 7.962067492493469345 ) ) ;
#5350=FACE_OUTER_BOUND ( 'NONE', #51042, .T. ) ;
#5351=CARTESIAN_POINT ( 'NONE',  ( 36.00000000000000711, -2.080187960898473243, 12.57916205664483122 ) ) ;
#5353=ORIENTED_EDGE ( 'NONE', *, *, #7362, .F. ) ;
#5354=CARTESIAN_POINT ( 'NONE',  ( 35.00000000000000000, 4.705694406421931860E-17, -3.469127814946512892E-15 ) ) ;
#5358=CARTESIAN_POINT ( 'NONE',  ( 22.22366945088117518, -13.44460711623439941, -1.270151499113232774 ) ) ;
#5359=ADVANCED_FACE ( 'NONE', ( #17225 ), #17558, .T. ) ;
#5363=DIRECTION ( 'NONE',  ( 0.000000000000000000, -0.01356324068817992175, 0.9999080150203990547 ) ) ;
#5364=CARTESIAN_POINT ( 'NONE',  ( -35.00000000000000000, -11.37311665002361494, -2.936739658819992549 ) ) ;
#5365=CIRCLE ( 'NONE', #58438, 5.000000000000000888 ) ;
#5366=CIRCLE ( 'NONE', #51035, 12.00000000000000000 ) ;
#5367=AXIS2_PLACEMENT_3D ( 'NONE', #36002, #17646, #51674 ) ;
#5370=CARTESIAN_POINT ( 'NONE',  ( -35.00000000000000000, -11.78745411414837818, -3.093009498344053032 ) ) ;
#5374=ORIENTED_EDGE ( 'NONE', *, *, #12286, .F. ) ;
#5375=ORIENTED_EDGE ( 'NONE', *, *, #41754, .T. ) ;
#5379=CIRCLE ( 'NONE', #53182, 12.18650000000000055 ) ;
#5380=EDGE_CURVE ( 'NONE', #62829, #39914, #32980, .T. ) ;
#5381=DIRECTION ( 'NONE',  ( -1.000000000000000000, -0.000000000000000000, -0.000000000000000000 ) ) ;
#5382=EDGE_LOOP ( 'NONE', ( #12078, #56682, #44010, #42765 ) ) ;
#5383=( LENGTH_UNIT ( ) NAMED_UNIT ( * ) SI_UNIT ( .MILLI., .METRE. ) );
#5386=AXIS2_PLACEMENT_3D ( 'NONE', #13837, #23191, #17878 ) ;
#5388=ORIENTED_EDGE ( 'NONE', *, *, #63224, .T. ) ;
#5389=DIRECTION ( 'NONE',  ( 0.4838294062566934617, -0.000000000000000000, 0.8751623310228197061 ) ) ;
#5392=DIRECTION ( 'NONE',  ( 0.000000000000000000, -1.000000000000000000, 0.000000000000000000 ) ) ;
#5393=EDGE_LOOP ( 'NONE', ( #61495, #51271, #36075, #15378 ) ) ;
#5394=CARTESIAN_POINT ( 'NONE',  ( -25.64778288570173004, 7.682669607182226024, 11.10295593026793881 ) ) ;
#5395=EDGE_LOOP ( 'NONE', ( #37409, #20370, #39695, #7081 ) ) ;
#5396=DIRECTION ( 'NONE',  ( 1.000000000000000000, 0.000000000000000000, 0.000000000000000000 ) ) ;
#5399=CARTESIAN_POINT ( 'NONE',  ( 13.15445328062423691, -9.891953278793183202, -6.796930734482528713 ) ) ;
#5401=CARTESIAN_POINT ( 'NONE',  ( -35.00000000000000000, -11.60979404548637461, 3.704519465651263221 ) ) ;
#5404=EDGE_CURVE ( 'NONE', #45182, #30052, #43620, .T. ) ;
#5406=DIRECTION ( 'NONE',  ( 1.000000000000000000, 0.000000000000000000, 0.000000000000000000 ) ) ;
#5407=CARTESIAN_POINT ( 'NONE',  ( 8.450039533779039047, 4.867621807257259015, -10.97047568558763686 ) ) ;
#5408=CARTESIAN_POINT ( 'NONE',  ( -18.14857107993011809, 3.486035047582784596, -13.04429203975358398 ) ) ;
#5411=ORIENTED_EDGE ( 'NONE', *, *, #20981, .F. ) ;
#5414=EDGE_CURVE ( 'NONE', #65324, #21734, #28777, .T. ) ;
#5416=DIRECTION ( 'NONE',  ( 1.000000000000000000, 0.000000000000000000, -0.000000000000000000 ) ) ;
#5419=ORIENTED_EDGE ( 'NONE', *, *, #52269, .T. ) ;
#5422=CARTESIAN_POINT ( 'NONE',  ( 22.68177428654798433, -4.560196341733016467, 11.10067150598529473 ) ) ;
#5424=CARTESIAN_POINT ( 'NONE',  ( 35.00000000000000000, 4.705694406421931860E-17, -3.469127814946512892E-15 ) ) ;
#5426=AXIS2_PLACEMENT_3D ( 'NONE', #41840, #16246, #17567 ) ;
#5429=CIRCLE ( 'NONE', #30887, 5.000000000000000000 ) ;
#5431=EDGE_CURVE ( 'NONE', #14694, #21888, #14949, .T. ) ;
#5432=PLANE ( 'NONE',  #1053 ) ;
#5433=CARTESIAN_POINT ( 'NONE',  ( -35.00000000000000000, -0.7214809346827719683, -11.72397916322013245 ) ) ;
#5434=CARTESIAN_POINT ( 'NONE',  ( 37.00000000000000711, -6.018036132182079889, 11.24036214326526562 ) ) ;
#5435=EDGE_CURVE ( 'NONE', #53566, #52362, #57467, .T. ) ;
#5436=EDGE_LOOP ( 'NONE', ( #40708, #37368, #33934, #63030 ) ) ;
#5438=EDGE_CURVE ( 'NONE', #16210, #13952, #54282, .T. ) ;
#5440=CIRCLE ( 'NONE', #29796, 4.999999999999999112 ) ;
#5441=ADVANCED_FACE ( 'NONE', ( #38813 ), #8224, .F. ) ;
#5444=( BOUNDED_CURVE ( )  B_SPLINE_CURVE ( 3, ( #13359, #33646, #12044, #17378 ),
 .UNSPECIFIED., .F., .F. ) 
 B_SPLINE_CURVE_WITH_KNOTS ( ( 4, 4 ),
 ( 4.547159998450355900, 4.564492336233753278 ),
 .UNSPECIFIED. ) 
 CURVE ( )  GEOMETRIC_REPRESENTATION_ITEM ( )  RATIONAL_B_SPLINE_CURVE ( ( 1.000000000000000000, 0.9999749659955903258, 0.9999749659955903258, 1.000000000000000000 ) ) 
 REPRESENTATION_ITEM ( '' )  );
#5445=CYLINDRICAL_SURFACE ( 'NONE', #14976, 4.999999999999999112 ) ;
#5446=CIRCLE ( 'NONE', #28782, 12.18650000000000055 ) ;
#5447=EDGE_CURVE ( 'NONE', #27171, #9320, #64079, .T. ) ;
#5448=CARTESIAN_POINT ( 'NONE',  ( -35.00000000000000000, 11.17622378668011685, -3.614449339633368119 ) ) ;
#5451=DIRECTION ( 'NONE',  ( 0.000000000000000000, 0.01356324068817998940, -0.9999080150203990547 ) ) ;
#5454=AXIS2_PLACEMENT_3D ( 'NONE', #6560, #51786, #6229 ) ;
#5455=CARTESIAN_POINT ( 'NONE',  ( -27.19357181888462094, 25.00000000000000000, 5.138615876886901468 ) ) ;
#5457=AXIS2_PLACEMENT_3D ( 'NONE', #2732, #22663, #37937 ) ;
#5465=AXIS2_PLACEMENT_3D ( 'NONE', #2850, #63010, #23109 ) ;
#5467=EDGE_LOOP ( 'NONE', ( #31384, #55400, #57620, #22218 ) ) ;
#5468=ORIENTED_EDGE ( 'NONE', *, *, #30287, .T. ) ;
#5470=CIRCLE ( 'NONE', #137, 12.74999999999999822 ) ;
#5471=EDGE_CURVE ( 'NONE', #62855, #35253, #59112, .T. ) ;
#5472=VECTOR ( 'NONE', #10476, 1000.000000000000000 ) ;
#5474=VERTEX_POINT ( 'NONE', #22878 ) ;
#5479=CARTESIAN_POINT ( 'NONE',  ( 37.00000000000000711, -2.865935305911543551, 12.42372387097884712 ) ) ;
#5481=CARTESIAN_POINT ( 'NONE',  ( -35.00000000000000000, -6.102719229070750373, 10.54834585426218041 ) ) ;
#5483=ORIENTED_EDGE ( 'NONE', *, *, #50683, .T. ) ;
#5485=ORIENTED_EDGE ( 'NONE', *, *, #865, .T. ) ;
#5487=ORIENTED_EDGE ( 'NONE', *, *, #42795, .T. ) ;
#5488=EDGE_CURVE ( 'NONE', #44279, #46540, #13522, .T. ) ;
#5490=ORIENTED_EDGE ( 'NONE', *, *, #45293, .F. ) ;
#5492=AXIS2_PLACEMENT_3D ( 'NONE', #62696, #2554, #7859 ) ;
#5496=DIRECTION ( 'NONE',  ( 0.000000000000000000, 0.01356324068817998940, -0.9999080150203990547 ) ) ;
#5497=AXIS2_PLACEMENT_3D ( 'NONE', #64688, #50739, #54752 ) ;
#5499=ORIENTED_EDGE ( 'NONE', *, *, #57282, .F. ) ;
#5502=CIRCLE ( 'NONE', #22466, 5.000000000000000000 ) ;
#5503=ADVANCED_FACE ( 'NONE', ( #8879 ), #54103, .F. ) ;
#5504=ORIENTED_EDGE ( 'NONE', *, *, #14327, .T. ) ;
#5505=VECTOR ( 'NONE', #56715, 1000.000000000000000 ) ;
#5508=CARTESIAN_POINT ( 'NONE',  ( -37.00000000000000711, 12.63095688309031495, -1.738225594539862584 ) ) ;
#5511=CYLINDRICAL_SURFACE ( 'NONE', #33097, 4.999999999999999112 ) ;
#5512=CIRCLE ( 'NONE', #13978, 5.000000000000000888 ) ;
#5513=ORIENTED_EDGE ( 'NONE', *, *, #48908, .F. ) ;
#5514=VERTEX_POINT ( 'NONE', #29171 ) ;
#5515=AXIS2_PLACEMENT_3D ( 'NONE', #64260, #39644, #9363 ) ;
#5517=DIRECTION ( 'NONE',  ( 1.000000000000000000, 0.000000000000000000, 0.000000000000000000 ) ) ;
#5518=CARTESIAN_POINT ( 'NONE',  ( -2.729227863478770111, -12.79029713166804250, 4.331329641846414447 ) ) ;
#5519=EDGE_CURVE ( 'NONE', #62845, #15867, #39125, .T. ) ;
#5521=AXIS2_PLACEMENT_3D ( 'NONE', #53514, #12265, #1661 ) ;
#5522=CYLINDRICAL_SURFACE ( 'NONE', #33408, 4.999999999999999112 ) ;
#5523=VECTOR ( 'NONE', #25385, 1000.000000000000000 ) ;
#5524=CARTESIAN_POINT ( 'NONE',  ( 35.00000000000000000, 4.705694406421931860E-17, -3.469127814946512892E-15 ) ) ;
#5526=CARTESIAN_POINT ( 'NONE',  ( 23.56735259781322611, 2.000748643224683487, -13.35387901052309800 ) ) ;
#5528=EDGE_CURVE ( 'NONE', #40710, #19771, #60597, .T. ) ;
#5529=CARTESIAN_POINT ( 'NONE',  ( 35.00000000000000000, 9.196955404009292678, -8.830544224262981245 ) ) ;
#5530=ORIENTED_EDGE ( 'NONE', *, *, #58041, .F. ) ;
#5532=CARTESIAN_POINT ( 'NONE',  ( 35.00000000000000000, -7.238157050195554554, 10.49626516989278180 ) ) ;
#5533=CIRCLE ( 'NONE', #48010, 5.000000000000000888 ) ;
#5534=CIRCLE ( 'NONE', #7655, 4.999999999999999112 ) ;
#5537=CARTESIAN_POINT ( 'NONE',  ( 35.00000000000000000, -10.54834585426224258, -6.102719229070642903 ) ) ;
#5541=AXIS2_PLACEMENT_3D ( 'NONE', #56932, #16354, #16992 ) ;
#5544=CARTESIAN_POINT ( 'NONE',  ( 19.28625800530496903, 6.413918128308424116, 11.87904264843580471 ) ) ;
#5545=CYLINDRICAL_SURFACE ( 'NONE', #43773, 12.75000000000000178 ) ;
#5546=DIRECTION ( 'NONE',  ( 0.000000000000000000, -0.07632122047555053856, 0.9970832820307050648 ) ) ;
#5547=AXIS2_PLACEMENT_3D ( 'NONE', #3305, #42863, #34189 ) ;
#5548=DIRECTION ( 'NONE',  ( 1.000000000000000000, 0.000000000000000000, -0.000000000000000000 ) ) ;
#5549=VERTEX_POINT ( 'NONE', #53122 ) ;
#5550=CARTESIAN_POINT ( 'NONE',  ( -35.00000000000000000, 0.7536123767500182424, -11.72195762423409171 ) ) ;
#5551=EDGE_CURVE ( 'NONE', #17913, #10194, #42362, .T. ) ;
#5552=DIRECTION ( 'NONE',  ( -1.000000000000000000, 0.000000000000000000, 0.000000000000000000 ) ) ;
#5554=PLANE ( 'NONE',  #38681 ) ;
#5555=EDGE_CURVE ( 'NONE', #57223, #61328, #13715, .T. ) ;
#5558=FACE_OUTER_BOUND ( 'NONE', #11866, .T. ) ;
#5559=DIRECTION ( 'NONE',  ( 0.000000000000000000, -0.01356324068817991481, 0.9999080150203990547 ) ) ;
#5561=DIRECTION ( 'NONE',  ( 1.000000000000000000, 0.000000000000000000, 0.000000000000000000 ) ) ;
#5562=ORIENTED_EDGE ( 'NONE', *, *, #46172, .T. ) ;
#5563=LINE ( 'NONE', #25832, #54422 ) ;
#5564=ORIENTED_EDGE ( 'NONE', *, *, #16681, .F. ) ;
#5566=CARTESIAN_POINT ( 'NONE',  ( -35.00000000000000000, -5.927257550915394191, 10.64792938439753378 ) ) ;
#5570=DIRECTION ( 'NONE',  ( 0.000000000000000000, 0.01356324068818000848, -0.9999080150203990547 ) ) ;
#5572=DIRECTION ( 'NONE',  ( -0.000000000000000000, -1.000000000000000000, -0.000000000000000000 ) ) ;
#5579=EDGE_CURVE ( 'NONE', #34891, #9460, #32784, .T. ) ;
#5581=CARTESIAN_POINT ( 'NONE',  ( -36.00000000000000711, 1.113475361586489631, 12.70128625845193326 ) ) ;
#5582=DIRECTION ( 'NONE',  ( -1.000000000000000000, 0.000000000000000000, -0.000000000000000000 ) ) ;
#5587=AXIS2_PLACEMENT_3D ( 'NONE', #4560, #40096, #8878 ) ;
#5588=DIRECTION ( 'NONE',  ( -1.000000000000000000, 0.000000000000000000, 0.000000000000000000 ) ) ;
#5590=CARTESIAN_POINT ( 'NONE',  ( -4.590058209962335489, 6.612760447609789871, 25.00000000000000000 ) ) ;
#5592=AXIS2_PLACEMENT_3D ( 'NONE', #42322, #36709, #52354 ) ;
#5593=FACE_OUTER_BOUND ( 'NONE', #19161, .T. ) ;
#5595=CARTESIAN_POINT ( 'NONE',  ( -37.00000000000000711, 0.000000000000000000, 0.000000000000000000 ) ) ;
#5596=CARTESIAN_POINT ( 'NONE',  ( -35.00000000000000000, 2.216820770815248309, -11.53507381115581332 ) ) ;
#5598=DIRECTION ( 'NONE',  ( -1.000000000000000000, 0.000000000000000000, 0.000000000000000000 ) ) ;
#5600=LINE ( 'NONE', #42681, #61064 ) ;
#5603=ORIENTED_EDGE ( 'NONE', *, *, #51532, .T. ) ;
#5605=ADVANCED_FACE ( 'NONE', ( #21095 ), #17095, .T. ) ;
#5612=ORIENTED_EDGE ( 'NONE', *, *, #45559, .T. ) ;
#5613=CIRCLE ( 'NONE', #31229, 12.74999999999999822 ) ;
#5614=CARTESIAN_POINT ( 'NONE',  ( 26.34661844826604593, 25.00000000000000000, 3.317828791472333005 ) ) ;
#5615=DIRECTION ( 'NONE',  ( 1.000000000000000000, 0.000000000000000000, 0.000000000000000000 ) ) ;
#5616=AXIS2_PLACEMENT_3D ( 'NONE', #48575, #49875, #64183 ) ;
#5618=CARTESIAN_POINT ( 'NONE',  ( -37.00000000000000711, 12.21925492305362049, 3.640372113593595582 ) ) ;
#5619=CIRCLE ( 'NONE', #44898, 12.75000000000000178 ) ;
#5620=LINE ( 'NONE', #13679, #29884 ) ;
#5622=ORIENTED_EDGE ( 'NONE', *, *, #40016, .F. ) ;
#5624=VERTEX_POINT ( 'NONE', #513 ) ;
#5625=CARTESIAN_POINT ( 'NONE',  ( -35.00000000000000000, 0.000000000000000000, 0.000000000000000000 ) ) ;
#5627=AXIS2_PLACEMENT_3D ( 'NONE', #12119, #37052, #22099 ) ;
#5628=DIRECTION ( 'NONE',  ( 1.000000000000000000, 0.000000000000000000, 0.000000000000000000 ) ) ;
#5629=CARTESIAN_POINT ( 'NONE',  ( -7.756689557399197632, -2.159283824347104641, 11.80546050376997869 ) ) ;
#5632=ORIENTED_EDGE ( 'NONE', *, *, #37503, .F. ) ;
#5635=EDGE_CURVE ( 'NONE', #31395, #924, #43425, .T. ) ;
#5639=DIRECTION ( 'NONE',  ( 0.000000000000000000, 0.01356324068817998940, -0.9999080150203989437 ) ) ;
#5640=DIRECTION ( 'NONE',  ( -1.000000000000000000, 0.000000000000000000, 0.000000000000000000 ) ) ;
#5643=CARTESIAN_POINT ( 'NONE',  ( -9.410738856732004720, -2.781742255745475401, 11.67413128860836302 ) ) ;
#5644=VERTEX_POINT ( 'NONE', #27081 ) ;
#5649=DIRECTION ( 'NONE',  ( 0.000000000000000000, 0.01356324068817998940, -0.9999080150203990547 ) ) ;
#5651=VERTEX_POINT ( 'NONE', #31413 ) ;
#5653=ORIENTED_EDGE ( 'NONE', *, *, #45519, .T. ) ;
#5655=( BOUNDED_CURVE ( )  B_SPLINE_CURVE ( 3, ( #10028, #59925, #19691, #34936 ),
 .UNSPECIFIED., .F., .F. ) 
 B_SPLINE_CURVE_WITH_KNOTS ( ( 4, 4 ),
 ( 2.276420903748625602, 2.328873244820985899 ),
 .UNSPECIFIED. ) 
 CURVE ( )  GEOMETRIC_REPRESENTATION_ITEM ( )  RATIONAL_B_SPLINE_CURVE ( ( 1.000000000000000000, 0.9997707424672948040, 0.9997707424672948040, 1.000000000000000000 ) ) 
 REPRESENTATION_ITEM ( '' )  );
#5656=CARTESIAN_POINT ( 'NONE',  ( 6.582987406907342631, -7.685813705153371700, -11.10488467197773232 ) ) ;
#5657=CARTESIAN_POINT ( 'NONE',  ( -36.00000000000000711, 10.39746860227890757, 7.379373053628905943 ) ) ;
#5661=CARTESIAN_POINT ( 'NONE',  ( -35.00000000000000000, -0.8294751490780184477, 12.15823808070322443 ) ) ;
#5662=ORIENTED_EDGE ( 'NONE', *, *, #34401, .T. ) ;
#5663=DIRECTION ( 'NONE',  ( 1.000000000000000000, 0.000000000000000000, 0.000000000000000000 ) ) ;
#5666=CIRCLE ( 'NONE', #42790, 4.999999999999999112 ) ;
#5671=AXIS2_PLACEMENT_3D ( 'NONE', #42901, #57226, #7006 ) ;
#5674=CARTESIAN_POINT ( 'NONE',  ( -37.00000000000000711, 0.000000000000000000, 0.000000000000000000 ) ) ;
#5675=VERTEX_POINT ( 'NONE', #56710 ) ;
#5678=LINE ( 'NONE', #27242, #3083 ) ;
#5680=AXIS2_PLACEMENT_3D ( 'NONE', #51643, #51318, #10388 ) ;
#5682=CARTESIAN_POINT ( 'NONE',  ( 37.00000000000000711, 4.705694406421931860E-17, -3.469127814946512892E-15 ) ) ;
#5683=CARTESIAN_POINT ( 'NONE',  ( -27.27811836728105632, 13.23177170242203537, -2.726413120567312109 ) ) ;
#5684=AXIS2_PLACEMENT_3D ( 'NONE', #33571, #28568, #37578 ) ;
#5685=CARTESIAN_POINT ( 'NONE',  ( 28.79300809604977474, 9.772829246361629529, 6.977156320580031768 ) ) ;
#5686=DIRECTION ( 'NONE',  ( 0.000000000000000000, -1.000000000000000000, 0.000000000000000000 ) ) ;
#5687=EDGE_CURVE ( 'NONE', #48764, #22402, #57267, .T. ) ;
#5688=AXIS2_PLACEMENT_3D ( 'NONE', #12545, #32823, #53133 ) ;
#5690=DIRECTION ( 'NONE',  ( 1.000000000000000000, 0.000000000000000000, 0.000000000000000000 ) ) ;
#5691=ORIENTED_EDGE ( 'NONE', *, *, #19251, .T. ) ;
#5693=AXIS2_PLACEMENT_3D ( 'NONE', #64210, #59227, #24290 ) ;
#5696=DIRECTION ( 'NONE',  ( 0.000000000000000000, -0.01356324068817998940, 0.9999080150203990547 ) ) ;
#5697=ORIENTED_EDGE ( 'NONE', *, *, #32702, .T. ) ;
#5699=DIRECTION ( 'NONE',  ( 1.000000000000000000, 0.000000000000000000, 0.000000000000000000 ) ) ;
#5701=CARTESIAN_POINT ( 'NONE',  ( 22.11934408877570135, -13.40694460789532449, -1.623494447580545952 ) ) ;
#5702=EDGE_CURVE ( 'NONE', #40383, #61423, #31743, .T. ) ;
#5703=AXIS2_PLACEMENT_3D ( 'NONE', #44405, #64687, #45402 ) ;
#5705=CARTESIAN_POINT ( 'NONE',  ( -35.00000000000000000, 8.258652103341553641, -8.352657516904583801 ) ) ;
#5706=CARTESIAN_POINT ( 'NONE',  ( -37.00000000000000711, -11.81949347079749302, 2.968224442958360410 ) ) ;
#5710=VECTOR ( 'NONE', #3422, 1000.000000000000000 ) ;
#5712=EDGE_CURVE ( 'NONE', #29524, #18956, #26442, .T. ) ;
#5716=CYLINDRICAL_SURFACE ( 'NONE', #34302, 4.999999999999999112 ) ;
#5717=CIRCLE ( 'NONE', #16335, 12.18649999999999878 ) ;
#5719=ADVANCED_FACE ( 'NONE', ( #36047 ), #36725, .T. ) ;
#5720=ORIENTED_EDGE ( 'NONE', *, *, #15803, .F. ) ;
#5721=CIRCLE ( 'NONE', #24831, 12.75000000000000178 ) ;
#5722=VERTEX_POINT ( 'NONE', #31718 ) ;
#5724=DIRECTION ( 'NONE',  ( 0.000000000000000000, -0.7790879021242441693, 0.6269146997508066033 ) ) ;
#5725=AXIS2_PLACEMENT_3D ( 'NONE', #488, #41681, #35694 ) ;
#5726=DIRECTION ( 'NONE',  ( 1.000000000000000000, 0.000000000000000000, 0.000000000000000000 ) ) ;
#5729=CARTESIAN_POINT ( 'NONE',  ( -16.98800322446194855, 2.922502605998049674, -11.63868456991314027 ) ) ;
#5731=ORIENTED_EDGE ( 'NONE', *, *, #3226, .F. ) ;
#5738=LINE ( 'NONE', #55614, #16151 ) ;
#5739=EDGE_LOOP ( 'NONE', ( #4009, #36151, #35383, #49915 ) ) ;
#5740=EDGE_CURVE ( 'NONE', #60025, #9428, #48772, .T. ) ;
#5741=CARTESIAN_POINT ( 'NONE',  ( -14.29135464769095520, 7.782112657557433977, 11.03126115115966499 ) ) ;
#5742=ORIENTED_EDGE ( 'NONE', *, *, #47744, .T. ) ;
#5743=CARTESIAN_POINT ( 'NONE',  ( -17.64665465971367553, -7.710886870156880235, 11.08500766144072891 ) ) ;
#5744=DIRECTION ( 'NONE',  ( 1.000000000000000000, -0.000000000000000000, 0.000000000000000000 ) ) ;
#5746=DIRECTION ( 'NONE',  ( 0.000000000000000000, -0.01356324068817992175, 0.9999080150203990547 ) ) ;
#5747=AXIS2_PLACEMENT_3D ( 'NONE', #36547, #7252, #62785 ) ;
#5749=CARTESIAN_POINT ( 'NONE',  ( 8.459648224137296779, 3.953564174085363092, 11.33341040866371863 ) ) ;
#5752=CARTESIAN_POINT ( 'NONE',  ( -18.45105770001609713, 4.180413819594255287, -12.83901097965013349 ) ) ;
#5753=ORIENTED_EDGE ( 'NONE', *, *, #32219, .F. ) ;
#5760=ORIENTED_EDGE ( 'NONE', *, *, #865, .F. ) ;
#5762=AXIS2_PLACEMENT_3D ( 'NONE', #10250, #25896, #30530 ) ;
#5767=CARTESIAN_POINT ( 'NONE',  ( 3.291290029914074378, 8.250315036047103590, -10.68561190601526079 ) ) ;
#5768=ORIENTED_EDGE ( 'NONE', *, *, #23033, .F. ) ;
#5769=CARTESIAN_POINT ( 'NONE',  ( -17.83419946441818027, -9.720786832536937538, -7.036071585506806336 ) ) ;
#5770=CIRCLE ( 'NONE', #16332, 5.000000000000000888 ) ;
#5771=ORIENTED_EDGE ( 'NONE', *, *, #54520, .T. ) ;
#5773=DIRECTION ( 'NONE',  ( 0.000000000000000000, 0.01356324068817998940, -0.9999080150203990547 ) ) ;
#5775=ORIENTED_EDGE ( 'NONE', *, *, #15696, .F. ) ;
#5776=CIRCLE ( 'NONE', #21715, 5.000000000000001776 ) ;
#5778=ADVANCED_FACE ( 'NONE', ( #16764 ), #32051, .T. ) ;
#5783=CARTESIAN_POINT ( 'NONE',  ( 8.437200413559441614, 4.476360154859203355, 25.00000000000000000 ) ) ;
#5788=AXIS2_PLACEMENT_3D ( 'NONE', #13988, #29295, #54587 ) ;
#5789=EDGE_CURVE ( 'NONE', #44959, #12280, #2897, .T. ) ;
#5792=CARTESIAN_POINT ( 'NONE',  ( 17.48646793688874013, -11.52800716181782370, 7.061530710347139639 ) ) ;
#5793=ORIENTED_EDGE ( 'NONE', *, *, #39680, .F. ) ;
#5794=ADVANCED_FACE ( 'NONE', ( #53989 ), #18087, .T. ) ;
#5797=CARTESIAN_POINT ( 'NONE',  ( 35.00000000000000000, 8.551552972817191289, 8.052525312709789773 ) ) ;
#5801=ADVANCED_FACE ( 'NONE', ( #33033 ), #22404, .T. ) ;
#5802=VERTEX_POINT ( 'NONE', #52689 ) ;
#5803=CIRCLE ( 'NONE', #45082, 4.999999999999999112 ) ;
#5804=AXIS2_PLACEMENT_3D ( 'NONE', #15159, #60726, #49768 ) ;
#5805=VERTEX_POINT ( 'NONE', #17438 ) ;
#5808=CARTESIAN_POINT ( 'NONE',  ( 36.00000000000000711, 2.865935305911623487, -12.42372387097883646 ) ) ;
#5809=EDGE_CURVE ( 'NONE', #5144, #42603, #28071, .T. ) ;
#5810=ORIENTED_EDGE ( 'NONE', *, *, #55574, .F. ) ;
#5811=CARTESIAN_POINT ( 'NONE',  ( -37.00000000000000711, 0.000000000000000000, 0.000000000000000000 ) ) ;
#5813=CARTESIAN_POINT ( 'NONE',  ( -47.00000000000000711, 0.000000000000000000, 0.000000000000000000 ) ) ;
#5815=VERTEX_POINT ( 'NONE', #7117 ) ;
#5817=FACE_OUTER_BOUND ( 'NONE', #29716, .T. ) ;
#5818=EDGE_CURVE ( 'NONE', #31374, #47315, #64586, .T. ) ;
#5820=CARTESIAN_POINT ( 'NONE',  ( 24.44290582448688554, -2.844751314854803592, -13.19810646351145067 ) ) ;
#5821=CARTESIAN_POINT ( 'NONE',  ( 37.00000000000000711, 4.705694406421931860E-17, -3.469127814946512892E-15 ) ) ;
#5822=EDGE_LOOP ( 'NONE', ( #12261, #43013, #13208, #15289 ) ) ;
#5824=ORIENTED_EDGE ( 'NONE', *, *, #31609, .F. ) ;
#5825=LINE ( 'NONE', #44697, #23181 ) ;
#5827=ORIENTED_EDGE ( 'NONE', *, *, #30102, .F. ) ;
#5828=CARTESIAN_POINT ( 'NONE',  ( 35.00000000000000000, -0.7008968033239626472, -12.16632754454236576 ) ) ;
#5831=AXIS2_PLACEMENT_3D ( 'NONE', #46120, #63026, #41762 ) ;
#5833=ORIENTED_EDGE ( 'NONE', *, *, #10070, .T. ) ;
#5839=ORIENTED_EDGE ( 'NONE', *, *, #45220, .F. ) ;
#5840=DIRECTION ( 'NONE',  ( 1.000000000000000000, -0.000000000000000000, 0.000000000000000000 ) ) ;
#5841=ORIENTED_EDGE ( 'NONE', *, *, #15074, .T. ) ;
#5843=ORIENTED_EDGE ( 'NONE', *, *, #64538, .F. ) ;
#5844=DIRECTION ( 'NONE',  ( 1.000000000000000000, 0.000000000000000000, -0.000000000000000000 ) ) ;
#5845=DIRECTION ( 'NONE',  ( 0.000000000000000000, 0.3218879778915972878, -0.9467777615094571386 ) ) ;
#5847=CARTESIAN_POINT ( 'NONE',  ( 18.75685862065280674, 1.097595231443926567, 11.95276324670687629 ) ) ;
#5849=LINE ( 'NONE', #46384, #5505 ) ;
#5850=AXIS2_PLACEMENT_3D ( 'NONE', #58017, #50802, #62636 ) ;
#5853=ORIENTED_EDGE ( 'NONE', *, *, #34976, .F. ) ;
#5854=CARTESIAN_POINT ( 'NONE',  ( 35.00000000000000000, -7.561043153948031836, -9.557269938331533154 ) ) ;
#5856=CARTESIAN_POINT ( 'NONE',  ( 35.00000000000000000, 10.07641281632177588, -6.036400161834603928 ) ) ;
#5858=EDGE_CURVE ( 'NONE', #29920, #18553, #11364, .T. ) ;
#5859=CARTESIAN_POINT ( 'NONE',  ( 6.750737678534439290, -5.599118668687368405, 10.61556038268959767 ) ) ;
#5862=AXIS2_PLACEMENT_3D ( 'NONE', #25292, #33711, #24982 ) ;
#5863=CARTESIAN_POINT ( 'NONE',  ( 35.00000000000000000, 4.041347439436019151, 11.02904044024204211 ) ) ;
#5866=ORIENTED_EDGE ( 'NONE', *, *, #15454, .F. ) ;
#5867=VECTOR ( 'NONE', #14614, 1000.000000000000000 ) ;
#5868=FACE_OUTER_BOUND ( 'NONE', #3097, .T. ) ;
#5869=CARTESIAN_POINT ( 'NONE',  ( 35.00000000000000000, 4.705694406421931860E-17, -3.469127814946512892E-15 ) ) ;
#5870=EDGE_CURVE ( 'NONE', #26580, #41890, #53862, .T. ) ;
#5872=EDGE_CURVE ( 'NONE', #29441, #22391, #43206, .T. ) ;
#5873=CARTESIAN_POINT ( 'NONE',  ( -25.57027579282264185, 10.04421752534342893, 6.567951868637986301 ) ) ;
#5874=CARTESIAN_POINT ( 'NONE',  ( 35.00000000000000000, -4.237620530777882699, -11.42599468261427909 ) ) ;
#5876=CARTESIAN_POINT ( 'NONE',  ( -17.57070937885803374, -9.283194252049366213, -9.806837742160563920 ) ) ;
#5877=DIRECTION ( 'NONE',  ( 1.000000000000000000, 0.000000000000000000, 0.000000000000000000 ) ) ;
#5879=ORIENTED_EDGE ( 'NONE', *, *, #33733, .T. ) ;
#5880=CARTESIAN_POINT ( 'NONE',  ( -9.044148139924335084, -12.95551142774388254, -3.795959767731165169 ) ) ;
#5881=CARTESIAN_POINT ( 'NONE',  ( -47.00000000000000711, 0.000000000000000000, 0.000000000000000000 ) ) ;
#5882=CARTESIAN_POINT ( 'NONE',  ( -47.00000000000000711, 0.000000000000000000, 0.000000000000000000 ) ) ;
#5884=DIRECTION ( 'NONE',  ( 0.000000000000000000, 0.6745969609292610247, 0.7381862504171999850 ) ) ;
#5887=AXIS2_PLACEMENT_3D ( 'NONE', #33389, #3148, #53687 ) ;
#5888=CARTESIAN_POINT ( 'NONE',  ( -35.00000000000000000, 11.44858830469740241, -2.627174906296955381 ) ) ;
#5889=EDGE_LOOP ( 'NONE', ( #41201, #38113, #38078, #52769 ) ) ;
#5890=CARTESIAN_POINT ( 'NONE',  ( -37.00000000000000711, -7.718225330433741149, -9.430788938294133672 ) ) ;
#5891=CARTESIAN_POINT ( 'NONE',  ( 32.00000000000000000, 15.00000000000000000, 1.836970198721028406E-15 ) ) ;
#5892=FACE_OUTER_BOUND ( 'NONE', #16686, .T. ) ;
#5894=CARTESIAN_POINT ( 'NONE',  ( -9.684784117213519394, 9.450766871535190461, -7.397823669409496539 ) ) ;
#5896=CYLINDRICAL_SURFACE ( 'NONE', #7955, 3.477897737712717152 ) ;
#5897=CARTESIAN_POINT ( 'NONE',  ( -35.00000000000000000, 10.42955799785328708, -6.303578524886837009 ) ) ;
#5898=VERTEX_POINT ( 'NONE', #9086 ) ;
#5899=LINE ( 'NONE', #45545, #50424 ) ;
#5900=VERTEX_POINT ( 'NONE', #29366 ) ;
#5902=ORIENTED_EDGE ( 'NONE', *, *, #6159, .T. ) ;
#5905=EDGE_CURVE ( 'NONE', #1113, #53238, #3973, .T. ) ;
#5909=EDGE_LOOP ( 'NONE', ( #48183, #29484, #48736, #19623 ) ) ;
#5910=CARTESIAN_POINT ( 'NONE',  ( -37.00000000000000711, 0.000000000000000000, 0.000000000000000000 ) ) ;
#5912=CARTESIAN_POINT ( 'NONE',  ( -24.43643092833920960, -9.282280370820542359, 7.608281883034075932 ) ) ;
#5914=ORIENTED_EDGE ( 'NONE', *, *, #39843, .T. ) ;
#5915=ORIENTED_EDGE ( 'NONE', *, *, #11984, .F. ) ;
#5918=VERTEX_POINT ( 'NONE', #39334 ) ;
#5919=DIRECTION ( 'NONE',  ( -1.000000000000000000, 0.000000000000000000, -0.000000000000000000 ) ) ;
#5927=ORIENTED_EDGE ( 'NONE', *, *, #4458, .F. ) ;
#5928=CARTESIAN_POINT ( 'NONE',  ( 35.00000000000000000, 10.14408668126221613, 5.921969905510239940 ) ) ;
#5929=CARTESIAN_POINT ( 'NONE',  ( -35.00000000000000000, -9.240395740215685549, 7.251710744571544964 ) ) ;
#5930=CYLINDRICAL_SURFACE ( 'NONE', #59322, 12.18650000000000055 ) ;
#5931=DIRECTION ( 'NONE',  ( -1.000000000000000000, 0.000000000000000000, -0.000000000000000000 ) ) ;
#5932=CARTESIAN_POINT ( 'NONE',  ( -2.676156797222403849, 7.839276155712927796, 10.99183054655308389 ) ) ;
#5933=CARTESIAN_POINT ( 'NONE',  ( 35.00000000000000000, -4.041347439435937439, -11.02904044024207764 ) ) ;
#5934=CARTESIAN_POINT ( 'NONE',  ( 37.00000000000000711, -3.511814412392203266, -11.66953048682398730 ) ) ;
#5937=AXIS2_PLACEMENT_3D ( 'NONE', #24555, #60133, #44834 ) ;
#5938=EDGE_CURVE ( 'NONE', #30257, #21056, #64926, .T. ) ;
#5939=ORIENTED_EDGE ( 'NONE', *, *, #25589, .F. ) ;
#5940=DIRECTION ( 'NONE',  ( -1.000000000000000000, -0.000000000000000000, 0.000000000000000000 ) ) ;
#5941=EDGE_CURVE ( 'NONE', #19644, #57557, #8193, .T. ) ;
#5942=ORIENTED_EDGE ( 'NONE', *, *, #49382, .T. ) ;
#5948=CYLINDRICAL_SURFACE ( 'NONE', #47331, 12.74999999999999822 ) ;
#5949=CARTESIAN_POINT ( 'NONE',  ( 36.00000000000000711, 2.080187960898561172, -12.57916205664482412 ) ) ;
#5950=EDGE_CURVE ( 'NONE', #17535, #4846, #14519, .T. ) ;
#5953=CARTESIAN_POINT ( 'NONE',  ( 9.268278201553693307, 6.103558304117178146, -12.04593591654801799 ) ) ;
#5955=ORIENTED_EDGE ( 'NONE', *, *, #2660, .F. ) ;
#5956=FACE_OUTER_BOUND ( 'NONE', #52267, .T. ) ;
#5958=LINE ( 'NONE', #15883, #8963 ) ;
#5959=DIRECTION ( 'NONE',  ( 0.000000000000000000, 0.01356324068817998940, -0.9999080150203990547 ) ) ;
#5960=CARTESIAN_POINT ( 'NONE',  ( 35.00000000000000000, -10.01317267707881165, 6.946017217730044990 ) ) ;
#5961=EDGE_CURVE ( 'NONE', #53475, #46122, #51725, .T. ) ;
#5962=CARTESIAN_POINT ( 'NONE',  ( -30.18541646480309026, -1.416020129149132334, -13.42553116244734746 ) ) ;
#5963=EDGE_CURVE ( 'NONE', #11560, #6736, #88, .T. ) ;
#5964=DIRECTION ( 'NONE',  ( 0.000000000000000000, -0.8827602140260367714, 0.4698238015817268187 ) ) ;
#5965=AXIS2_PLACEMENT_3D ( 'NONE', #25034, #60934, #60593 ) ;
#5969=ORIENTED_EDGE ( 'NONE', *, *, #28704, .F. ) ;
#5970=CARTESIAN_POINT ( 'NONE',  ( -18.04458733766117362, 25.00000000000000000, 3.916728392552376370 ) ) ;
#5971=CARTESIAN_POINT ( 'NONE',  ( 3.115331810559627712, 4.248790708446858133, -12.82013328618461223 ) ) ;
#5972=CARTESIAN_POINT ( 'NONE',  ( -18.04458733766117362, -11.34280559204704097, 3.916728392552376370 ) ) ;
#5975=DIRECTION ( 'NONE',  ( -1.000000000000000000, -1.836970198721029688E-16, -0.000000000000000000 ) ) ;
#5977=ORIENTED_EDGE ( 'NONE', *, *, #6654, .F. ) ;
#5978=B_SPLINE_CURVE_WITH_KNOTS ( 'NONE', 3,
 ( #47311, #5518, #12679, #1752, #37961, #62904, #27016, #58257, #22690, #27649, #526, #20793, #37304, #36059, #51063, #53271 ),
 .UNSPECIFIED., .F., .F.,
 ( 4, 2, 2, 2, 2, 2, 2, 4 ),
 ( 0.000000000000000000, 0.001108109431372354420, 0.002216218862744708841, 0.003324328294117063261, 0.004432437725489417682, 0.006648656588234126523, 0.007756766019606478775, 0.008864875450978831894 ),
 .UNSPECIFIED. ) ;
#5980=ORIENTED_EDGE ( 'NONE', *, *, #27999, .T. ) ;
#5982=CARTESIAN_POINT ( 'NONE',  ( 22.58646936605650168, -11.74531380756754828, -6.665220879160888678 ) ) ;
#5985=ADVANCED_FACE ( 'NONE', ( #26340 ), #21012, .T. ) ;
#5988=ORIENTED_EDGE ( 'NONE', *, *, #64580, .T. ) ;
#5989=LINE ( 'NONE', #20262, #24806 ) ;
#5991=DIRECTION ( 'NONE',  ( 1.000000000000000000, 0.000000000000000000, -0.000000000000000000 ) ) ;
#5992=ORIENTED_EDGE ( 'NONE', *, *, #21176, .F. ) ;
#5994=EDGE_CURVE ( 'NONE', #15359, #63312, #45983, .T. ) ;
#5995=CARTESIAN_POINT ( 'NONE',  ( 36.00000000000000711, 11.24036214326529048, 6.018036132182036368 ) ) ;
#5996=ORIENTED_EDGE ( 'NONE', *, *, #60786, .T. ) ;
#5997=DIRECTION ( 'NONE',  ( 1.000000000000000000, -0.000000000000000000, 0.000000000000000000 ) ) ;
#5998=ORIENTED_EDGE ( 'NONE', *, *, #44285, .T. ) ;
#6000=ORIENTED_EDGE ( 'NONE', *, *, #62112, .F. ) ;
#6002=DIRECTION ( 'NONE',  ( 1.000000000000000000, 0.000000000000000000, -0.000000000000000000 ) ) ;
#6004=CARTESIAN_POINT ( 'NONE',  ( 9.575800908719084958, 11.95193887484099093, -1.072919909436247154 ) ) ;
#6005=FACE_OUTER_BOUND ( 'NONE', #23698, .T. ) ;
#6006=ORIENTED_EDGE ( 'NONE', *, *, #61029, .T. ) ;
#6007=AXIS2_PLACEMENT_3D ( 'NONE', #63284, #53332, #44003 ) ;
#6012=B_SPLINE_CURVE_WITH_KNOTS ( 'NONE', 3,
 ( #24171, #44437, #14188, #65055, #10503, #44772, #15497, #45768, #30149, #60737, #20826, #230, #30779, #40789, #5213, #25158 ),
 .UNSPECIFIED., .F., .F.,
 ( 4, 2, 2, 2, 2, 2, 2, 4 ),
 ( 0.000000000000000000, 0.002138034596868667800, 0.003207051895303000832, 0.004276069193737333865, 0.005345086492171666898, 0.006414103790605999930, 0.007483121089040332963, 0.008552138387474665995 ),
 .UNSPECIFIED. ) ;
#6014=CYLINDRICAL_SURFACE ( 'NONE', #19414, 6.842778212674966554 ) ;
#6016=CARTESIAN_POINT ( 'NONE',  ( 29.08103898107091112, 5.276197063807976484, 10.78770863057103568 ) ) ;
#6019=CARTESIAN_POINT ( 'NONE',  ( -36.00000000000000711, -12.73293890771483028, -0.6593684648221820321 ) ) ;
#6020=EDGE_CURVE ( 'NONE', #61618, #55634, #34023, .T. ) ;
#6021=EDGE_LOOP ( 'NONE', ( #41764, #48451, #50400, #44731 ) ) ;
#6025=DIRECTION ( 'NONE',  ( 0.000000000000000000, 0.01356324068817992175, -0.9999080150203990547 ) ) ;
#6027=VERTEX_POINT ( 'NONE', #55950 ) ;
#6028=PLANE ( 'NONE',  #60048 ) ;
#6029=DIRECTION ( 'NONE',  ( 1.000000000000000000, 0.000000000000000000, 0.000000000000000000 ) ) ;
#6030=CARTESIAN_POINT ( 'NONE',  ( -35.00000000000000000, 12.74921544981111055, -0.1414404973752581562 ) ) ;
#6033=DIRECTION ( 'NONE',  ( 1.000000000000000000, 0.000000000000000000, 0.000000000000000000 ) ) ;
#6037=CARTESIAN_POINT ( 'NONE',  ( -37.00000000000000711, 0.000000000000000000, 0.000000000000000000 ) ) ;
#6038=VECTOR ( 'NONE', #51297, 1000.000000000000000 ) ;
#6039=EDGE_CURVE ( 'NONE', #6851, #58393, #19166, .T. ) ;
#6040=ORIENTED_EDGE ( 'NONE', *, *, #9124, .F. ) ;
#6045=DIRECTION ( 'NONE',  ( 0.000000000000000000, -0.5767582926624852391, -0.8169148498130358593 ) ) ;
#6046=DIRECTION ( 'NONE',  ( -1.000000000000000000, 0.000000000000000000, 0.000000000000000000 ) ) ;
#6048=ORIENTED_EDGE ( 'NONE', *, *, #37551, .F. ) ;
#6049=ORIENTED_EDGE ( 'NONE', *, *, #11391, .F. ) ;
#6050=CARTESIAN_POINT ( 'NONE',  ( 36.00000000000000711, -11.80185301892977279, 4.824807283154243898 ) ) ;
#6052=LINE ( 'NONE', #52588, #40612 ) ;
#6054=FACE_OUTER_BOUND ( 'NONE', #2548, .T. ) ;
#6056=EDGE_LOOP ( 'NONE', ( #36359, #53154, #14270, #22903 ) ) ;
#6057=DIRECTION ( 'NONE',  ( 1.000000000000000000, 0.000000000000000000, 0.000000000000000000 ) ) ;
#6063=CARTESIAN_POINT ( 'NONE',  ( 35.00000000000000000, -0.6593684648219556577, 12.73293890771483383 ) ) ;
#6065=CARTESIAN_POINT ( 'NONE',  ( 35.00000000000000000, -12.46157735505187247, 2.696588552979187536 ) ) ;
#6068=EDGE_CURVE ( 'NONE', #20284, #7532, #61262, .T. ) ;
#6070=LINE ( 'NONE', #56939, #13365 ) ;
#6071=CARTESIAN_POINT ( 'NONE',  ( -35.00000000000000000, -8.496612874013223404, 9.506317355798342916 ) ) ;
#6072=LINE ( 'NONE', #55277, #55880 ) ;
#6074=CARTESIAN_POINT ( 'NONE',  ( 35.00000000000000000, 4.705694406421931860E-17, -3.469127814946512892E-15 ) ) ;
#6076=DIRECTION ( 'NONE',  ( -1.000000000000000000, -0.000000000000000000, 0.000000000000000000 ) ) ;
#6084=VECTOR ( 'NONE', #6002, 1000.000000000000000 ) ;
#6085=DIRECTION ( 'NONE',  ( 1.000000000000000000, -0.000000000000000000, 0.000000000000000000 ) ) ;
#6087=ORIENTED_EDGE ( 'NONE', *, *, #29389, .T. ) ;
#6089=CARTESIAN_POINT ( 'NONE',  ( -17.73204436170163234, -5.329256642071285910, -10.75287752448376644 ) ) ;
#6090=ADVANCED_FACE ( 'NONE', ( #36649 ), #11370, .T. ) ;
#6091=ORIENTED_EDGE ( 'NONE', *, *, #43589, .F. ) ;
#6095=DIRECTION ( 'NONE',  ( 0.9364047569793457759, -0.3509218304786018705, 0.000000000000000000 ) ) ;
#6096=ORIENTED_EDGE ( 'NONE', *, *, #38405, .F. ) ;
#6099=CARTESIAN_POINT ( 'NONE',  ( 29.15566506771730104, 8.541154756424255368, 10.48791489529884480 ) ) ;
#6100=DIRECTION ( 'NONE',  ( -1.000000000000000000, 0.000000000000000000, 0.000000000000000000 ) ) ;
#6101=FACE_OUTER_BOUND ( 'NONE', #35367, .T. ) ;
#6104=ADVANCED_FACE ( 'NONE', ( #63222 ), #63535, .F. ) ;
#6106=DIRECTION ( 'NONE',  ( 0.000000000000000000, -0.9105187689795911643, 0.4134677391718609707 ) ) ;
#6107=VERTEX_POINT ( 'NONE', #62550 ) ;
#6108=CARTESIAN_POINT ( 'NONE',  ( -17.96034788017830053, 6.012426159432092909, 12.08945883540747346 ) ) ;
#6109=CARTESIAN_POINT ( 'NONE',  ( 6.742624838446524826, -7.056336534564969121, 11.51515283083395857 ) ) ;
#6112=CARTESIAN_POINT ( 'NONE',  ( -37.00000000000000711, 0.000000000000000000, 0.000000000000000000 ) ) ;
#6113=CARTESIAN_POINT ( 'NONE',  ( -9.824501563233303258, 11.81955781327371291, -6.534828226117857852 ) ) ;
#6114=EDGE_LOOP ( 'NONE', ( #65729, #58789, #2302, #64270 ) ) ;
#6117=VERTEX_POINT ( 'NONE', #7706 ) ;
#6120=VERTEX_POINT ( 'NONE', #47611 ) ;
#6121=DIRECTION ( 'NONE',  ( 0.000000000000000000, 0.01356324068817998940, -0.9999080150203990547 ) ) ;
#6124=DIRECTION ( 'NONE',  ( 0.000000000000000000, -0.01356324068817998940, 0.9999080150203990547 ) ) ;
#6126=DIRECTION ( 'NONE',  ( -1.000000000000000000, 0.000000000000000000, -0.000000000000000000 ) ) ;
#6127=DIRECTION ( 'NONE',  ( 0.000000000000000000, 0.01356324068817998940, -0.9999080150203990547 ) ) ;
#6131=DIRECTION ( 'NONE',  ( 1.000000000000000000, 0.000000000000000000, -0.000000000000000000 ) ) ;
#6133=VERTEX_POINT ( 'NONE', #27639 ) ;
#6137=ORIENTED_EDGE ( 'NONE', *, *, #9124, .T. ) ;
#6139=DIRECTION ( 'NONE',  ( 0.000000000000000000, -0.7196168960969719919, -0.6943713148249717193 ) ) ;
#6141=DIRECTION ( 'NONE',  ( 0.000000000000000000, -0.01356324068817997726, 0.9999080150203990547 ) ) ;
#6144=CARTESIAN_POINT ( 'NONE',  ( 47.00000000000000711, 4.705694406421931860E-17, -3.469127814946512892E-15 ) ) ;
#6146=CARTESIAN_POINT ( 'NONE',  ( 36.00000000000000711, 12.70128625845192794, -1.113475361586537593 ) ) ;
#6147=ORIENTED_EDGE ( 'NONE', *, *, #42387, .F. ) ;
#6148=ORIENTED_EDGE ( 'NONE', *, *, #64302, .F. ) ;
#6149=DIRECTION ( 'NONE',  ( -1.000000000000000000, 0.000000000000000000, 0.000000000000000000 ) ) ;
#6151=ORIENTED_EDGE ( 'NONE', *, *, #55702, .T. ) ;
#6152=DIRECTION ( 'NONE',  ( -0.5244426074294280538, 0.000000000000000000, 0.8514458006899926490 ) ) ;
#6153=CARTESIAN_POINT ( 'NONE',  ( -37.00000000000000711, 0.000000000000000000, 0.000000000000000000 ) ) ;
#6154=CARTESIAN_POINT ( 'NONE',  ( -37.00000000000000711, 0.000000000000000000, 0.000000000000000000 ) ) ;
#6156=DIRECTION ( 'NONE',  ( 0.000000000000000000, 0.9796553971857736576, 0.2006870767258926158 ) ) ;
#6157=VECTOR ( 'NONE', #55859, 1000.000000000000000 ) ;
#6159=EDGE_CURVE ( 'NONE', #47988, #9409, #45703, .T. ) ;
#6160=DIRECTION ( 'NONE',  ( 0.000000000000000000, -0.01356324068817999114, 0.9999080150203989437 ) ) ;
#6161=CIRCLE ( 'NONE', #45430, 12.74999999999999822 ) ;
#6163=ORIENTED_EDGE ( 'NONE', *, *, #39496, .F. ) ;
#6166=CARTESIAN_POINT ( 'NONE',  ( 35.00000000000000000, -0.7214809346829402781, -11.72397916322012179 ) ) ;
#6167=CIRCLE ( 'NONE', #31625, 5.000000000000002665 ) ;
#6170=AXIS2_PLACEMENT_3D ( 'NONE', #40457, #14841, #60757 ) ;
#6171=EDGE_CURVE ( 'NONE', #40578, #37945, #5366, .T. ) ;
#6172=CARTESIAN_POINT ( 'NONE',  ( 24.17999985073118197, -2.133694974929364552, -13.33140535122455717 ) ) ;
#6173=ADVANCED_FACE ( 'NONE', ( #44908 ), #4028, .T. ) ;
#6174=CARTESIAN_POINT ( 'NONE',  ( 3.334832302356885769, 3.396901620706510361, -11.51108694095134766 ) ) ;
#6175=CARTESIAN_POINT ( 'NONE',  ( 8.553052268354708332, 3.426888109790365622, -11.50363822801515568 ) ) ;
#6176=ORIENTED_EDGE ( 'NONE', *, *, #55728, .F. ) ;
#6177=CARTESIAN_POINT ( 'NONE',  ( -37.00000000000000711, 0.000000000000000000, 0.000000000000000000 ) ) ;
#6179=CARTESIAN_POINT ( 'NONE',  ( -35.00000000000000000, 9.913596905230113165, 8.017674001891819557 ) ) ;
#6181=EDGE_CURVE ( 'NONE', #31335, #25218, #42503, .T. ) ;
#6186=CARTESIAN_POINT ( 'NONE',  ( 37.00000000000000711, 9.196955404009292678, -8.830544224262981245 ) ) ;
#6188=EDGE_CURVE ( 'NONE', #59781, #37175, #59520, .T. ) ;
#6191=DIRECTION ( 'NONE',  ( 0.000000000000000000, -0.01356324068817998940, 0.9999080150203990547 ) ) ;
#6193=CYLINDRICAL_SURFACE ( 'NONE', #40253, 12.18649999999999878 ) ;
#6194=EDGE_LOOP ( 'NONE', ( #60636, #17466, #7603, #31172 ) ) ;
#6196=DIRECTION ( 'NONE',  ( 1.000000000000000000, 0.000000000000000000, -0.000000000000000000 ) ) ;
#6197=ORIENTED_EDGE ( 'NONE', *, *, #39819, .T. ) ;
#6199=CARTESIAN_POINT ( 'NONE',  ( 37.00000000000000711, 4.705694406421931860E-17, -3.469127814946512892E-15 ) ) ;
#6200=CIRCLE ( 'NONE', #40153, 5.000000000000002665 ) ;
#6201=CARTESIAN_POINT ( 'NONE',  ( 23.57323689665027544, 1.992445679240424150, -11.83683888636838333 ) ) ;
#6202=CARTESIAN_POINT ( 'NONE',  ( -3.992345480360331766, -11.80960273735984600, 6.553217067094195158 ) ) ;
#6203=CARTESIAN_POINT ( 'NONE',  ( 26.25882823526612597, 13.04980996862090947, 3.460358416528618086 ) ) ;
#6206=ORIENTED_EDGE ( 'NONE', *, *, #65639, .T. ) ;
#6207=CIRCLE ( 'NONE', #9347, 5.000000000000002665 ) ;
#6209=CARTESIAN_POINT ( 'NONE',  ( -29.76531599071173062, -3.714239038275569449, 12.97905452356682865 ) ) ;
#6211=DIRECTION ( 'NONE',  ( 0.000000000000000000, -0.01356324068817998940, 0.9999080150203990547 ) ) ;
#6212=CARTESIAN_POINT ( 'NONE',  ( -18.08686583997218733, 4.947294784127231893, 10.93504697000629911 ) ) ;
#6214=DIRECTION ( 'NONE',  ( 0.000000000000000000, -0.1740410799127470320, -0.9847383929261643853 ) ) ;
#6217=( BOUNDED_CURVE ( )  B_SPLINE_CURVE ( 3, ( #56940, #42248, #37624, #46300 ),
 .UNSPECIFIED., .F., .F. ) 
 B_SPLINE_CURVE_WITH_KNOTS ( ( 4, 4 ),
 ( 0.8821975705743981822, 0.9242421917074130633 ),
 .UNSPECIFIED. ) 
 CURVE ( )  GEOMETRIC_REPRESENTATION_ITEM ( )  RATIONAL_B_SPLINE_CURVE ( ( 1.000000000000000000, 0.9998526929113126238, 0.9998526929113126238, 1.000000000000000000 ) ) 
 REPRESENTATION_ITEM ( '' )  );
#6219=DIRECTION ( 'NONE',  ( 0.000000000000000000, -1.000000000000000000, 0.000000000000000000 ) ) ;
#6221=VERTEX_POINT ( 'NONE', #64521 ) ;
#6225=LINE ( 'NONE', #5581, #33781 ) ;
#6227=DIRECTION ( 'NONE',  ( 1.000000000000000000, 0.000000000000000000, 0.000000000000000000 ) ) ;
#6228=DIRECTION ( 'NONE',  ( -1.000000000000000000, 0.000000000000000000, -0.000000000000000000 ) ) ;
#6229=DIRECTION ( 'NONE',  ( 0.000000000000000000, -0.01356324068817999114, 0.9999080150203989437 ) ) ;
#6230=DIRECTION ( 'NONE',  ( 0.000000000000000000, 0.6478160128811893959, -0.7617968321374923857 ) ) ;
#6232=FACE_OUTER_BOUND ( 'NONE', #38088, .T. ) ;
#6233=ORIENTED_EDGE ( 'NONE', *, *, #40531, .F. ) ;
#6234=CARTESIAN_POINT ( 'NONE',  ( 35.00000000000000000, 4.705694406421931860E-17, -3.469127814946512892E-15 ) ) ;
#6235=CIRCLE ( 'NONE', #23219, 12.18650000000000411 ) ;
#6236=DIRECTION ( 'NONE',  ( -1.000000000000000000, 0.000000000000000000, 0.000000000000000000 ) ) ;
#6237=EDGE_CURVE ( 'NONE', #24509, #33400, #58371, .T. ) ;
#6238=CARTESIAN_POINT ( 'NONE',  ( 35.00000000000000000, -11.37311665002365579, -2.936739658819832677 ) ) ;
#6240=CARTESIAN_POINT ( 'NONE',  ( -35.00000000000000000, 8.551552972817082932, 8.052525312709914118 ) ) ;
#6241=DIRECTION ( 'NONE',  ( -1.000000000000000000, -0.000000000000000000, -0.000000000000000000 ) ) ;
#6242=VECTOR ( 'NONE', #26711, 1000.000000000000000 ) ;
#6243=ORIENTED_EDGE ( 'NONE', *, *, #62896, .F. ) ;
#6246=VECTOR ( 'NONE', #53938, 1000.000000000000000 ) ;
#6250=ADVANCED_FACE ( 'NONE', ( #14315 ), #54890, .T. ) ;
#6251=CARTESIAN_POINT ( 'NONE',  ( -15.93470253878248322, 7.893290767330796598, -10.95207400281732113 ) ) ;
#6252=AXIS2_PLACEMENT_3D ( 'NONE', #12661, #53255, #54580 ) ;
#6254=DIRECTION ( 'NONE',  ( 1.000000000000000000, 0.000000000000000000, 0.000000000000000000 ) ) ;
#6255=EDGE_CURVE ( 'NONE', #60004, #1502, #43154, .T. ) ;
#6256=ORIENTED_EDGE ( 'NONE', *, *, #54436, .T. ) ;
#6258=DIRECTION ( 'NONE',  ( 0.000000000000000000, 0.01356324068817998940, -0.9999080150203990547 ) ) ;
#6260=CIRCLE ( 'NONE', #42284, 5.000000000000001776 ) ;
#6263=EDGE_CURVE ( 'NONE', #53784, #4915, #40571, .T. ) ;
#6267=EDGE_LOOP ( 'NONE', ( #60858, #4504, #29415, #39487 ) ) ;
#6268=CARTESIAN_POINT ( 'NONE',  ( -37.00000000000000711, 0.000000000000000000, 0.000000000000000000 ) ) ;
#6269=EDGE_CURVE ( 'NONE', #35192, #12635, #20940, .T. ) ;
#6271=CARTESIAN_POINT ( 'NONE',  ( -2.532614230583026593, -7.965877694534051479, 10.89930238848911337 ) ) ;
#6272=CYLINDRICAL_SURFACE ( 'NONE', #41579, 5.000000000000000888 ) ;
#6274=CARTESIAN_POINT ( 'NONE',  ( 28.91057078075369802, -9.499749482217620056, 7.335151099638228978 ) ) ;
#6275=CARTESIAN_POINT ( 'NONE',  ( -4.975205859172452172, -1.416020129149132778, 11.91616074890920451 ) ) ;
#6276=CIRCLE ( 'NONE', #43416, 12.75000000000000178 ) ;
#6277=ORIENTED_EDGE ( 'NONE', *, *, #4876, .T. ) ;
#6278=ORIENTED_EDGE ( 'NONE', *, *, #50608, .T. ) ;
#6279=CARTESIAN_POINT ( 'NONE',  ( 35.00000000000000000, 11.37311665002363270, 2.936739658819908616 ) ) ;
#6280=ORIENTED_EDGE ( 'NONE', *, *, #60352, .T. ) ;
#6288=VERTEX_POINT ( 'NONE', #26271 ) ;
#6290=ORIENTED_EDGE ( 'NONE', *, *, #592, .F. ) ;
#6291=DIRECTION ( 'NONE',  ( -1.000000000000000000, 0.000000000000000000, -0.000000000000000000 ) ) ;
#6292=CARTESIAN_POINT ( 'NONE',  ( 17.31227647733753017, 10.56962781760056380, 8.406781232797083447 ) ) ;
#6293=EDGE_CURVE ( 'NONE', #52168, #28250, #17478, .T. ) ;
#6295=CYLINDRICAL_SURFACE ( 'NONE', #42554, 12.75000000000000178 ) ;
#6296=AXIS2_PLACEMENT_3D ( 'NONE', #54839, #4296, #31516 ) ;
#6297=ORIENTED_EDGE ( 'NONE', *, *, #49771, .F. ) ;
#6300=DIRECTION ( 'NONE',  ( -1.000000000000000000, 0.000000000000000000, 0.000000000000000000 ) ) ;
#6301=EDGE_LOOP ( 'NONE', ( #17092, #1236, #14500, #25660 ) ) ;
#6304=VERTEX_POINT ( 'NONE', #26589 ) ;
#6305=CARTESIAN_POINT ( 'NONE',  ( 12.52750123246316072, 0.4973700281276248192, 25.00000000000000000 ) ) ;
#6306=VERTEX_POINT ( 'NONE', #30917 ) ;
#6308=ORIENTED_EDGE ( 'NONE', *, *, #59465, .F. ) ;
#6309=AXIS2_PLACEMENT_3D ( 'NONE', #17448, #37722, #7445 ) ;
#6310=ORIENTED_EDGE ( 'NONE', *, *, #26584, .F. ) ;
#6313=DIRECTION ( 'NONE',  ( -1.000000000000000000, 0.000000000000000000, 0.000000000000000000 ) ) ;
#6315=CARTESIAN_POINT ( 'NONE',  ( -37.00000000000000711, 11.47758908105694786, 2.497432891016883261 ) ) ;
#6316=ORIENTED_EDGE ( 'NONE', *, *, #49829, .T. ) ;
#6317=CARTESIAN_POINT ( 'NONE',  ( -35.00000000000000000, -4.400442035671030538, 11.96656215839367299 ) ) ;
#6318=EDGE_LOOP ( 'NONE', ( #58486, #15188, #7829, #17643 ) ) ;
#6319=CARTESIAN_POINT ( 'NONE',  ( -29.43980975494970309, -3.641506875706034041, -12.99959336572439561 ) ) ;
#6322=EDGE_CURVE ( 'NONE', #62732, #63634, #42960, .T. ) ;
#6327=AXIS2_PLACEMENT_3D ( 'NONE', #44494, #34531, #18925 ) ;
#6329=AXIS2_PLACEMENT_3D ( 'NONE', #35655, #26028, #437 ) ;
#6330=ORIENTED_EDGE ( 'NONE', *, *, #53074, .F. ) ;
#6335=DIRECTION ( 'NONE',  ( -1.000000000000000000, 0.000000000000000000, -0.000000000000000000 ) ) ;
#6340=CARTESIAN_POINT ( 'NONE',  ( 21.94561096463932870, -13.06103434740021108, -3.434726814316783727 ) ) ;
#6342=EDGE_CURVE ( 'NONE', #62669, #50699, #16298, .T. ) ;
#6343=VECTOR ( 'NONE', #42, 1000.000000000000000 ) ;
#6345=CARTESIAN_POINT ( 'NONE',  ( -37.00000000000000711, 0.000000000000000000, 0.000000000000000000 ) ) ;
#6346=CYLINDRICAL_SURFACE ( 'NONE', #42366, 5.000000000000000888 ) ;
#6348=DIRECTION ( 'NONE',  ( 1.000000000000000000, 0.000000000000000000, 0.000000000000000000 ) ) ;
#6350=DIRECTION ( 'NONE',  ( 1.000000000000000000, 0.000000000000000000, 0.000000000000000000 ) ) ;
#6351=AXIS2_PLACEMENT_3D ( 'NONE', #57578, #11997, #32279 ) ;
#6352=ADVANCED_FACE ( 'NONE', ( #22597 ), #27248, .T. ) ;
#6353=ORIENTED_EDGE ( 'NONE', *, *, #19207, .T. ) ;
#6354=ORIENTED_EDGE ( 'NONE', *, *, #52931, .T. ) ;
#6357=FACE_OUTER_BOUND ( 'NONE', #10917, .T. ) ;
#6358=CARTESIAN_POINT ( 'NONE',  ( 36.00000000000000711, 12.54989509947654192, 2.250029553613614564 ) ) ;
#6359=ORIENTED_EDGE ( 'NONE', *, *, #37005, .F. ) ;
#6360=EDGE_LOOP ( 'NONE', ( #35528, #26225, #10770, #8747 ) ) ;
#6361=ORIENTED_EDGE ( 'NONE', *, *, #15168, .F. ) ;
#6364=DIRECTION ( 'NONE',  ( -1.000000000000000000, 0.000000000000000000, 0.000000000000000000 ) ) ;
#6367=CARTESIAN_POINT ( 'NONE',  ( -37.00000000000000711, -12.74921544981111055, 0.1414404973751688388 ) ) ;
#6369=ADVANCED_FACE ( 'NONE', ( #32538 ), #32868, .T. ) ;
#6370=EDGE_LOOP ( 'NONE', ( #16511, #54228, #48420, #61154 ) ) ;
#6371=CARTESIAN_POINT ( 'NONE',  ( 19.67311005600952711, -0.7004819783312107306, 25.00000000000000000 ) ) ;
#6374=CARTESIAN_POINT ( 'NONE',  ( 24.17672931252117152, -3.380230056746429401, 11.51978025207018241 ) ) ;
#6375=ORIENTED_EDGE ( 'NONE', *, *, #29339, .T. ) ;
#6377=EDGE_LOOP ( 'NONE', ( #60681, #56289, #4877, #8261 ) ) ;
#6378=DIRECTION ( 'NONE',  ( 1.000000000000000000, 0.000000000000000000, -0.000000000000000000 ) ) ;
#6382=CARTESIAN_POINT ( 'NONE',  ( -37.00000000000000711, 0.000000000000000000, 0.000000000000000000 ) ) ;
#6384=LINE ( 'NONE', #31956, #3271 ) ;
#6387=ORIENTED_EDGE ( 'NONE', *, *, #36887, .F. ) ;
#6389=ORIENTED_EDGE ( 'NONE', *, *, #65123, .T. ) ;
#6390=CARTESIAN_POINT ( 'NONE',  ( -35.00000000000000000, 0.000000000000000000, 0.000000000000000000 ) ) ;
#6392=EDGE_CURVE ( 'NONE', #46044, #57324, #23579, .T. ) ;
#6394=VERTEX_POINT ( 'NONE', #57525 ) ;
#6397=VECTOR ( 'NONE', #35220, 1000.000000000000000 ) ;
#6400=EDGE_CURVE ( 'NONE', #38220, #46560, #19126, .T. ) ;
#6403=CARTESIAN_POINT ( 'NONE',  ( -37.00000000000000711, -6.475373545682229448, -10.32377448871674908 ) ) ;
#6404=ORIENTED_EDGE ( 'NONE', *, *, #44870, .F. ) ;
#6405=DIRECTION ( 'NONE',  ( 0.000000000000000000, -1.000000000000000000, 0.000000000000000000 ) ) ;
#6406=FACE_OUTER_BOUND ( 'NONE', #18161, .T. ) ;
#6407=CARTESIAN_POINT ( 'NONE',  ( 35.00000000000000000, 5.865551165831078606, -11.32068061209297483 ) ) ;
#6408=EDGE_LOOP ( 'NONE', ( #48471, #63028, #59772, #24919 ) ) ;
#6410=ADVANCED_FACE ( 'NONE', ( #6974 ), #37558, .T. ) ;
#6412=CIRCLE ( 'NONE', #52068, 12.18650000000000055 ) ;
#6413=AXIS2_PLACEMENT_3D ( 'NONE', #48306, #3404, #23013 ) ;
#6418=DIRECTION ( 'NONE',  ( 0.000000000000000000, -0.7790879021242573810, 0.6269146997507903940 ) ) ;
#6419=DIRECTION ( 'NONE',  ( 1.000000000000000000, 0.000000000000000000, 0.000000000000000000 ) ) ;
#6420=CARTESIAN_POINT ( 'NONE',  ( 35.00000000000000000, -11.98254675519226531, 2.220215194442026974 ) ) ;
#6423=CIRCLE ( 'NONE', #10673, 12.74999999999999822 ) ;
#6424=ORIENTED_EDGE ( 'NONE', *, *, #28011, .T. ) ;
#6425=CARTESIAN_POINT ( 'NONE',  ( -17.29810829516095794, 7.115115252187681705, 11.47444202231375598 ) ) ;
#6426=DIRECTION ( 'NONE',  ( -1.000000000000000000, -0.000000000000000000, -0.000000000000000000 ) ) ;
#6427=AXIS2_PLACEMENT_3D ( 'NONE', #51328, #452, #16392 ) ;
#6429=CARTESIAN_POINT ( 'NONE',  ( 35.00000000000000000, 4.705694406421931860E-17, -3.469127814946512892E-15 ) ) ;
#6430=CARTESIAN_POINT ( 'NONE',  ( -37.00000000000000711, 10.84030624090606665, 6.711949091238182064 ) ) ;
#6431=VERTEX_POINT ( 'NONE', #32229 ) ;
#6433=ORIENTED_EDGE ( 'NONE', *, *, #57835, .F. ) ;
#6434=AXIS2_PLACEMENT_3D ( 'NONE', #62228, #31324, #51625 ) ;
#6436=ORIENTED_EDGE ( 'NONE', *, *, #27493, .T. ) ;
#6438=CARTESIAN_POINT ( 'NONE',  ( 35.00000000000000000, 4.705694406421931860E-17, -3.469127814946512892E-15 ) ) ;
#6439=ORIENTED_EDGE ( 'NONE', *, *, #1389, .T. ) ;
#6440=CARTESIAN_POINT ( 'NONE',  ( -24.90381799016406461, -9.122167393312837547, 7.798732004451876421 ) ) ;
#6442=CARTESIAN_POINT ( 'NONE',  ( -35.00000000000000000, -6.303578524886872536, -10.42955799785326576 ) ) ;
#6443=CARTESIAN_POINT ( 'NONE',  ( 35.00000000000000000, 4.705694406421931860E-17, -3.469127814946512892E-15 ) ) ;
#6444=EDGE_CURVE ( 'NONE', #29772, #43237, #17616, .T. ) ;
#6445=ORIENTED_EDGE ( 'NONE', *, *, #57163, .F. ) ;
#6446=CARTESIAN_POINT ( 'NONE',  ( 35.00000000000000000, -2.021542716731485001, -12.01765980939841327 ) ) ;
#6450=ORIENTED_EDGE ( 'NONE', *, *, #32469, .T. ) ;
#6451=CARTESIAN_POINT ( 'NONE',  ( -18.04458733766117362, -12.91933584589293282, 3.916728392552376370 ) ) ;
#6452=AXIS2_PLACEMENT_3D ( 'NONE', #65057, #4898, #15178 ) ;
#6456=LINE ( 'NONE', #27067, #46454 ) ;
#6457=DIRECTION ( 'NONE',  ( 1.000000000000000000, 0.000000000000000000, 0.000000000000000000 ) ) ;
#6459=CIRCLE ( 'NONE', #42500, 12.75000000000000178 ) ;
#6460=ORIENTED_EDGE ( 'NONE', *, *, #30627, .T. ) ;
#6461=EDGE_CURVE ( 'NONE', #24932, #63728, #12695, .T. ) ;
#6463=CIRCLE ( 'NONE', #10717, 12.74999999999999822 ) ;
#6466=EDGE_LOOP ( 'NONE', ( #4599, #38624, #19733, #38902 ) ) ;
#6468=CYLINDRICAL_SURFACE ( 'NONE', #47589, 5.000000000000000888 ) ;
#6469=ORIENTED_EDGE ( 'NONE', *, *, #43077, .T. ) ;
#6470=EDGE_CURVE ( 'NONE', #22718, #19643, #49895, .T. ) ;
#6471=ORIENTED_EDGE ( 'NONE', *, *, #50608, .F. ) ;
#6472=CARTESIAN_POINT ( 'NONE',  ( 37.00000000000000711, 4.705694406421931860E-17, -3.469127814946512892E-15 ) ) ;
#6474=CARTESIAN_POINT ( 'NONE',  ( 35.00000000000000000, 7.817610399097634222, 8.766823244861901898 ) ) ;
#6476=CARTESIAN_POINT ( 'NONE',  ( -37.00000000000000711, 10.49591321039680736, 5.273331777780375873 ) ) ;
#6477=AXIS2_PLACEMENT_3D ( 'NONE', #52821, #63122, #28520 ) ;
#6478=VECTOR ( 'NONE', #65290, 1000.000000000000000 ) ;
#6480=CARTESIAN_POINT ( 'NONE',  ( 29.51976981715666781, 25.00000000000000000, 11.09513982864076276 ) ) ;
#6481=CIRCLE ( 'NONE', #40436, 12.75000000000000178 ) ;
#6482=CIRCLE ( 'NONE', #26637, 12.75000000000000178 ) ;
#6483=ORIENTED_EDGE ( 'NONE', *, *, #29079, .T. ) ;
#6485=CARTESIAN_POINT ( 'NONE',  ( -3.161163348754353120, -5.207994443204945867, 10.84706555580636511 ) ) ;
#6486=AXIS2_PLACEMENT_3D ( 'NONE', #31253, #16284, #16614 ) ;
#6487=B_SPLINE_CURVE_WITH_KNOTS ( 'NONE', 3,
 ( #15062, #15708, #10733, #36333 ),
 .UNSPECIFIED., .F., .F.,
 ( 4, 4 ),
 ( 5.898697549827394244E-18, 0.002289549871878519133 ),
 .UNSPECIFIED. ) ;
#6492=CARTESIAN_POINT ( 'NONE',  ( 37.00000000000000711, 5.644643009979216863, 10.30098186818242922 ) ) ;
#6493=CIRCLE ( 'NONE', #58532, 12.75000000000000178 ) ;
#6496=ADVANCED_FACE ( 'NONE', ( #38533 ), #58168, .T. ) ;
#6497=CARTESIAN_POINT ( 'NONE',  ( 35.00000000000000000, 2.250029553613756228, -12.54989509947652060 ) ) ;
#6499=CARTESIAN_POINT ( 'NONE',  ( -18.24403761432370175, -13.49999999999999822, 0.6264592723685493691 ) ) ;
#6501=AXIS2_PLACEMENT_3D ( 'NONE', #7131, #17454, #23091 ) ;
#6502=AXIS2_PLACEMENT_3D ( 'NONE', #42448, #26524, #56820 ) ;
#6504=CARTESIAN_POINT ( 'NONE',  ( -25.10029369095171248, -9.207521581778740583, 9.878167689217567826 ) ) ;
#6505=ORIENTED_EDGE ( 'NONE', *, *, #2299, .T. ) ;
#6507=CARTESIAN_POINT ( 'NONE',  ( 35.00000000000000000, 4.705694406421931860E-17, -3.469127814946512892E-15 ) ) ;
#6510=DIRECTION ( 'NONE',  ( -1.000000000000000000, 0.000000000000000000, -0.000000000000000000 ) ) ;
#6511=DIRECTION ( 'NONE',  ( 0.000000000000000000, 0.01356324068817998940, -0.9999080150203990547 ) ) ;
#6514=ORIENTED_EDGE ( 'NONE', *, *, #20659, .T. ) ;
#6515=DIRECTION ( 'NONE',  ( 0.000000000000000000, -0.01356324068817998940, 0.9999080150203990547 ) ) ;
#6516=EDGE_CURVE ( 'NONE', #44564, #32447, #33217, .T. ) ;
#6517=CARTESIAN_POINT ( 'NONE',  ( 32.00000000000000000, 15.00000000000000000, 0.000000000000000000 ) ) ;
#6518=ORIENTED_EDGE ( 'NONE', *, *, #31940, .T. ) ;
#6519=CIRCLE ( 'NONE', #19243, 5.000000000000000888 ) ;
#6520=CYLINDRICAL_SURFACE ( 'NONE', #12082, 4.999999999999999112 ) ;
#6521=DIRECTION ( 'NONE',  ( -1.000000000000000000, 0.000000000000000000, -0.000000000000000000 ) ) ;
#6522=DIRECTION ( 'NONE',  ( 1.000000000000000000, -0.000000000000000000, 0.000000000000000000 ) ) ;
#6523=CARTESIAN_POINT ( 'NONE',  ( -35.00000000000000000, 0.000000000000000000, 0.000000000000000000 ) ) ;
#6525=DIRECTION ( 'NONE',  ( 0.8386510381079236298, 0.5446691071471760903, -0.000000000000000000 ) ) ;
#6528=CARTESIAN_POINT ( 'NONE',  ( -10.95212338237647920, -9.902220863987562183, 9.175839033069923545 ) ) ;
#6530=VERTEX_POINT ( 'NONE', #44175 ) ;
#6532=ORIENTED_EDGE ( 'NONE', *, *, #28608, .T. ) ;
#6533=CARTESIAN_POINT ( 'NONE',  ( -29.92777678363736626, -3.750539801530011985, 12.96855624952674724 ) ) ;
#6534=AXIS2_PLACEMENT_3D ( 'NONE', #34176, #65407, #49504 ) ;
#6535=VERTEX_POINT ( 'NONE', #13894 ) ;
#6537=FACE_OUTER_BOUND ( 'NONE', #7933, .T. ) ;
#6540=FACE_OUTER_BOUND ( 'NONE', #63246, .T. ) ;
#6542=AXIS2_PLACEMENT_3D ( 'NONE', #3636, #38854, #48841 ) ;
#6544=LINE ( 'NONE', #11834, #34666 ) ;
#6545=FACE_BOUND ( 'NONE', #27766, .T. ) ;
#6546=EDGE_CURVE ( 'NONE', #3310, #56510, #10517, .T. ) ;
#6547=VERTEX_POINT ( 'NONE', #23581 ) ;
#6550=CIRCLE ( 'NONE', #5515, 4.999999999999998224 ) ;
#6551=AXIS2_PLACEMENT_3D ( 'NONE', #15084, #55669, #10752 ) ;
#6553=CARTESIAN_POINT ( 'NONE',  ( 35.00000000000000000, 4.705694406421931860E-17, -3.469127814946512892E-15 ) ) ;
#6554=CARTESIAN_POINT ( 'NONE',  ( 29.03457606387295087, -4.854210015632035358, 10.97436308512422265 ) ) ;
#6556=DIRECTION ( 'NONE',  ( 1.000000000000000000, 0.000000000000000000, 0.000000000000000000 ) ) ;
#6558=AXIS2_PLACEMENT_3D ( 'NONE', #34546, #20236, #59500 ) ;
#6559=CIRCLE ( 'NONE', #19328, 12.18649999999999878 ) ;
#6560=CARTESIAN_POINT ( 'NONE',  ( -35.00000000000000000, 0.000000000000000000, 0.000000000000000000 ) ) ;
#6563=ADVANCED_FACE ( 'NONE', ( #38867 ), #13573, .T. ) ;
#6564=CARTESIAN_POINT ( 'NONE',  ( -36.00000000000000711, 7.094637218249359556, 10.59380114696472752 ) ) ;
#6565=ORIENTED_EDGE ( 'NONE', *, *, #26283, .F. ) ;
#6567=ORIENTED_EDGE ( 'NONE', *, *, #48177, .F. ) ;
#6569=DIRECTION ( 'NONE',  ( 0.000000000000000000, -0.4380125133593849029, 0.8989688749565220016 ) ) ;
#6570=CARTESIAN_POINT ( 'NONE',  ( -9.146844076892975295, 9.365293060442926532, -7.512015364276853013 ) ) ;
#6571=CARTESIAN_POINT ( 'NONE',  ( 37.00000000000000711, -11.50504120060945823, -4.018060380616357286 ) ) ;
#6573=CARTESIAN_POINT ( 'NONE',  ( -27.45775109278351067, -11.83395752356219255, -1.989333891161980894 ) ) ;
#6574=AXIS2_PLACEMENT_3D ( 'NONE', #12817, #59062, #33753 ) ;
#6575=EDGE_LOOP ( 'NONE', ( #34657, #51216 ) ) ;
#6576=CIRCLE ( 'NONE', #64972, 12.75000000000000178 ) ;
#6577=ORIENTED_EDGE ( 'NONE', *, *, #63735, .T. ) ;
#6579=AXIS2_PLACEMENT_3D ( 'NONE', #22861, #18192, #63711 ) ;
#6581=DIRECTION ( 'NONE',  ( 0.000000000000000000, 0.9903235168508545128, 0.1387779952735854194 ) ) ;
#6582=DIRECTION ( 'NONE',  ( -1.000000000000000000, -0.000000000000000000, 0.000000000000000000 ) ) ;
#6583=VECTOR ( 'NONE', #17415, 1000.000000000000000 ) ;
#6584=CARTESIAN_POINT ( 'NONE',  ( -37.00000000000000711, 11.16627499335650242, 3.645068577060221582 ) ) ;
#6586=VERTEX_POINT ( 'NONE', #15852 ) ;
#6588=DIRECTION ( 'NONE',  ( 0.000000000000000000, 0.9903235168508555120, 0.1387779952735781475 ) ) ;
#6589=CIRCLE ( 'NONE', #43733, 5.000000000000000000 ) ;
#6592=EDGE_CURVE ( 'NONE', #20113, #21123, #34996, .T. ) ;
#6595=CARTESIAN_POINT ( 'NONE',  ( -17.29244623348158783, 2.525873743887551814, -11.73115347397429176 ) ) ;
#6596=ORIENTED_EDGE ( 'NONE', *, *, #14140, .F. ) ;
#6598=ORIENTED_EDGE ( 'NONE', *, *, #56982, .T. ) ;
#6599=DIRECTION ( 'NONE',  ( 0.000000000000000000, 0.5987040770935622147, -0.8009703041134208501 ) ) ;
#6600=CARTESIAN_POINT ( 'NONE',  ( -37.00000000000000711, 0.000000000000000000, 0.000000000000000000 ) ) ;
#6601=DIRECTION ( 'NONE',  ( 0.000000000000000000, 0.01356324068817998940, -0.9999080150203990547 ) ) ;
#6602=VECTOR ( 'NONE', #62682, 1000.000000000000000 ) ;
#6603=CARTESIAN_POINT ( 'NONE',  ( -6.606501376987225171, -1.681841871581811088, 11.88175788702164404 ) ) ;
#6605=CIRCLE ( 'NONE', #245, 12.18650000000000055 ) ;
#6606=AXIS2_PLACEMENT_3D ( 'NONE', #40147, #29522, #9907 ) ;
#6608=ORIENTED_EDGE ( 'NONE', *, *, #22629, .T. ) ;
#6610=LINE ( 'NONE', #60816, #12717 ) ;
#6611=VERTEX_POINT ( 'NONE', #35804 ) ;
#6612=LINE ( 'NONE', #16583, #3295 ) ;
#6615=DIRECTION ( 'NONE',  ( 1.000000000000000000, -0.000000000000000000, -0.000000000000000000 ) ) ;
#6617=EDGE_CURVE ( 'NONE', #53922, #59346, #62633, .T. ) ;
#6619=CARTESIAN_POINT ( 'NONE',  ( -7.173176924626749162, -1.348899530466227015, 11.92417379687110568 ) ) ;
#6620=VERTEX_POINT ( 'NONE', #36488 ) ;
#6621=EDGE_CURVE ( 'NONE', #56717, #37109, #17868, .T. ) ;
#6623=ORIENTED_EDGE ( 'NONE', *, *, #16533, .F. ) ;
#6624=CARTESIAN_POINT ( 'NONE',  ( 37.00000000000000711, 12.68495603654573500, 1.286231064351171627 ) ) ;
#6626=CARTESIAN_POINT ( 'NONE',  ( -8.891032880924177206, 11.36194426013951997, -3.860857758255646921 ) ) ;
#6629=EDGE_LOOP ( 'NONE', ( #46684, #804, #3527, #63415 ) ) ;
#6630=CARTESIAN_POINT ( 'NONE',  ( 37.00000000000000711, 4.705694406421931860E-17, -3.469127814946512892E-15 ) ) ;
#6632=CARTESIAN_POINT ( 'NONE',  ( 35.00000000000000000, 4.705694406421931860E-17, -3.469127814946512892E-15 ) ) ;
#6635=ORIENTED_EDGE ( 'NONE', *, *, #11639, .T. ) ;
#6637=EDGE_CURVE ( 'NONE', #42088, #45883, #273, .T. ) ;
#6638=ORIENTED_EDGE ( 'NONE', *, *, #63479, .T. ) ;
#6639=EDGE_LOOP ( 'NONE', ( #47844, #3854, #42478, #21067 ) ) ;
#6640=ORIENTED_EDGE ( 'NONE', *, *, #16948, .T. ) ;
#6641=ORIENTED_EDGE ( 'NONE', *, *, #19755, .T. ) ;
#6642=EDGE_CURVE ( 'NONE', #57337, #62155, #51795, .T. ) ;
#6644=CYLINDRICAL_SURFACE ( 'NONE', #17784, 4.999999999999999112 ) ;
#6646=DIRECTION ( 'NONE',  ( 0.000000000000000000, 0.000000000000000000, -1.000000000000000000 ) ) ;
#6647=CARTESIAN_POINT ( 'NONE',  ( 37.00000000000000711, 4.705694406421931860E-17, -3.469127814946512892E-15 ) ) ;
#6649=ADVANCED_FACE ( 'NONE', ( #50800 ), #60778, .T. ) ;
#6651=ORIENTED_EDGE ( 'NONE', *, *, #63970, .F. ) ;
#6652=CARTESIAN_POINT ( 'NONE',  ( 35.00000000000000000, -1.456211999474423369, -11.65554240571057143 ) ) ;
#6653=DIRECTION ( 'NONE',  ( -1.000000000000000000, 0.000000000000000000, 0.000000000000000000 ) ) ;
#6654=EDGE_CURVE ( 'NONE', #6851, #797, #5253, .T. ) ;
#6657=DIRECTION ( 'NONE',  ( 0.000000000000000000, 0.7196168960969817618, 0.6943713148249615053 ) ) ;
#6659=CIRCLE ( 'NONE', #38480, 5.000000000000000888 ) ;
#6660=CIRCLE ( 'NONE', #52318, 12.18650000000000055 ) ;
#6664=ORIENTED_EDGE ( 'NONE', *, *, #33756, .T. ) ;
#6665=DIRECTION ( 'NONE',  ( 0.000000000000000000, -0.01356324068817991828, 0.9999080150203990547 ) ) ;
#6668=CARTESIAN_POINT ( 'NONE',  ( 35.00000000000000000, -4.309077947445731027, -10.92721691015454510 ) ) ;
#6670=ORIENTED_EDGE ( 'NONE', *, *, #9633, .F. ) ;
#6671=CARTESIAN_POINT ( 'NONE',  ( 37.00000000000000711, -11.74226168163341555, -0.3025107581130825896 ) ) ;
#6672=CARTESIAN_POINT ( 'NONE',  ( 36.00000000000000711, 7.745827850123149005, 10.12742074351888100 ) ) ;
#6673=CARTESIAN_POINT ( 'NONE',  ( 35.00000000000000000, -12.26766708251988724, 3.473736367725380969 ) ) ;
#6674=DIRECTION ( 'NONE',  ( -1.000000000000000000, 0.000000000000000000, 0.000000000000000000 ) ) ;
#6675=AXIS2_PLACEMENT_3D ( 'NONE', #10585, #55503, #30230 ) ;
#6676=EDGE_CURVE ( 'NONE', #9320, #24124, #46238, .T. ) ;
#6677=CARTESIAN_POINT ( 'NONE',  ( -37.00000000000000711, 0.000000000000000000, 0.000000000000000000 ) ) ;
#6678=AXIS2_PLACEMENT_3D ( 'NONE', #14287, #55519, #15274 ) ;
#6680=AXIS2_PLACEMENT_3D ( 'NONE', #31242, #46524, #41523 ) ;
#6683=ADVANCED_FACE ( 'NONE', ( #35499 ), #16207, .T. ) ;
#6684=EDGE_CURVE ( 'NONE', #17893, #21858, #9903, .T. ) ;
#6685=ORIENTED_EDGE ( 'NONE', *, *, #5740, .T. ) ;
#6686=ORIENTED_EDGE ( 'NONE', *, *, #38646, .F. ) ;
#6689=CARTESIAN_POINT ( 'NONE',  ( 47.00000000000000711, 4.705694406421931860E-17, -3.469127814946512892E-15 ) ) ;
#6692=EDGE_CURVE ( 'NONE', #47761, #64752, #21203, .T. ) ;
#6693=CIRCLE ( 'NONE', #9850, 5.000000000000000888 ) ;
#6695=VERTEX_POINT ( 'NONE', #20863 ) ;
#6697=CIRCLE ( 'NONE', #19422, 4.999999999999999112 ) ;
#6698=CARTESIAN_POINT ( 'NONE',  ( -4.975205859172452172, -1.416020129149132778, 25.00000000000000000 ) ) ;
#6699=VECTOR ( 'NONE', #55247, 1000.000000000000000 ) ;
#6701=CARTESIAN_POINT ( 'NONE',  ( 35.00000000000000000, 11.86701198550355940, -2.772148766916162188 ) ) ;
#6702=FACE_OUTER_BOUND ( 'NONE', #27162, .T. ) ;
#6703=ORIENTED_EDGE ( 'NONE', *, *, #25038, .T. ) ;
#6704=DIRECTION ( 'NONE',  ( -1.000000000000000000, 0.000000000000000000, 0.000000000000000000 ) ) ;
#6705=DIRECTION ( 'NONE',  ( 0.000000000000000000, -0.01356324068817999114, 0.9999080150203989437 ) ) ;
#6706=CYLINDRICAL_SURFACE ( 'NONE', #56897, 4.999999999999999112 ) ;
#6709=CARTESIAN_POINT ( 'NONE',  ( -37.00000000000000711, -11.80185301892984384, 4.824807283154077808 ) ) ;
#6710=ORIENTED_EDGE ( 'NONE', *, *, #47652, .F. ) ;
#6711=CARTESIAN_POINT ( 'NONE',  ( -10.95212338237647920, -9.902220863987562183, 25.00000000000000000 ) ) ;
#6712=AXIS2_PLACEMENT_3D ( 'NONE', #65208, #35598, #49923 ) ;
#6713=CARTESIAN_POINT ( 'NONE',  ( -17.64392624464051806, -7.224638894555154955, 11.40788166233496170 ) ) ;
#6714=EDGE_CURVE ( 'NONE', #26131, #41694, #22940, .T. ) ;
#6719=FACE_OUTER_BOUND ( 'NONE', #48296, .T. ) ;
#6720=DIRECTION ( 'NONE',  ( 0.000000000000000000, 0.8989688749565142301, 0.4380125133594005016 ) ) ;
#6722=LINE ( 'NONE', #427, #40517 ) ;
#6723=ORIENTED_EDGE ( 'NONE', *, *, #15643, .T. ) ;
#6724=EDGE_CURVE ( 'NONE', #14872, #20098, #26188, .T. ) ;
#6726=VERTEX_POINT ( 'NONE', #11222 ) ;
#6727=CYLINDRICAL_SURFACE ( 'NONE', #5165, 12.75000000000000178 ) ;
#6728=CARTESIAN_POINT ( 'NONE',  ( -28.41827485489077532, 3.509237424706437292, -13.03592162821790801 ) ) ;
#6730=ORIENTED_EDGE ( 'NONE', *, *, #14613, .T. ) ;
#6736=VERTEX_POINT ( 'NONE', #58091 ) ;
#6737=CARTESIAN_POINT ( 'NONE',  ( 36.00000000000000711, 12.49688848680884234, -2.527899948230686089 ) ) ;
#6738=VERTEX_POINT ( 'NONE', #6571 ) ;
#6740=CARTESIAN_POINT ( 'NONE',  ( 36.00000000000000711, -5.710938531231790627, -11.39945968423469580 ) ) ;
#6742=ORIENTED_EDGE ( 'NONE', *, *, #19074, .T. ) ;
#6745=CIRCLE ( 'NONE', #30079, 12.18650000000000055 ) ;
#6746=ADVANCED_FACE ( 'NONE', ( #22170 ), #63378, .F. ) ;
#6747=EDGE_CURVE ( 'NONE', #53954, #29924, #29691, .T. ) ;
#6748=DIRECTION ( 'NONE',  ( 1.000000000000000000, 0.000000000000000000, 0.000000000000000000 ) ) ;
#6749=CARTESIAN_POINT ( 'NONE',  ( -37.00000000000000711, -10.30098186818253758, 5.644643009979033899 ) ) ;
#6750=AXIS2_PLACEMENT_3D ( 'NONE', #50894, #5690, #45910 ) ;
#6751=DIRECTION ( 'NONE',  ( 0.000000000000000000, 0.4134677391718510897, 0.9105187689795954942 ) ) ;
#6752=LINE ( 'NONE', #35673, #16862 ) ;
#6753=DIRECTION ( 'NONE',  ( 1.000000000000000000, 0.000000000000000000, 0.000000000000000000 ) ) ;
#6754=DIRECTION ( 'NONE',  ( 0.000000000000000000, 0.01356324068817998940, -0.9999080150203990547 ) ) ;
#6755=CARTESIAN_POINT ( 'NONE',  ( 37.00000000000000711, 4.705694406421931860E-17, -3.469127814946512892E-15 ) ) ;
#6756=CIRCLE ( 'NONE', #8839, 5.000000000000001776 ) ;
#6760=ORIENTED_EDGE ( 'NONE', *, *, #15444, .F. ) ;
#6763=VERTEX_POINT ( 'NONE', #36814 ) ;
#6764=CARTESIAN_POINT ( 'NONE',  ( 36.00000000000000711, -1.908798535168467536, -12.60630747491662618 ) ) ;
#6766=ORIENTED_EDGE ( 'NONE', *, *, #17173, .F. ) ;
#6767=DIRECTION ( 'NONE',  ( 1.000000000000000000, 0.000000000000000000, 0.000000000000000000 ) ) ;
#6768=ORIENTED_EDGE ( 'NONE', *, *, #39716, .F. ) ;
#6771=ORIENTED_EDGE ( 'NONE', *, *, #4380, .F. ) ;
#6772=ORIENTED_EDGE ( 'NONE', *, *, #10043, .F. ) ;
#6773=EDGE_CURVE ( 'NONE', #5329, #24551, #27821, .T. ) ;
#6774=LINE ( 'NONE', #21746, #1921 ) ;
#6775=AXIS2_PLACEMENT_3D ( 'NONE', #39148, #34162, #28857 ) ;
#6776=VERTEX_POINT ( 'NONE', #17531 ) ;
#6777=CARTESIAN_POINT ( 'NONE',  ( -24.81264729437695848, -8.085877654816028937, 8.874484760932165983 ) ) ;
#6779=CARTESIAN_POINT ( 'NONE',  ( 22.78406729994189561, -4.691424615418254618, -12.65938842238563744 ) ) ;
#6780=DIRECTION ( 'NONE',  ( 0.000000000000000000, 0.9903235168508555120, 0.1387779952735782862 ) ) ;
#6781=VERTEX_POINT ( 'NONE', #37798 ) ;
#6782=FACE_OUTER_BOUND ( 'NONE', #56016, .T. ) ;
#6785=DIRECTION ( 'NONE',  ( -1.000000000000000000, -0.000000000000000000, 0.000000000000000000 ) ) ;
#6786=ORIENTED_EDGE ( 'NONE', *, *, #44938, .F. ) ;
#6787=CARTESIAN_POINT ( 'NONE',  ( -28.19916972693312829, 11.19825076026768151, -4.324271721581003369 ) ) ;
#6791=ORIENTED_EDGE ( 'NONE', *, *, #42958, .F. ) ;
#6792=CARTESIAN_POINT ( 'NONE',  ( 21.53315970858584549, -11.27100376921459635, -4.123804204784697447 ) ) ;
#6793=DIRECTION ( 'NONE',  ( 0.000000000000000000, 0.6478160128811948359, -0.7617968321374878338 ) ) ;
#6794=EDGE_CURVE ( 'NONE', #27971, #19813, #53091, .T. ) ;
#6797=ORIENTED_EDGE ( 'NONE', *, *, #54934, .T. ) ;
#6798=CARTESIAN_POINT ( 'NONE',  ( -37.00000000000000711, -9.557269938331609538, 7.561043153947932360 ) ) ;
#6801=ORIENTED_EDGE ( 'NONE', *, *, #34589, .T. ) ;
#6803=( BOUNDED_CURVE ( )  B_SPLINE_CURVE ( 3, ( #5212, #40437, #21138, #20502 ),
 .UNSPECIFIED., .F., .F. ) 
 B_SPLINE_CURVE_WITH_KNOTS ( ( 4, 4 ),
 ( 1.570796326794897446, 1.605031943246829185 ),
 .UNSPECIFIED. ) 
 CURVE ( )  GEOMETRIC_REPRESENTATION_ITEM ( )  RATIONAL_B_SPLINE_CURVE ( ( 1.000000000000000000, 0.9999023292654991568, 0.9999023292654991568, 1.000000000000000000 ) ) 
 REPRESENTATION_ITEM ( '' )  );
#6804=AXIS2_PLACEMENT_3D ( 'NONE', #58357, #26780, #42368 ) ;
#6805=EDGE_LOOP ( 'NONE', ( #6256, #23946, #65084, #4554 ) ) ;
#6807=ORIENTED_EDGE ( 'NONE', *, *, #53978, .F. ) ;
#6808=VECTOR ( 'NONE', #63072, 1000.000000000000000 ) ;
#6809=ORIENTED_EDGE ( 'NONE', *, *, #59482, .T. ) ;
#6810=AXIS2_PLACEMENT_3D ( 'NONE', #60942, #5416, #36956 ) ;
#6812=DIRECTION ( 'NONE',  ( 1.000000000000000000, 0.000000000000000000, -0.000000000000000000 ) ) ;
#6813=DIRECTION ( 'NONE',  ( 0.000000000000000000, 0.9105187689795967154, -0.4134677391718482586 ) ) ;
#6814=DIRECTION ( 'NONE',  ( 1.000000000000000000, 0.000000000000000000, 0.000000000000000000 ) ) ;
#6816=AXIS2_PLACEMENT_3D ( 'NONE', #47656, #27053, #22727 ) ;
#6818=ADVANCED_FACE ( 'NONE', ( #7882 ), #28158, .T. ) ;
#6819=DIRECTION ( 'NONE',  ( 1.000000000000000000, 0.000000000000000000, 0.000000000000000000 ) ) ;
#6822=CIRCLE ( 'NONE', #22715, 12.18650000000000055 ) ;
#6824=CARTESIAN_POINT ( 'NONE',  ( 12.51043786959929527, 0.3316631525046815909, -11.99656223984053760 ) ) ;
#6825=CYLINDRICAL_SURFACE ( 'NONE', #61982, 5.000000000000000888 ) ;
#6826=AXIS2_PLACEMENT_3D ( 'NONE', #44637, #25693, #10384 ) ;
#6828=EDGE_CURVE ( 'NONE', #2293, #55606, #42447, .T. ) ;
#6829=CARTESIAN_POINT ( 'NONE',  ( 35.00000000000000000, 4.705694406421931860E-17, -3.469127814946512892E-15 ) ) ;
#6830=CARTESIAN_POINT ( 'NONE',  ( 47.00000000000000711, 4.705694406421931860E-17, -3.469127814946512892E-15 ) ) ;
#6831=ORIENTED_EDGE ( 'NONE', *, *, #49622, .F. ) ;
#6832=DIRECTION ( 'NONE',  ( -1.000000000000000000, 0.000000000000000000, 0.000000000000000000 ) ) ;
#6835=FACE_OUTER_BOUND ( 'NONE', #62461, .T. ) ;
#6839=CARTESIAN_POINT ( 'NONE',  ( -24.82456806599946830, 8.749941039790773090, 8.214224094661178199 ) ) ;
#6840=CARTESIAN_POINT ( 'NONE',  ( -25.50184365408103204, -8.498472128355658128, 10.49391108592481814 ) ) ;
#6841=ORIENTED_EDGE ( 'NONE', *, *, #54743, .F. ) ;
#6842=DIRECTION ( 'NONE',  ( 1.000000000000000000, 0.000000000000000000, 0.000000000000000000 ) ) ;
#6843=DIRECTION ( 'NONE',  ( 0.000000000000000000, -0.3218879778915842427, 0.9467777615094614685 ) ) ;
#6845=VERTEX_POINT ( 'NONE', #18182 ) ;
#6847=DIRECTION ( 'NONE',  ( -1.000000000000000000, 0.000000000000000000, -0.000000000000000000 ) ) ;
#6848=EDGE_CURVE ( 'NONE', #12145, #57976, #50985, .T. ) ;
#6850=CARTESIAN_POINT ( 'NONE',  ( 22.57855258442565116, 3.026812727784649493, -13.15630665159948975 ) ) ;
#6851=VERTEX_POINT ( 'NONE', #38786 ) ;
#6852=CARTESIAN_POINT ( 'NONE',  ( -35.00000000000000000, 0.000000000000000000, 0.000000000000000000 ) ) ;
#6853=ADVANCED_FACE ( 'NONE', ( #44734 ), #14470, .T. ) ;
#6854=VECTOR ( 'NONE', #16508, 1000.000000000000000 ) ;
#6857=FACE_OUTER_BOUND ( 'NONE', #64406, .T. ) ;
#6858=DIRECTION ( 'NONE',  ( -1.000000000000000000, -0.000000000000000000, 0.000000000000000000 ) ) ;
#6861=CARTESIAN_POINT ( 'NONE',  ( -9.514445118316093186, 11.30297198722328567, -4.050438551049715841 ) ) ;
#6862=CARTESIAN_POINT ( 'NONE',  ( -35.00000000000000000, 4.725891942574755866, 10.75351884295729477 ) ) ;
#6863=CARTESIAN_POINT ( 'NONE',  ( 35.00000000000000000, -10.62137734850271364, -5.015831474386272859 ) ) ;
#6864=VERTEX_POINT ( 'NONE', #49441 ) ;
#6865=CARTESIAN_POINT ( 'NONE',  ( 10.47226376122552516, 7.645066471088986404, 11.12901864558550180 ) ) ;
#6867=CARTESIAN_POINT ( 'NONE',  ( 23.46994683125024750, -4.312020184895027697, -11.20298071244178573 ) ) ;
#6870=ADVANCED_FACE ( 'NONE', ( #34743 ), #59083, .T. ) ;
#6871=CARTESIAN_POINT ( 'NONE',  ( -3.191470641060126567, 11.27526359945950496, 4.125568914908559925 ) ) ;
#6872=VECTOR ( 'NONE', #64443, 1000.000000000000000 ) ;
#6875=ORIENTED_EDGE ( 'NONE', *, *, #33853, .F. ) ;
#6876=CARTESIAN_POINT ( 'NONE',  ( 35.00000000000000000, 11.60979404548634619, -3.704519465651352483 ) ) ;
#6879=ORIENTED_EDGE ( 'NONE', *, *, #34457, .T. ) ;
#6880=CARTESIAN_POINT ( 'NONE',  ( 29.03457606387295087, -7.862146963512102182, 10.97436308512422265 ) ) ;
#6881=ORIENTED_EDGE ( 'NONE', *, *, #42480, .F. ) ;
#6882=FACE_OUTER_BOUND ( 'NONE', #17739, .T. ) ;
#6883=CARTESIAN_POINT ( 'NONE',  ( -10.95212338237647920, -9.902220863987562183, -6.778349501228825069 ) ) ;
#6884=CARTESIAN_POINT ( 'NONE',  ( 35.00000000000000000, 4.705694406421931860E-17, -3.469127814946512892E-15 ) ) ;
#6889=CARTESIAN_POINT ( 'NONE',  ( -37.00000000000000711, -5.130401251914653571, -11.05394794832835359 ) ) ;
#6892=ORIENTED_EDGE ( 'NONE', *, *, #22856, .F. ) ;
#6893=DIRECTION ( 'NONE',  ( -1.000000000000000000, 0.000000000000000000, 0.000000000000000000 ) ) ;
#6894=DIRECTION ( 'NONE',  ( 1.000000000000000000, 0.000000000000000000, -0.000000000000000000 ) ) ;
#6896=DIRECTION ( 'NONE',  ( 1.000000000000000000, 0.000000000000000000, 0.000000000000000000 ) ) ;
#6900=VERTEX_POINT ( 'NONE', #9475 ) ;
#6903=EDGE_CURVE ( 'NONE', #65435, #53879, #27607, .T. ) ;
#6906=CARTESIAN_POINT ( 'NONE',  ( -37.00000000000000711, 10.39746860227890757, 7.379373053628906831 ) ) ;
#6908=ADVANCED_FACE ( 'NONE', ( #8197 ), #13810, .T. ) ;
#6910=CARTESIAN_POINT ( 'NONE',  ( 35.00000000000000000, 9.240395740215630482, -7.251710744571611578 ) ) ;
#6913=DIRECTION ( 'NONE',  ( -1.000000000000000000, 0.000000000000000000, 0.000000000000000000 ) ) ;
#6915=CIRCLE ( 'NONE', #49421, 12.18649999999999878 ) ;
#6917=DIRECTION ( 'NONE',  ( 1.000000000000000000, -0.000000000000000000, -0.000000000000000000 ) ) ;
#6918=CARTESIAN_POINT ( 'NONE',  ( -35.00000000000000000, 0.000000000000000000, 0.000000000000000000 ) ) ;
#6922=DIRECTION ( 'NONE',  ( 1.000000000000000000, 0.000000000000000000, 0.000000000000000000 ) ) ;
#6931=ADVANCED_FACE ( 'NONE', ( #48770 ), #44398, .T. ) ;
#6932=ORIENTED_EDGE ( 'NONE', *, *, #17856, .T. ) ;
#6934=CARTESIAN_POINT ( 'NONE',  ( 37.00000000000000711, 4.545979934229410269, -11.30684963584391234 ) ) ;
#6935=VECTOR ( 'NONE', #30933, 1000.000000000000000 ) ;
#6936=DIRECTION ( 'NONE',  ( 0.000000000000000000, 0.01356324068817992175, -0.9999080150203990547 ) ) ;
#6938=CARTESIAN_POINT ( 'NONE',  ( -37.00000000000000711, 3.640372113593720815, -12.21925492305358318 ) ) ;
#6940=DIRECTION ( 'NONE',  ( 0.000000000000000000, -0.01356324068818000328, 0.9999080150203990547 ) ) ;
#6942=ORIENTED_EDGE ( 'NONE', *, *, #32611, .T. ) ;
#6946=DIRECTION ( 'NONE',  ( 0.000000000000000000, 0.01356324068817998940, -0.9999080150203990547 ) ) ;
#6947=CARTESIAN_POINT ( 'NONE',  ( -35.00000000000000000, -1.463443770872689509, -12.09831040184925577 ) ) ;
#6949=EDGE_LOOP ( 'NONE', ( #33492, #34577, #43633, #38608 ) ) ;
#6953=ORIENTED_EDGE ( 'NONE', *, *, #12025, .T. ) ;
#6957=ORIENTED_EDGE ( 'NONE', *, *, #45243, .F. ) ;
#6958=EDGE_LOOP ( 'NONE', ( #29863, #59050, #46446, #41986 ) ) ;
#6959=VERTEX_POINT ( 'NONE', #3221 ) ;
#6962=EDGE_CURVE ( 'NONE', #23964, #55391, #14867, .T. ) ;
#6964=CARTESIAN_POINT ( 'NONE',  ( -35.00000000000000000, 10.49591321039680736, 5.273331777780375873 ) ) ;
#6966=CARTESIAN_POINT ( 'NONE',  ( -35.00000000000000000, 0.000000000000000000, 0.000000000000000000 ) ) ;
#6967=CARTESIAN_POINT ( 'NONE',  ( 37.00000000000000711, 9.430788938294046631, -7.718225330433843290 ) ) ;
#6968=ORIENTED_EDGE ( 'NONE', *, *, #7271, .F. ) ;
#6969=CARTESIAN_POINT ( 'NONE',  ( -35.00000000000000000, 10.91072401419410554, 5.428340790341743549 ) ) ;
#6970=CYLINDRICAL_SURFACE ( 'NONE', #2333, 12.18650000000000055 ) ;
#6974=FACE_OUTER_BOUND ( 'NONE', #34658, .T. ) ;
#6976=EDGE_CURVE ( 'NONE', #33925, #17893, #4325, .T. ) ;
#6977=ORIENTED_EDGE ( 'NONE', *, *, #46484, .F. ) ;
#6979=VECTOR ( 'NONE', #40760, 1000.000000000000000 ) ;
#6980=ORIENTED_EDGE ( 'NONE', *, *, #34398, .F. ) ;
#6981=EDGE_CURVE ( 'NONE', #56228, #61588, #10805, .T. ) ;
#6983=DIRECTION ( 'NONE',  ( -1.000000000000000000, 0.000000000000000000, 0.000000000000000000 ) ) ;
#6984=CYLINDRICAL_SURFACE ( 'NONE', #52634, 12.75000000000000178 ) ;
#6985=DIRECTION ( 'NONE',  ( -1.000000000000000000, 0.000000000000000000, 0.000000000000000000 ) ) ;
#6986=EDGE_CURVE ( 'NONE', #21944, #45661, #40072, .T. ) ;
#6990=DIRECTION ( 'NONE',  ( 1.000000000000000000, 0.000000000000000000, -0.000000000000000000 ) ) ;
#6991=DIRECTION ( 'NONE',  ( 1.000000000000000000, 0.000000000000000000, 0.000000000000000000 ) ) ;
#6992=CARTESIAN_POINT ( 'NONE',  ( -21.17861794710831091, 25.00000000000000000, -3.604945070120774808 ) ) ;
#6993=AXIS2_PLACEMENT_3D ( 'NONE', #43328, #17084, #62962 ) ;
#6994=EDGE_CURVE ( 'NONE', #41167, #665, #62672, .T. ) ;
#6996=( BOUNDED_CURVE ( )  B_SPLINE_CURVE ( 3, ( #28277, #16659, #37258, #36931 ),
 .UNSPECIFIED., .F., .T. ) 
 B_SPLINE_CURVE_WITH_KNOTS ( ( 4, 4 ),
 ( 4.635356053521499931, 4.651107231023391186 ),
 .UNSPECIFIED. ) 
 CURVE ( )  GEOMETRIC_REPRESENTATION_ITEM ( )  RATIONAL_B_SPLINE_CURVE ( ( 1.000000000000000000, 0.9999793251408052308, 0.9999793251408052308, 1.000000000000000000 ) ) 
 REPRESENTATION_ITEM ( '' )  );
#6997=ORIENTED_EDGE ( 'NONE', *, *, #24242, .T. ) ;
#6998=ADVANCED_FACE ( 'NONE', ( #60359 ), #56028, .T. ) ;
#7001=ORIENTED_EDGE ( 'NONE', *, *, #28993, .F. ) ;
#7006=DIRECTION ( 'NONE',  ( 0.000000000000000000, -0.4935949184179322380, 0.8696919319575150409 ) ) ;
#7007=EDGE_CURVE ( 'NONE', #4699, #63989, #524, .T. ) ;
#7009=VERTEX_POINT ( 'NONE', #5179 ) ;
#7010=ORIENTED_EDGE ( 'NONE', *, *, #56543, .T. ) ;
#7012=CARTESIAN_POINT ( 'NONE',  ( 35.00000000000000000, -12.73293890771483383, -0.6593684648220086153 ) ) ;
#7013=DIRECTION ( 'NONE',  ( -1.000000000000000000, 0.000000000000000000, 0.000000000000000000 ) ) ;
#7014=EDGE_LOOP ( 'NONE', ( #14218, #20819, #42010, #19956 ) ) ;
#7016=CYLINDRICAL_SURFACE ( 'NONE', #37904, 5.000000000000000888 ) ;
#7018=EDGE_LOOP ( 'NONE', ( #62340, #1978, #40542, #16762 ) ) ;
#7022=DIRECTION ( 'NONE',  ( 0.000000000000000000, -0.01356324068817998940, 0.9999080150203990547 ) ) ;
#7023=ORIENTED_EDGE ( 'NONE', *, *, #6724, .F. ) ;
#7024=DIRECTION ( 'NONE',  ( -1.000000000000000000, -0.000000000000000000, 0.000000000000000000 ) ) ;
#7029=FACE_OUTER_BOUND ( 'NONE', #65297, .T. ) ;
#7031=CARTESIAN_POINT ( 'NONE',  ( -37.00000000000000711, 11.90598845858533750, 4.561791185930457182 ) ) ;
#7032=DIRECTION ( 'NONE',  ( -1.000000000000000000, -0.000000000000000000, 0.000000000000000000 ) ) ;
#7033=DIRECTION ( 'NONE',  ( 1.000000000000000000, -0.000000000000000000, 0.000000000000000000 ) ) ;
#7035=ORIENTED_EDGE ( 'NONE', *, *, #28329, .T. ) ;
#7036=LINE ( 'NONE', #46954, #16251 ) ;
#7037=ORIENTED_EDGE ( 'NONE', *, *, #63896, .F. ) ;
#7040=ORIENTED_EDGE ( 'NONE', *, *, #40363, .F. ) ;
#7042=FACE_OUTER_BOUND ( 'NONE', #49879, .T. ) ;
#7046=EDGE_LOOP ( 'NONE', ( #33677, #6703, #10179, #8429 ) ) ;
#7047=ADVANCED_FACE ( 'NONE', ( #27093 ), #31094, .T. ) ;
#7051=CYLINDRICAL_SURFACE ( 'NONE', #55205, 12.75000000000000178 ) ;
#7054=EDGE_CURVE ( 'NONE', #54831, #39860, #8189, .T. ) ;
#7055=CARTESIAN_POINT ( 'NONE',  ( -35.00000000000000000, -9.348667969174350389, -7.817492529713957694 ) ) ;
#7056=ORIENTED_EDGE ( 'NONE', *, *, #6263, .T. ) ;
#7058=AXIS2_PLACEMENT_3D ( 'NONE', #28995, #19350, #49307 ) ;
#7060=DIRECTION ( 'NONE',  ( 0.000000000000000000, 0.01356324068817998940, -0.9999080150203990547 ) ) ;
#7061=EDGE_CURVE ( 'NONE', #82, #27703, #37198, .T. ) ;
#7062=CARTESIAN_POINT ( 'NONE',  ( -35.00000000000000000, 12.16632754454237819, -0.7008968033237440443 ) ) ;
#7064=EDGE_CURVE ( 'NONE', #7826, #45182, #34022, .T. ) ;
#7065=CARTESIAN_POINT ( 'NONE',  ( 37.00000000000000711, -0.8294751490778421443, 12.15823808070322976 ) ) ;
#7066=DIRECTION ( 'NONE',  ( 1.000000000000000000, -0.000000000000000000, 0.000000000000000000 ) ) ;
#7068=EDGE_CURVE ( 'NONE', #65184, #19802, #37048, .T. ) ;
#7071=CARTESIAN_POINT ( 'NONE',  ( -14.73932195233055609, 7.919210176484706487, 10.93330280096819074 ) ) ;
#7073=ORIENTED_EDGE ( 'NONE', *, *, #62336, .F. ) ;
#7075=LINE ( 'NONE', #2088, #58740 ) ;
#7076=EDGE_LOOP ( 'NONE', ( #27806, #58221, #50069, #63938, #7193 ) ) ;
#7077=EDGE_CURVE ( 'NONE', #47218, #3051, #13027, .T. ) ;
#7078=CARTESIAN_POINT ( 'NONE',  ( 47.00000000000000711, 4.705694406421931860E-17, -3.469127814946512892E-15 ) ) ;
#7079=ORIENTED_EDGE ( 'NONE', *, *, #28541, .F. ) ;
#7080=FACE_OUTER_BOUND ( 'NONE', #53658, .T. ) ;
#7081=ORIENTED_EDGE ( 'NONE', *, *, #43223, .T. ) ;
#7083=FACE_OUTER_BOUND ( 'NONE', #31474, .T. ) ;
#7084=ORIENTED_EDGE ( 'NONE', *, *, #47893, .T. ) ;
#7087=CARTESIAN_POINT ( 'NONE',  ( 35.00000000000000000, -0.06441628369827803735, 12.18632975068352309 ) ) ;
#7088=CARTESIAN_POINT ( 'NONE',  ( 22.57855258442564761, -4.427776684447072952, -12.75322679295976691 ) ) ;
#7090=VERTEX_POINT ( 'NONE', #48616 ) ;
#7091=FACE_OUTER_BOUND ( 'NONE', #3777, .T. ) ;
#7093=DIRECTION ( 'NONE',  ( 0.000000000000000000, 0.9467777615094560284, 0.3218879778916007295 ) ) ;
#7094=CARTESIAN_POINT ( 'NONE',  ( -26.14647939271262800, 10.67107426152631788, 5.490406654534011999 ) ) ;
#7095=VERTEX_POINT ( 'NONE', #3069 ) ;
#7096=LINE ( 'NONE', #32029, #41587 ) ;
#7097=ORIENTED_EDGE ( 'NONE', *, *, #31480, .F. ) ;
#7100=CIRCLE ( 'NONE', #51697, 4.999999999999999112 ) ;
#7101=CARTESIAN_POINT ( 'NONE',  ( 21.61122408824027374, -11.12492833342144216, -4.503027499503673425 ) ) ;
#7102=CARTESIAN_POINT ( 'NONE',  ( -18.25006854224444908, -9.443202773001939221, 25.00000000000000000 ) ) ;
#7103=CYLINDRICAL_SURFACE ( 'NONE', #13134, 4.999999999999999112 ) ;
#7105=EDGE_CURVE ( 'NONE', #41254, #47877, #49933, .T. ) ;
#7106=DIRECTION ( 'NONE',  ( 1.000000000000000000, 0.000000000000000000, 0.000000000000000000 ) ) ;
#7109=EDGE_LOOP ( 'NONE', ( #39986, #54631, #53564, #3543 ) ) ;
#7110=EDGE_CURVE ( 'NONE', #39817, #9384, #5365, .T. ) ;
#7111=EDGE_LOOP ( 'NONE', ( #42813, #1695, #4466, #14105 ) ) ;
#7112=DIRECTION ( 'NONE',  ( 0.000000000000000000, -0.6943713148249534006, 0.7196168960969896444 ) ) ;
#7115=EDGE_CURVE ( 'NONE', #12300, #8992, #29740, .T. ) ;
#7117=CARTESIAN_POINT ( 'NONE',  ( 37.00000000000000711, 10.42955799785319826, -6.303578524886986223 ) ) ;
#7118=DIRECTION ( 'NONE',  ( 0.000000000000000000, -0.01356324068817998940, 0.9999080150203990547 ) ) ;
#7120=CARTESIAN_POINT ( 'NONE',  ( -35.00000000000000000, 0.000000000000000000, 0.000000000000000000 ) ) ;
#7121=DIRECTION ( 'NONE',  ( 0.000000000000000000, 0.01356324068817991828, -0.9999080150203990547 ) ) ;
#7122=DIRECTION ( 'NONE',  ( -1.000000000000000000, 0.000000000000000000, 0.000000000000000000 ) ) ;
#7123=VERTEX_POINT ( 'NONE', #54597 ) ;
#7126=EDGE_CURVE ( 'NONE', #40853, #18660, #42502, .T. ) ;
#7129=DIRECTION ( 'NONE',  ( -1.000000000000000000, 0.000000000000000000, 0.000000000000000000 ) ) ;
#7130=DIRECTION ( 'NONE',  ( 1.000000000000000000, 0.000000000000000000, -0.000000000000000000 ) ) ;
#7131=CARTESIAN_POINT ( 'NONE',  ( -47.00000000000000711, 0.000000000000000000, 0.000000000000000000 ) ) ;
#7133=ORIENTED_EDGE ( 'NONE', *, *, #59433, .F. ) ;
#7134=DIRECTION ( 'NONE',  ( 1.000000000000000000, 0.000000000000000000, 0.000000000000000000 ) ) ;
#7136=DIRECTION ( 'NONE',  ( 0.000000000000000000, 0.01356324068817998940, -0.9999080150203990547 ) ) ;
#7139=AXIS2_PLACEMENT_3D ( 'NONE', #2308, #22584, #36882 ) ;
#7140=ADVANCED_FACE ( 'NONE', ( #49596 ), #19001, .T. ) ;
#7142=ADVANCED_FACE ( 'NONE', ( #3743 ), #34911, .T. ) ;
#7143=CYLINDRICAL_SURFACE ( 'NONE', #30940, 4.500030059823568074 ) ;
#7144=DIRECTION ( 'NONE',  ( 1.000000000000000000, -0.000000000000000000, 0.000000000000000000 ) ) ;
#7147=CARTESIAN_POINT ( 'NONE',  ( -27.64986549192623499, -12.88105143700861888, -4.050455452492842667 ) ) ;
#7151=EDGE_CURVE ( 'NONE', #47299, #27224, #53167, .T. ) ;
#7152=DIRECTION ( 'NONE',  ( -1.000000000000000000, 0.000000000000000000, -0.000000000000000000 ) ) ;
#7153=LINE ( 'NONE', #27428, #59613 ) ;
#7154=ORIENTED_EDGE ( 'NONE', *, *, #50173, .T. ) ;
#7155=CARTESIAN_POINT ( 'NONE',  ( -36.00000000000000711, -12.60630747491664572, 1.908798535168333643 ) ) ;
#7157=ORIENTED_EDGE ( 'NONE', *, *, #48450, .F. ) ;
#7158=DIRECTION ( 'NONE',  ( -1.000000000000000000, 0.000000000000000000, 0.000000000000000000 ) ) ;
#7164=CARTESIAN_POINT ( 'NONE',  ( -2.952869152607107139, 12.96714474214482138, 3.755417052241487585 ) ) ;
#7165=EDGE_LOOP ( 'NONE', ( #45416, #32914, #15881, #61110 ) ) ;
#7167=ORIENTED_EDGE ( 'NONE', *, *, #37051, .T. ) ;
#7168=CARTESIAN_POINT ( 'NONE',  ( 22.88594695219327235, -4.822122601967141264, -10.98850006195556261 ) ) ;
#7172=AXIS2_PLACEMENT_3D ( 'NONE', #35635, #34962, #25023 ) ;
#7175=DIRECTION ( 'NONE',  ( 0.000000000000000000, 0.2006870767258889243, -0.9796553971857742127 ) ) ;
#7177=EDGE_CURVE ( 'NONE', #27528, #476, #39267, .T. ) ;
#7178=CARTESIAN_POINT ( 'NONE',  ( -24.42312813602775634, -7.374403702826844764, 9.469279496625576442 ) ) ;
#7179=CARTESIAN_POINT ( 'NONE',  ( 3.991229212642302127, 6.917749631459077619, -11.62716796859311863 ) ) ;
#7180=ORIENTED_EDGE ( 'NONE', *, *, #60559, .T. ) ;
#7181=ORIENTED_EDGE ( 'NONE', *, *, #25198, .T. ) ;
#7182=CARTESIAN_POINT ( 'NONE',  ( 35.00000000000000000, -2.080187960898473243, 12.57916205664482945 ) ) ;
#7183=ORIENTED_EDGE ( 'NONE', *, *, #29771, .F. ) ;
#7186=CARTESIAN_POINT ( 'NONE',  ( -35.00000000000000000, -4.824807283154036952, -11.80185301892985805 ) ) ;
#7187=DIRECTION ( 'NONE',  ( 0.000000000000000000, -0.04924826701375289995, -0.9987865678893274035 ) ) ;
#7189=CARTESIAN_POINT ( 'NONE',  ( -37.00000000000000711, 11.01837265713082203, -6.415447294506590126 ) ) ;
#7191=AXIS2_PLACEMENT_3D ( 'NONE', #29658, #65254, #24694 ) ;
#7193=ORIENTED_EDGE ( 'NONE', *, *, #33691, .T. ) ;
#7194=DIRECTION ( 'NONE',  ( 1.000000000000000000, 0.000000000000000000, 0.000000000000000000 ) ) ;
#7195=ORIENTED_EDGE ( 'NONE', *, *, #47009, .T. ) ;
#7196=DIRECTION ( 'NONE',  ( 0.000000000000000000, 0.01356324068817992175, -0.9999080150203990547 ) ) ;
#7200=DIRECTION ( 'NONE',  ( 0.000000000000000000, -0.9987865678893272925, 0.04924826701375684818 ) ) ;
#7201=EDGE_CURVE ( 'NONE', #39829, #46242, #24474, .T. ) ;
#7202=VERTEX_POINT ( 'NONE', #19335 ) ;
#7204=CARTESIAN_POINT ( 'NONE',  ( -35.00000000000000000, 2.346765782874606465, -11.95840593935198903 ) ) ;
#7207=DIRECTION ( 'NONE',  ( 0.000000000000000000, -0.01356324068817992175, 0.9999080150203990547 ) ) ;
#7212=CARTESIAN_POINT ( 'NONE',  ( 37.00000000000000711, -11.66664283989683426, -5.143145423404238414 ) ) ;
#7215=EDGE_CURVE ( 'NONE', #27631, #49629, #17694, .T. ) ;
#7216=AXIS2_PLACEMENT_3D ( 'NONE', #47923, #19945, #29277 ) ;
#7218=LINE ( 'NONE', #53459, #10657 ) ;
#7220=ORIENTED_EDGE ( 'NONE', *, *, #41243, .T. ) ;
#7224=DIRECTION ( 'NONE',  ( 0.000000000000000000, 0.01356324068817991828, -0.9999080150203990547 ) ) ;
#7226=CARTESIAN_POINT ( 'NONE',  ( 37.00000000000000711, 7.146664589317909488, -9.321877890560465119 ) ) ;
#7228=PLANE ( 'NONE',  #58312 ) ;
#7229=DIRECTION ( 'NONE',  ( 0.000000000000000000, 0.01356324068817992522, -0.9999080150203990547 ) ) ;
#7230=EDGE_CURVE ( 'NONE', #33155, #19644, #61645, .T. ) ;
#7231=VERTEX_POINT ( 'NONE', #50254 ) ;
#7232=EDGE_LOOP ( 'NONE', ( #14773, #39236, #11311, #55159 ) ) ;
#7234=EDGE_LOOP ( 'NONE', ( #16277, #61881, #32297, #5411 ) ) ;
#7235=CARTESIAN_POINT ( 'NONE',  ( -37.00000000000000711, 12.16893194857550142, 3.805206332242515366 ) ) ;
#7236=DIRECTION ( 'NONE',  ( 0.000000000000000000, -0.6943713148249690548, 0.7196168960969744344 ) ) ;
#7238=FACE_OUTER_BOUND ( 'NONE', #32430, .T. ) ;
#7240=CARTESIAN_POINT ( 'NONE',  ( -4.806344283790351390, -7.508992741355383416, 25.00000000000000000 ) ) ;
#7241=CARTESIAN_POINT ( 'NONE',  ( -18.04458733766117362, 12.91933584589294703, 3.916728392552376370 ) ) ;
#7242=EDGE_LOOP ( 'NONE', ( #3994, #8994, #8240, #1706 ) ) ;
#7243=ORIENTED_EDGE ( 'NONE', *, *, #37172, .T. ) ;
#7244=CARTESIAN_POINT ( 'NONE',  ( 35.00000000000000000, 1.039216533672905785, -11.70009620280412221 ) ) ;
#7245=ORIENTED_EDGE ( 'NONE', *, *, #29515, .F. ) ;
#7249=DIRECTION ( 'NONE',  ( -0.000000000000000000, -1.000000000000000000, -0.000000000000000000 ) ) ;
#7252=DIRECTION ( 'NONE',  ( 1.000000000000000000, -0.000000000000000000, 0.000000000000000000 ) ) ;
#7257=VERTEX_POINT ( 'NONE', #61509 ) ;
#7259=CARTESIAN_POINT ( 'NONE',  ( -16.98800322446194855, 2.922502605998049674, -11.63868456991314027 ) ) ;
#7260=EDGE_CURVE ( 'NONE', #49200, #27489, #26278, .T. ) ;
#7266=CARTESIAN_POINT ( 'NONE',  ( 35.00000000000000000, 4.705694406421931860E-17, -3.469127814946512892E-15 ) ) ;
#7268=CIRCLE ( 'NONE', #51863, 5.000000000000000000 ) ;
#7269=CARTESIAN_POINT ( 'NONE',  ( 36.00000000000000711, 10.12742074351896449, -7.745827850123049529 ) ) ;
#7270=FACE_OUTER_BOUND ( 'NONE', #63258, .T. ) ;
#7271=EDGE_CURVE ( 'NONE', #39378, #9622, #52123, .T. ) ;
#7272=CARTESIAN_POINT ( 'NONE',  ( -37.00000000000000711, -10.93004082984014147, -6.564808257521884904 ) ) ;
#7273=LINE ( 'NONE', #1975, #43934 ) ;
#7274=AXIS2_PLACEMENT_3D ( 'NONE', #26, #16317, #40251 ) ;
#7275=AXIS2_PLACEMENT_3D ( 'NONE', #16090, #31698, #36378 ) ;
#7276=ORIENTED_EDGE ( 'NONE', *, *, #22198, .T. ) ;
#7277=CARTESIAN_POINT ( 'NONE',  ( -35.00000000000000000, 10.25474254703952859, 6.584150480049587806 ) ) ;
#7279=AXIS2_PLACEMENT_3D ( 'NONE', #54886, #5332, #19653 ) ;
#7281=EDGE_CURVE ( 'NONE', #49136, #5918, #64863, .T. ) ;
#7285=CIRCLE ( 'NONE', #15769, 12.75000000000000178 ) ;
#7287=DIRECTION ( 'NONE',  ( 1.000000000000000000, 0.000000000000000000, 0.000000000000000000 ) ) ;
#7289=DIRECTION ( 'NONE',  ( -1.000000000000000000, 0.000000000000000000, 0.000000000000000000 ) ) ;
#7290=DIRECTION ( 'NONE',  ( 0.000000000000000000, -0.01356324068817991828, 0.9999080150203990547 ) ) ;
#7291=CARTESIAN_POINT ( 'NONE',  ( 12.52916646628448127, -13.04480612694435671, -3.481077218509882165 ) ) ;
#7294=ORIENTED_EDGE ( 'NONE', *, *, #15988, .T. ) ;
#7295=DIRECTION ( 'NONE',  ( 1.000000000000000000, 0.000000000000000000, 0.000000000000000000 ) ) ;
#7297=DIRECTION ( 'NONE',  ( 0.000000000000000000, -0.9999080150203992767, -0.01356324068816951341 ) ) ;
#7298=CARTESIAN_POINT ( 'NONE',  ( -3.936294612518189684, 11.99894110015778814, 6.199062502346824211 ) ) ;
#7300=DIRECTION ( 'NONE',  ( 0.000000000000000000, -0.2960891610144378849, -0.9551603052523520709 ) ) ;
#7301=ORIENTED_EDGE ( 'NONE', *, *, #6444, .T. ) ;
#7302=CIRCLE ( 'NONE', #44457, 4.999999999999999112 ) ;
#7307=EDGE_CURVE ( 'NONE', #18956, #48492, #48954, .T. ) ;
#7308=ORIENTED_EDGE ( 'NONE', *, *, #47313, .F. ) ;
#7309=CARTESIAN_POINT ( 'NONE',  ( -9.730999143771754234, 11.41738891610202344, -7.214510183280433253 ) ) ;
#7310=ORIENTED_EDGE ( 'NONE', *, *, #63153, .F. ) ;
#7311=DIRECTION ( 'NONE',  ( 0.000000000000000000, 0.01356324068817991828, -0.9999080150203990547 ) ) ;
#7316=VERTEX_POINT ( 'NONE', #32547 ) ;
#7318=CIRCLE ( 'NONE', #43440, 4.999999999999999112 ) ;
#7319=ORIENTED_EDGE ( 'NONE', *, *, #4712, .F. ) ;
#7320=CARTESIAN_POINT ( 'NONE',  ( 36.00000000000000711, 0.4871980014161481631, -12.74068829017554272 ) ) ;
#7321=CARTESIAN_POINT ( 'NONE',  ( -36.00000000000000711, -11.24036214326516436, -6.018036132182281506 ) ) ;
#7323=ORIENTED_EDGE ( 'NONE', *, *, #62677, .F. ) ;
#7328=EDGE_CURVE ( 'NONE', #4893, #58346, #26618, .T. ) ;
#7330=CARTESIAN_POINT ( 'NONE',  ( 22.21055375121777686, -11.96926186085320154, -0.8606626411553354172 ) ) ;
#7331=DIRECTION ( 'NONE',  ( 1.000000000000000000, 0.000000000000000000, 0.000000000000000000 ) ) ;
#7332=ORIENTED_EDGE ( 'NONE', *, *, #41595, .F. ) ;
#7334=CARTESIAN_POINT ( 'NONE',  ( -35.00000000000000000, -12.08216339958899788, -1.591260454995368390 ) ) ;
#7335=ADVANCED_FACE ( 'NONE', ( #43516 ), #43193, .T. ) ;
#7337=CARTESIAN_POINT ( 'NONE',  ( -19.30822655423815348, 11.87722838305601591, -1.744063228020214185 ) ) ;
#7338=VERTEX_POINT ( 'NONE', #38203 ) ;
#7341=CARTESIAN_POINT ( 'NONE',  ( 37.00000000000000711, -10.92721691015452912, 4.309077947445766554 ) ) ;
#7343=CARTESIAN_POINT ( 'NONE',  ( -35.00000000000000000, 0.000000000000000000, 0.000000000000000000 ) ) ;
#7345=EDGE_CURVE ( 'NONE', #43267, #56626, #31919, .T. ) ;
#7347=CARTESIAN_POINT ( 'NONE',  ( 37.00000000000000711, 4.705694406421931860E-17, -3.469127814946512892E-15 ) ) ;
#7349=DIRECTION ( 'NONE',  ( 0.000000000000000000, -1.000000000000000000, 0.000000000000000000 ) ) ;
#7350=ORIENTED_EDGE ( 'NONE', *, *, #10696, .F. ) ;
#7351=CARTESIAN_POINT ( 'NONE',  ( 35.00000000000000000, -1.171570255487531131, -11.68758509253248157 ) ) ;
#7353=CARTESIAN_POINT ( 'NONE',  ( 35.00000000000000000, 3.645068577060024850, -11.16627499335656815 ) ) ;
#7355=DIRECTION ( 'NONE',  ( -1.000000000000000000, 0.000000000000000000, 0.000000000000000000 ) ) ;
#7358=CIRCLE ( 'NONE', #29660, 12.18650000000000055 ) ;
#7361=CARTESIAN_POINT ( 'NONE',  ( 35.00000000000000000, 4.309077947445811851, 10.92721691015450780 ) ) ;
#7362=EDGE_CURVE ( 'NONE', #58571, #61612, #62727, .T. ) ;
#7364=( BOUNDED_CURVE ( )  B_SPLINE_CURVE ( 3, ( #56966, #770, #11708, #62257 ),
 .UNSPECIFIED., .F., .F. ) 
 B_SPLINE_CURVE_WITH_KNOTS ( ( 4, 4 ),
 ( 4.028742991341328405, 4.061025088278432449 ),
 .UNSPECIFIED. ) 
 CURVE ( )  GEOMETRIC_REPRESENTATION_ITEM ( )  RATIONAL_B_SPLINE_CURVE ( ( 1.000000000000000000, 0.9999131574035865500, 0.9999131574035865500, 1.000000000000000000 ) ) 
 REPRESENTATION_ITEM ( '' )  );
#7367=CYLINDRICAL_SURFACE ( 'NONE', #11177, 12.75000000000000178 ) ;
#7368=DIRECTION ( 'NONE',  ( 0.000000000000000000, -0.01356324068817998940, 0.9999080150203990547 ) ) ;
#7369=CARTESIAN_POINT ( 'NONE',  ( -18.41858249652232615, -5.215518226302011229, 10.80810004108996125 ) ) ;
#7372=CARTESIAN_POINT ( 'NONE',  ( -35.00000000000000000, -7.717887834988307105, 8.854740511458828678 ) ) ;
#7374=DIRECTION ( 'NONE',  ( 0.000000000000000000, -0.01356324068817991828, 0.9999080150203990547 ) ) ;
#7376=DIRECTION ( 'NONE',  ( 0.000000000000000000, -0.9847383929261599445, 0.1740410799127720953 ) ) ;
#7377=CYLINDRICAL_SURFACE ( 'NONE', #25639, 4.999999999999999112 ) ;
#7381=EDGE_CURVE ( 'NONE', #58319, #21005, #19248, .T. ) ;
#7382=AXIS2_PLACEMENT_3D ( 'NONE', #62313, #52690, #2134 ) ;
#7385=CARTESIAN_POINT ( 'NONE',  ( 5.632405787856444412, -9.296918358879166178, 9.794213099898851027 ) ) ;
#7387=AXIS2_PLACEMENT_3D ( 'NONE', #51485, #10541, #16206 ) ;
#7388=DIRECTION ( 'NONE',  ( -1.000000000000000000, -0.000000000000000000, 0.000000000000000000 ) ) ;
#7390=EDGE_LOOP ( 'NONE', ( #27137, #43168, #47001, #57148 ) ) ;
#7392=EDGE_LOOP ( 'NONE', ( #45874, #47356, #65473, #6330 ) ) ;
#7393=CARTESIAN_POINT ( 'NONE',  ( -35.00000000000000000, -4.545979934229492869, 11.30684963584387681 ) ) ;
#7395=EDGE_LOOP ( 'NONE', ( #2775, #14574, #1258, #15762 ) ) ;
#7396=CARTESIAN_POINT ( 'NONE',  ( 37.00000000000000711, -7.718225330433870823, -9.430788938294027091 ) ) ;
#7398=ORIENTED_EDGE ( 'NONE', *, *, #44516, .T. ) ;
#7400=CARTESIAN_POINT ( 'NONE',  ( 35.00000000000000000, 5.710938531231874116, 11.39945968423464784 ) ) ;
#7401=CIRCLE ( 'NONE', #53085, 5.000000000000000000 ) ;
#7403=FACE_OUTER_BOUND ( 'NONE', #63574, .T. ) ;
#7405=FACE_OUTER_BOUND ( 'NONE', #39946, .T. ) ;
#7406=ADVANCED_FACE ( 'NONE', ( #18622 ), #28895, .T. ) ;
#7407=DIRECTION ( 'NONE',  ( 1.000000000000000000, 0.000000000000000000, 0.000000000000000000 ) ) ;
#7408=B_SPLINE_CURVE_WITH_KNOTS ( 'NONE', 3,
 ( #19689, #14650, #60230, #4055 ),
 .UNSPECIFIED., .F., .F.,
 ( 4, 4 ),
 ( 1.734723475976807094E-18, 0.002404377236383827953 ),
 .UNSPECIFIED. ) ;
#7410=CARTESIAN_POINT ( 'NONE',  ( 35.00000000000000000, -11.95840593935202811, -2.346765782874394635 ) ) ;
#7413=EDGE_CURVE ( 'NONE', #56567, #41081, #45744, .T. ) ;
#7415=CARTESIAN_POINT ( 'NONE',  ( 35.00000000000000000, -1.039216533672818299, 11.70009620280412399 ) ) ;
#7416=ORIENTED_EDGE ( 'NONE', *, *, #58570, .T. ) ;
#7420=VERTEX_POINT ( 'NONE', #33873 ) ;
#7424=ORIENTED_EDGE ( 'NONE', *, *, #43826, .T. ) ;
#7425=ORIENTED_EDGE ( 'NONE', *, *, #35653, .T. ) ;
#7428=ADVANCED_FACE ( 'NONE', ( #49205 ), #29227, .T. ) ;
#7430=VERTEX_POINT ( 'NONE', #9564 ) ;
#7431=CARTESIAN_POINT ( 'NONE',  ( -3.740102306720532788, 25.00000000000000000, -6.044082642436763742 ) ) ;
#7432=CARTESIAN_POINT ( 'NONE',  ( -35.00000000000000000, -6.584150480049623333, 10.25474254703950905 ) ) ;
#7433=CARTESIAN_POINT ( 'NONE',  ( 36.00000000000000711, -4.400442035670862673, 11.96656215839372983 ) ) ;
#7435=ADVANCED_FACE ( 'NONE', ( #44185 ), #64453, .T. ) ;
#7436=DIRECTION ( 'NONE',  ( 1.000000000000000000, -0.000000000000000000, -0.000000000000000000 ) ) ;
#7438=VECTOR ( 'NONE', #50087, 1000.000000000000000 ) ;
#7439=AXIS2_PLACEMENT_3D ( 'NONE', #2900, #21865, #42109 ) ;
#7444=CARTESIAN_POINT ( 'NONE',  ( 35.00000000000000000, 5.273331777780336793, -10.49591321039682690 ) ) ;
#7445=DIRECTION ( 'NONE',  ( 0.000000000000000000, 0.01356324068817998940, -0.9999080150203990547 ) ) ;
#7446=CIRCLE ( 'NONE', #44599, 12.00000000000000000 ) ;
#7447=DIRECTION ( 'NONE',  ( -1.000000000000000000, 0.000000000000000000, 0.000000000000000000 ) ) ;
#7448=CARTESIAN_POINT ( 'NONE',  ( -35.00000000000000000, -11.05394794832833583, 5.130401251914692651 ) ) ;
#7450=CIRCLE ( 'NONE', #60528, 12.18649999999999878 ) ;
#7451=CYLINDRICAL_SURFACE ( 'NONE', #44737, 4.999999999999999112 ) ;
#7453=ORIENTED_EDGE ( 'NONE', *, *, #36672, .T. ) ;
#7454=CARTESIAN_POINT ( 'NONE',  ( -27.01437459610461644, 25.00000000000000000, -2.220455681983952267 ) ) ;
#7456=LINE ( 'NONE', #18465, #19466 ) ;
#7458=CIRCLE ( 'NONE', #30803, 12.74999999999999822 ) ;
#7461=DIRECTION ( 'NONE',  ( 0.000000000000000000, -0.9551603052523510717, 0.2960891610144409936 ) ) ;
#7462=CARTESIAN_POINT ( 'NONE',  ( -35.00000000000000000, 11.73808581813437968, -0.4353888892048790038 ) ) ;
#7465=CARTESIAN_POINT ( 'NONE',  ( 18.12964925673133010, -7.571604912534921183, 9.321062701759899483 ) ) ;
#7469=ORIENTED_EDGE ( 'NONE', *, *, #7755, .T. ) ;
#7470=CYLINDRICAL_SURFACE ( 'NONE', #38236, 13.50000000000000178 ) ;
#7477=AXIS2_PLACEMENT_3D ( 'NONE', #47481, #53114, #27187 ) ;
#7478=CIRCLE ( 'NONE', #16027, 12.75000000000000178 ) ;
#7480=ORIENTED_EDGE ( 'NONE', *, *, #28389, .F. ) ;
#7481=CYLINDRICAL_SURFACE ( 'NONE', #13232, 12.18650000000000055 ) ;
#7482=LINE ( 'NONE', #8153, #52729 ) ;
#7485=CARTESIAN_POINT ( 'NONE',  ( 37.00000000000000711, -12.57916205664482767, -2.080187960898521649 ) ) ;
#7490=ADVANCED_FACE ( 'NONE', ( #31190 ), #10899, .F. ) ;
#7491=VERTEX_POINT ( 'NONE', #283 ) ;
#7494=EDGE_LOOP ( 'NONE', ( #50657, #58047, #20022, #41351 ) ) ;
#7496=CARTESIAN_POINT ( 'NONE',  ( -2.952869152607107139, -12.96714474214480717, 3.755417052241487585 ) ) ;
#7497=VECTOR ( 'NONE', #42389, 1000.000000000000000 ) ;
#7501=DIRECTION ( 'NONE',  ( -1.000000000000000000, 0.000000000000000000, 0.000000000000000000 ) ) ;
#7505=FACE_OUTER_BOUND ( 'NONE', #43251, .T. ) ;
#7506=DIRECTION ( 'NONE',  ( 0.000000000000000000, 0.01356324068818000328, -0.9999080150203990547 ) ) ;
#7509=ORIENTED_EDGE ( 'NONE', *, *, #14104, .F. ) ;
#7510=AXIS2_PLACEMENT_3D ( 'NONE', #20713, #56954, #65581 ) ;
#7512=VERTEX_POINT ( 'NONE', #46165 ) ;
#7513=DIRECTION ( 'NONE',  ( 0.000000000000000000, -0.9651210252299821102, -0.2618041379715529970 ) ) ;
#7514=DIRECTION ( 'NONE',  ( -1.000000000000000000, 0.000000000000000000, 0.000000000000000000 ) ) ;
#7515=DIRECTION ( 'NONE',  ( 1.000000000000000000, 0.000000000000000000, 0.000000000000000000 ) ) ;
#7516=EDGE_CURVE ( 'NONE', #14900, #23975, #57435, .T. ) ;
#7517=DIRECTION ( 'NONE',  ( 0.000000000000000000, -0.01356324068817998940, 0.9999080150203990547 ) ) ;
#7518=DIRECTION ( 'NONE',  ( 0.000000000000000000, -0.01356324068817998940, 0.9999080150203990547 ) ) ;
#7521=DIRECTION ( 'NONE',  ( 0.000000000000000000, 0.01356324068817992001, -0.9999080150203990547 ) ) ;
#7527=CIRCLE ( 'NONE', #62775, 12.74999999999999822 ) ;
#7528=DIRECTION ( 'NONE',  ( 0.000000000000000000, -1.000000000000000000, 0.000000000000000000 ) ) ;
#7529=CYLINDRICAL_SURFACE ( 'NONE', #18978, 4.999999999999999112 ) ;
#7530=CARTESIAN_POINT ( 'NONE',  ( 36.00000000000000711, -7.882940143791699050, 10.02106554660717030 ) ) ;
#7531=CARTESIAN_POINT ( 'NONE',  ( -35.00000000000000000, -11.73808581813438323, 0.4353888892047964587 ) ) ;
#7532=VERTEX_POINT ( 'NONE', #20217 ) ;
#7535=AXIS2_PLACEMENT_3D ( 'NONE', #61705, #62053, #36772 ) ;
#7537=ORIENTED_EDGE ( 'NONE', *, *, #16997, .F. ) ;
#7538=CIRCLE ( 'NONE', #15874, 5.000000000000001776 ) ;
#7540=CARTESIAN_POINT ( 'NONE',  ( -28.56473390530002021, 3.589939350442142185, -11.45074047018220753 ) ) ;
#7541=DIRECTION ( 'NONE',  ( 0.000000000000000000, -0.9847383929261636082, 0.1740410799127514174 ) ) ;
#7542=CARTESIAN_POINT ( 'NONE',  ( -37.00000000000000711, -8.389074212634351824, 8.839356091080015076 ) ) ;
#7546=CARTESIAN_POINT ( 'NONE',  ( 2.798553295784531159, 25.00000000000000000, 7.462808788758677814 ) ) ;
#7547=CYLINDRICAL_SURFACE ( 'NONE', #64638, 13.50000000000000178 ) ;
#7548=AXIS2_PLACEMENT_3D ( 'NONE', #20839, #1226, #6214 ) ;
#7549=CIRCLE ( 'NONE', #32976, 12.75000000000000178 ) ;
#7551=EDGE_CURVE ( 'NONE', #27477, #29748, #20558, .T. ) ;
#7554=ADVANCED_FACE ( 'NONE', ( #62103 ), #25531, .T. ) ;
#7557=VERTEX_POINT ( 'NONE', #45479 ) ;
#7559=CARTESIAN_POINT ( 'NONE',  ( 29.51976981715666781, 7.690765383426390045, 11.09513982864076276 ) ) ;
#7560=CIRCLE ( 'NONE', #11775, 12.74999999999999822 ) ;
#7561=CARTESIAN_POINT ( 'NONE',  ( -36.00000000000000711, -12.46157735505191333, 2.696588552979013009 ) ) ;
#7562=ORIENTED_EDGE ( 'NONE', *, *, #21431, .T. ) ;
#7564=CARTESIAN_POINT ( 'NONE',  ( -35.00000000000000000, 0.000000000000000000, 0.000000000000000000 ) ) ;
#7567=EDGE_CURVE ( 'NONE', #33417, #59719, #35508, .T. ) ;
#7568=CARTESIAN_POINT ( 'NONE',  ( -29.95711186975066198, 0.8286516086034492190, -13.48164454051215877 ) ) ;
#7570=VERTEX_POINT ( 'NONE', #58100 ) ;
#7571=ORIENTED_EDGE ( 'NONE', *, *, #44421, .F. ) ;
#7575=DIRECTION ( 'NONE',  ( -1.000000000000000000, 0.000000000000000000, 0.000000000000000000 ) ) ;
#7576=CARTESIAN_POINT ( 'NONE',  ( -35.00000000000000000, 0.000000000000000000, 0.000000000000000000 ) ) ;
#7577=DIRECTION ( 'NONE',  ( 1.000000000000000000, 0.000000000000000000, 0.000000000000000000 ) ) ;
#7578=( BOUNDED_CURVE ( )  B_SPLINE_CURVE ( 3, ( #62018, #21452, #6824, #26765 ),
 .UNSPECIFIED., .F., .F. ) 
 B_SPLINE_CURVE_WITH_KNOTS ( ( 4, 4 ),
 ( 1.570796326794895892, 1.612255705401422601 ),
 .UNSPECIFIED. ) 
 CURVE ( )  GEOMETRIC_REPRESENTATION_ITEM ( )  RATIONAL_B_SPLINE_CURVE ( ( 1.000000000000000000, 0.9998567651231480280, 0.9998567651231480280, 1.000000000000000000 ) ) 
 REPRESENTATION_ITEM ( '' )  );
#7582=DIRECTION ( 'NONE',  ( 0.000000000000000000, 0.7381862504171974315, -0.6745969609292639113 ) ) ;
#7583=ORIENTED_EDGE ( 'NONE', *, *, #8335, .F. ) ;
#7585=EDGE_CURVE ( 'NONE', #20717, #40151, #37241, .T. ) ;
#7586=EDGE_CURVE ( 'NONE', #9622, #21959, #12513, .T. ) ;
#7588=DIRECTION ( 'NONE',  ( 1.000000000000000000, 0.000000000000000000, 0.000000000000000000 ) ) ;
#7592=CIRCLE ( 'NONE', #41567, 5.000000000000000888 ) ;
#7594=AXIS2_PLACEMENT_3D ( 'NONE', #59090, #54427, #44404 ) ;
#7595=CARTESIAN_POINT ( 'NONE',  ( 37.00000000000000711, -1.591260454995155671, 12.08216339958901742 ) ) ;
#7596=ORIENTED_EDGE ( 'NONE', *, *, #31727, .F. ) ;
#7597=CARTESIAN_POINT ( 'NONE',  ( -37.00000000000000711, 0.000000000000000000, 0.000000000000000000 ) ) ;
#7599=DIRECTION ( 'NONE',  ( 0.000000000000000000, 0.07632122047555796318, -0.9970832820307042876 ) ) ;
#7600=ORIENTED_EDGE ( 'NONE', *, *, #43212, .T. ) ;
#7602=DIRECTION ( 'NONE',  ( 0.000000000000000000, 0.01356324068817998940, -0.9999080150203990547 ) ) ;
#7603=ORIENTED_EDGE ( 'NONE', *, *, #35830, .F. ) ;
#7605=ORIENTED_EDGE ( 'NONE', *, *, #44065, .F. ) ;
#7606=ORIENTED_EDGE ( 'NONE', *, *, #13868, .T. ) ;
#7607=VECTOR ( 'NONE', #26814, 1000.000000000000000 ) ;
#7611=CIRCLE ( 'NONE', #13946, 12.18650000000000055 ) ;
#7613=CARTESIAN_POINT ( 'NONE',  ( 12.93723047338301058, 4.476360154859203355, 25.00000000000000000 ) ) ;
#7616=CIRCLE ( 'NONE', #38403, 5.000000000000000888 ) ;
#7619=ORIENTED_EDGE ( 'NONE', *, *, #55231, .T. ) ;
#7620=DIRECTION ( 'NONE',  ( -1.000000000000000000, -0.000000000000000000, 0.000000000000000000 ) ) ;
#7622=VECTOR ( 'NONE', #28432, 1000.000000000000000 ) ;
#7623=DIRECTION ( 'NONE',  ( 0.000000000000000000, -0.01356324068817992175, 0.9999080150203990547 ) ) ;
#7624=DIRECTION ( 'NONE',  ( 0.000000000000000000, 0.6478160128811893959, -0.7617968321374923857 ) ) ;
#7625=CARTESIAN_POINT ( 'NONE',  ( -35.00000000000000000, -9.390600770287930388, -8.624332853796161658 ) ) ;
#7626=CARTESIAN_POINT ( 'NONE',  ( 35.00000000000000000, -11.02904044024205987, 4.041347439435972966 ) ) ;
#7627=CIRCLE ( 'NONE', #51161, 12.18649999999999878 ) ;
#7629=DIRECTION ( 'NONE',  ( 0.000000000000000000, -0.01356324068817991828, 0.9999080150203990547 ) ) ;
#7631=ORIENTED_EDGE ( 'NONE', *, *, #65309, .T. ) ;
#7635=CARTESIAN_POINT ( 'NONE',  ( -11.08072612429806014, -9.571970673523852113, 7.260798853501513328 ) ) ;
#7637=FACE_OUTER_BOUND ( 'NONE', #55001, .T. ) ;
#7639=CARTESIAN_POINT ( 'NONE',  ( -35.00000000000000000, 7.110831038798278492, 9.896810808925417646 ) ) ;
#7640=ORIENTED_EDGE ( 'NONE', *, *, #24222, .F. ) ;
#7641=DIRECTION ( 'NONE',  ( 0.000000000000000000, -0.01356324068817999114, 0.9999080150203989437 ) ) ;
#7642=CARTESIAN_POINT ( 'NONE',  ( 37.00000000000000711, 12.54989509947654192, 2.250029553613615452 ) ) ;
#7645=VECTOR ( 'NONE', #42379, 1000.000000000000000 ) ;
#7646=CIRCLE ( 'NONE', #12956, 12.18649999999999878 ) ;
#7647=AXIS2_PLACEMENT_3D ( 'NONE', #43966, #22352, #13687 ) ;
#7650=ORIENTED_EDGE ( 'NONE', *, *, #60671, .T. ) ;
#7654=VECTOR ( 'NONE', #37176, 1000.000000000000000 ) ;
#7655=AXIS2_PLACEMENT_3D ( 'NONE', #4961, #25223, #45497 ) ;
#7657=VERTEX_POINT ( 'NONE', #27176 ) ;
#7658=AXIS2_PLACEMENT_3D ( 'NONE', #36980, #15401, #20727 ) ;
#7659=FACE_OUTER_BOUND ( 'NONE', #29655, .T. ) ;
#7664=DIRECTION ( 'NONE',  ( -1.000000000000000000, -0.000000000000000000, 0.000000000000000000 ) ) ;
#7665=CIRCLE ( 'NONE', #17203, 12.74999999999999822 ) ;
#7666=CARTESIAN_POINT ( 'NONE',  ( 37.00000000000000711, 9.390600770288115129, 8.624332853795948495 ) ) ;
#7668=EDGE_CURVE ( 'NONE', #53854, #22894, #39376, .T. ) ;
#7669=AXIS2_PLACEMENT_3D ( 'NONE', #43852, #64136, #18614 ) ;
#7670=EDGE_LOOP ( 'NONE', ( #2380, #10607, #41145, #50326 ) ) ;
#7673=DIRECTION ( 'NONE',  ( 0.000000000000000000, 0.01356324068817998940, -0.9999080150203990547 ) ) ;
#7674=ORIENTED_EDGE ( 'NONE', *, *, #49298, .T. ) ;
#7678=ORIENTED_EDGE ( 'NONE', *, *, #12198, .F. ) ;
#7681=CARTESIAN_POINT ( 'NONE',  ( 36.00000000000000711, 8.830544224263075392, 9.196955404009196755 ) ) ;
#7682=VERTEX_POINT ( 'NONE', #2590 ) ;
#7683=ORIENTED_EDGE ( 'NONE', *, *, #55574, .T. ) ;
#7684=CARTESIAN_POINT ( 'NONE',  ( 37.00000000000000711, 4.426194442447407340, 11.35427606708800852 ) ) ;
#7685=ORIENTED_EDGE ( 'NONE', *, *, #49636, .T. ) ;
#7688=AXIS2_PLACEMENT_3D ( 'NONE', #48411, #18137, #2862 ) ;
#7691=EDGE_CURVE ( 'NONE', #11726, #49219, #56376, .T. ) ;
#7694=CARTESIAN_POINT ( 'NONE',  ( 37.00000000000000711, -12.42372387097884001, -2.865935305911582631 ) ) ;
#7697=DIRECTION ( 'NONE',  ( 0.000000000000000000, -1.000000000000000000, 0.000000000000000000 ) ) ;
#7698=CARTESIAN_POINT ( 'NONE',  ( -27.39679304536733540, -9.459809594864578841, -7.405314960163760674 ) ) ;
#7700=DIRECTION ( 'NONE',  ( 0.000000000000000000, -0.01356324068817992175, 0.9999080150203990547 ) ) ;
#7701=VERTEX_POINT ( 'NONE', #38117 ) ;
#7705=CARTESIAN_POINT ( 'NONE',  ( -16.35697571030837594, 8.282848916715964904, 8.683172938416127806 ) ) ;
#7706=CARTESIAN_POINT ( 'NONE',  ( -37.00000000000000711, -2.220215194441820916, -11.98254675519230616 ) ) ;
#7707=CARTESIAN_POINT ( 'NONE',  ( 35.00000000000000000, 0.2661492558803343345, -12.18359334611896649 ) ) ;
#7708=CIRCLE ( 'NONE', #44855, 5.000000000000000888 ) ;
#7709=ORIENTED_EDGE ( 'NONE', *, *, #34292, .F. ) ;
#7710=ADVANCED_FACE ( 'NONE', ( #32146 ), #1601, .T. ) ;
#7712=ORIENTED_EDGE ( 'NONE', *, *, #20674, .T. ) ;
#7714=AXIS2_PLACEMENT_3D ( 'NONE', #20678, #36619, #47274 ) ;
#7715=VERTEX_POINT ( 'NONE', #17200 ) ;
#7716=CARTESIAN_POINT ( 'NONE',  ( 145.1370849898475797, 3.309064568108273190E-14, 0.000000000000000000 ) ) ;
#7717=VECTOR ( 'NONE', #44461, 1000.000000000000000 ) ;
#7718=DIRECTION ( 'NONE',  ( 0.000000000000000000, 0.01356324068817998940, -0.9999080150203990547 ) ) ;
#7720=CARTESIAN_POINT ( 'NONE',  ( -7.489022030332961322, 5.127957880411581293, -10.84914964302385521 ) ) ;
#7723=AXIS2_PLACEMENT_3D ( 'NONE', #31054, #1129, #10430 ) ;
#7724=ADVANCED_FACE ( 'NONE', ( #57784 ), #3228, .T. ) ;
#7726=CARTESIAN_POINT ( 'NONE',  ( 21.97889514767880925, 13.29909890247968285, -2.348602380154369396 ) ) ;
#7728=EDGE_CURVE ( 'NONE', #35757, #23816, #36751, .T. ) ;
#7732=VECTOR ( 'NONE', #35998, 1000.000000000000000 ) ;
#7733=AXIS2_PLACEMENT_3D ( 'NONE', #402, #20331, #25323 ) ;
#7734=B_SPLINE_CURVE_WITH_KNOTS ( 'NONE', 3,
 ( #58650, #9061, #53320, #4078, #63934, #23723 ),
 .UNSPECIFIED., .F., .F.,
 ( 4, 2, 4 ),
 ( 0.005173693434891112747, 0.006312000079627475523, 0.007450306724363838298 ),
 .UNSPECIFIED. ) ;
#7735=AXIS2_PLACEMENT_3D ( 'NONE', #5869, #47401, #51073 ) ;
#7736=AXIS2_PLACEMENT_3D ( 'NONE', #56570, #25001, #65532 ) ;
#7737=ADVANCED_FACE ( 'NONE', ( #54750 ), #64371, .T. ) ;
#7738=EDGE_LOOP ( 'NONE', ( #13398, #1922, #21836, #58608 ) ) ;
#7740=VERTEX_POINT ( 'NONE', #23500 ) ;
#7741=CYLINDRICAL_SURFACE ( 'NONE', #34222, 12.18649999999999878 ) ;
#7743=CARTESIAN_POINT ( 'NONE',  ( 32.00000000000000000, -11.99999999999997513, 0.000000000000000000 ) ) ;
#7748=DIRECTION ( 'NONE',  ( -1.000000000000000000, 0.000000000000000000, 0.000000000000000000 ) ) ;
#7754=ORIENTED_EDGE ( 'NONE', *, *, #19383, .F. ) ;
#7755=EDGE_CURVE ( 'NONE', #57555, #54366, #20026, .T. ) ;
#7758=CYLINDRICAL_SURFACE ( 'NONE', #6816, 13.50000000000000178 ) ;
#7759=DIRECTION ( 'NONE',  ( 0.000000000000000000, -0.8369827122275287357, -0.5472293298355360713 ) ) ;
#7760=EDGE_LOOP ( 'NONE', ( #40395, #54620, #17923, #51750 ) ) ;
#7765=FACE_OUTER_BOUND ( 'NONE', #7760, .T. ) ;
#7768=ORIENTED_EDGE ( 'NONE', *, *, #54154, .F. ) ;
#7769=CARTESIAN_POINT ( 'NONE',  ( -17.61945576107935452, 13.14228823968358384, 3.170957093146434147 ) ) ;
#7770=ORIENTED_EDGE ( 'NONE', *, *, #16135, .T. ) ;
#7771=DIRECTION ( 'NONE',  ( -1.000000000000000000, -0.000000000000000000, -0.000000000000000000 ) ) ;
#7772=DIRECTION ( 'NONE',  ( 0.000000000000000000, -0.01356324068817999114, 0.9999080150203989437 ) ) ;
#7773=CYLINDRICAL_SURFACE ( 'NONE', #47835, 12.18650000000000055 ) ;
#7775=CIRCLE ( 'NONE', #5703, 5.000000000000000000 ) ;
#7777=CYLINDRICAL_SURFACE ( 'NONE', #48442, 4.999999999999999112 ) ;
#7782=ORIENTED_EDGE ( 'NONE', *, *, #37005, .T. ) ;
#7783=AXIS2_PLACEMENT_3D ( 'NONE', #27276, #28588, #22633 ) ;
#7785=CARTESIAN_POINT ( 'NONE',  ( 18.98898312442693737, -6.102278294184944940, 12.04338967756598500 ) ) ;
#7788=CARTESIAN_POINT ( 'NONE',  ( 35.00000000000000000, -10.28547182238011715, -5.672855678558653914 ) ) ;
#7791=AXIS2_PLACEMENT_3D ( 'NONE', #4804, #24740, #14725 ) ;
#7793=CYLINDRICAL_SURFACE ( 'NONE', #29923, 5.000000000000000888 ) ;
#7794=AXIS2_PLACEMENT_3D ( 'NONE', #32179, #52808, #52504 ) ;
#7795=DIRECTION ( 'NONE',  ( 1.000000000000000000, 0.000000000000000000, -0.000000000000000000 ) ) ;
#7797=AXIS2_PLACEMENT_3D ( 'NONE', #56194, #20944, #57199 ) ;
#7798=CARTESIAN_POINT ( 'NONE',  ( -37.00000000000000711, 9.700295462048664774, 7.376655759824919834 ) ) ;
#7799=CARTESIAN_POINT ( 'NONE',  ( -37.00000000000000711, -12.60630747491664572, 1.908798535168333643 ) ) ;
#7800=AXIS2_PLACEMENT_3D ( 'NONE', #21491, #6522, #41759 ) ;
#7802=DIRECTION ( 'NONE',  ( 1.000000000000000000, -0.000000000000000000, 0.000000000000000000 ) ) ;
#7803=EDGE_CURVE ( 'NONE', #12091, #28250, #49119, .T. ) ;
#7805=AXIS2_PLACEMENT_3D ( 'NONE', #6443, #32351, #47016 ) ;
#7806=FACE_OUTER_BOUND ( 'NONE', #31645, .T. ) ;
#7807=ADVANCED_FACE ( 'NONE', ( #40405 ), #41065, .T. ) ;
#7808=CIRCLE ( 'NONE', #50301, 5.000000000000000888 ) ;
#7810=ADVANCED_FACE ( 'NONE', ( #60709 ), #197, .T. ) ;
#7814=FACE_OUTER_BOUND ( 'NONE', #19196, .T. ) ;
#7816=CIRCLE ( 'NONE', #13120, 12.75000000000000178 ) ;
#7818=CARTESIAN_POINT ( 'NONE',  ( -37.00000000000000711, 0.000000000000000000, 0.000000000000000000 ) ) ;
#7819=CARTESIAN_POINT ( 'NONE',  ( -24.87682914247800881, -10.97525152144739202, 7.868201376384557300 ) ) ;
#7820=ORIENTED_EDGE ( 'NONE', *, *, #10086, .F. ) ;
#7821=FACE_OUTER_BOUND ( 'NONE', #52258, .T. ) ;
#7822=CARTESIAN_POINT ( 'NONE',  ( 35.00000000000000000, -6.475373545682373333, -10.32377448871666026 ) ) ;
#7823=EDGE_CURVE ( 'NONE', #11411, #32398, #22436, .T. ) ;
#7825=CARTESIAN_POINT ( 'NONE',  ( -18.56158150824929010, 4.674298569737585396, -11.05522311479379205 ) ) ;
#7826=VERTEX_POINT ( 'NONE', #51413 ) ;
#7829=ORIENTED_EDGE ( 'NONE', *, *, #49283, .F. ) ;
#7831=ORIENTED_EDGE ( 'NONE', *, *, #65454, .T. ) ;
#7833=EDGE_CURVE ( 'NONE', #28337, #45163, #61040, .T. ) ;
#7834=EDGE_LOOP ( 'NONE', ( #27011, #2207, #39484, #5504 ) ) ;
#7835=EDGE_CURVE ( 'NONE', #46122, #57170, #50420, .T. ) ;
#7838=CARTESIAN_POINT ( 'NONE',  ( 37.00000000000000711, 4.705694406421931860E-17, -3.469127814946512892E-15 ) ) ;
#7840=VECTOR ( 'NONE', #16493, 1000.000000000000000 ) ;
#7842=AXIS2_PLACEMENT_3D ( 'NONE', #58175, #57529, #42517 ) ;
#7843=ADVANCED_FACE ( 'NONE', ( #15473 ), #5184, .T. ) ;
#7844=CARTESIAN_POINT ( 'NONE',  ( 35.00000000000000000, 10.02106554660720050, 7.882940143791660859 ) ) ;
#7848=VERTEX_POINT ( 'NONE', #25132 ) ;
#7853=CARTESIAN_POINT ( 'NONE',  ( -24.85695914810692386, 10.87191068482259126, 8.004987175091917706 ) ) ;
#7855=AXIS2_PLACEMENT_3D ( 'NONE', #12389, #62944, #42989 ) ;
#7856=CARTESIAN_POINT ( 'NONE',  ( -35.00000000000000000, 7.499679039484183463, -9.040300684349618976 ) ) ;
#7857=CARTESIAN_POINT ( 'NONE',  ( 22.57855258442564761, -4.427776684447072952, 11.15324139578564910 ) ) ;
#7859=DIRECTION ( 'NONE',  ( 0.000000000000000000, 0.01356324068817998940, -0.9999080150203990547 ) ) ;
#7860=VERTEX_POINT ( 'NONE', #45401 ) ;
#7861=CARTESIAN_POINT ( 'NONE',  ( -25.77583339569473964, -10.55051720252683722, 5.718653903698916352 ) ) ;
#7864=VECTOR ( 'NONE', #55788, 1000.000000000000000 ) ;
#7867=VERTEX_POINT ( 'NONE', #41386 ) ;
#7868=DIRECTION ( 'NONE',  ( 1.000000000000000000, 0.000000000000000000, 0.000000000000000000 ) ) ;
#7871=CARTESIAN_POINT ( 'NONE',  ( 35.00000000000000000, 9.557269938331552694, -7.561043153948004303 ) ) ;
#7875=CIRCLE ( 'NONE', #39754, 12.75000000000000178 ) ;
#7877=ORIENTED_EDGE ( 'NONE', *, *, #46322, .F. ) ;
#7878=CARTESIAN_POINT ( 'NONE',  ( -37.00000000000000711, 9.321877890560440250, 7.146664589317944127 ) ) ;
#7879=ORIENTED_EDGE ( 'NONE', *, *, #29370, .T. ) ;
#7880=DIRECTION ( 'NONE',  ( 0.000000000000000000, 0.2355298848897446895, 0.9718671068226476528 ) ) ;
#7881=CIRCLE ( 'NONE', #47190, 5.000000000000000000 ) ;
#7882=FACE_OUTER_BOUND ( 'NONE', #48068, .T. ) ;
#7883=EDGE_CURVE ( 'NONE', #61480, #4911, #35141, .T. ) ;
#7887=EDGE_CURVE ( 'NONE', #10303, #36936, #22367, .T. ) ;
#7891=CARTESIAN_POINT ( 'NONE',  ( 8.633087204097703804, 5.803048762801607197, 10.50557656966853592 ) ) ;
#7895=VERTEX_POINT ( 'NONE', #62328 ) ;
#7896=AXIS2_PLACEMENT_3D ( 'NONE', #31724, #6819, #31091 ) ;
#7901=CIRCLE ( 'NONE', #45057, 12.18649999999999878 ) ;
#7903=DIRECTION ( 'NONE',  ( 1.000000000000000000, -0.000000000000000000, -0.000000000000000000 ) ) ;
#7904=ORIENTED_EDGE ( 'NONE', *, *, #43244, .T. ) ;
#7906=CARTESIAN_POINT ( 'NONE',  ( 29.64698554648902729, 8.428051259464909961, 10.58407887936916758 ) ) ;
#7907=VECTOR ( 'NONE', #29755, 1000.000000000000000 ) ;
#7910=VERTEX_POINT ( 'NONE', #12120 ) ;
#7911=CARTESIAN_POINT ( 'NONE',  ( -10.66655393549213393, -4.452669714455520733, -12.75039268524656855 ) ) ;
#7912=CYLINDRICAL_SURFACE ( 'NONE', #12923, 4.999999999999998224 ) ;
#7914=ADVANCED_FACE ( 'NONE', ( #33053 ), #7451, .T. ) ;
#7916=CYLINDRICAL_SURFACE ( 'NONE', #50910, 12.74999999999999822 ) ;
#7917=DIRECTION ( 'NONE',  ( 0.000000000000000000, -0.9999080150203992767, -0.01356324068816951341 ) ) ;
#7918=ADVANCED_FACE ( 'NONE', ( #7806 ), #1833, .T. ) ;
#7919=AXIS2_PLACEMENT_3D ( 'NONE', #18274, #58507, #38535 ) ;
#7922=EDGE_CURVE ( 'NONE', #19174, #35378, #38341, .T. ) ;
#7923=VERTEX_POINT ( 'NONE', #28090 ) ;
#7924=DIRECTION ( 'NONE',  ( -1.000000000000000000, 0.000000000000000000, -0.000000000000000000 ) ) ;
#7927=DIRECTION ( 'NONE',  ( 0.7932577242209934987, -0.6088860180392799970, 0.000000000000000000 ) ) ;
#7928=DIRECTION ( 'NONE',  ( 1.000000000000000000, 0.000000000000000000, 0.000000000000000000 ) ) ;
#7929=EDGE_CURVE ( 'NONE', #59672, #20489, #2835, .T. ) ;
#7931=DIRECTION ( 'NONE',  ( 0.000000000000000000, 0.01356324068817991828, -0.9999080150203990547 ) ) ;
#7932=ORIENTED_EDGE ( 'NONE', *, *, #38256, .T. ) ;
#7933=EDGE_LOOP ( 'NONE', ( #40029, #52833, #44939, #64283 ) ) ;
#7934=AXIS2_PLACEMENT_3D ( 'NONE', #40095, #44425, #19175 ) ;
#7940=CARTESIAN_POINT ( 'NONE',  ( -35.00000000000000000, 0.000000000000000000, 0.000000000000000000 ) ) ;
#7943=CIRCLE ( 'NONE', #16430, 12.18649999999999878 ) ;
#7946=ORIENTED_EDGE ( 'NONE', *, *, #27900, .T. ) ;
#7948=DIRECTION ( 'NONE',  ( -1.000000000000000000, -0.000000000000000000, 0.000000000000000000 ) ) ;
#7950=ORIENTED_EDGE ( 'NONE', *, *, #6322, .F. ) ;
#7951=DIRECTION ( 'NONE',  ( 1.000000000000000000, 0.000000000000000000, 0.000000000000000000 ) ) ;
#7952=EDGE_LOOP ( 'NONE', ( #60061, #32171, #46523, #40520 ) ) ;
#7954=CARTESIAN_POINT ( 'NONE',  ( -19.69476066079020171, -4.201994156881551312, -11.24025111398909615 ) ) ;
#7955=AXIS2_PLACEMENT_3D ( 'NONE', #40795, #36452, #26465 ) ;
#7957=EDGE_CURVE ( 'NONE', #24707, #9063, #26768, .T. ) ;
#7958=DIRECTION ( 'NONE',  ( 0.000000000000000000, 0.2006870767258820687, -0.9796553971857756560 ) ) ;
#7959=CYLINDRICAL_SURFACE ( 'NONE', #1221, 12.75000000000000178 ) ;
#7960=CARTESIAN_POINT ( 'NONE',  ( 37.00000000000000711, 2.220215194442072271, 11.98254675519225287 ) ) ;
#7961=CARTESIAN_POINT ( 'NONE',  ( -35.00000000000000000, -5.273331777780412288, 10.49591321039678959 ) ) ;
#7962=ADVANCED_FACE ( 'NONE', ( #11784 ), #52706, .T. ) ;
#7970=CARTESIAN_POINT ( 'NONE',  ( 35.00000000000000000, 11.42599468261429152, -4.237620530777845396 ) ) ;
#7972=EDGE_CURVE ( 'NONE', #40710, #46217, #38651, .T. ) ;
#7973=CARTESIAN_POINT ( 'NONE',  ( -4.975205859172452172, -1.416020129149132778, 11.91616074890920451 ) ) ;
#7974=AXIS2_PLACEMENT_3D ( 'NONE', #449, #61273, #31013 ) ;
#7977=( BOUNDED_CURVE ( )  B_SPLINE_CURVE ( 3, ( #39791, #9507, #60393, #54105 ),
 .UNSPECIFIED., .F., .F. ) 
 B_SPLINE_CURVE_WITH_KNOTS ( ( 4, 4 ),
 ( 3.954312062358600333, 4.006764403430960186 ),
 .UNSPECIFIED. ) 
 CURVE ( )  GEOMETRIC_REPRESENTATION_ITEM ( )  RATIONAL_B_SPLINE_CURVE ( ( 1.000000000000000000, 0.9997707424672948040, 0.9997707424672948040, 1.000000000000000000 ) ) 
 REPRESENTATION_ITEM ( '' )  );
#7978=VERTEX_POINT ( 'NONE', #32706 ) ;
#7979=CARTESIAN_POINT ( 'NONE',  ( 35.00000000000000000, -9.217970097227778936, -7.971186206369441862 ) ) ;
#7981=DIRECTION ( 'NONE',  ( 1.000000000000000000, 0.000000000000000000, -0.000000000000000000 ) ) ;
#7986=( GEOMETRIC_REPRESENTATION_CONTEXT ( 3 ) GLOBAL_UNCERTAINTY_ASSIGNED_CONTEXT ( ( #27676 ) ) GLOBAL_UNIT_ASSIGNED_CONTEXT ( ( #5383, #15005, #21587 ) ) REPRESENTATION_CONTEXT ( 'NONE', 'WORKASPACE' ) );
#7989=DIRECTION ( 'NONE',  ( 0.000000000000000000, 0.01356324068817991828, -0.9999080150203990547 ) ) ;
#7991=EDGE_CURVE ( 'NONE', #6431, #29014, #8633, .T. ) ;
#7993=AXIS2_PLACEMENT_3D ( 'NONE', #43199, #12951, #57539 ) ;
#7994=ORIENTED_EDGE ( 'NONE', *, *, #13774, .F. ) ;
#8000=CIRCLE ( 'NONE', #45146, 12.18650000000000055 ) ;
#8002=ORIENTED_EDGE ( 'NONE', *, *, #39502, .T. ) ;
#8004=EDGE_CURVE ( 'NONE', #22247, #14897, #46186, .T. ) ;
#8005=ORIENTED_EDGE ( 'NONE', *, *, #222, .F. ) ;
#8007=CARTESIAN_POINT ( 'NONE',  ( 35.00000000000000000, 4.705694406421931860E-17, -3.469127814946512892E-15 ) ) ;
#8009=CARTESIAN_POINT ( 'NONE',  ( 35.00000000000000000, 10.70999494708492250, -5.814360711498331113 ) ) ;
#8011=DIRECTION ( 'NONE',  ( -0.000000000000000000, -1.000000000000000000, -0.000000000000000000 ) ) ;
#8012=ORIENTED_EDGE ( 'NONE', *, *, #49946, .F. ) ;
#8013=VERTEX_POINT ( 'NONE', #34035 ) ;
#8018=EDGE_CURVE ( 'NONE', #11746, #52324, #29071, .T. ) ;
#8019=CARTESIAN_POINT ( 'NONE',  ( -37.00000000000000711, 0.000000000000000000, 0.000000000000000000 ) ) ;
#8021=ORIENTED_EDGE ( 'NONE', *, *, #22340, .F. ) ;
#8023=CARTESIAN_POINT ( 'NONE',  ( 37.00000000000000711, 4.705694406421931860E-17, -3.469127814946512892E-15 ) ) ;
#8025=ORIENTED_EDGE ( 'NONE', *, *, #23571, .F. ) ;
#8026=EDGE_LOOP ( 'NONE', ( #48919, #39897, #52413, #11999 ) ) ;
#8027=DIRECTION ( 'NONE',  ( 1.000000000000000000, 0.000000000000000000, -0.000000000000000000 ) ) ;
#8028=VERTEX_POINT ( 'NONE', #29694 ) ;
#8029=VERTEX_POINT ( 'NONE', #8451 ) ;
#8032=DIRECTION ( 'NONE',  ( -1.000000000000000000, 0.000000000000000000, 0.000000000000000000 ) ) ;
#8033=DIRECTION ( 'NONE',  ( 0.000000000000000000, 0.2355298848897447728, 0.9718671068226475418 ) ) ;
#8034=PLANE ( 'NONE',  #39360 ) ;
#8036=CARTESIAN_POINT ( 'NONE',  ( -27.75684343571922952, -10.82790328082247377, -5.180978323404352714 ) ) ;
#8037=ORIENTED_EDGE ( 'NONE', *, *, #44065, .T. ) ;
#8039=EDGE_CURVE ( 'NONE', #62061, #38335, #34373, .T. ) ;
#8040=AXIS2_PLACEMENT_3D ( 'NONE', #12605, #42528, #22949 ) ;
#8043=CARTESIAN_POINT ( 'NONE',  ( 37.00000000000000711, 4.705694406421931860E-17, -3.469127814946512892E-15 ) ) ;
#8044=ORIENTED_EDGE ( 'NONE', *, *, #46405, .T. ) ;
#8045=CARTESIAN_POINT ( 'NONE',  ( -19.47984447937493613, -3.750539801530005768, 12.96855624952674724 ) ) ;
#8048=ORIENTED_EDGE ( 'NONE', *, *, #35872, .T. ) ;
#8049=ORIENTED_EDGE ( 'NONE', *, *, #31011, .F. ) ;
#8051=ORIENTED_EDGE ( 'NONE', *, *, #35056, .F. ) ;
#8052=DIRECTION ( 'NONE',  ( 1.000000000000000000, -0.000000000000000000, 0.000000000000000000 ) ) ;
#8053=CARTESIAN_POINT ( 'NONE',  ( -3.761952589723977169, -7.433916943621393436, 9.430559907043596368 ) ) ;
#8054=LINE ( 'NONE', #28982, #62159 ) ;
#8055=CARTESIAN_POINT ( 'NONE',  ( -2.747965937637946165, 11.18537856137285580, 4.360398752428172209 ) ) ;
#8059=CYLINDRICAL_SURFACE ( 'NONE', #18919, 4.999999999999999112 ) ;
#8060=EDGE_CURVE ( 'NONE', #1336, #7532, #6487, .T. ) ;
#8061=AXIS2_PLACEMENT_3D ( 'NONE', #28562, #2680, #23593 ) ;
#8065=CARTESIAN_POINT ( 'NONE',  ( 7.313837862481380014, -6.193139553693423949, -10.28892890405838223 ) ) ;
#8067=EDGE_CURVE ( 'NONE', #17999, #52684, #64913, .T. ) ;
#8072=DIRECTION ( 'NONE',  ( -1.000000000000000000, 0.000000000000000000, 0.000000000000000000 ) ) ;
#8073=CARTESIAN_POINT ( 'NONE',  ( 35.00000000000000000, 4.705694406421931860E-17, -3.469127814946512892E-15 ) ) ;
#8074=CARTESIAN_POINT ( 'NONE',  ( 36.00000000000000711, 6.950793414699941053, 10.68873102412834797 ) ) ;
#8078=VERTEX_POINT ( 'NONE', #55966 ) ;
#8083=EDGE_CURVE ( 'NONE', #12489, #62829, #35343, .T. ) ;
#8085=VERTEX_POINT ( 'NONE', #55653 ) ;
#8086=CARTESIAN_POINT ( 'NONE',  ( -47.00000000000000711, 0.000000000000000000, 0.000000000000000000 ) ) ;
#8088=DIRECTION ( 'NONE',  ( -0.000000000000000000, -0.000000000000000000, -1.000000000000000000 ) ) ;
#8089=CARTESIAN_POINT ( 'NONE',  ( 18.12752167935788705, 7.578978283205488609, 9.315231351494983159 ) ) ;
#8090=VERTEX_POINT ( 'NONE', #10399 ) ;
#8095=ORIENTED_EDGE ( 'NONE', *, *, #47562, .T. ) ;
#8098=CARTESIAN_POINT ( 'NONE',  ( -18.10219876433327357, 13.45940644062556757, 1.101009084313006037 ) ) ;
#8099=ORIENTED_EDGE ( 'NONE', *, *, #9999, .T. ) ;
#8100=DIRECTION ( 'NONE',  ( 0.000000000000000000, -0.01356324068817998940, 0.9999080150203990547 ) ) ;
#8102=CYLINDRICAL_SURFACE ( 'NONE', #32956, 12.74999999999999822 ) ;
#8105=CARTESIAN_POINT ( 'NONE',  ( -4.975205859172449507, -1.416020129149132778, -13.42553116244733680 ) ) ;
#8107=ADVANCED_FACE ( 'NONE', ( #19752 ), #5445, .T. ) ;
#8108=ORIENTED_EDGE ( 'NONE', *, *, #11374, .T. ) ;
#8111=EDGE_CURVE ( 'NONE', #35473, #17729, #51331, .T. ) ;
#8112=ORIENTED_EDGE ( 'NONE', *, *, #152, .F. ) ;
#8115=CARTESIAN_POINT ( 'NONE',  ( 37.00000000000000711, 4.705694406421931860E-17, -3.469127814946512892E-15 ) ) ;
#8119=DIRECTION ( 'NONE',  ( 0.000000000000000000, 0.5767582926624970074, 0.8169148498130275327 ) ) ;
#8120=EDGE_CURVE ( 'NONE', #13346, #17960, #29833, .T. ) ;
#8121=AXIS2_PLACEMENT_3D ( 'NONE', #27688, #20334, #15353 ) ;
#8124=ORIENTED_EDGE ( 'NONE', *, *, #35210, .F. ) ;
#8126=LINE ( 'NONE', #45647, #36664 ) ;
#8127=CARTESIAN_POINT ( 'NONE',  ( 6.661406098020970390, -4.211117136771884262, -11.23710102852283299 ) ) ;
#8128=ADVANCED_FACE ( 'NONE', ( #52311 ), #62569, .T. ) ;
#8130=CARTESIAN_POINT ( 'NONE',  ( 36.00000000000000711, 8.235637554476776145, 9.733281772932070197 ) ) ;
#8131=CARTESIAN_POINT ( 'NONE',  ( 37.00000000000000711, 1.908798535168559241, 12.60630747491660486 ) ) ;
#8132=CARTESIAN_POINT ( 'NONE',  ( -10.66677318034315292, -4.454008058369508305, 12.74975837362279485 ) ) ;
#8133=CARTESIAN_POINT ( 'NONE',  ( 35.00000000000000000, 9.348667969174517367, 7.817492529713752525 ) ) ;
#8134=ORIENTED_EDGE ( 'NONE', *, *, #18077, .T. ) ;
#8136=CARTESIAN_POINT ( 'NONE',  ( 47.00000000000000711, 4.705694406421931860E-17, -3.469127814946512892E-15 ) ) ;
#8137=DIRECTION ( 'NONE',  ( -1.000000000000000000, 0.000000000000000000, 0.000000000000000000 ) ) ;
#8138=DIRECTION ( 'NONE',  ( 1.000000000000000000, 0.000000000000000000, 0.000000000000000000 ) ) ;
#8140=CARTESIAN_POINT ( 'NONE',  ( -18.08686583997219088, 4.946258258172888667, 12.56318811865292062 ) ) ;
#8143=ORIENTED_EDGE ( 'NONE', *, *, #29896, .F. ) ;
#8144=DIRECTION ( 'NONE',  ( 1.000000000000000000, 0.000000000000000000, 0.000000000000000000 ) ) ;
#8145=FACE_OUTER_BOUND ( 'NONE', #43577, .T. ) ;
#8146=EDGE_LOOP ( 'NONE', ( #22031, #35231, #55530, #35135 ) ) ;
#8148=DIRECTION ( 'NONE',  ( -1.000000000000000000, -0.000000000000000000, 0.000000000000000000 ) ) ;
#8151=ORIENTED_EDGE ( 'NONE', *, *, #54972, .F. ) ;
#8153=CARTESIAN_POINT ( 'NONE',  ( 35.00000000000000000, -6.584150480049477672, 10.25474254703959431 ) ) ;
#8154=CARTESIAN_POINT ( 'NONE',  ( 37.00000000000000711, -11.90598845858536947, -4.561791185930372805 ) ) ;
#8156=( BOUNDED_CURVE ( )  B_SPLINE_CURVE ( 3, ( #14675, #48997, #34958, #13709 ),
 .UNSPECIFIED., .F., .F. ) 
 B_SPLINE_CURVE_WITH_KNOTS ( ( 4, 4 ),
 ( 3.922071288503527153, 3.961819178845479517 ),
 .UNSPECIFIED. ) 
 CURVE ( )  GEOMETRIC_REPRESENTATION_ITEM ( )  RATIONAL_B_SPLINE_CURVE ( ( 1.000000000000000000, 0.9998683464345071714, 0.9998683464345071714, 1.000000000000000000 ) ) 
 REPRESENTATION_ITEM ( '' )  );
#8163=CARTESIAN_POINT ( 'NONE',  ( -47.00000000000000711, 0.000000000000000000, 0.000000000000000000 ) ) ;
#8164=EDGE_LOOP ( 'NONE', ( #431, #50830, #25766, #51922 ) ) ;
#8165=ORIENTED_EDGE ( 'NONE', *, *, #57289, .F. ) ;
#8166=CARTESIAN_POINT ( 'NONE',  ( -24.85993732546052470, 9.902695843592100644, 9.181557340668950573 ) ) ;
#8168=CARTESIAN_POINT ( 'NONE',  ( -2.952869152607111136, 4.384817011589738911, 11.17020052527586138 ) ) ;
#8172=DIRECTION ( 'NONE',  ( 1.000000000000000000, 0.000000000000000000, 0.000000000000000000 ) ) ;
#8173=ORIENTED_EDGE ( 'NONE', *, *, #42942, .T. ) ;
#8174=DIRECTION ( 'NONE',  ( -1.000000000000000000, 0.000000000000000000, 0.000000000000000000 ) ) ;
#8175=EDGE_CURVE ( 'NONE', #46293, #56608, #60650, .T. ) ;
#8177=DIRECTION ( 'NONE',  ( 1.000000000000000000, 0.000000000000000000, 0.000000000000000000 ) ) ;
#8178=ORIENTED_EDGE ( 'NONE', *, *, #33995, .T. ) ;
#8180=EDGE_CURVE ( 'NONE', #9450, #19224, #22023, .T. ) ;
#8181=ORIENTED_EDGE ( 'NONE', *, *, #51948, .F. ) ;
#8185=DIRECTION ( 'NONE',  ( 0.000000000000000000, -0.5767582926624851281, -0.8169148498130358593 ) ) ;
#8187=LINE ( 'NONE', #2893, #3076 ) ;
#8188=ADVANCED_FACE ( 'NONE', ( #1440 ), #47318, .T. ) ;
#8189=B_SPLINE_CURVE_WITH_KNOTS ( 'NONE', 3,
 ( #36739, #6485, #41721, #33309, #8053, #57353, #48946, #57032, #21793, #58939, #26761, #52040, #59245, #47059, #1516, #42041, #2757, #62325 ),
 .UNSPECIFIED., .F., .F.,
 ( 4, 2, 2, 2, 2, 2, 2, 2, 4 ),
 ( 9.697399036122160616E-19, 0.002700019232399850349, 0.004050028848599774439, 0.005400038464799701565, 0.006075043272899665996, 0.006750048080999626089, 0.008100057697199548878, 0.009450067313399469066, 0.01080007692959938925 ),
 .UNSPECIFIED. ) ;
#8190=CARTESIAN_POINT ( 'NONE',  ( 36.00000000000000711, 11.96656215839374937, 4.400442035670817376 ) ) ;
#8191=VERTEX_POINT ( 'NONE', #12363 ) ;
#8193=CIRCLE ( 'NONE', #38987, 5.000000000000000000 ) ;
#8195=ORIENTED_EDGE ( 'NONE', *, *, #52209, .T. ) ;
#8197=FACE_OUTER_BOUND ( 'NONE', #8914, .T. ) ;
#8198=AXIS2_PLACEMENT_3D ( 'NONE', #29508, #38519, #38855 ) ;
#8200=LINE ( 'NONE', #44401, #23842 ) ;
#8201=CARTESIAN_POINT ( 'NONE',  ( -27.94768133936596399, 13.15239037730114369, -3.102958909511970731 ) ) ;
#8202=AXIS2_PLACEMENT_3D ( 'NONE', #11747, #32364, #56329 ) ;
#8203=ADVANCED_FACE ( 'NONE', ( #42610 ), #62256, .T. ) ;
#8204=VERTEX_POINT ( 'NONE', #12045 ) ;
#8206=LINE ( 'NONE', #28473, #53586 ) ;
#8207=ADVANCED_FACE ( 'NONE', ( #62913 ), #41648, .T. ) ;
#8209=CARTESIAN_POINT ( 'NONE',  ( 37.00000000000000711, 4.705694406421931860E-17, -3.469127814946512892E-15 ) ) ;
#8210=ORIENTED_EDGE ( 'NONE', *, *, #43768, .F. ) ;
#8216=CARTESIAN_POINT ( 'NONE',  ( -27.95869044047065799, -11.60004630023460948, -3.134771106759090653 ) ) ;
#8219=FACE_OUTER_BOUND ( 'NONE', #51325, .T. ) ;
#8221=EDGE_LOOP ( 'NONE', ( #62924, #23988, #55913, #25592 ) ) ;
#8223=DIRECTION ( 'NONE',  ( 1.000000000000000000, 0.000000000000000000, 0.000000000000000000 ) ) ;
#8224=CYLINDRICAL_SURFACE ( 'NONE', #5386, 2.809571291727933851 ) ;
#8225=CYLINDRICAL_SURFACE ( 'NONE', #57268, 5.000000000000000888 ) ;
#8227=B_SPLINE_CURVE_WITH_KNOTS ( 'NONE', 3,
 ( #57154, #36182, #56488, #50532, #316, #16588 ),
 .UNSPECIFIED., .F., .F.,
 ( 4, 2, 4 ),
 ( 1.124229303124644401E-17, 0.001589257412050233947, 0.003178514824100456618 ),
 .UNSPECIFIED. ) ;
#8228=CIRCLE ( 'NONE', #5056, 4.999999999999999112 ) ;
#8229=EDGE_CURVE ( 'NONE', #46663, #14288, #49010, .T. ) ;
#8230=LINE ( 'NONE', #64395, #55218 ) ;
#8231=ORIENTED_EDGE ( 'NONE', *, *, #62800, .T. ) ;
#8233=CARTESIAN_POINT ( 'NONE',  ( 37.00000000000000711, 10.14408668126221613, 5.921969905510239940 ) ) ;
#8236=LINE ( 'NONE', #3610, #24813 ) ;
#8237=DIRECTION ( 'NONE',  ( 1.000000000000000000, 0.000000000000000000, 0.000000000000000000 ) ) ;
#8240=ORIENTED_EDGE ( 'NONE', *, *, #25913, .T. ) ;
#8242=EDGE_CURVE ( 'NONE', #7848, #30956, #47948, .T. ) ;
#8243=CARTESIAN_POINT ( 'NONE',  ( -19.04306142112764633, -4.598438116554168786, -11.08446069010050827 ) ) ;
#8244=VERTEX_POINT ( 'NONE', #27657 ) ;
#8245=VECTOR ( 'NONE', #29436, 1000.000000000000000 ) ;
#8246=DIRECTION ( 'NONE',  ( 0.000000000000000000, 0.01356324068818000328, -0.9999080150203990547 ) ) ;
#8247=CARTESIAN_POINT ( 'NONE',  ( -36.00000000000000711, 11.24036214326520700, 6.018036132182203346 ) ) ;
#8248=EDGE_CURVE ( 'NONE', #40729, #41862, #51179, .T. ) ;
#8250=EDGE_LOOP ( 'NONE', ( #63592, #15052, #49710, #39008 ) ) ;
#8253=DIRECTION ( 'NONE',  ( -1.000000000000000000, -0.000000000000000000, 0.000000000000000000 ) ) ;
#8255=ORIENTED_EDGE ( 'NONE', *, *, #22119, .F. ) ;
#8256=DIRECTION ( 'NONE',  ( 0.000000000000000000, -0.7617968321374811724, -0.6478160128812026075 ) ) ;
#8257=EDGE_CURVE ( 'NONE', #46698, #22470, #51973, .T. ) ;
#8258=EDGE_LOOP ( 'NONE', ( #49847, #494, #17576, #44556 ) ) ;
#8260=VERTEX_POINT ( 'NONE', #991 ) ;
#8261=ORIENTED_EDGE ( 'NONE', *, *, #49689, .T. ) ;
#8264=DIRECTION ( 'NONE',  ( 1.000000000000000000, 0.000000000000000000, -0.000000000000000000 ) ) ;
#8265=DIRECTION ( 'NONE',  ( 0.000000000000000000, -0.01356324068817998940, 0.9999080150203990547 ) ) ;
#8269=CARTESIAN_POINT ( 'NONE',  ( -36.00000000000000711, 3.473736367725253960, 12.26766708251992988 ) ) ;
#8271=CARTESIAN_POINT ( 'NONE',  ( -15.83651567491729395, 7.907244717092745567, 9.026412348056238599 ) ) ;
#8272=CARTESIAN_POINT ( 'NONE',  ( -37.00000000000000711, -4.074242145635923684, -12.08151691381194581 ) ) ;
#8273=EDGE_CURVE ( 'NONE', #28113, #11187, #59663, .T. ) ;
#8277=CARTESIAN_POINT ( 'NONE',  ( -37.00000000000000711, -7.745827850122939395, -10.12742074351904975 ) ) ;
#8278=CARTESIAN_POINT ( 'NONE',  ( -36.00000000000000711, 9.621072037177118119, -8.366449238204259231 ) ) ;
#8279=CARTESIAN_POINT ( 'NONE',  ( -35.00000000000000000, 6.102719229070827645, -10.54834585426213422 ) ) ;
#8281=AXIS2_PLACEMENT_3D ( 'NONE', #16107, #25429, #55362 ) ;
#8282=ORIENTED_EDGE ( 'NONE', *, *, #1904, .F. ) ;
#8284=EDGE_CURVE ( 'NONE', #50289, #3042, #47991, .T. ) ;
#8286=AXIS2_PLACEMENT_3D ( 'NONE', #57771, #12188, #38106 ) ;
#8287=ORIENTED_EDGE ( 'NONE', *, *, #37699, .T. ) ;
#8288=CARTESIAN_POINT ( 'NONE',  ( -17.29244623348158783, 2.525873743887551814, 11.73115347397430597 ) ) ;
#8289=DIRECTION ( 'NONE',  ( 1.000000000000000000, 0.000000000000000000, -0.000000000000000000 ) ) ;
#8290=CARTESIAN_POINT ( 'NONE',  ( 12.82394711127995812, -12.76747887865895592, -4.390754480898809042 ) ) ;
#8295=ORIENTED_EDGE ( 'NONE', *, *, #47616, .F. ) ;
#8299=VECTOR ( 'NONE', #53347, 1000.000000000000000 ) ;
#8301=FACE_OUTER_BOUND ( 'NONE', #12643, .T. ) ;
#8302=ORIENTED_EDGE ( 'NONE', *, *, #39948, .T. ) ;
#8303=CARTESIAN_POINT ( 'NONE',  ( -35.00000000000000000, 9.063649021439076137, -8.146229107149299153 ) ) ;
#8306=ADVANCED_FACE ( 'NONE', ( #46229 ), #51222, .T. ) ;
#8309=CARTESIAN_POINT ( 'NONE',  ( -9.656847648909668180, 11.20398564923865514, -7.540956407560663877 ) ) ;
#8311=DIRECTION ( 'NONE',  ( 0.000000000000000000, 0.01356324068817991828, -0.9999080150203990547 ) ) ;
#8314=VECTOR ( 'NONE', #58752, 1000.000000000000000 ) ;
#8317=EDGE_LOOP ( 'NONE', ( #26160, #54050, #46617, #4666 ) ) ;
#8319=ORIENTED_EDGE ( 'NONE', *, *, #39280, .T. ) ;
#8320=ORIENTED_EDGE ( 'NONE', *, *, #43153, .T. ) ;
#8322=FACE_OUTER_BOUND ( 'NONE', #43467, .T. ) ;
#8324=DIRECTION ( 'NONE',  ( 1.000000000000000000, 0.000000000000000000, -0.000000000000000000 ) ) ;
#8331=VERTEX_POINT ( 'NONE', #9985 ) ;
#8335=EDGE_CURVE ( 'NONE', #311, #59495, #6559, .T. ) ;
#8336=VERTEX_POINT ( 'NONE', #16283 ) ;
#8337=CARTESIAN_POINT ( 'NONE',  ( -19.88622662114644513, 11.70525051340494116, -2.725500476031548658 ) ) ;
#8338=ORIENTED_EDGE ( 'NONE', *, *, #9405, .T. ) ;
#8339=VECTOR ( 'NONE', #48851, 1000.000000000000000 ) ;
#8344=CARTESIAN_POINT ( 'NONE',  ( -47.00000000000000711, 0.000000000000000000, 0.000000000000000000 ) ) ;
#8346=ORIENTED_EDGE ( 'NONE', *, *, #60729, .F. ) ;
#8349=ORIENTED_EDGE ( 'NONE', *, *, #27664, .T. ) ;
#8351=CARTESIAN_POINT ( 'NONE',  ( -17.85139933901853482, -6.218234000768075198, -11.98572918122005326 ) ) ;
#8352=ORIENTED_EDGE ( 'NONE', *, *, #51041, .F. ) ;
#8353=CARTESIAN_POINT ( 'NONE',  ( -35.00000000000000000, -3.916263239775430005, 11.07407352312211302 ) ) ;
#8358=AXIS2_PLACEMENT_3D ( 'NONE', #21630, #7289, #6665 ) ;
#8361=EDGE_CURVE ( 'NONE', #53066, #56700, #16613, .T. ) ;
#8362=AXIS2_PLACEMENT_3D ( 'NONE', #65649, #50718, #61020 ) ;
#8363=ORIENTED_EDGE ( 'NONE', *, *, #35824, .T. ) ;
#8366=ADVANCED_FACE ( 'NONE', ( #53166, #27555 ), #32528, .F. ) ;
#8367=FACE_OUTER_BOUND ( 'NONE', #5121, .T. ) ;
#8368=DIRECTION ( 'NONE',  ( -1.000000000000000000, 0.000000000000000000, 0.000000000000000000 ) ) ;
#8371=VECTOR ( 'NONE', #60159, 1000.000000000000000 ) ;
#8374=CIRCLE ( 'NONE', #15655, 12.18650000000000055 ) ;
#8376=CARTESIAN_POINT ( 'NONE',  ( 23.64999694718868994, 11.46135651385800180, -7.139647639458894801 ) ) ;
#8379=CARTESIAN_POINT ( 'NONE',  ( 35.00000000000000000, -2.968224442958486975, -11.81949347079746282 ) ) ;
#8380=CARTESIAN_POINT ( 'NONE',  ( 4.199947675780304479, -10.87007255795022687, -5.085750118326637370 ) ) ;
#8382=CIRCLE ( 'NONE', #16875, 12.75000000000000178 ) ;
#8383=EDGE_CURVE ( 'NONE', #21953, #40162, #45849, .T. ) ;
#8384=ORIENTED_EDGE ( 'NONE', *, *, #54436, .F. ) ;
#8385=CARTESIAN_POINT ( 'NONE',  ( 12.29300949244506924, -11.61203561930438255, -3.031982959488972451 ) ) ;
#8387=ORIENTED_EDGE ( 'NONE', *, *, #8556, .F. ) ;
#8390=DIRECTION ( 'NONE',  ( -0.000000000000000000, -1.000000000000000000, -0.000000000000000000 ) ) ;
#8392=EDGE_CURVE ( 'NONE', #3042, #53140, #30984, .T. ) ;
#8393=ORIENTED_EDGE ( 'NONE', *, *, #34457, .F. ) ;
#8395=CARTESIAN_POINT ( 'NONE',  ( 35.00000000000000000, 11.10408318471059275, -6.265926637539534383 ) ) ;
#8397=AXIS2_PLACEMENT_3D ( 'NONE', #369, #6335, #5696 ) ;
#8398=EDGE_LOOP ( 'NONE', ( #237, #42494, #6518, #15555 ) ) ;
#8400=DIRECTION ( 'NONE',  ( 0.000000000000000000, -1.000000000000000000, 0.000000000000000000 ) ) ;
#8403=ORIENTED_EDGE ( 'NONE', *, *, #9586, .F. ) ;
#8408=CARTESIAN_POINT ( 'NONE',  ( -47.00000000000000711, 0.000000000000000000, 0.000000000000000000 ) ) ;
#8409=ORIENTED_EDGE ( 'NONE', *, *, #56311, .T. ) ;
#8412=ADVANCED_FACE ( 'NONE', ( #1972 ), #31878, .T. ) ;
#8414=CARTESIAN_POINT ( 'NONE',  ( -18.32962124502519075, 13.49796943741737998, 0.4155283434849697533 ) ) ;
#8415=VERTEX_POINT ( 'NONE', #33203 ) ;
#8417=VECTOR ( 'NONE', #33803, 1000.000000000000000 ) ;
#8419=EDGE_CURVE ( 'NONE', #31240, #46276, #7646, .T. ) ;
#8420=AXIS2_PLACEMENT_3D ( 'NONE', #62045, #25815, #65689 ) ;
#8421=CARTESIAN_POINT ( 'NONE',  ( -35.00000000000000000, -12.38385022362079724, -3.033604067594711129 ) ) ;
#8422=CARTESIAN_POINT ( 'NONE',  ( 35.00000000000000000, 11.72195762423409704, 0.7536123767498881243 ) ) ;
#8424=CARTESIAN_POINT ( 'NONE',  ( -8.564638015981364205, -2.705928108065259963, -13.22659762878139489 ) ) ;
#8426=AXIS2_PLACEMENT_3D ( 'NONE', #60144, #33578, #54184 ) ;
#8429=ORIENTED_EDGE ( 'NONE', *, *, #36728, .F. ) ;
#8433=AXIS2_PLACEMENT_3D ( 'NONE', #28602, #47917, #17332 ) ;
#8434=CYLINDRICAL_SURFACE ( 'NONE', #44550, 12.18649999999999878 ) ;
#8438=DIRECTION ( 'NONE',  ( 0.000000000000000000, -0.01356324068817991828, 0.9999080150203990547 ) ) ;
#8439=DIRECTION ( 'NONE',  ( 0.000000000000000000, -0.01356324068817998940, 0.9999080150203990547 ) ) ;
#8440=ADVANCED_FACE ( 'NONE', ( #17268 ), #37545, .T. ) ;
#8441=ORIENTED_EDGE ( 'NONE', *, *, #44678, .T. ) ;
#8445=B_SPLINE_CURVE_WITH_KNOTS ( 'NONE', 3,
 ( #40307, #25686, #45978, #39667, #24708, #30351, #50965, #46307, #30995, #54957, #60273, #60602, #29670, #15684, #14387, #15039, #49977, #4779, #44986, #39989, #14695, #9725, #30014, #432, #40978, #50325 ),
 .UNSPECIFIED., .F., .F.,
 ( 4, 2, 2, 2, 2, 2, 2, 2, 2, 2, 2, 2, 4 ),
 ( 0.000000000000000000, 0.001329167301762024245, 0.001993750952643036367, 0.002658334603524048489, 0.003322918254405061913, 0.003987501905286075336, 0.004652085556167088326, 0.005316669207048102183, 0.005981252857929116040, 0.006645836508810130765, 0.007975003810572164550, 0.009304171112334199203, 0.01063333841409623212 ),
 .UNSPECIFIED. ) ;
#8446=CYLINDRICAL_SURFACE ( 'NONE', #44093, 4.999999999999999112 ) ;
#8447=DIRECTION ( 'NONE',  ( 0.000000000000000000, 0.01356324068817998940, -0.9999080150203990547 ) ) ;
#8448=AXIS2_PLACEMENT_3D ( 'NONE', #59484, #19253, #44188 ) ;
#8449=EDGE_CURVE ( 'NONE', #21988, #62960, #64409, .T. ) ;
#8450=CIRCLE ( 'NONE', #32714, 12.75000000000000178 ) ;
#8451=CARTESIAN_POINT ( 'NONE',  ( 37.00000000000000711, 10.84030624090615724, 6.711949091238026632 ) ) ;
#8452=CARTESIAN_POINT ( 'NONE',  ( 10.87910344070132140, 1.037424946074062992, -11.95562161342227192 ) ) ;
#8457=CARTESIAN_POINT ( 'NONE',  ( -37.00000000000000711, 8.235637554476644695, 9.733281772932190989 ) ) ;
#8458=DIRECTION ( 'NONE',  ( -1.000000000000000000, 0.000000000000000000, -0.000000000000000000 ) ) ;
#8459=VECTOR ( 'NONE', #18783, 1000.000000000000000 ) ;
#8460=ADVANCED_FACE ( 'NONE', ( #22918 ), #21928, .F. ) ;
#8464=LINE ( 'NONE', #33726, #44567 ) ;
#8468=ORIENTED_EDGE ( 'NONE', *, *, #884, .T. ) ;
#8470=CYLINDRICAL_SURFACE ( 'NONE', #50180, 5.000000000000000888 ) ;
#8471=ADVANCED_FACE ( 'NONE', ( #11933 ), #50719, .T. ) ;
#8475=CYLINDRICAL_SURFACE ( 'NONE', #65177, 12.18649999999999878 ) ;
#8477=DIRECTION ( 'NONE',  ( 0.000000000000000000, -0.4698238015817236546, -0.8827602140260383257 ) ) ;
#8479=ORIENTED_EDGE ( 'NONE', *, *, #17635, .T. ) ;
#8480=DIRECTION ( 'NONE',  ( 0.000000000000000000, -0.01356324068817998940, 0.9999080150203990547 ) ) ;
#8481=ORIENTED_EDGE ( 'NONE', *, *, #25043, .T. ) ;
#8482=DIRECTION ( 'NONE',  ( -1.000000000000000000, 0.000000000000000000, 0.000000000000000000 ) ) ;
#8483=ORIENTED_EDGE ( 'NONE', *, *, #64611, .F. ) ;
#8484=ORIENTED_EDGE ( 'NONE', *, *, #49874, .F. ) ;
#8485=CARTESIAN_POINT ( 'NONE',  ( -27.10931547487525251, 12.25599567157371439, 5.660530150648361847 ) ) ;
#8487=CARTESIAN_POINT ( 'NONE',  ( -4.033318401586639013, 9.047516634271627112, 7.886307366337261371 ) ) ;
#8489=CARTESIAN_POINT ( 'NONE',  ( 3.347841273039249721, -10.61118957148187825, -5.603807266321158664 ) ) ;
#8491=VERTEX_POINT ( 'NONE', #8583 ) ;
#8493=VERTEX_POINT ( 'NONE', #13260 ) ;
#8495=DIRECTION ( 'NONE',  ( 1.000000000000000000, -0.000000000000000000, 0.000000000000000000 ) ) ;
#8496=DIRECTION ( 'NONE',  ( 0.000000000000000000, 0.01356324068817998940, -0.9999080150203989437 ) ) ;
#8506=FACE_OUTER_BOUND ( 'NONE', #41069, .T. ) ;
#8509=DIRECTION ( 'NONE',  ( 0.000000000000000000, -0.1118654143051476951, -0.9937233664769775654 ) ) ;
#8510=DIRECTION ( 'NONE',  ( 0.000000000000000000, 0.6943713148249639477, -0.7196168960969794304 ) ) ;
#8511=CIRCLE ( 'NONE', #12773, 12.74999999999999822 ) ;
#8513=EDGE_CURVE ( 'NONE', #47206, #26332, #21451, .T. ) ;
#8514=CARTESIAN_POINT ( 'NONE',  ( 35.00000000000000000, -11.61976888909157246, -3.827969819614423841 ) ) ;
#8517=CARTESIAN_POINT ( 'NONE',  ( 3.459614771489464946, -11.09853614738469396, -7.685863346768205595 ) ) ;
#8518=CARTESIAN_POINT ( 'NONE',  ( 37.00000000000000711, -11.10408318471055011, 6.265926637539605437 ) ) ;
#8521=ORIENTED_EDGE ( 'NONE', *, *, #24959, .T. ) ;
#8522=DIRECTION ( 'NONE',  ( 0.000000000000000000, 0.7381862504171926576, -0.6745969609292691294 ) ) ;
#8524=CARTESIAN_POINT ( 'NONE',  ( 35.00000000000000000, -12.09831040184922912, 1.463443770872898453 ) ) ;
#8527=AXIS2_PLACEMENT_3D ( 'NONE', #5856, #25446, #35732 ) ;
#8528=AXIS2_PLACEMENT_3D ( 'NONE', #8804, #64965, #19442 ) ;
#8534=EDGE_CURVE ( 'NONE', #56493, #22570, #8918, .T. ) ;
#8535=DIRECTION ( 'NONE',  ( 0.000000000000000000, -0.6943713148249534006, 0.7196168960969896444 ) ) ;
#8538=ORIENTED_EDGE ( 'NONE', *, *, #20735, .F. ) ;
#8540=CARTESIAN_POINT ( 'NONE',  ( -11.23710731435352983, -5.993765267744247005, -12.10435126123341654 ) ) ;
#8541=CARTESIAN_POINT ( 'NONE',  ( 36.00000000000000711, -12.66641127287626745, -1.457575200925504300 ) ) ;
#8545=CARTESIAN_POINT ( 'NONE',  ( 37.00000000000000711, 4.705694406421931860E-17, -3.469127814946512892E-15 ) ) ;
#8546=CIRCLE ( 'NONE', #1161, 12.74999999999999822 ) ;
#8548=CARTESIAN_POINT ( 'NONE',  ( 35.00000000000000000, 4.705694406421931860E-17, -3.469127814946512892E-15 ) ) ;
#8549=ORIENTED_EDGE ( 'NONE', *, *, #3625, .F. ) ;
#8555=CARTESIAN_POINT ( 'NONE',  ( 37.00000000000000711, -12.26766708251988902, 3.473736367725380969 ) ) ;
#8556=EDGE_CURVE ( 'NONE', #38380, #57471, #20734, .T. ) ;
#8558=CARTESIAN_POINT ( 'NONE',  ( -27.45775109278351067, -8.499184579339635448, -8.471355351200609007 ) ) ;
#8559=VERTEX_POINT ( 'NONE', #46302 ) ;
#8560=ORIENTED_EDGE ( 'NONE', *, *, #35880, .F. ) ;
#8566=EDGE_CURVE ( 'NONE', #63385, #45445, #6722, .T. ) ;
#8568=ORIENTED_EDGE ( 'NONE', *, *, #47600, .T. ) ;
#8569=AXIS2_PLACEMENT_3D ( 'NONE', #60100, #20522, #45786 ) ;
#8570=FACE_OUTER_BOUND ( 'NONE', #36526, .T. ) ;
#8573=ORIENTED_EDGE ( 'NONE', *, *, #59929, .T. ) ;
#8577=CYLINDRICAL_SURFACE ( 'NONE', #17418, 12.18649999999999878 ) ;
#8578=VERTEX_POINT ( 'NONE', #1410 ) ;
#8579=ORIENTED_EDGE ( 'NONE', *, *, #45409, .T. ) ;
#8581=DIRECTION ( 'NONE',  ( -1.000000000000000000, 0.000000000000000000, 0.000000000000000000 ) ) ;
#8582=AXIS2_PLACEMENT_3D ( 'NONE', #21121, #20484, #25463 ) ;
#8583=CARTESIAN_POINT ( 'NONE',  ( -35.00000000000000000, 10.68873102412852560, -6.950793414699680817 ) ) ;
#8584=DIRECTION ( 'NONE',  ( 1.000000000000000000, 0.000000000000000000, -0.000000000000000000 ) ) ;
#8586=AXIS2_PLACEMENT_3D ( 'NONE', #2623, #2933, #28503 ) ;
#8587=CYLINDRICAL_SURFACE ( 'NONE', #30109, 5.000000000000000888 ) ;
#8588=ORIENTED_EDGE ( 'NONE', *, *, #30900, .F. ) ;
#8589=CARTESIAN_POINT ( 'NONE',  ( 36.00000000000000711, 9.733281772932160791, -8.235637554476683775 ) ) ;
#8590=AXIS2_PLACEMENT_3D ( 'NONE', #6474, #27082, #16765 ) ;
#8591=FACE_OUTER_BOUND ( 'NONE', #13307, .T. ) ;
#8592=CARTESIAN_POINT ( 'NONE',  ( -19.16411987593509991, -13.50000000000000000, -0.3278540726586408049 ) ) ;
#8593=DIRECTION ( 'NONE',  ( 0.000000000000000000, -0.9551603052523509607, 0.2960891610144411601 ) ) ;
#8594=CARTESIAN_POINT ( 'NONE',  ( 37.00000000000000711, 4.705694406421931860E-17, -3.469127814946512892E-15 ) ) ;
#8597=DIRECTION ( 'NONE',  ( -1.000000000000000000, 0.000000000000000000, 0.000000000000000000 ) ) ;
#8598=LINE ( 'NONE', #53530, #34209 ) ;
#8599=VECTOR ( 'NONE', #49488, 1000.000000000000000 ) ;
#8600=EDGE_CURVE ( 'NONE', #31543, #42706, #56942, .T. ) ;
#8601=AXIS2_PLACEMENT_3D ( 'NONE', #12663, #27990, #62547 ) ;
#8604=CIRCLE ( 'NONE', #38362, 12.75000000000000178 ) ;
#8605=CIRCLE ( 'NONE', #109, 12.18650000000000411 ) ;
#8606=ORIENTED_EDGE ( 'NONE', *, *, #31329, .F. ) ;
#8607=CARTESIAN_POINT ( 'NONE',  ( 35.00000000000000000, 4.603882218679549609, -10.80631716521668828 ) ) ;
#8609=CARTESIAN_POINT ( 'NONE',  ( 12.90095149745135039, -12.25278169605762635, -5.681374632462030227 ) ) ;
#8610=CIRCLE ( 'NONE', #44717, 12.74999999999999822 ) ;
#8613=ORIENTED_EDGE ( 'NONE', *, *, #54370, .F. ) ;
#8614=CYLINDRICAL_SURFACE ( 'NONE', #41985, 5.000000000000000888 ) ;
#8615=CARTESIAN_POINT ( 'NONE',  ( 22.78406729994189561, -4.691424615418254618, 12.65938842238563744 ) ) ;
#8616=CIRCLE ( 'NONE', #16051, 5.000000000000001776 ) ;
#8624=CARTESIAN_POINT ( 'NONE',  ( -18.04458733766117362, 11.34280559204706584, 3.916728392552376370 ) ) ;
#8625=ORIENTED_EDGE ( 'NONE', *, *, #40382, .T. ) ;
#8626=CIRCLE ( 'NONE', #61676, 12.74999999999999822 ) ;
#8627=ADVANCED_FACE ( 'NONE', ( #35955 ), #56256, .T. ) ;
#8630=CARTESIAN_POINT ( 'NONE',  ( -35.00000000000000000, -11.90598845858530552, -4.561791185930540671 ) ) ;
#8633=CIRCLE ( 'NONE', #58598, 12.18650000000000233 ) ;
#8635=ORIENTED_EDGE ( 'NONE', *, *, #12603, .F. ) ;
#8638=FACE_OUTER_BOUND ( 'NONE', #24535, .T. ) ;
#8639=PLANE ( 'NONE',  #26579 ) ;
#8640=CARTESIAN_POINT ( 'NONE',  ( 37.00000000000000711, 4.705694406421931860E-17, -3.469127814946512892E-15 ) ) ;
#8648=VERTEX_POINT ( 'NONE', #41283 ) ;
#8649=DIRECTION ( 'NONE',  ( 0.000000000000000000, -0.01356324068817999114, 0.9999080150203989437 ) ) ;
#8651=CIRCLE ( 'NONE', #29904, 5.000000000000001776 ) ;
#8652=VECTOR ( 'NONE', #59577, 1000.000000000000000 ) ;
#8653=CARTESIAN_POINT ( 'NONE',  ( 35.00000000000000000, -9.700295462048712736, -7.376655759824850556 ) ) ;
#8654=ORIENTED_EDGE ( 'NONE', *, *, #12140, .T. ) ;
#8657=EDGE_CURVE ( 'NONE', #51572, #48935, #52234, .T. ) ;
#8659=ORIENTED_EDGE ( 'NONE', *, *, #48685, .T. ) ;
#8663=VERTEX_POINT ( 'NONE', #50959 ) ;
#8664=EDGE_CURVE ( 'NONE', #40351, #11560, #49051, .T. ) ;
#8666=ORIENTED_EDGE ( 'NONE', *, *, #59345, .F. ) ;
#8667=CYLINDRICAL_SURFACE ( 'NONE', #23235, 4.999999999999999112 ) ;
#8668=ORIENTED_EDGE ( 'NONE', *, *, #16873, .F. ) ;
#8669=CIRCLE ( 'NONE', #42618, 4.999999999999999112 ) ;
#8670=ORIENTED_EDGE ( 'NONE', *, *, #10421, .T. ) ;
#8671=VERTEX_POINT ( 'NONE', #14217 ) ;
#8672=DIRECTION ( 'NONE',  ( 0.000000000000000000, -0.01356324068817998940, 0.9999080150203990547 ) ) ;
#8673=DIRECTION ( 'NONE',  ( -0.000000000000000000, -1.000000000000000000, -0.000000000000000000 ) ) ;
#8674=CARTESIAN_POINT ( 'NONE',  ( 37.00000000000000711, -10.49626516989275693, -7.238157050195595410 ) ) ;
#8678=CARTESIAN_POINT ( 'NONE',  ( -37.00000000000000711, -0.3137578094508294280, -12.74613886779085625 ) ) ;
#8683=AXIS2_PLACEMENT_3D ( 'NONE', #13070, #63587, #32354 ) ;
#8684=CIRCLE ( 'NONE', #45843, 4.999999999999999112 ) ;
#8691=AXIS2_PLACEMENT_3D ( 'NONE', #63410, #43455, #7917 ) ;
#8692=EDGE_CURVE ( 'NONE', #55868, #12091, #57545, .T. ) ;
#8693=VECTOR ( 'NONE', #8264, 1000.000000000000000 ) ;
#8694=AXIS2_PLACEMENT_3D ( 'NONE', #41319, #16408, #27034 ) ;
#8697=ORIENTED_EDGE ( 'NONE', *, *, #51478, .T. ) ;
#8699=CARTESIAN_POINT ( 'NONE',  ( -47.00000000000000711, 0.000000000000000000, 0.000000000000000000 ) ) ;
#8700=CARTESIAN_POINT ( 'NONE',  ( 35.00000000000000000, 1.738225594540169894, 12.63095688309026698 ) ) ;
#8701=CARTESIAN_POINT ( 'NONE',  ( -36.00000000000000711, 12.31350058095527977, -3.307597835713114609 ) ) ;
#8703=EDGE_LOOP ( 'NONE', ( #55703, #24365, #53099, #56780 ) ) ;
#8709=ADVANCED_FACE ( 'NONE', ( #24524 ), #47602, .T. ) ;
#8715=EDGE_CURVE ( 'NONE', #43149, #49536, #22498, .T. ) ;
#8716=DIRECTION ( 'NONE',  ( 0.000000000000000000, -0.01356324068817998940, 0.9999080150203990547 ) ) ;
#8718=CARTESIAN_POINT ( 'NONE',  ( 35.00000000000000000, 11.23004253107771078, 4.732539170486136371 ) ) ;
#8721=CARTESIAN_POINT ( 'NONE',  ( -35.00000000000000000, 3.340853584269533716, 11.26103545359857350 ) ) ;
#8722=ORIENTED_EDGE ( 'NONE', *, *, #52776, .T. ) ;
#8725=CARTESIAN_POINT ( 'NONE',  ( 21.90174657591892071, 25.00000000000000000, -0.7349207973210698519 ) ) ;
#8729=ORIENTED_EDGE ( 'NONE', *, *, #23711, .T. ) ;
#8730=EDGE_LOOP ( 'NONE', ( #46585, #63041, #59448, #36277 ) ) ;
#8732=EDGE_CURVE ( 'NONE', #10033, #20614, #31774, .T. ) ;
#8733=VECTOR ( 'NONE', #5615, 1000.000000000000000 ) ;
#8734=CIRCLE ( 'NONE', #40577, 12.18649999999999878 ) ;
#8735=ORIENTED_EDGE ( 'NONE', *, *, #51640, .F. ) ;
#8736=EDGE_CURVE ( 'NONE', #4226, #30464, #3443, .T. ) ;
#8737=LINE ( 'NONE', #53646, #35580 ) ;
#8738=DIRECTION ( 'NONE',  ( 1.000000000000000000, -0.000000000000000000, 0.000000000000000000 ) ) ;
#8740=CARTESIAN_POINT ( 'NONE',  ( 17.92267017372352456, 8.274325337764011579, 8.703446854781846653 ) ) ;
#8743=CARTESIAN_POINT ( 'NONE',  ( -27.25055598261694456, -10.68287079889101321, 5.469009518302874184 ) ) ;
#8744=CARTESIAN_POINT ( 'NONE',  ( 35.00000000000000000, 4.705694406421931860E-17, -3.469127814946512892E-15 ) ) ;
#8745=DIRECTION ( 'NONE',  ( -1.000000000000000000, 0.000000000000000000, 0.000000000000000000 ) ) ;
#8747=ORIENTED_EDGE ( 'NONE', *, *, #37883, .T. ) ;
#8748=EDGE_CURVE ( 'NONE', #5051, #13765, #40576, .T. ) ;
#8750=ORIENTED_EDGE ( 'NONE', *, *, #2370, .F. ) ;
#8752=EDGE_LOOP ( 'NONE', ( #52665, #34170, #34533, #36288 ) ) ;
#8754=AXIS2_PLACEMENT_3D ( 'NONE', #45439, #65703, #238 ) ;
#8756=DIRECTION ( 'NONE',  ( -0.000000000000000000, -0.000000000000000000, -1.000000000000000000 ) ) ;
#8759=DIRECTION ( 'NONE',  ( 0.000000000000000000, -0.9651210252299766701, -0.2618041379715732586 ) ) ;
#8760=LINE ( 'NONE', #29043, #43771 ) ;
#8764=CARTESIAN_POINT ( 'NONE',  ( -37.00000000000000711, -9.926225166347071749, 6.280308599560108007 ) ) ;
#8767=VERTEX_POINT ( 'NONE', #3937 ) ;
#8769=DIRECTION ( 'NONE',  ( 1.000000000000000000, 0.000000000000000000, 0.000000000000000000 ) ) ;
#8774=EDGE_CURVE ( 'NONE', #44861, #42088, #34134, .T. ) ;
#8775=DIRECTION ( 'NONE',  ( -1.000000000000000000, 0.000000000000000000, -0.000000000000000000 ) ) ;
#8779=CARTESIAN_POINT ( 'NONE',  ( 35.00000000000000000, 6.584150480049550502, -10.25474254703955701 ) ) ;
#8781=CARTESIAN_POINT ( 'NONE',  ( 6.812204945636112896, -4.138731716409435712, -11.26369831714194092 ) ) ;
#8782=EDGE_LOOP ( 'NONE', ( #33332, #56272, #45052, #22194 ) ) ;
#8783=CIRCLE ( 'NONE', #34256, 12.18650000000000233 ) ;
#8785=AXIS2_PLACEMENT_3D ( 'NONE', #21879, #52786, #618 ) ;
#8790=DIRECTION ( 'NONE',  ( 0.000000000000000000, -0.01356324068817998940, 0.9999080150203990547 ) ) ;
#8792=DIRECTION ( 'NONE',  ( 0.000000000000000000, 0.01356324068817998940, -0.9999080150203990547 ) ) ;
#8793=AXIS2_PLACEMENT_3D ( 'NONE', #40077, #61341, #15783 ) ;
#8795=VECTOR ( 'NONE', #16650, 1000.000000000000000 ) ;
#8798=ORIENTED_EDGE ( 'NONE', *, *, #49107, .F. ) ;
#8799=FACE_OUTER_BOUND ( 'NONE', #24015, .T. ) ;
#8800=CARTESIAN_POINT ( 'NONE',  ( -9.634191421358215379, -11.15524410274445621, -4.443362378840637561 ) ) ;
#8801=CIRCLE ( 'NONE', #2455, 4.999999999999999112 ) ;
#8803=EDGE_LOOP ( 'NONE', ( #2216, #10108, #48059, #26647 ) ) ;
#8804=CARTESIAN_POINT ( 'NONE',  ( -35.00000000000000000, 6.891188680298823144, 9.512294188640927572 ) ) ;
#8808=LINE ( 'NONE', #44681, #58690 ) ;
#8810=ORIENTED_EDGE ( 'NONE', *, *, #41815, .F. ) ;
#8811=EDGE_CURVE ( 'NONE', #31809, #60956, #9758, .T. ) ;
#8812=LINE ( 'NONE', #43379, #21741 ) ;
#8813=FACE_OUTER_BOUND ( 'NONE', #16807, .T. ) ;
#8814=DIRECTION ( 'NONE',  ( 0.000000000000000000, -0.01356324068817998940, 0.9999080150203990547 ) ) ;
#8815=DIRECTION ( 'NONE',  ( 0.000000000000000000, -0.01356324068818000328, 0.9999080150203990547 ) ) ;
#8817=CARTESIAN_POINT ( 'NONE',  ( 37.00000000000000711, 9.913596905230228629, 8.017674001891673896 ) ) ;
#8818=ORIENTED_EDGE ( 'NONE', *, *, #7201, .T. ) ;
#8820=ORIENTED_EDGE ( 'NONE', *, *, #172, .T. ) ;
#8822=EDGE_LOOP ( 'NONE', ( #34719, #56140, #14936, #42174 ) ) ;
#8825=CARTESIAN_POINT ( 'NONE',  ( -18.55576795264365941, 5.671152142829758880, 12.25417085568500219 ) ) ;
#8827=AXIS2_PLACEMENT_3D ( 'NONE', #9412, #3828, #44343 ) ;
#8828=CARTESIAN_POINT ( 'NONE',  ( -37.00000000000000711, -11.05394794832833583, 5.130401251914692651 ) ) ;
#8829=CARTESIAN_POINT ( 'NONE',  ( 24.19939926762688032, 0.7067538267882510494, 11.98446061403317131 ) ) ;
#8830=CARTESIAN_POINT ( 'NONE',  ( 36.00000000000000711, -2.865935305911542663, 12.42372387097884712 ) ) ;
#8831=LINE ( 'NONE', #23815, #13945 ) ;
#8832=ORIENTED_EDGE ( 'NONE', *, *, #12662, .T. ) ;
#8833=VERTEX_POINT ( 'NONE', #45143 ) ;
#8834=CARTESIAN_POINT ( 'NONE',  ( -35.00000000000000000, 15.00000000000000000, 1.836970198721029589E-15 ) ) ;
#8835=VECTOR ( 'NONE', #20297, 1000.000000000000000 ) ;
#8836=DIRECTION ( 'NONE',  ( 1.000000000000000000, 0.000000000000000000, 0.000000000000000000 ) ) ;
#8837=B_SPLINE_CURVE_WITH_KNOTS ( 'NONE', 3,
 ( #46787, #61410, #10539, #46152, #60776, #51483, #15210, #30817, #19882, #35148, #40823, #35494, #61101, #10222, #9898, #35801, #51137, #11219 ),
 .UNSPECIFIED., .F., .F.,
 ( 4, 2, 2, 2, 2, 2, 2, 2, 4 ),
 ( 1.409462824231155764E-18, 0.001129207483351105362, 0.002258414966702208988, 0.003387622450053312615, 0.004516829933404417109, 0.005646037416755521170, 0.006775244900106624363, 0.007904452383457728423, 0.009033659866808832484 ),
 .UNSPECIFIED. ) ;
#8839=AXIS2_PLACEMENT_3D ( 'NONE', #50507, #25212, #45488 ) ;
#8840=DIRECTION ( 'NONE',  ( 1.000000000000000000, 0.000000000000000000, 0.000000000000000000 ) ) ;
#8842=CARTESIAN_POINT ( 'NONE',  ( -35.00000000000000000, 11.91791701451266405, 2.544412758415886877 ) ) ;
#8844=CARTESIAN_POINT ( 'NONE',  ( -36.00000000000000711, 12.74921544981111232, -0.1414404973752581562 ) ) ;
#8846=ADVANCED_FACE ( 'NONE', ( #55781 ), #30175, .T. ) ;
#8847=VERTEX_POINT ( 'NONE', #10212 ) ;
#8850=DIRECTION ( 'NONE',  ( 1.000000000000000000, 0.000000000000000000, 0.000000000000000000 ) ) ;
#8851=DIRECTION ( 'NONE',  ( -1.000000000000000000, 0.000000000000000000, 0.000000000000000000 ) ) ;
#8852=LINE ( 'NONE', #2903, #3688 ) ;
#8853=EDGE_CURVE ( 'NONE', #63312, #35169, #6605, .T. ) ;
#8856=CARTESIAN_POINT ( 'NONE',  ( -10.75289514965179549, -6.158246205637091464, -10.30132767016891471 ) ) ;
#8859=CARTESIAN_POINT ( 'NONE',  ( 37.00000000000000711, 11.96656215839374759, 4.400442035670818264 ) ) ;
#8861=EDGE_LOOP ( 'NONE', ( #45033, #43162 ) ) ;
#8862=CIRCLE ( 'NONE', #9955, 12.18650000000000055 ) ;
#8864=CARTESIAN_POINT ( 'NONE',  ( 17.36549340976883116, 11.88942698613074178, 6.436805334688243008 ) ) ;
#8865=CARTESIAN_POINT ( 'NONE',  ( 35.00000000000000000, 4.705694406421931860E-17, -3.469127814946512892E-15 ) ) ;
#8866=EDGE_CURVE ( 'NONE', #40799, #28364, #26764, .T. ) ;
#8867=AXIS2_PLACEMENT_3D ( 'NONE', #54911, #39942, #49931 ) ;
#8868=AXIS2_PLACEMENT_3D ( 'NONE', #57735, #17487, #41417 ) ;
#8870=DIRECTION ( 'NONE',  ( 1.000000000000000000, 0.000000000000000000, 0.000000000000000000 ) ) ;
#8871=EDGE_LOOP ( 'NONE', ( #62124, #54873, #3370, #9589 ) ) ;
#8876=EDGE_LOOP ( 'NONE', ( #9244, #21220, #56690, #19306 ) ) ;
#8877=CARTESIAN_POINT ( 'NONE',  ( -11.40165637462999904, -7.742630519260993438, -9.172861531003599467 ) ) ;
#8878=DIRECTION ( 'NONE',  ( 0.000000000000000000, -0.01356324068817991828, 0.9999080150203990547 ) ) ;
#8879=FACE_OUTER_BOUND ( 'NONE', #31318, .T. ) ;
#8880=DIRECTION ( 'NONE',  ( -1.000000000000000000, 0.000000000000000000, 0.000000000000000000 ) ) ;
#8882=ADVANCED_FACE ( 'NONE', ( #56426 ), #51125, .T. ) ;
#8883=CIRCLE ( 'NONE', #5725, 12.18650000000000055 ) ;
#8886=CYLINDRICAL_SURFACE ( 'NONE', #19555, 12.74999999999999822 ) ;
#8889=VECTOR ( 'NONE', #34636, 1000.000000000000000 ) ;
#8891=CARTESIAN_POINT ( 'NONE',  ( 37.00000000000000711, 6.753013023069713405, -10.14433819232436917 ) ) ;
#8893=CIRCLE ( 'NONE', #17394, 12.18650000000000055 ) ;
#8894=CARTESIAN_POINT ( 'NONE',  ( -30.15674304214251933, -0.5118533057020833166, -11.99746462915879697 ) ) ;
#8895=FACE_OUTER_BOUND ( 'NONE', #62220, .T. ) ;
#8896=ORIENTED_EDGE ( 'NONE', *, *, #10424, .F. ) ;
#8897=ORIENTED_EDGE ( 'NONE', *, *, #33828, .F. ) ;
#8899=VERTEX_POINT ( 'NONE', #7186 ) ;
#8900=EDGE_CURVE ( 'NONE', #24451, #48418, #11520, .T. ) ;
#8901=CARTESIAN_POINT ( 'NONE',  ( 37.00000000000000711, -0.01609748574436820068, 11.74614673114903596 ) ) ;
#8902=CIRCLE ( 'NONE', #48186, 12.18649999999999878 ) ;
#8906=DIRECTION ( 'NONE',  ( 0.000000000000000000, -0.01356324068817991828, 0.9999080150203990547 ) ) ;
#8907=VERTEX_POINT ( 'NONE', #6554 ) ;
#8908=ORIENTED_EDGE ( 'NONE', *, *, #15582, .F. ) ;
#8910=CIRCLE ( 'NONE', #52458, 12.75000000000000178 ) ;
#8911=CYLINDRICAL_SURFACE ( 'NONE', #39712, 12.18649999999999878 ) ;
#8912=CIRCLE ( 'NONE', #46091, 5.000000000000000888 ) ;
#8914=EDGE_LOOP ( 'NONE', ( #43319, #19436, #52977, #16717 ) ) ;
#8916=CARTESIAN_POINT ( 'NONE',  ( 35.00000000000000000, 4.705694406421931860E-17, -3.469127814946512892E-15 ) ) ;
#8917=VECTOR ( 'NONE', #23036, 1000.000000000000000 ) ;
#8918=LINE ( 'NONE', #49180, #8693 ) ;
#8920=DIRECTION ( 'NONE',  ( 0.000000000000000000, -0.01356324068817998940, 0.9999080150203990547 ) ) ;
#8922=( BOUNDED_CURVE ( )  B_SPLINE_CURVE ( 3, ( #52051, #56735, #16139, #16786 ),
 .UNSPECIFIED., .F., .F. ) 
 B_SPLINE_CURVE_WITH_KNOTS ( ( 4, 4 ),
 ( 3.502726250925535023, 3.584222553583020332 ),
 .UNSPECIFIED. ) 
 CURVE ( )  GEOMETRIC_REPRESENTATION_ITEM ( )  RATIONAL_B_SPLINE_CURVE ( ( 1.000000000000000000, 0.9994466059659543600, 0.9994466059659543600, 1.000000000000000000 ) ) 
 REPRESENTATION_ITEM ( '' )  );
#8926=AXIS2_PLACEMENT_3D ( 'NONE', #11867, #12511, #26845 ) ;
#8928=EDGE_CURVE ( 'NONE', #11758, #7009, #60751, .T. ) ;
#8929=LINE ( 'NONE', #39832, #20447 ) ;
#8930=DIRECTION ( 'NONE',  ( -1.000000000000000000, 0.000000000000000000, -0.000000000000000000 ) ) ;
#8931=CARTESIAN_POINT ( 'NONE',  ( 27.15326549950207635, 11.36256450630621728, 3.875020145684566764 ) ) ;
#8932=AXIS2_PLACEMENT_3D ( 'NONE', #55121, #9547, #29841 ) ;
#8935=CARTESIAN_POINT ( 'NONE',  ( -37.00000000000000711, 10.93004082984018588, 6.564808257521811186 ) ) ;
#8936=CARTESIAN_POINT ( 'NONE',  ( -35.00000000000000000, 0.000000000000000000, 0.000000000000000000 ) ) ;
#8942=ORIENTED_EDGE ( 'NONE', *, *, #15666, .F. ) ;
#8946=CARTESIAN_POINT ( 'NONE',  ( -36.00000000000000711, -8.496612874013226957, 9.506317355798342916 ) ) ;
#8948=CARTESIAN_POINT ( 'NONE',  ( -35.00000000000000000, 2.544412758416015219, -11.91791701451263741 ) ) ;
#8951=DIRECTION ( 'NONE',  ( 0.000000000000000000, -0.9796553971857722143, -0.2006870767258996102 ) ) ;
#8952=DIRECTION ( 'NONE',  ( 0.000000000000000000, -0.9970832820307031774, -0.07632122047557582389 ) ) ;
#8955=EDGE_CURVE ( 'NONE', #37930, #27528, #46852, .T. ) ;
#8956=DIRECTION ( 'NONE',  ( 1.000000000000000000, 0.000000000000000000, 0.000000000000000000 ) ) ;
#8957=ORIENTED_EDGE ( 'NONE', *, *, #6293, .F. ) ;
#8958=DIRECTION ( 'NONE',  ( -0.000000000000000000, -1.000000000000000000, -0.000000000000000000 ) ) ;
#8961=DIRECTION ( 'NONE',  ( -1.000000000000000000, 0.000000000000000000, 0.000000000000000000 ) ) ;
#8962=CIRCLE ( 'NONE', #56784, 12.74999999999999822 ) ;
#8963=VECTOR ( 'NONE', #26215, 1000.000000000000000 ) ;
#8964=CARTESIAN_POINT ( 'NONE',  ( 37.00000000000000711, 4.705694406421931860E-17, -3.469127814946512892E-15 ) ) ;
#8966=ORIENTED_EDGE ( 'NONE', *, *, #65188, .F. ) ;
#8967=ORIENTED_EDGE ( 'NONE', *, *, #3894, .T. ) ;
#8968=CARTESIAN_POINT ( 'NONE',  ( 3.780834652287974773, 8.352030633203074927, -10.60629927458383470 ) ) ;
#8970=CYLINDRICAL_SURFACE ( 'NONE', #17300, 12.18649999999999878 ) ;
#8971=CARTESIAN_POINT ( 'NONE',  ( -37.00000000000000711, 4.237620530777800987, 11.42599468261430928 ) ) ;
#8974=CARTESIAN_POINT ( 'NONE',  ( -18.04458733766117362, -11.34280559204704097, 3.916728392552376370 ) ) ;
#8975=ORIENTED_EDGE ( 'NONE', *, *, #49656, .T. ) ;
#8976=VERTEX_POINT ( 'NONE', #47450 ) ;
#8977=EDGE_LOOP ( 'NONE', ( #62373, #58401, #53420, #39294 ) ) ;
#8979=AXIS2_PLACEMENT_3D ( 'NONE', #50036, #38747, #55010 ) ;
#8980=EDGE_CURVE ( 'NONE', #5010, #11924, #52445, .T. ) ;
#8982=VERTEX_POINT ( 'NONE', #6883 ) ;
#8983=CARTESIAN_POINT ( 'NONE',  ( -37.00000000000000711, -9.348667969174352166, -7.817492529713958582 ) ) ;
#8984=FACE_BOUND ( 'NONE', #9121, .T. ) ;
#8985=ORIENTED_EDGE ( 'NONE', *, *, #13, .T. ) ;
#8990=ORIENTED_EDGE ( 'NONE', *, *, #62250, .T. ) ;
#8991=FACE_OUTER_BOUND ( 'NONE', #26171, .T. ) ;
#8992=VERTEX_POINT ( 'NONE', #32451 ) ;
#8993=CARTESIAN_POINT ( 'NONE',  ( 35.00000000000000000, -11.17622378668003691, 3.614449339633606595 ) ) ;
#8994=ORIENTED_EDGE ( 'NONE', *, *, #63483, .T. ) ;
#8996=ORIENTED_EDGE ( 'NONE', *, *, #27889, .T. ) ;
#8997=CARTESIAN_POINT ( 'NONE',  ( -27.01437459610461644, 8.723448335974111956, -8.240233560378637634 ) ) ;
#9001=DIRECTION ( 'NONE',  ( 1.000000000000000000, 0.000000000000000000, 0.000000000000000000 ) ) ;
#9003=ORIENTED_EDGE ( 'NONE', *, *, #59582, .F. ) ;
#9008=CARTESIAN_POINT ( 'NONE',  ( -17.64636966839529109, -7.707522472056596463, -11.08736416828873850 ) ) ;
#9009=EDGE_CURVE ( 'NONE', #35706, #50717, #58079, .T. ) ;
#9015=ORIENTED_EDGE ( 'NONE', *, *, #41723, .T. ) ;
#9019=ADVANCED_FACE ( 'NONE', ( #62378 ), #53077, .T. ) ;
#9024=CARTESIAN_POINT ( 'NONE',  ( -19.55186598411636467, -3.901828651817480953, -12.92480312515320229 ) ) ;
#9025=AXIS2_PLACEMENT_3D ( 'NONE', #37625, #57922, #52912 ) ;
#9026=ORIENTED_EDGE ( 'NONE', *, *, #30080, .T. ) ;
#9029=CIRCLE ( 'NONE', #4818, 5.000000000000000000 ) ;
#9030=EDGE_CURVE ( 'NONE', #64802, #33595, #65122, .T. ) ;
#9034=DIRECTION ( 'NONE',  ( 0.000000000000000000, 0.01356324068817998940, -0.9999080150203990547 ) ) ;
#9035=CARTESIAN_POINT ( 'NONE',  ( 6.987038089383098338, -8.045544563376781255, -8.914883656081883601 ) ) ;
#9037=AXIS2_PLACEMENT_3D ( 'NONE', #16699, #41641, #61928 ) ;
#9039=ORIENTED_EDGE ( 'NONE', *, *, #55650, .F. ) ;
#9040=CARTESIAN_POINT ( 'NONE',  ( 35.00000000000000000, -5.130401251914806338, -11.05394794832827898 ) ) ;
#9041=EDGE_LOOP ( 'NONE', ( #30156, #52584, #44895, #39219 ) ) ;
#9042=DIRECTION ( 'NONE',  ( -1.000000000000000000, 0.000000000000000000, 0.000000000000000000 ) ) ;
#9046=VERTEX_POINT ( 'NONE', #18821 ) ;
#9048=ORIENTED_EDGE ( 'NONE', *, *, #5789, .T. ) ;
#9050=CARTESIAN_POINT ( 'NONE',  ( -17.83419946441818027, -9.720786832536937538, 9.367833439828872955 ) ) ;
#9052=ORIENTED_EDGE ( 'NONE', *, *, #55805, .F. ) ;
#9053=DIRECTION ( 'NONE',  ( -1.000000000000000000, 0.000000000000000000, -0.000000000000000000 ) ) ;
#9054=DIRECTION ( 'NONE',  ( 1.000000000000000000, 0.000000000000000000, 0.000000000000000000 ) ) ;
#9055=LINE ( 'NONE', #64894, #47162 ) ;
#9056=CARTESIAN_POINT ( 'NONE',  ( -2.532614230583026593, 25.00000000000000000, 10.89930238848911337 ) ) ;
#9058=AXIS2_PLACEMENT_3D ( 'NONE', #62185, #25970, #20952 ) ;
#9061=CARTESIAN_POINT ( 'NONE',  ( -29.68541646480307250, -1.795142075051132657, -11.87110896435279095 ) ) ;
#9062=DIRECTION ( 'NONE',  ( 1.000000000000000000, 0.000000000000000000, 0.000000000000000000 ) ) ;
#9063=VERTEX_POINT ( 'NONE', #53427 ) ;
#9066=CARTESIAN_POINT ( 'NONE',  ( -29.43980975494970309, -3.641506875706030488, -11.43413432115371364 ) ) ;
#9068=ORIENTED_EDGE ( 'NONE', *, *, #58195, .T. ) ;
#9071=AXIS2_PLACEMENT_3D ( 'NONE', #38244, #48582, #17983 ) ;
#9072=CARTESIAN_POINT ( 'NONE',  ( 47.00000000000000711, 4.705694406421931860E-17, -3.469127814946512892E-15 ) ) ;
#9073=CARTESIAN_POINT ( 'NONE',  ( -35.00000000000000000, 11.47758908105694786, 2.497432891016883261 ) ) ;
#9075=EDGE_CURVE ( 'NONE', #62046, #31684, #53063, .T. ) ;
#9079=ORIENTED_EDGE ( 'NONE', *, *, #19364, .T. ) ;
#9080=ORIENTED_EDGE ( 'NONE', *, *, #62412, .F. ) ;
#9082=ORIENTED_EDGE ( 'NONE', *, *, #7922, .F. ) ;
#9083=EDGE_CURVE ( 'NONE', #9626, #29988, #44085, .T. ) ;
#9084=ORIENTED_EDGE ( 'NONE', *, *, #64014, .F. ) ;
#9086=CARTESIAN_POINT ( 'NONE',  ( -37.00000000000000711, -4.426194442447159538, -11.35427606708811332 ) ) ;
#9088=DIRECTION ( 'NONE',  ( 0.000000000000000000, 0.8989688749565142301, 0.4380125133594005016 ) ) ;
#9090=FACE_OUTER_BOUND ( 'NONE', #14510, .T. ) ;
#9091=CYLINDRICAL_SURFACE ( 'NONE', #12000, 12.18650000000000055 ) ;
#9094=CARTESIAN_POINT ( 'NONE',  ( 37.00000000000000711, -6.584150480049477672, 10.25474254703959431 ) ) ;
#9096=DIRECTION ( 'NONE',  ( 0.000000000000000000, -0.1118654143051477368, -0.9937233664769776764 ) ) ;
#9098=VERTEX_POINT ( 'NONE', #38776 ) ;
#9101=CIRCLE ( 'NONE', #18682, 5.000000000000000888 ) ;
#9102=CARTESIAN_POINT ( 'NONE',  ( -11.12450214041353291, -5.606564972075692488, 12.28260682454939179 ) ) ;
#9104=CARTESIAN_POINT ( 'NONE',  ( -10.61430208547403886, -9.391830329834835567, -9.709184090487172014 ) ) ;
#9105=ORIENTED_EDGE ( 'NONE', *, *, #65433, .T. ) ;
#9106=CARTESIAN_POINT ( 'NONE',  ( -35.00000000000000000, 2.021542716731397071, 12.01765980939842748 ) ) ;
#9107=DIRECTION ( 'NONE',  ( -1.000000000000000000, 0.000000000000000000, 0.000000000000000000 ) ) ;
#9108=CARTESIAN_POINT ( 'NONE',  ( 3.847381992255190841, 5.216794478567112314, 10.80899677692140592 ) ) ;
#9109=AXIS2_PLACEMENT_3D ( 'NONE', #55699, #36038, #5496 ) ;
#9110=CARTESIAN_POINT ( 'NONE',  ( 6.812204945636112896, -4.138731716409435712, 12.84993773446340803 ) ) ;
#9113=VERTEX_POINT ( 'NONE', #9466 ) ;
#9115=CARTESIAN_POINT ( 'NONE',  ( 35.00000000000000000, 8.029056188533806093, 8.573591947375229338 ) ) ;
#9116=CARTESIAN_POINT ( 'NONE',  ( 37.00000000000000711, 10.30098186818249673, -5.644643009979106729 ) ) ;
#9118=CARTESIAN_POINT ( 'NONE',  ( 21.74669156475645693, 13.45922031030403332, -1.115717662970064694 ) ) ;
#9121=EDGE_LOOP ( 'NONE', ( #40940, #50778, #14602, #13193 ) ) ;
#9122=VERTEX_POINT ( 'NONE', #30424 ) ;
#9123=CYLINDRICAL_SURFACE ( 'NONE', #14029, 4.999999999999999112 ) ;
#9124=EDGE_CURVE ( 'NONE', #53395, #17729, #5429, .T. ) ;
#9125=VERTEX_POINT ( 'NONE', #29750 ) ;
#9126=CARTESIAN_POINT ( 'NONE',  ( -37.00000000000000711, 6.753013023069858178, -10.14433819232427147 ) ) ;
#9133=CARTESIAN_POINT ( 'NONE',  ( 35.00000000000000000, -10.23119532541066867, 7.608228585767831120 ) ) ;
#9134=VERTEX_POINT ( 'NONE', #5170 ) ;
#9135=CARTESIAN_POINT ( 'NONE',  ( -35.00000000000000000, 10.62137734850268345, 5.015831474386344802 ) ) ;
#9136=EDGE_LOOP ( 'NONE', ( #51631, #17796, #10008, #30569 ) ) ;
#9137=EDGE_CURVE ( 'NONE', #52774, #28155, #18189, .T. ) ;
#9138=VERTEX_POINT ( 'NONE', #5508 ) ;
#9139=CARTESIAN_POINT ( 'NONE',  ( -37.00000000000000711, 0.000000000000000000, 0.000000000000000000 ) ) ;
#9141=CARTESIAN_POINT ( 'NONE',  ( -24.67206623709094515, 8.916871779494830008, 10.14344027151376615 ) ) ;
#9142=CARTESIAN_POINT ( 'NONE',  ( 24.40079717985569374, -0.3635673505086269852, 11.99993777491598834 ) ) ;
#9145=DIRECTION ( 'NONE',  ( 0.000000000000000000, 0.01356324068817999114, -0.9999080150203990547 ) ) ;
#9148=ORIENTED_EDGE ( 'NONE', *, *, #52671, .T. ) ;
#9152=ORIENTED_EDGE ( 'NONE', *, *, #2718, .T. ) ;
#9155=FACE_OUTER_BOUND ( 'NONE', #56684, .T. ) ;
#9164=CARTESIAN_POINT ( 'NONE',  ( -35.00000000000000000, -11.59605747147782928, -5.300372733891765442 ) ) ;
#9165=ADVANCED_FACE ( 'NONE', ( #35059 ), #10796, .T. ) ;
#9166=CARTESIAN_POINT ( 'NONE',  ( 47.00000000000000711, 4.705694406421931860E-17, -3.469127814946512892E-15 ) ) ;
#9167=CARTESIAN_POINT ( 'NONE',  ( -36.00000000000000711, 10.23119532541083743, -7.608228585767615293 ) ) ;
#9168=EDGE_CURVE ( 'NONE', #35378, #26733, #30097, .T. ) ;
#9169=CARTESIAN_POINT ( 'NONE',  ( 7.302720544406653858, -6.253920029920363000, -11.96596573125614960 ) ) ;
#9170=CARTESIAN_POINT ( 'NONE',  ( 35.00000000000000000, 12.17626345777663488, -0.4993900848167889817 ) ) ;
#9173=DIRECTION ( 'NONE',  ( -0.9790892447477997917, -0.2034311943119418153, 0.000000000000000000 ) ) ;
#9177=DIRECTION ( 'NONE',  ( -1.000000000000000000, 0.000000000000000000, 0.000000000000000000 ) ) ;
#9178=AXIS2_PLACEMENT_3D ( 'NONE', #43999, #3790, #13399 ) ;
#9179=EDGE_CURVE ( 'NONE', #59672, #60252, #24386, .T. ) ;
#9180=CIRCLE ( 'NONE', #58045, 12.75000000000000178 ) ;
#9183=ORIENTED_EDGE ( 'NONE', *, *, #5347, .F. ) ;
#9185=FACE_OUTER_BOUND ( 'NONE', #47747, .T. ) ;
#9188=CARTESIAN_POINT ( 'NONE',  ( 37.00000000000000711, 4.705694406421931860E-17, -3.469127814946512892E-15 ) ) ;
#9189=CARTESIAN_POINT ( 'NONE',  ( -27.88094468144726790, -11.21297357817068452, -7.541748090003880911 ) ) ;
#9190=DIRECTION ( 'NONE',  ( 1.000000000000000000, -0.000000000000000000, -0.000000000000000000 ) ) ;
#9194=VERTEX_POINT ( 'NONE', #51713 ) ;
#9196=EDGE_CURVE ( 'NONE', #21896, #22627, #22405, .T. ) ;
#9197=CARTESIAN_POINT ( 'NONE',  ( 36.00000000000000711, -11.47561260193572963, 5.556331110570524423 ) ) ;
#9198=DIRECTION ( 'NONE',  ( 0.000000000000000000, -1.000000000000000000, 0.000000000000000000 ) ) ;
#9200=CARTESIAN_POINT ( 'NONE',  ( -35.00000000000000000, 2.772148766916116891, 11.86701198550357361 ) ) ;
#9202=DIRECTION ( 'NONE',  ( 0.000000000000000000, -0.7790879021242440583, 0.6269146997508067143 ) ) ;
#9203=DIRECTION ( 'NONE',  ( -1.000000000000000000, -0.000000000000000000, 0.000000000000000000 ) ) ;
#9204=ORIENTED_EDGE ( 'NONE', *, *, #18430, .T. ) ;
#9205=ORIENTED_EDGE ( 'NONE', *, *, #64676, .T. ) ;
#9207=ORIENTED_EDGE ( 'NONE', *, *, #38065, .F. ) ;
#9209=DIRECTION ( 'NONE',  ( 0.6088860180392798860, 0.7932577242209933877, 0.000000000000000000 ) ) ;
#9210=EDGE_LOOP ( 'NONE', ( #51044, #42750, #39048, #8165 ) ) ;
#9212=CARTESIAN_POINT ( 'NONE',  ( 12.18100207966124415, 11.65630975953624393, -2.856157803748045509 ) ) ;
#9214=ORIENTED_EDGE ( 'NONE', *, *, #27357, .F. ) ;
#9215=ORIENTED_EDGE ( 'NONE', *, *, #42615, .F. ) ;
#9217=EDGE_CURVE ( 'NONE', #16581, #30718, #4385, .T. ) ;
#9219=DIRECTION ( 'NONE',  ( 1.000000000000000000, 0.000000000000000000, 0.000000000000000000 ) ) ;
#9221=CIRCLE ( 'NONE', #17704, 4.999999999999999112 ) ;
#9223=EDGE_LOOP ( 'NONE', ( #19969, #30951, #8666, #33867 ) ) ;
#9226=DIRECTION ( 'NONE',  ( -1.000000000000000000, 0.000000000000000000, 0.000000000000000000 ) ) ;
#9227=DIRECTION ( 'NONE',  ( 1.000000000000000000, -0.000000000000000000, 0.000000000000000000 ) ) ;
#9229=AXIS2_PLACEMENT_3D ( 'NONE', #50296, #4751, #10041 ) ;
#9230=CARTESIAN_POINT ( 'NONE',  ( 36.00000000000000711, -9.506317355798431734, -8.496612874013129257 ) ) ;
#9231=ORIENTED_EDGE ( 'NONE', *, *, #41570, .F. ) ;
#9233=CARTESIAN_POINT ( 'NONE',  ( -18.08686583997241115, 5.151216734910855521, 10.83812558286605920 ) ) ;
#9234=CARTESIAN_POINT ( 'NONE',  ( 37.00000000000000711, -12.09831040184922912, 1.463443770872898453 ) ) ;
#9235=CARTESIAN_POINT ( 'NONE',  ( -37.00000000000000711, 0.000000000000000000, 0.000000000000000000 ) ) ;
#9238=CARTESIAN_POINT ( 'NONE',  ( 19.28625800530497258, -6.413918128308385036, 11.87904264843581537 ) ) ;
#9240=LINE ( 'NONE', #30192, #22547 ) ;
#9241=EDGE_CURVE ( 'NONE', #55845, #21734, #23449, .T. ) ;
#9244=ORIENTED_EDGE ( 'NONE', *, *, #1259, .F. ) ;
#9249=DIRECTION ( 'NONE',  ( -1.000000000000000000, 0.000000000000000000, 0.000000000000000000 ) ) ;
#9250=ORIENTED_EDGE ( 'NONE', *, *, #2579, .F. ) ;
#9253=FACE_OUTER_BOUND ( 'NONE', #52814, .T. ) ;
#9255=ADVANCED_FACE ( 'NONE', ( #1819 ), #11139, .T. ) ;
#9256=CARTESIAN_POINT ( 'NONE',  ( 37.00000000000000711, 11.42599468261429152, -4.237620530777845396 ) ) ;
#9258=CARTESIAN_POINT ( 'NONE',  ( -18.55764555710201336, 11.94984199981902862, 1.281878970701318510 ) ) ;
#9259=ORIENTED_EDGE ( 'NONE', *, *, #28512, .F. ) ;
#9260=DIRECTION ( 'NONE',  ( 0.000000000000000000, 0.01356324068817992175, -0.9999080150203990547 ) ) ;
#9261=DIRECTION ( 'NONE',  ( 1.000000000000000000, 0.000000000000000000, 0.000000000000000000 ) ) ;
#9262=B_SPLINE_CURVE_WITH_KNOTS ( 'NONE', 3,
 ( #40158, #60451, #9916, #30203, #50501, #4944, #25205, #60791, #15227, #55809, #10236, #18923, #6251, #26200, #1602, #15550, #26514, #926, #31191, #31816 ),
 .UNSPECIFIED., .F., .F.,
 ( 4, 2, 2, 2, 2, 2, 2, 2, 2, 4 ),
 ( 0.002662675774314247901, 0.003376488722711035520, 0.004090301671107823139, 0.004804114619504610759, 0.005517927567901398378, 0.006231740516298185997, 0.006945553464694973617, 0.007659366413091766440, 0.008016272887290162852, 0.008373179361488559264 ),
 .UNSPECIFIED. ) ;
#9263=AXIS2_PLACEMENT_3D ( 'NONE', #8916, #29206, #49503 ) ;
#9264=CARTESIAN_POINT ( 'NONE',  ( 35.00000000000000000, 12.16632754454236398, -0.7008968033239244555 ) ) ;
#9265=CARTESIAN_POINT ( 'NONE',  ( 6.521272285098597798, -4.688064980771462942, 12.66474591211187040 ) ) ;
#9269=ORIENTED_EDGE ( 'NONE', *, *, #10532, .T. ) ;
#9270=EDGE_CURVE ( 'NONE', #26831, #49092, #7538, .T. ) ;
#9272=FACE_OUTER_BOUND ( 'NONE', #11175, .T. ) ;
#9276=DIRECTION ( 'NONE',  ( 0.000000000000000000, 0.01356324068817998940, -0.9999080150203990547 ) ) ;
#9277=CARTESIAN_POINT ( 'NONE',  ( -14.29135464769095520, 7.782112657557433089, 9.134479874907178498 ) ) ;
#9279=VERTEX_POINT ( 'NONE', #32052 ) ;
#9285=EDGE_LOOP ( 'NONE', ( #49688, #8722, #23848, #46499 ) ) ;
#9286=FACE_BOUND ( 'NONE', #7018, .T. ) ;
#9287=VERTEX_POINT ( 'NONE', #26753 ) ;
#9288=CYLINDRICAL_SURFACE ( 'NONE', #49281, 5.000000000000000888 ) ;
#9290=CARTESIAN_POINT ( 'NONE',  ( 7.006458457944364504, -4.543415500168663357, 11.11500136487966195 ) ) ;
#9293=CARTESIAN_POINT ( 'NONE',  ( 37.00000000000000711, -12.08216339958901564, -1.591260454995201412 ) ) ;
#9294=ORIENTED_EDGE ( 'NONE', *, *, #3077, .F. ) ;
#9296=EDGE_CURVE ( 'NONE', #43631, #1814, #36401, .T. ) ;
#9298=VERTEX_POINT ( 'NONE', #52369 ) ;
#9300=CARTESIAN_POINT ( 'NONE',  ( 37.00000000000000711, -1.262958560998847624, -12.12087942037209665 ) ) ;
#9302=CIRCLE ( 'NONE', #60291, 12.18650000000000233 ) ;
#9303=DIRECTION ( 'NONE',  ( 1.000000000000000000, 0.000000000000000000, 0.000000000000000000 ) ) ;
#9304=CARTESIAN_POINT ( 'NONE',  ( 35.00000000000000000, -8.235637554476710420, -9.733281772932135922 ) ) ;
#9305=ORIENTED_EDGE ( 'NONE', *, *, #43203, .F. ) ;
#9309=CYLINDRICAL_SURFACE ( 'NONE', #11502, 5.000000000000000888 ) ;
#9310=CARTESIAN_POINT ( 'NONE',  ( -35.00000000000000000, 0.000000000000000000, 0.000000000000000000 ) ) ;
#9311=ORIENTED_EDGE ( 'NONE', *, *, #41123, .F. ) ;
#9312=CARTESIAN_POINT ( 'NONE',  ( -27.01437459610461644, 13.31613970204373132, -2.220455681983952267 ) ) ;
#9313=CARTESIAN_POINT ( 'NONE',  ( -47.00000000000000711, 0.000000000000000000, 0.000000000000000000 ) ) ;
#9314=CARTESIAN_POINT ( 'NONE',  ( 9.687175622948609899, 25.00000000000000000, -0.5854820436212360146 ) ) ;
#9316=ORIENTED_EDGE ( 'NONE', *, *, #35720, .F. ) ;
#9320=VERTEX_POINT ( 'NONE', #42033 ) ;
#9325=CARTESIAN_POINT ( 'NONE',  ( 11.70595570239210836, 11.89565203838692575, -1.585121128597035467 ) ) ;
#9326=EDGE_LOOP ( 'NONE', ( #37507, #20381, #63236, #57303, #16987 ) ) ;
#9327=EDGE_CURVE ( 'NONE', #28181, #37836, #24537, .T. ) ;
#9330=EDGE_CURVE ( 'NONE', #56916, #95, #44690, .T. ) ;
#9333=DIRECTION ( 'NONE',  ( -1.000000000000000000, 0.000000000000000000, 0.000000000000000000 ) ) ;
#9334=DIRECTION ( 'NONE',  ( 0.000000000000000000, -0.01356324068817998940, 0.9999080150203990547 ) ) ;
#9335=CARTESIAN_POINT ( 'NONE',  ( 47.00000000000000711, 4.705694406421931860E-17, -3.469127814946512892E-15 ) ) ;
#9336=AXIS2_PLACEMENT_3D ( 'NONE', #54810, #30495, #55115 ) ;
#9337=ADVANCED_FACE ( 'NONE', ( #38700 ), #48682, .T. ) ;
#9338=ORIENTED_EDGE ( 'NONE', *, *, #40363, .T. ) ;
#9339=DIRECTION ( 'NONE',  ( 1.000000000000000000, 0.000000000000000000, 0.000000000000000000 ) ) ;
#9340=AXIS2_PLACEMENT_3D ( 'NONE', #24985, #24311, #64227 ) ;
#9344=ADVANCED_FACE ( 'NONE', ( #53345 ), #8434, .T. ) ;
#9345=DIRECTION ( 'NONE',  ( 0.000000000000000000, 0.9467777615094582488, 0.3218879778915939571 ) ) ;
#9346=FACE_OUTER_BOUND ( 'NONE', #42395, .T. ) ;
#9347=AXIS2_PLACEMENT_3D ( 'NONE', #4845, #30419, #45710 ) ;
#9348=CARTESIAN_POINT ( 'NONE',  ( -35.00000000000000000, 9.506317355798367785, 8.496612874013193206 ) ) ;
#9349=EDGE_CURVE ( 'NONE', #57134, #30777, #17090, .T. ) ;
#9350=VERTEX_POINT ( 'NONE', #53990 ) ;
#9352=CIRCLE ( 'NONE', #19968, 12.74999999999999822 ) ;
#9353=ORIENTED_EDGE ( 'NONE', *, *, #14028, .F. ) ;
#9355=CARTESIAN_POINT ( 'NONE',  ( -27.01437459610461644, 11.79277645698183363, -2.220455681983952267 ) ) ;
#9356=EDGE_CURVE ( 'NONE', #38593, #37413, #54271, .T. ) ;
#9357=ORIENTED_EDGE ( 'NONE', *, *, #25393, .T. ) ;
#9358=DIRECTION ( 'NONE',  ( 0.000000000000000000, 0.8009703041134188517, 0.5987040770935649903 ) ) ;
#9359=CARTESIAN_POINT ( 'NONE',  ( 3.347841273039249721, -10.61118957148187825, -8.345816669330458737 ) ) ;
#9361=FACE_OUTER_BOUND ( 'NONE', #30196, .T. ) ;
#9362=ORIENTED_EDGE ( 'NONE', *, *, #63970, .T. ) ;
#9363=DIRECTION ( 'NONE',  ( 0.000000000000000000, 0.5243256840888563808, 0.8515178078024868702 ) ) ;
#9364=EDGE_CURVE ( 'NONE', #21416, #12178, #49021, .T. ) ;
#9366=DIRECTION ( 'NONE',  ( -1.000000000000000000, 0.000000000000000000, 0.000000000000000000 ) ) ;
#9367=LINE ( 'NONE', #29992, #48967 ) ;
#9368=ORIENTED_EDGE ( 'NONE', *, *, #62318, .F. ) ;
#9369=CARTESIAN_POINT ( 'NONE',  ( 35.00000000000000000, 9.896810808925392777, -7.110831038798317572 ) ) ;
#9374=CARTESIAN_POINT ( 'NONE',  ( 11.72287332632499179, -11.90030359961621009, -1.578241357430486769 ) ) ;
#9375=LINE ( 'NONE', #49007, #11734 ) ;
#9377=AXIS2_PLACEMENT_3D ( 'NONE', #64144, #58516, #39515 ) ;
#9379=CARTESIAN_POINT ( 'NONE',  ( -5.388163386660410836, -1.427464897260812160, -13.42432405772846238 ) ) ;
#9380=CARTESIAN_POINT ( 'NONE',  ( -35.00000000000000000, -12.12087942037210553, 1.262958560998716617 ) ) ;
#9381=CARTESIAN_POINT ( 'NONE',  ( 35.00000000000000000, -11.95840593935202811, -2.346765782874394635 ) ) ;
#9382=ORIENTED_EDGE ( 'NONE', *, *, #35425, .F. ) ;
#9384=VERTEX_POINT ( 'NONE', #3479 ) ;
#9385=DIRECTION ( 'NONE',  ( 0.000000000000000000, -0.7381862504171877726, 0.6745969609292743474 ) ) ;
#9386=ORIENTED_EDGE ( 'NONE', *, *, #916, .T. ) ;
#9387=APPLICATION_CONTEXT ( 'automotive_design' ) ;
#9388=ORIENTED_EDGE ( 'NONE', *, *, #23337, .F. ) ;
#9390=DIRECTION ( 'NONE',  ( 0.000000000000000000, -0.01356324068817998940, 0.9999080150203990547 ) ) ;
#9391=CARTESIAN_POINT ( 'NONE',  ( -35.00000000000000000, -4.603882218679629545, 10.80631716521665453 ) ) ;
#9393=DIRECTION ( 'NONE',  ( -1.000000000000000000, 0.000000000000000000, 0.000000000000000000 ) ) ;
#9394=AXIS2_PLACEMENT_3D ( 'NONE', #28149, #17838, #33465 ) ;
#9397=AXIS2_PLACEMENT_3D ( 'NONE', #44930, #49927, #23687 ) ;
#9398=ORIENTED_EDGE ( 'NONE', *, *, #25913, .F. ) ;
#9399=CARTESIAN_POINT ( 'NONE',  ( -4.989057617119008192, -0.9162120371760335003, -13.46887357958837406 ) ) ;
#9400=CARTESIAN_POINT ( 'NONE',  ( -35.00000000000000000, 0.000000000000000000, 0.000000000000000000 ) ) ;
#9401=AXIS2_PLACEMENT_3D ( 'NONE', #6390, #26661, #46956 ) ;
#9403=VERTEX_POINT ( 'NONE', #13413 ) ;
#9405=EDGE_CURVE ( 'NONE', #36570, #5549, #62733, .T. ) ;
#9406=CARTESIAN_POINT ( 'NONE',  ( -7.358538974955358469, -1.423543355122588672, 13.42505237639485038 ) ) ;
#9409=VERTEX_POINT ( 'NONE', #63294 ) ;
#9412=CARTESIAN_POINT ( 'NONE',  ( 35.00000000000000000, 0.01609748574445066943, -11.74614673114903773 ) ) ;
#9413=VECTOR ( 'NONE', #48426, 1000.000000000000000 ) ;
#9414=EDGE_CURVE ( 'NONE', #8078, #42463, #12748, .T. ) ;
#9415=CYLINDRICAL_SURFACE ( 'NONE', #20358, 4.999999999999999112 ) ;
#9416=DIRECTION ( 'NONE',  ( 0.000000000000000000, 0.8169148498130256453, -0.5767582926624997830 ) ) ;
#9418=VECTOR ( 'NONE', #33697, 1000.000000000000000 ) ;
#9419=ADVANCED_FACE ( 'NONE', ( #38020 ), #44016, .T. ) ;
#9421=CARTESIAN_POINT ( 'NONE',  ( -7.904491797223720972, -5.813757704850941899, -10.52499957321815138 ) ) ;
#9422=CARTESIAN_POINT ( 'NONE',  ( -35.00000000000000000, -7.215058775251326217, 9.821084925794544063 ) ) ;
#9424=DIRECTION ( 'NONE',  ( 1.000000000000000000, 0.000000000000000000, 0.000000000000000000 ) ) ;
#9425=DIRECTION ( 'NONE',  ( 0.000000000000000000, -0.01356324068817998940, 0.9999080150203990547 ) ) ;
#9427=ORIENTED_EDGE ( 'NONE', *, *, #17776, .T. ) ;
#9428=VERTEX_POINT ( 'NONE', #48370 ) ;
#9430=DIRECTION ( 'NONE',  ( -1.000000000000000000, 0.000000000000000000, 0.000000000000000000 ) ) ;
#9431=AXIS2_PLACEMENT_3D ( 'NONE', #52028, #46380, #16458 ) ;
#9432=CIRCLE ( 'NONE', #55113, 12.74999999999999822 ) ;
#9433=ORIENTED_EDGE ( 'NONE', *, *, #63099, .F. ) ;
#9435=CARTESIAN_POINT ( 'NONE',  ( -35.00000000000000000, 0.000000000000000000, 0.000000000000000000 ) ) ;
#9436=VECTOR ( 'NONE', #22956, 1000.000000000000000 ) ;
#9442=CARTESIAN_POINT ( 'NONE',  ( -35.00000000000000000, 7.146664589318047156, -9.321877890560362090 ) ) ;
#9444=CARTESIAN_POINT ( 'NONE',  ( 22.57855258442564761, -4.427776684447072952, 11.15324139578564910 ) ) ;
#9445=ADVANCED_FACE ( 'NONE', ( #3808 ), #58676, .T. ) ;
#9446=ORIENTED_EDGE ( 'NONE', *, *, #54269, .F. ) ;
#9447=CARTESIAN_POINT ( 'NONE',  ( 37.00000000000000711, 4.705694406421931860E-17, -3.469127814946512892E-15 ) ) ;
#9450=VERTEX_POINT ( 'NONE', #50333 ) ;
#9451=CARTESIAN_POINT ( 'NONE',  ( 37.00000000000000711, -2.936739658819788712, 11.37311665002366290 ) ) ;
#9452=EDGE_CURVE ( 'NONE', #56769, #51818, #29692, .T. ) ;
#9454=CARTESIAN_POINT ( 'NONE',  ( -35.00000000000000000, 0.000000000000000000, 0.000000000000000000 ) ) ;
#9455=FACE_OUTER_BOUND ( 'NONE', #35131, .T. ) ;
#9456=LINE ( 'NONE', #8830, #61093 ) ;
#9457=CARTESIAN_POINT ( 'NONE',  ( 37.00000000000000711, 10.49626516989280844, 7.238157050195514586 ) ) ;
#9460=VERTEX_POINT ( 'NONE', #19737 ) ;
#9461=CARTESIAN_POINT ( 'NONE',  ( 22.88594695219327235, -4.822122601967141264, 25.00000000000000000 ) ) ;
#9462=ORIENTED_EDGE ( 'NONE', *, *, #9270, .F. ) ;
#9463=EDGE_CURVE ( 'NONE', #57334, #63621, #24716, .T. ) ;
#9464=ORIENTED_EDGE ( 'NONE', *, *, #14322, .T. ) ;
#9466=CARTESIAN_POINT ( 'NONE',  ( -35.00000000000000000, 12.66641127287625856, 1.457575200925591341 ) ) ;
#9471=CARTESIAN_POINT ( 'NONE',  ( 28.01964047808447944, -12.64055115429361820, 4.742990486147117046 ) ) ;
#9474=DIRECTION ( 'NONE',  ( 0.000000000000000000, 0.6943713148249588407, -0.7196168960969843154 ) ) ;
#9475=CARTESIAN_POINT ( 'NONE',  ( 37.00000000000000711, -10.84030624090611283, -6.711949091238110121 ) ) ;
#9479=EDGE_CURVE ( 'NONE', #50460, #13265, #62019, .T. ) ;
#9480=DIRECTION ( 'NONE',  ( 1.000000000000000000, 0.000000000000000000, 0.000000000000000000 ) ) ;
#9481=CARTESIAN_POINT ( 'NONE',  ( -37.00000000000000711, -11.68758509253249223, 1.171570255487406786 ) ) ;
#9482=AXIS2_PLACEMENT_3D ( 'NONE', #22874, #62116, #1615 ) ;
#9484=CARTESIAN_POINT ( 'NONE',  ( -10.78957422984094983, -6.332470062474154560, -10.19518144049010644 ) ) ;
#9486=DIRECTION ( 'NONE',  ( 1.000000000000000000, 0.000000000000000000, 0.000000000000000000 ) ) ;
#9487=DIRECTION ( 'NONE',  ( 0.000000000000000000, 0.01356324068817998940, -0.9999080150203990547 ) ) ;
#9488=VERTEX_POINT ( 'NONE', #15386 ) ;
#9491=EDGE_CURVE ( 'NONE', #34871, #50610, #51458, .T. ) ;
#9493=VECTOR ( 'NONE', #36971, 1000.000000000000000 ) ;
#9494=ADVANCED_FACE ( 'NONE', ( #14393 ), #60948, .T. ) ;
#9497=ORIENTED_EDGE ( 'NONE', *, *, #62843, .F. ) ;
#9498=CYLINDRICAL_SURFACE ( 'NONE', #21657, 4.999999999999999112 ) ;
#9499=DIRECTION ( 'NONE',  ( 1.000000000000000000, 0.000000000000000000, -0.000000000000000000 ) ) ;
#9503=DIRECTION ( 'NONE',  ( -0.000000000000000000, -1.000000000000000000, -0.000000000000000000 ) ) ;
#9506=CARTESIAN_POINT ( 'NONE',  ( -35.00000000000000000, -9.430788938294105250, 7.718225330433773124 ) ) ;
#9507=CARTESIAN_POINT ( 'NONE',  ( -14.17299601508879014, 8.097942500480233008, 8.858180248946752045 ) ) ;
#9510=CARTESIAN_POINT ( 'NONE',  ( 35.00000000000000000, -2.220215194441986561, -11.98254675519227597 ) ) ;
#9511=EDGE_LOOP ( 'NONE', ( #5793, #9386, #33307, #14343 ) ) ;
#9512=FACE_OUTER_BOUND ( 'NONE', #23739, .T. ) ;
#9514=CARTESIAN_POINT ( 'NONE',  ( -18.12134786527529684, 6.862502072565634492, -11.62855658186334651 ) ) ;
#9515=DIRECTION ( 'NONE',  ( 0.000000000000000000, 0.01356324068818000848, -0.9999080150203990547 ) ) ;
#9518=DIRECTION ( 'NONE',  ( -1.000000000000000000, 0.000000000000000000, -0.000000000000000000 ) ) ;
#9521=ORIENTED_EDGE ( 'NONE', *, *, #65428, .F. ) ;
#9522=CARTESIAN_POINT ( 'NONE',  ( -2.952869152607106251, 11.39722960915212724, 3.755417052241485365 ) ) ;
#9523=ORIENTED_EDGE ( 'NONE', *, *, #39144, .F. ) ;
#9528=CARTESIAN_POINT ( 'NONE',  ( -37.00000000000000711, 4.986700593229701717, 10.63508530065523772 ) ) ;
#9530=DIRECTION ( 'NONE',  ( 1.000000000000000000, 0.000000000000000000, 0.000000000000000000 ) ) ;
#9531=DIRECTION ( 'NONE',  ( 1.000000000000000000, 0.000000000000000000, 0.000000000000000000 ) ) ;
#9532=CARTESIAN_POINT ( 'NONE',  ( 22.88594695219327235, 3.421158645304719137, 13.05931366970166962 ) ) ;
#9537=ORIENTED_EDGE ( 'NONE', *, *, #17377, .T. ) ;
#9540=ORIENTED_EDGE ( 'NONE', *, *, #20063, .F. ) ;
#9542=DIRECTION ( 'NONE',  ( 0.000000000000000000, -0.01356324068817991828, 0.9999080150203990547 ) ) ;
#9547=DIRECTION ( 'NONE',  ( -1.000000000000000000, 0.000000000000000000, 0.000000000000000000 ) ) ;
#9548=DIRECTION ( 'NONE',  ( 0.000000000000000000, 0.01356324068817998940, -0.9999080150203989437 ) ) ;
#9550=CARTESIAN_POINT ( 'NONE',  ( 12.91288097661053236, 12.55977324591722954, -4.965784564771029252 ) ) ;
#9551=CARTESIAN_POINT ( 'NONE',  ( 22.57855258442565116, 3.026812727784649493, 13.15630665159948975 ) ) ;
#9552=CARTESIAN_POINT ( 'NONE',  ( -35.00000000000000000, -10.14433819232429812, -6.753013023069823539 ) ) ;
#9554=DIRECTION ( 'NONE',  ( -1.000000000000000000, 0.000000000000000000, 0.000000000000000000 ) ) ;
#9555=AXIS2_PLACEMENT_3D ( 'NONE', #4639, #55148, #54837 ) ;
#9558=EDGE_LOOP ( 'NONE', ( #64335, #39643, #41692, #86 ) ) ;
#9561=ADVANCED_FACE ( 'NONE', ( #16379 ), #36650, .T. ) ;
#9564=CARTESIAN_POINT ( 'NONE',  ( -37.00000000000000711, -6.303578524886872536, -10.42955799785326576 ) ) ;
#9565=CYLINDRICAL_SURFACE ( 'NONE', #5937, 12.18649999999999878 ) ;
#9569=CARTESIAN_POINT ( 'NONE',  ( -11.20050441550567299, -9.175587222235860096, -9.916315835339821305 ) ) ;
#9572=CARTESIAN_POINT ( 'NONE',  ( 11.32539125054619689, 0.8069478436655108666, 11.97338806366722785 ) ) ;
#9575=AXIS2_PLACEMENT_3D ( 'NONE', #21136, #21486, #41755 ) ;
#9576=DIRECTION ( 'NONE',  ( 1.000000000000000000, 0.000000000000000000, 0.000000000000000000 ) ) ;
#9577=EDGE_LOOP ( 'NONE', ( #12412, #21475, #45405, #1881 ) ) ;
#9582=ADVANCED_FACE ( 'NONE', ( #21701 ), #26030, .T. ) ;
#9583=EDGE_CURVE ( 'NONE', #38770, #58222, #50358, .T. ) ;
#9584=CIRCLE ( 'NONE', #6434, 12.18650000000000055 ) ;
#9585=CARTESIAN_POINT ( 'NONE',  ( -30.18541646480307250, -1.416020129149132334, 25.00000000000000000 ) ) ;
#9586=EDGE_CURVE ( 'NONE', #35395, #64071, #22320, .T. ) ;
#9588=ORIENTED_EDGE ( 'NONE', *, *, #13841, .F. ) ;
#9589=ORIENTED_EDGE ( 'NONE', *, *, #36386, .T. ) ;
#9591=ORIENTED_EDGE ( 'NONE', *, *, #59929, .F. ) ;
#9592=VECTOR ( 'NONE', #14049, 1000.000000000000000 ) ;
#9594=DIRECTION ( 'NONE',  ( -1.000000000000000000, 0.000000000000000000, 0.000000000000000000 ) ) ;
#9595=CARTESIAN_POINT ( 'NONE',  ( 35.00000000000000000, -9.493370459201747380, -6.917234959366797220 ) ) ;
#9597=CYLINDRICAL_SURFACE ( 'NONE', #2488, 12.18649999999999878 ) ;
#9598=DIRECTION ( 'NONE',  ( 1.000000000000000000, 0.000000000000000000, 0.000000000000000000 ) ) ;
#9599=FACE_OUTER_BOUND ( 'NONE', #60697, .T. ) ;
#9601=CIRCLE ( 'NONE', #62719, 12.18650000000000055 ) ;
#9603=ORIENTED_EDGE ( 'NONE', *, *, #62214, .F. ) ;
#9605=CARTESIAN_POINT ( 'NONE',  ( -35.00000000000000000, -10.14408668126209001, -5.921969905510467314 ) ) ;
#9606=EDGE_CURVE ( 'NONE', #23040, #44827, #20638, .T. ) ;
#9609=AXIS2_PLACEMENT_3D ( 'NONE', #65111, #38880, #50500 ) ;
#9610=VECTOR ( 'NONE', #20082, 1000.000000000000000 ) ;
#9611=ORIENTED_EDGE ( 'NONE', *, *, #12857, .T. ) ;
#9612=ADVANCED_FACE ( 'NONE', ( #41956 ), #47612, .T. ) ;
#9613=CARTESIAN_POINT ( 'NONE',  ( 35.00000000000000000, 7.499679039484058229, -9.040300684349723781 ) ) ;
#9614=VERTEX_POINT ( 'NONE', #26667 ) ;
#9616=CARTESIAN_POINT ( 'NONE',  ( 6.471884597807777695, -7.981883161988641895, -10.89336526951398021 ) ) ;
#9618=CARTESIAN_POINT ( 'NONE',  ( 3.459614771489464946, -11.09853614738469396, 4.563167253695070258 ) ) ;
#9619=ORIENTED_EDGE ( 'NONE', *, *, #57917, .F. ) ;
#9621=CYLINDRICAL_SURFACE ( 'NONE', #40548, 5.000000000000000888 ) ;
#9622=VERTEX_POINT ( 'NONE', #17013 ) ;
#9623=DIRECTION ( 'NONE',  ( 1.000000000000000000, 0.000000000000000000, 0.000000000000000000 ) ) ;
#9624=ORIENTED_EDGE ( 'NONE', *, *, #37993, .F. ) ;
#9626=VERTEX_POINT ( 'NONE', #11691 ) ;
#9628=FACE_OUTER_BOUND ( 'NONE', #18801, .T. ) ;
#9630=DIRECTION ( 'NONE',  ( 0.000000000000000000, 0.04924826701374583615, 0.9987865678893277366 ) ) ;
#9632=ORIENTED_EDGE ( 'NONE', *, *, #16595, .F. ) ;
#9633=EDGE_CURVE ( 'NONE', #62352, #9772, #18525, .T. ) ;
#9634=AXIS2_PLACEMENT_3D ( 'NONE', #7531, #54079, #23837 ) ;
#9635=CARTESIAN_POINT ( 'NONE',  ( -37.00000000000000711, 8.029056188533687077, 8.573591947375351907 ) ) ;
#9636=CIRCLE ( 'NONE', #31938, 5.000000000000000888 ) ;
#9637=EDGE_LOOP ( 'NONE', ( #36231, #1011, #64663, #9943 ) ) ;
#9640=VECTOR ( 'NONE', #20546, 1000.000000000000000 ) ;
#9644=AXIS2_PLACEMENT_3D ( 'NONE', #32216, #49181, #38521 ) ;
#9648=CIRCLE ( 'NONE', #55320, 12.75000000000000178 ) ;
#9649=EDGE_CURVE ( 'NONE', #47974, #4279, #19545, .T. ) ;
#9650=ORIENTED_EDGE ( 'NONE', *, *, #39691, .T. ) ;
#9651=CARTESIAN_POINT ( 'NONE',  ( -24.38812357031636679, -11.02047918387278180, 7.799809501265555056 ) ) ;
#9652=DIRECTION ( 'NONE',  ( 1.000000000000000000, -0.000000000000000000, 0.000000000000000000 ) ) ;
#9654=CYLINDRICAL_SURFACE ( 'NONE', #3312, 12.75000000000000178 ) ;
#9655=AXIS2_PLACEMENT_3D ( 'NONE', #3170, #64319, #63648 ) ;
#9656=CARTESIAN_POINT ( 'NONE',  ( 35.00000000000000000, 4.705694406421931860E-17, -3.469127814946512892E-15 ) ) ;
#9658=CARTESIAN_POINT ( 'NONE',  ( 36.00000000000000711, -6.415447294506781084, -11.01837265713071368 ) ) ;
#9661=DIRECTION ( 'NONE',  ( 0.000000000000000000, 0.1118654143051617117, 0.9937233664769761221 ) ) ;
#9662=CIRCLE ( 'NONE', #10715, 5.000000000000001776 ) ;
#9663=VECTOR ( 'NONE', #27024, 1000.000000000000000 ) ;
#9666=CARTESIAN_POINT ( 'NONE',  ( 37.00000000000000711, 4.705694406421931860E-17, -3.469127814946512892E-15 ) ) ;
#9668=CARTESIAN_POINT ( 'NONE',  ( 3.291290029914074378, 8.250315036047103590, -8.713914264323182834 ) ) ;
#9669=CARTESIAN_POINT ( 'NONE',  ( 37.00000000000000711, 9.348667969174517367, 7.817492529713752525 ) ) ;
#9672=DIRECTION ( 'NONE',  ( 0.000000000000000000, 0.01356324068817998593, -0.9999080150203990547 ) ) ;
#9673=EDGE_CURVE ( 'NONE', #22062, #55015, #56773, .T. ) ;
#9674=EDGE_CURVE ( 'NONE', #37639, #20061, #15690, .T. ) ;
#9676=EDGE_LOOP ( 'NONE', ( #24662, #64001, #30634, #61066 ) ) ;
#9677=CARTESIAN_POINT ( 'NONE',  ( 11.95035458199039624, -11.72822567559551743, -2.544750170429570080 ) ) ;
#9678=CIRCLE ( 'NONE', #31937, 4.999999999999999112 ) ;
#9679=AXIS2_PLACEMENT_3D ( 'NONE', #43323, #13716, #38998 ) ;
#9681=VERTEX_POINT ( 'NONE', #61919 ) ;
#9682=CARTESIAN_POINT ( 'NONE',  ( -37.00000000000000711, 12.70128625845194392, -1.113475361586356627 ) ) ;
#9683=DIRECTION ( 'NONE',  ( -1.000000000000000000, 0.000000000000000000, 0.000000000000000000 ) ) ;
#9684=CARTESIAN_POINT ( 'NONE',  ( -35.00000000000000000, 1.591260454995410578, -12.08216339958899077 ) ) ;
#9688=ORIENTED_EDGE ( 'NONE', *, *, #34802, .F. ) ;
#9690=CARTESIAN_POINT ( 'NONE',  ( 29.18521670982013916, -10.00068734037119178, 6.636238164281968999 ) ) ;
#9693=ORIENTED_EDGE ( 'NONE', *, *, #4193, .T. ) ;
#9694=DIRECTION ( 'NONE',  ( 1.000000000000000000, 0.000000000000000000, 0.000000000000000000 ) ) ;
#9695=CARTESIAN_POINT ( 'NONE',  ( 35.00000000000000000, 5.921969905510355403, -10.14408668126215929 ) ) ;
#9696=VECTOR ( 'NONE', #31165, 1000.000000000000000 ) ;
#9699=DIRECTION ( 'NONE',  ( 0.000000000000000000, -0.1387779952735679057, 0.9903235168508568442 ) ) ;
#9702=DIRECTION ( 'NONE',  ( 0.000000000000000000, -0.4935949184179322380, 0.8696919319575150409 ) ) ;
#9704=ORIENTED_EDGE ( 'NONE', *, *, #63157, .F. ) ;
#9705=AXIS2_PLACEMENT_3D ( 'NONE', #33673, #44609, #64899 ) ;
#9707=ORIENTED_EDGE ( 'NONE', *, *, #5209, .F. ) ;
#9710=CARTESIAN_POINT ( 'NONE',  ( -37.00000000000000711, 0.000000000000000000, 0.000000000000000000 ) ) ;
#9714=EDGE_CURVE ( 'NONE', #24950, #33918, #27641, .T. ) ;
#9715=CARTESIAN_POINT ( 'NONE',  ( -26.75616027029648691, -10.79764998130141151, 5.236257343771399064 ) ) ;
#9716=AXIS2_PLACEMENT_3D ( 'NONE', #46995, #1453, #27667 ) ;
#9719=DIRECTION ( 'NONE',  ( 1.000000000000000000, -0.000000000000000000, 0.000000000000000000 ) ) ;
#9720=DIRECTION ( 'NONE',  ( 1.000000000000000000, 0.000000000000000000, -0.000000000000000000 ) ) ;
#9721=CARTESIAN_POINT ( 'NONE',  ( 37.00000000000000711, 4.705694406421931860E-17, -3.469127814946512892E-15 ) ) ;
#9724=ORIENTED_EDGE ( 'NONE', *, *, #16703, .T. ) ;
#9725=CARTESIAN_POINT ( 'NONE',  ( 13.12628618392431079, -11.60359632220612092, -6.913481910311843670 ) ) ;
#9727=ORIENTED_EDGE ( 'NONE', *, *, #41227, .F. ) ;
#9728=LINE ( 'NONE', #46311, #35961 ) ;
#9729=DIRECTION ( 'NONE',  ( 1.000000000000000000, -0.000000000000000000, 0.000000000000000000 ) ) ;
#9731=DIRECTION ( 'NONE',  ( 1.000000000000000000, -0.000000000000000000, 0.000000000000000000 ) ) ;
#9733=CIRCLE ( 'NONE', #2354, 12.18649999999999700 ) ;
#9734=DIRECTION ( 'NONE',  ( 0.000000000000000000, 0.9467777615094560284, 0.3218879778916007850 ) ) ;
#9735=DIRECTION ( 'NONE',  ( 0.000000000000000000, 0.01356324068817992001, -0.9999080150203990547 ) ) ;
#9736=CIRCLE ( 'NONE', #57517, 12.74999999999999822 ) ;
#9741=FACE_OUTER_BOUND ( 'NONE', #24996, .T. ) ;
#9747=EDGE_CURVE ( 'NONE', #33435, #21760, #59235, .T. ) ;
#9750=DIRECTION ( 'NONE',  ( 1.000000000000000000, 0.000000000000000000, 0.000000000000000000 ) ) ;
#9751=CARTESIAN_POINT ( 'NONE',  ( -27.01437459610461644, 11.79277645698183363, -2.220455681983952267 ) ) ;
#9752=ORIENTED_EDGE ( 'NONE', *, *, #37390, .F. ) ;
#9755=CARTESIAN_POINT ( 'NONE',  ( 35.00000000000000000, -11.98254675519226531, 2.220215194442026974 ) ) ;
#9756=DIRECTION ( 'NONE',  ( 0.000000000000000000, 0.01356324068817992175, -0.9999080150203990547 ) ) ;
#9757=CIRCLE ( 'NONE', #36295, 5.000000000000000888 ) ;
#9758=CIRCLE ( 'NONE', #46946, 5.000000000000000000 ) ;
#9760=DIRECTION ( 'NONE',  ( 1.000000000000000000, 0.000000000000000000, -0.000000000000000000 ) ) ;
#9762=ORIENTED_EDGE ( 'NONE', *, *, #47322, .T. ) ;
#9768=CARTESIAN_POINT ( 'NONE',  ( 8.460390590667396182, 3.946828837481929586, 12.91309979171136213 ) ) ;
#9769=CARTESIAN_POINT ( 'NONE',  ( -35.00000000000000000, 0.000000000000000000, 0.000000000000000000 ) ) ;
#9770=VERTEX_POINT ( 'NONE', #55555 ) ;
#9772=VERTEX_POINT ( 'NONE', #24297 ) ;
#9773=ORIENTED_EDGE ( 'NONE', *, *, #11391, .T. ) ;
#9774=AXIS2_PLACEMENT_3D ( 'NONE', #13723, #39663, #19398 ) ;
#9775=AXIS2_PLACEMENT_3D ( 'NONE', #20968, #60554, #39 ) ;
#9777=CARTESIAN_POINT ( 'NONE',  ( 35.00000000000000000, 4.705694406421931860E-17, -3.469127814946512892E-15 ) ) ;
#9778=DIRECTION ( 'NONE',  ( 1.000000000000000000, 0.000000000000000000, 0.000000000000000000 ) ) ;
#9779=CARTESIAN_POINT ( 'NONE',  ( -47.00000000000000711, 0.000000000000000000, 0.000000000000000000 ) ) ;
#9780=CARTESIAN_POINT ( 'NONE',  ( 24.82652845881425208, -10.42385221765392700, -8.578654028722157321 ) ) ;
#9781=CIRCLE ( 'NONE', #23575, 12.74999999999999822 ) ;
#9783=CARTESIAN_POINT ( 'NONE',  ( 24.52118107989806006, -2.661457398423999532, -13.23640138053051984 ) ) ;
#9784=CARTESIAN_POINT ( 'NONE',  ( -35.00000000000000000, 5.246972444134173408, -10.99909370905151995 ) ) ;
#9786=DIRECTION ( 'NONE',  ( 0.000000000000000000, -1.000000000000000000, 0.000000000000000000 ) ) ;
#9787=ORIENTED_EDGE ( 'NONE', *, *, #11728, .T. ) ;
#9790=ORIENTED_EDGE ( 'NONE', *, *, #58602, .F. ) ;
#9793=DIRECTION ( 'NONE',  ( -1.000000000000000000, -0.000000000000000000, 0.000000000000000000 ) ) ;
#9794=EDGE_CURVE ( 'NONE', #64905, #18784, #44251, .T. ) ;
#9798=DIRECTION ( 'NONE',  ( -0.000000000000000000, -0.000000000000000000, -1.000000000000000000 ) ) ;
#9799=ORIENTED_EDGE ( 'NONE', *, *, #38434, .F. ) ;
#9800=VECTOR ( 'NONE', #42106, 1000.000000000000000 ) ;
#9801=ORIENTED_EDGE ( 'NONE', *, *, #13034, .T. ) ;
#9804=ORIENTED_EDGE ( 'NONE', *, *, #25382, .T. ) ;
#9806=DIRECTION ( 'NONE',  ( 0.000000000000000000, 0.01356324068817998940, -0.9999080150203989437 ) ) ;
#9809=CARTESIAN_POINT ( 'NONE',  ( -11.14133641294997901, -5.663661283019989057, -10.58164429124088457 ) ) ;
#9812=DIRECTION ( 'NONE',  ( 0.000000000000000000, -0.6478160128811839558, 0.7617968321374969376 ) ) ;
#9816=EDGE_CURVE ( 'NONE', #18660, #28337, #7875, .T. ) ;
#9819=DIRECTION ( 'NONE',  ( 0.000000000000000000, -0.01356324068817999114, 0.9999080150203989437 ) ) ;
#9820=AXIS2_PLACEMENT_3D ( 'NONE', #27596, #47260, #31923 ) ;
#9821=LINE ( 'NONE', #30114, #46195 ) ;
#9822=DIRECTION ( 'NONE',  ( 0.000000000000000000, -0.2960891610144577579, -0.9551603052523459647 ) ) ;
#9824=AXIS2_PLACEMENT_3D ( 'NONE', #46931, #1392, #61232 ) ;
#9826=ADVANCED_FACE ( 'NONE', ( #50890 ), #14958, .T. ) ;
#9827=DIRECTION ( 'NONE',  ( 0.000000000000000000, 0.01356324068817991828, -0.9999080150203990547 ) ) ;
#9828=AXIS2_PLACEMENT_3D ( 'NONE', #585, #56781, #22152 ) ;
#9829=DIRECTION ( 'NONE',  ( -0.000000000000000000, -1.000000000000000000, -0.000000000000000000 ) ) ;
#9831=DIRECTION ( 'NONE',  ( 0.000000000000000000, 0.01356324068817992175, -0.9999080150203990547 ) ) ;
#9832=CARTESIAN_POINT ( 'NONE',  ( 37.00000000000000711, 6.584150480049550502, -10.25474254703955701 ) ) ;
#9834=EDGE_CURVE ( 'NONE', #57839, #23170, #54634, .T. ) ;
#9836=CYLINDRICAL_SURFACE ( 'NONE', #25630, 5.000000000000000888 ) ;
#9837=AXIS2_PLACEMENT_3D ( 'NONE', #21410, #46356, #21754 ) ;
#9845=VERTEX_POINT ( 'NONE', #30277 ) ;
#9846=CYLINDRICAL_SURFACE ( 'NONE', #31278, 12.18650000000000055 ) ;
#9847=CARTESIAN_POINT ( 'NONE',  ( -28.24248022282097992, -12.24705570707973301, -5.688045095021857733 ) ) ;
#9849=VECTOR ( 'NONE', #51001, 1000.000000000000000 ) ;
#9850=AXIS2_PLACEMENT_3D ( 'NONE', #3620, #44149, #64413 ) ;
#9851=FACE_OUTER_BOUND ( 'NONE', #931, .T. ) ;
#9852=ORIENTED_EDGE ( 'NONE', *, *, #64314, .F. ) ;
#9854=AXIS2_PLACEMENT_3D ( 'NONE', #33789, #13201, #47794 ) ;
#9855=AXIS2_PLACEMENT_3D ( 'NONE', #715, #5046, #55592 ) ;
#9857=ORIENTED_EDGE ( 'NONE', *, *, #30315, .F. ) ;
#9858=DIRECTION ( 'NONE',  ( -1.000000000000000000, -0.000000000000000000, 0.000000000000000000 ) ) ;
#9860=FACE_OUTER_BOUND ( 'NONE', #3992, .T. ) ;
#9863=CIRCLE ( 'NONE', #29154, 12.74999999999999822 ) ;
#9864=DIRECTION ( 'NONE',  ( 1.000000000000000000, 0.000000000000000000, 0.000000000000000000 ) ) ;
#9865=DIRECTION ( 'NONE',  ( 0.000000000000000000, 0.01356324068817998940, -0.9999080150203990547 ) ) ;
#9866=ORIENTED_EDGE ( 'NONE', *, *, #19391, .T. ) ;
#9867=FACE_OUTER_BOUND ( 'NONE', #32684, .T. ) ;
#9868=CIRCLE ( 'NONE', #18394, 12.74999999999999822 ) ;
#9873=PLANE ( 'NONE',  #54278 ) ;
#9874=ORIENTED_EDGE ( 'NONE', *, *, #22706, .T. ) ;
#9876=CARTESIAN_POINT ( 'NONE',  ( 12.91052848813855469, 10.81303340823124692, -5.207629998415853834 ) ) ;
#9877=CARTESIAN_POINT ( 'NONE',  ( -37.00000000000000711, -12.17626345777664021, 0.4993900848166987760 ) ) ;
#9878=VERTEX_POINT ( 'NONE', #10310 ) ;
#9880=EDGE_LOOP ( 'NONE', ( #27692, #3938, #51083, #58335 ) ) ;
#9882=ADVANCED_FACE ( 'NONE', ( #16944 ), #11306, .T. ) ;
#9883=ORIENTED_EDGE ( 'NONE', *, *, #36721, .F. ) ;
#9884=CARTESIAN_POINT ( 'NONE',  ( 23.00432781815466754, -10.16387028742533793, -6.387888675388155413 ) ) ;
#9888=LINE ( 'NONE', #25185, #49035 ) ;
#9890=VECTOR ( 'NONE', #25133, 1000.000000000000000 ) ;
#9891=ADVANCED_FACE ( 'NONE', ( #51881 ), #32230, .T. ) ;
#9894=ORIENTED_EDGE ( 'NONE', *, *, #44484, .F. ) ;
#9895=( BOUNDED_CURVE ( )  B_SPLINE_CURVE ( 3, ( #6533, #6209, #26469, #47106 ),
 .UNSPECIFIED., .F., .F. ) 
 B_SPLINE_CURVE_WITH_KNOTS ( ( 4, 4 ),
 ( 1.289274629942205985, 1.297672015718555949 ),
 .UNSPECIFIED. ) 
 CURVE ( )  GEOMETRIC_REPRESENTATION_ITEM ( )  RATIONAL_B_SPLINE_CURVE ( ( 1.000000000000000000, 0.9999941236679763534, 0.9999941236679763534, 1.000000000000000000 ) ) 
 REPRESENTATION_ITEM ( '' )  );
#9898=CARTESIAN_POINT ( 'NONE',  ( 23.90871877840727322, 9.468420019444938163, -7.376992196490170350 ) ) ;
#9899=EDGE_CURVE ( 'NONE', #22914, #48293, #61502, .T. ) ;
#9900=LINE ( 'NONE', #55459, #63563 ) ;
#9901=AXIS2_PLACEMENT_3D ( 'NONE', #24667, #65223, #19692 ) ;
#9902=CARTESIAN_POINT ( 'NONE',  ( 35.00000000000000000, 12.16893194857555294, 3.805206332242343059 ) ) ;
#9903=LINE ( 'NONE', #56442, #45654 ) ;
#9906=VECTOR ( 'NONE', #52014, 1000.000000000000000 ) ;
#9907=DIRECTION ( 'NONE',  ( -1.000000000000000000, 0.000000000000000000, 0.000000000000000000 ) ) ;
#9908=VECTOR ( 'NONE', #41981, 1000.000000000000000 ) ;
#9909=AXIS2_PLACEMENT_3D ( 'NONE', #32262, #46919, #22966 ) ;
#9910=ORIENTED_EDGE ( 'NONE', *, *, #17573, .T. ) ;
#9912=VERTEX_POINT ( 'NONE', #57196 ) ;
#9914=CARTESIAN_POINT ( 'NONE',  ( 35.00000000000000000, 11.66953048682399441, -3.511814412392164186 ) ) ;
#9916=CARTESIAN_POINT ( 'NONE',  ( -18.06042000159870042, 5.592353769334478919, -12.28941745365187543 ) ) ;
#9917=AXIS2_PLACEMENT_3D ( 'NONE', #3065, #53608, #3401 ) ;
#9920=EDGE_CURVE ( 'NONE', #40631, #33417, #56819, .T. ) ;
#9921=VERTEX_POINT ( 'NONE', #42190 ) ;
#9924=DIRECTION ( 'NONE',  ( 1.000000000000000000, 0.000000000000000000, 0.000000000000000000 ) ) ;
#9925=DIRECTION ( 'NONE',  ( 1.000000000000000000, -0.000000000000000000, 0.000000000000000000 ) ) ;
#9928=AXIS2_PLACEMENT_3D ( 'NONE', #2859, #43382, #63659 ) ;
#9929=EDGE_CURVE ( 'NONE', #45204, #25848, #65284, .T. ) ;
#9930=CARTESIAN_POINT ( 'NONE',  ( -17.34047990058653710, -6.189094570992181410, 10.28225073071224038 ) ) ;
#9931=DIRECTION ( 'NONE',  ( 0.000000000000000000, 0.01356324068817998940, -0.9999080150203990547 ) ) ;
#9932=AXIS2_PLACEMENT_3D ( 'NONE', #37344, #10764, #32660 ) ;
#9933=ORIENTED_EDGE ( 'NONE', *, *, #56000, .T. ) ;
#9934=CIRCLE ( 'NONE', #57701, 5.000000000000000888 ) ;
#9939=CARTESIAN_POINT ( 'NONE',  ( -35.00000000000000000, -4.732539170486343316, 11.23004253107762906 ) ) ;
#9940=DIRECTION ( 'NONE',  ( 1.000000000000000000, 0.000000000000000000, 0.000000000000000000 ) ) ;
#9941=CARTESIAN_POINT ( 'NONE',  ( -37.00000000000000711, 3.614449339633491576, 11.17622378668007777 ) ) ;
#9943=ORIENTED_EDGE ( 'NONE', *, *, #5579, .T. ) ;
#9944=ORIENTED_EDGE ( 'NONE', *, *, #59979, .T. ) ;
#9945=CARTESIAN_POINT ( 'NONE',  ( 37.00000000000000711, -10.30098186818245409, 5.644643009979177783 ) ) ;
#9946=ORIENTED_EDGE ( 'NONE', *, *, #62965, .T. ) ;
#9947=DIRECTION ( 'NONE',  ( 0.000000000000000000, -0.01356324068817998940, 0.9999080150203990547 ) ) ;
#9951=CYLINDRICAL_SURFACE ( 'NONE', #4622, 4.999999999999997335 ) ;
#9952=CARTESIAN_POINT ( 'NONE',  ( -17.08907783926314394, 2.790822428529207144, 11.67174978956914266 ) ) ;
#9955=AXIS2_PLACEMENT_3D ( 'NONE', #17451, #43353, #47393 ) ;
#9956=AXIS2_PLACEMENT_3D ( 'NONE', #51295, #38172, #58485 ) ;
#9957=ORIENTED_EDGE ( 'NONE', *, *, #11098, .T. ) ;
#9959=AXIS2_PLACEMENT_3D ( 'NONE', #49765, #16488, #855 ) ;
#9961=ADVANCED_FACE ( 'NONE', ( #1004 ), #57527, .T. ) ;
#9962=VERTEX_POINT ( 'NONE', #31892 ) ;
#9964=CARTESIAN_POINT ( 'NONE',  ( -35.00000000000000000, 2.544412758416015219, -11.91791701451263741 ) ) ;
#9967=DIRECTION ( 'NONE',  ( 0.000000000000000000, -0.01356324068817992175, 0.9999080150203990547 ) ) ;
#9968=CARTESIAN_POINT ( 'NONE',  ( -35.00000000000000000, 0.000000000000000000, 0.000000000000000000 ) ) ;
#9969=CARTESIAN_POINT ( 'NONE',  ( 35.00000000000000000, -7.971186206369405447, 9.217970097227802029 ) ) ;
#9973=ORIENTED_EDGE ( 'NONE', *, *, #30239, .T. ) ;
#9974=DIRECTION ( 'NONE',  ( -1.000000000000000000, 0.000000000000000000, -0.000000000000000000 ) ) ;
#9975=ORIENTED_EDGE ( 'NONE', *, *, #65269, .T. ) ;
#9977=VERTEX_POINT ( 'NONE', #57862 ) ;
#9985=CARTESIAN_POINT ( 'NONE',  ( 37.00000000000000711, 8.235637554476776145, 9.733281772932070197 ) ) ;
#9986=CARTESIAN_POINT ( 'NONE',  ( 35.00000000000000000, -11.39945968423467448, 5.710938531231826154 ) ) ;
#9988=ORIENTED_EDGE ( 'NONE', *, *, #16472, .F. ) ;
#9990=ORIENTED_EDGE ( 'NONE', *, *, #32996, .F. ) ;
#9992=VECTOR ( 'NONE', #27815, 1000.000000000000000 ) ;
#9993=CYLINDRICAL_SURFACE ( 'NONE', #23541, 12.18649999999999878 ) ;
#9994=EDGE_CURVE ( 'NONE', #19210, #23964, #42968, .T. ) ;
#9995=ORIENTED_EDGE ( 'NONE', *, *, #28608, .F. ) ;
#9999=EDGE_CURVE ( 'NONE', #34871, #44514, #22253, .T. ) ;
#10000=AXIS2_PLACEMENT_3D ( 'NONE', #42591, #57265, #31643 ) ;
#10001=VERTEX_POINT ( 'NONE', #27567 ) ;
#10002=EDGE_LOOP ( 'NONE', ( #20809, #42729, #2761, #12568 ) ) ;
#10003=CARTESIAN_POINT ( 'NONE',  ( -24.46505758082295756, -9.480231875006323250, 9.613209244406563769 ) ) ;
#10004=DIRECTION ( 'NONE',  ( -0.7648446667472313942, 0.000000000000000000, 0.6442147435043042991 ) ) ;
#10008=ORIENTED_EDGE ( 'NONE', *, *, #468, .F. ) ;
#10009=CIRCLE ( 'NONE', #34394, 12.18649999999999878 ) ;
#10010=DIRECTION ( 'NONE',  ( 0.000000000000000000, 0.2618041379715563277, -0.9651210252299812220 ) ) ;
#10014=EDGE_CURVE ( 'NONE', #42153, #18413, #2, .T. ) ;
#10018=EDGE_CURVE ( 'NONE', #62900, #58284, #17932, .T. ) ;
#10022=CIRCLE ( 'NONE', #15333, 5.000000000000000888 ) ;
#10024=ADVANCED_FACE ( 'NONE', ( #17280 ), #28239, .T. ) ;
#10027=ORIENTED_EDGE ( 'NONE', *, *, #38765, .F. ) ;
#10028=CARTESIAN_POINT ( 'NONE',  ( -14.29135464769095520, 7.782112657557433089, -9.134479874907182051 ) ) ;
#10031=AXIS2_PLACEMENT_3D ( 'NONE', #16342, #26970, #5724 ) ;
#10033=VERTEX_POINT ( 'NONE', #38193 ) ;
#10034=ORIENTED_EDGE ( 'NONE', *, *, #51532, .F. ) ;
#10035=VERTEX_POINT ( 'NONE', #48855 ) ;
#10039=ORIENTED_EDGE ( 'NONE', *, *, #35088, .F. ) ;
#10040=CARTESIAN_POINT ( 'NONE',  ( 0.000000000000000000, 0.000000000000000000, 0.000000000000000000 ) ) ;
#10041=DIRECTION ( 'NONE',  ( 0.000000000000000000, -0.3218879778915842427, 0.9467777615094616905 ) ) ;
#10042=DIRECTION ( 'NONE',  ( -1.000000000000000000, -0.000000000000000000, 0.000000000000000000 ) ) ;
#10043=EDGE_CURVE ( 'NONE', #20774, #29997, #59986, .T. ) ;
#10044=VERTEX_POINT ( 'NONE', #27249 ) ;
#10047=DIRECTION ( 'NONE',  ( 0.000000000000000000, 0.01356324068817998940, -0.9999080150203990547 ) ) ;
#10049=ORIENTED_EDGE ( 'NONE', *, *, #43881, .F. ) ;
#10050=DIRECTION ( 'NONE',  ( -1.000000000000000000, -0.000000000000000000, -0.000000000000000000 ) ) ;
#10051=ORIENTED_EDGE ( 'NONE', *, *, #58894, .T. ) ;
#10053=VERTEX_POINT ( 'NONE', #13273 ) ;
#10054=CARTESIAN_POINT ( 'NONE',  ( -25.54417658651491863, 4.240019242199842608, 11.22596262356930197 ) ) ;
#10055=DIRECTION ( 'NONE',  ( 0.000000000000000000, -0.01356324068817999114, 0.9999080150203989437 ) ) ;
#10056=CARTESIAN_POINT ( 'NONE',  ( -35.00000000000000000, 9.040300684349693583, 7.499679039484089316 ) ) ;
#10057=CARTESIAN_POINT ( 'NONE',  ( 35.00000000000000000, -4.237620530777882699, -11.42599468261427909 ) ) ;
#10060=DIRECTION ( 'NONE',  ( 0.000000000000000000, 0.01356324068817991481, -0.9999080150203990547 ) ) ;
#10062=CARTESIAN_POINT ( 'NONE',  ( 19.28625800530496903, 25.00000000000000000, 11.87904264843580471 ) ) ;
#10065=CARTESIAN_POINT ( 'NONE',  ( -37.00000000000000711, -2.527899948230555971, -12.49688848680887077 ) ) ;
#10066=CIRCLE ( 'NONE', #56838, 12.75000000000000178 ) ;
#10068=DIRECTION ( 'NONE',  ( 1.000000000000000000, 0.000000000000000000, -0.000000000000000000 ) ) ;
#10070=EDGE_CURVE ( 'NONE', #31308, #173, #43853, .T. ) ;
#10071=CIRCLE ( 'NONE', #38737, 5.000000000000001776 ) ;
#10072=EDGE_LOOP ( 'NONE', ( #21246, #360, #3436, #583 ) ) ;
#10073=FACE_OUTER_BOUND ( 'NONE', #36918, .T. ) ;
#10074=DIRECTION ( 'NONE',  ( 0.000000000000000000, -0.8009703041134232926, -0.5987040770935588840 ) ) ;
#10078=CIRCLE ( 'NONE', #18600, 4.999999999999999112 ) ;
#10080=DIRECTION ( 'NONE',  ( 1.000000000000000000, 0.000000000000000000, 0.000000000000000000 ) ) ;
#10081=VERTEX_POINT ( 'NONE', #14545 ) ;
#10083=CARTESIAN_POINT ( 'NONE',  ( 35.00000000000000000, 12.18359334611896116, 0.2661492558803733588 ) ) ;
#10086=EDGE_CURVE ( 'NONE', #47572, #18051, #34190, .T. ) ;
#10087=AXIS2_PLACEMENT_3D ( 'NONE', #56277, #50343, #50659 ) ;
#10088=( BOUNDED_CURVE ( )  B_SPLINE_CURVE ( 3, ( #56801, #11862, #31807, #913 ),
 .UNSPECIFIED., .F., .F. ) 
 B_SPLINE_CURVE_WITH_KNOTS ( ( 4, 4 ),
 ( 5.040318585505245252, 5.044875135688600132 ),
 .UNSPECIFIED. ) 
 CURVE ( )  GEOMETRIC_REPRESENTATION_ITEM ( )  RATIONAL_B_SPLINE_CURVE ( ( 1.000000000000000000, 0.9999982698216172139, 0.9999982698216172139, 1.000000000000000000 ) ) 
 REPRESENTATION_ITEM ( '' )  );
#10093=CARTESIAN_POINT ( 'NONE',  ( 36.00000000000000711, 9.621072037176993774, -8.366449238204399563 ) ) ;
#10094=AXIS2_PLACEMENT_3D ( 'NONE', #25011, #30321, #14360 ) ;
#10096=CARTESIAN_POINT ( 'NONE',  ( 29.51976981715666781, 25.00000000000000000, 11.09513982864076276 ) ) ;
#10097=B_SPLINE_CURVE_WITH_KNOTS ( 'NONE', 3,
 ( #33279, #42925, #8337, #7337, #58572, #48588, #27621, #63850 ),
 .UNSPECIFIED., .F., .F.,
 ( 4, 2, 2, 4 ),
 ( 8.673617379884035472E-19, 0.002302291593524604611, 0.003453437390286906265, 0.004604583187049208354 ),
 .UNSPECIFIED. ) ;
#10098=EDGE_CURVE ( 'NONE', #58893, #12098, #58919, .T. ) ;
#10099=CARTESIAN_POINT ( 'NONE',  ( -35.00000000000000000, -9.063649021439015740, 8.146229107149364879 ) ) ;
#10100=CARTESIAN_POINT ( 'NONE',  ( -37.00000000000000711, 0.000000000000000000, 0.000000000000000000 ) ) ;
#10101=VERTEX_POINT ( 'NONE', #3654 ) ;
#10104=CARTESIAN_POINT ( 'NONE',  ( -35.00000000000000000, -11.96656215839365700, -4.400442035671072283 ) ) ;
#10105=ORIENTED_EDGE ( 'NONE', *, *, #9999, .F. ) ;
#10107=DIRECTION ( 'NONE',  ( -1.000000000000000000, 0.000000000000000000, -0.000000000000000000 ) ) ;
#10108=ORIENTED_EDGE ( 'NONE', *, *, #61134, .F. ) ;
#10109=ORIENTED_EDGE ( 'NONE', *, *, #21555, .F. ) ;
#10110=VERTEX_POINT ( 'NONE', #55128 ) ;
#10111=AXIS2_PLACEMENT_3D ( 'NONE', #20018, #58, #25018 ) ;
#10113=VERTEX_POINT ( 'NONE', #18914 ) ;
#10114=CYLINDRICAL_SURFACE ( 'NONE', #65250, 12.18649999999999878 ) ;
#10115=FACE_OUTER_BOUND ( 'NONE', #61842, .T. ) ;
#10118=EDGE_CURVE ( 'NONE', #44987, #1336, #40483, .T. ) ;
#10121=CARTESIAN_POINT ( 'NONE',  ( 23.97054589082751974, -3.699621146969923391, -12.98704298055938011 ) ) ;
#10123=ORIENTED_EDGE ( 'NONE', *, *, #5635, .T. ) ;
#10124=ADVANCED_FACE ( 'NONE', ( #39179 ), #4933, .T. ) ;
#10126=VERTEX_POINT ( 'NONE', #55463 ) ;
#10127=CARTESIAN_POINT ( 'NONE',  ( 37.00000000000000711, 3.704519465651471499, 11.60979404548630178 ) ) ;
#10133=CIRCLE ( 'NONE', #45162, 12.74999999999999822 ) ;
#10134=ADVANCED_FACE ( 'NONE', ( #19887 ), #50161, .T. ) ;
#10135=LINE ( 'NONE', #20109, #4742 ) ;
#10136=DIRECTION ( 'NONE',  ( -1.000000000000000000, -0.000000000000000000, 0.000000000000000000 ) ) ;
#10138=VERTEX_POINT ( 'NONE', #24884 ) ;
#10140=CYLINDRICAL_SURFACE ( 'NONE', #31621, 12.74999999999999822 ) ;
#10141=ORIENTED_EDGE ( 'NONE', *, *, #10014, .F. ) ;
#10147=CARTESIAN_POINT ( 'NONE',  ( 18.78223320782606010, 0.2848378300378480721, 11.99965915797046989 ) ) ;
#10149=CARTESIAN_POINT ( 'NONE',  ( -35.00000000000000000, 10.02106554660708859, 7.882940143791811849 ) ) ;
#10151=ORIENTED_EDGE ( 'NONE', *, *, #63115, .F. ) ;
#10152=ORIENTED_EDGE ( 'NONE', *, *, #7972, .F. ) ;
#10155=DIRECTION ( 'NONE',  ( -1.000000000000000000, 0.000000000000000000, 0.000000000000000000 ) ) ;
#10156=AXIS2_PLACEMENT_3D ( 'NONE', #60032, #60339, #39401 ) ;
#10157=CARTESIAN_POINT ( 'NONE',  ( 3.533297333898360204, -10.56865501033795773, 5.684349346051587482 ) ) ;
#10159=CARTESIAN_POINT ( 'NONE',  ( 23.56133193085831934, -3.409936927882566859, -13.06535930819385882 ) ) ;
#10160=CARTESIAN_POINT ( 'NONE',  ( 3.915429104661797055, 7.704244136310878233, -9.244377499037618406 ) ) ;
#10162=ORIENTED_EDGE ( 'NONE', *, *, #47460, .F. ) ;
#10164=CARTESIAN_POINT ( 'NONE',  ( -29.43980975494970309, -3.641506875706030488, -11.43413432115371364 ) ) ;
#10166=EDGE_CURVE ( 'NONE', #12385, #37272, #21729, .T. ) ;
#10167=AXIS2_PLACEMENT_3D ( 'NONE', #57121, #11547, #52131 ) ;
#10169=FACE_OUTER_BOUND ( 'NONE', #27780, .T. ) ;
#10170=ORIENTED_EDGE ( 'NONE', *, *, #7307, .F. ) ;
#10171=CARTESIAN_POINT ( 'NONE',  ( -17.79128287606087255, -5.234468747551053625, -12.44476184210350844 ) ) ;
#10178=DIRECTION ( 'NONE',  ( 1.000000000000000000, 0.000000000000000000, -0.000000000000000000 ) ) ;
#10179=ORIENTED_EDGE ( 'NONE', *, *, #39239, .F. ) ;
#10181=EDGE_CURVE ( 'NONE', #42983, #30009, #60442, .T. ) ;
#10182=AXIS2_PLACEMENT_3D ( 'NONE', #14381, #30985, #44623 ) ;
#10184=ORIENTED_EDGE ( 'NONE', *, *, #30193, .F. ) ;
#10187=CARTESIAN_POINT ( 'NONE',  ( 22.85866972464958025, -4.209424148273988919, -11.23992617506626601 ) ) ;
#10189=CARTESIAN_POINT ( 'NONE',  ( 8.534769016306631428, 5.427010460188671281, -12.36273961895021323 ) ) ;
#10191=DIRECTION ( 'NONE',  ( 1.000000000000000000, -0.000000000000000000, 0.000000000000000000 ) ) ;
#10193=ADVANCED_FACE ( 'NONE', ( #45469 ), #28886, .T. ) ;
#10194=VERTEX_POINT ( 'NONE', #8935 ) ;
#10195=FACE_OUTER_BOUND ( 'NONE', #63488, .T. ) ;
#10196=ORIENTED_EDGE ( 'NONE', *, *, #50810, .F. ) ;
#10197=CARTESIAN_POINT ( 'NONE',  ( -35.00000000000000000, -12.73293890771483028, -0.6593684648221820321 ) ) ;
#10198=AXIS2_PLACEMENT_3D ( 'NONE', #63605, #4432, #8759 ) ;
#10201=FACE_OUTER_BOUND ( 'NONE', #18358, .T. ) ;
#10202=VERTEX_POINT ( 'NONE', #49195 ) ;
#10203=CARTESIAN_POINT ( 'NONE',  ( 35.00000000000000000, -1.771820996347075017, 11.61175578952787113 ) ) ;
#10204=CARTESIAN_POINT ( 'NONE',  ( 12.83856522484696860, 11.13998188696922398, -4.465410698652262589 ) ) ;
#10206=ADVANCED_FACE ( 'NONE', ( #50492 ), #65737, .T. ) ;
#10207=EDGE_LOOP ( 'NONE', ( #44859, #34245, #33535, #34305 ) ) ;
#10209=LINE ( 'NONE', #14845, #13028 ) ;
#10210=ORIENTED_EDGE ( 'NONE', *, *, #25769, .F. ) ;
#10212=CARTESIAN_POINT ( 'NONE',  ( -35.00000000000000000, -0.6593684648221378453, 12.73293890771483028 ) ) ;
#10214=CARTESIAN_POINT ( 'NONE',  ( -29.11697232824620940, 1.969303236402622170, 11.84416604000747064 ) ) ;
#10217=EDGE_CURVE ( 'NONE', #26820, #6851, #47229, .T. ) ;
#10218=LINE ( 'NONE', #60434, #32278 ) ;
#10221=EDGE_CURVE ( 'NONE', #29813, #18977, #14235, .T. ) ;
#10222=CARTESIAN_POINT ( 'NONE',  ( 23.65879480623153341, 9.643861506414504348, -7.147527680982785903 ) ) ;
#10224=CARTESIAN_POINT ( 'NONE',  ( 11.98572745786314719, 10.93103263098930178, -7.928810397812742217 ) ) ;
#10225=CARTESIAN_POINT ( 'NONE',  ( -19.62351202312758502, -4.052328796303131142, 12.87840960595547557 ) ) ;
#10228=DIRECTION ( 'NONE',  ( 0.000000000000000000, -0.01356324068817991828, 0.9999080150203990547 ) ) ;
#10230=DIRECTION ( 'NONE',  ( 0.000000000000000000, 0.01356324068817998940, -0.9999080150203990547 ) ) ;
#10232=AXIS2_PLACEMENT_3D ( 'NONE', #25980, #20963, #45265 ) ;
#10234=CARTESIAN_POINT ( 'NONE',  ( -2.532614230583026593, -5.020478806276874373, 10.89930238848911337 ) ) ;
#10236=CARTESIAN_POINT ( 'NONE',  ( -16.58812090467340283, 7.647128368881745075, -11.12581290275694457 ) ) ;
#10238=FACE_OUTER_BOUND ( 'NONE', #37710, .T. ) ;
#10239=ORIENTED_EDGE ( 'NONE', *, *, #3322, .T. ) ;
#10240=LINE ( 'NONE', #5614, #65382 ) ;
#10241=CARTESIAN_POINT ( 'NONE',  ( 36.00000000000000711, -10.49626516989275693, -7.238157050195595410 ) ) ;
#10245=CARTESIAN_POINT ( 'NONE',  ( -19.16048775240928848, -3.902570516164022507, 11.34881310738079740 ) ) ;
#10246=CARTESIAN_POINT ( 'NONE',  ( -28.41827485489077532, 3.509237424706437292, 25.00000000000000000 ) ) ;
#10247=EDGE_LOOP ( 'NONE', ( #3276, #48861, #1039, #41677 ) ) ;
#10249=ORIENTED_EDGE ( 'NONE', *, *, #10342, .T. ) ;
#10250=CARTESIAN_POINT ( 'NONE',  ( -35.00000000000000000, 0.000000000000000000, 0.000000000000000000 ) ) ;
#10252=EDGE_CURVE ( 'NONE', #18553, #13952, #48034, .T. ) ;
#10253=CARTESIAN_POINT ( 'NONE',  ( 28.26028539291078800, -10.45631606572639249, 5.900903393808790476 ) ) ;
#10255=EDGE_CURVE ( 'NONE', #7701, #55855, #29174, .T. ) ;
#10256=EDGE_LOOP ( 'NONE', ( #49796, #511, #19972, #21706 ) ) ;
#10261=CARTESIAN_POINT ( 'NONE',  ( -35.00000000000000000, 5.130401251914729954, 11.05394794832831451 ) ) ;
#10262=DIRECTION ( 'NONE',  ( 0.000000000000000000, 0.01356324068817998940, -0.9999080150203990547 ) ) ;
#10268=VERTEX_POINT ( 'NONE', #5934 ) ;
#10269=EDGE_CURVE ( 'NONE', #36872, #24889, #39792, .T. ) ;
#10271=ORIENTED_EDGE ( 'NONE', *, *, #44522, .T. ) ;
#10272=CIRCLE ( 'NONE', #32564, 4.999999999999999112 ) ;
#10273=CARTESIAN_POINT ( 'NONE',  ( 0.000000000000000000, -1.734723475976807094E-15, 13.50000000000000178 ) ) ;
#10278=DIRECTION ( 'NONE',  ( -1.000000000000000000, -0.000000000000000000, 0.000000000000000000 ) ) ;
#10280=DIRECTION ( 'NONE',  ( 1.000000000000000000, -0.000000000000000000, 0.000000000000000000 ) ) ;
#10281=CARTESIAN_POINT ( 'NONE',  ( 35.00000000000000000, 11.47758908105697806, 2.497432891016712286 ) ) ;
#10282=EDGE_CURVE ( 'NONE', #22247, #41192, #61415, .T. ) ;
#10284=ORIENTED_EDGE ( 'NONE', *, *, #3045, .T. ) ;
#10287=ADVANCED_FACE ( 'NONE', ( #26190 ), #15854, .T. ) ;
#10288=ORIENTED_EDGE ( 'NONE', *, *, #48209, .F. ) ;
#10289=DIRECTION ( 'NONE',  ( -1.000000000000000000, 0.000000000000000000, 0.000000000000000000 ) ) ;
#10290=VERTEX_POINT ( 'NONE', #275 ) ;
#10291=VERTEX_POINT ( 'NONE', #10891 ) ;
#10292=EDGE_LOOP ( 'NONE', ( #44199, #48579, #40581, #51056 ) ) ;
#10293=EDGE_CURVE ( 'NONE', #37272, #15604, #12426, .T. ) ;
#10297=DIRECTION ( 'NONE',  ( -1.000000000000000000, -1.836970198721029688E-16, -0.000000000000000000 ) ) ;
#10298=CARTESIAN_POINT ( 'NONE',  ( 37.00000000000000711, -11.47561260193572963, 5.556331110570524423 ) ) ;
#10299=ORIENTED_EDGE ( 'NONE', *, *, #11984, .T. ) ;
#10300=EDGE_CURVE ( 'NONE', #19566, #60035, #17108, .T. ) ;
#10302=DIRECTION ( 'NONE',  ( 1.000000000000000000, 0.000000000000000000, 0.000000000000000000 ) ) ;
#10303=VERTEX_POINT ( 'NONE', #47385 ) ;
#10304=DIRECTION ( 'NONE',  ( 0.000000000000000000, 0.01356324068817998940, -0.9999080150203990547 ) ) ;
#10305=FACE_OUTER_BOUND ( 'NONE', #59680, .T. ) ;
#10307=ORIENTED_EDGE ( 'NONE', *, *, #6654, .T. ) ;
#10310=CARTESIAN_POINT ( 'NONE',  ( -37.00000000000000711, 12.18632975068353197, 0.06441628369840694812 ) ) ;
#10311=VERTEX_POINT ( 'NONE', #52700 ) ;
#10313=AXIS2_PLACEMENT_3D ( 'NONE', #20372, #30019, #50332 ) ;
#10314=EDGE_LOOP ( 'NONE', ( #47846, #39668, #12776, #5483 ) ) ;
#10315=CARTESIAN_POINT ( 'NONE',  ( -10.48620311856347875, -9.720786832536937538, -7.036071585506805448 ) ) ;
#10321=CARTESIAN_POINT ( 'NONE',  ( -35.00000000000000000, -10.32377448871672598, 6.475373545682264975 ) ) ;
#10322=CARTESIAN_POINT ( 'NONE',  ( 35.00000000000000000, -8.534258022646033837, 8.699265615723071221 ) ) ;
#10323=DIRECTION ( 'NONE',  ( 1.000000000000000000, -0.000000000000000000, 0.000000000000000000 ) ) ;
#10324=CIRCLE ( 'NONE', #40031, 5.000000000000002665 ) ;
#10325=CARTESIAN_POINT ( 'NONE',  ( 22.22052407907419180, -12.61035851597580049, -4.822980926764052434 ) ) ;
#10330=DIRECTION ( 'NONE',  ( -1.000000000000000000, 0.000000000000000000, 0.000000000000000000 ) ) ;
#10334=EDGE_CURVE ( 'NONE', #14286, #44679, #54720, .T. ) ;
#10335=ORIENTED_EDGE ( 'NONE', *, *, #19283, .T. ) ;
#10337=LINE ( 'NONE', #5370, #28973 ) ;
#10339=CYLINDRICAL_SURFACE ( 'NONE', #7736, 12.18650000000000055 ) ;
#10342=EDGE_CURVE ( 'NONE', #2029, #6394, #27401, .T. ) ;
#10344=ORIENTED_EDGE ( 'NONE', *, *, #20981, .T. ) ;
#10345=DIRECTION ( 'NONE',  ( -1.000000000000000000, 0.000000000000000000, -0.000000000000000000 ) ) ;
#10346=CIRCLE ( 'NONE', #44333, 5.000000000000000000 ) ;
#10350=FACE_OUTER_BOUND ( 'NONE', #3561, .T. ) ;
#10352=AXIS2_PLACEMENT_3D ( 'NONE', #6234, #16540, #36808 ) ;
#10353=ORIENTED_EDGE ( 'NONE', *, *, #49107, .T. ) ;
#10354=LINE ( 'NONE', #61891, #1425 ) ;
#10357=ORIENTED_EDGE ( 'NONE', *, *, #25890, .T. ) ;
#10358=FACE_OUTER_BOUND ( 'NONE', #54527, .T. ) ;
#10362=DIRECTION ( 'NONE',  ( 0.000000000000000000, -1.000000000000000000, 0.000000000000000000 ) ) ;
#10363=EDGE_CURVE ( 'NONE', #10393, #40729, #5600, .T. ) ;
#10364=DIRECTION ( 'NONE',  ( 0.000000000000000000, -0.01356324068818000328, 0.9999080150203990547 ) ) ;
#10365=CYLINDRICAL_SURFACE ( 'NONE', #46045, 5.000000000000000888 ) ;
#10367=CARTESIAN_POINT ( 'NONE',  ( 35.00000000000000000, -6.547236723513950807, 9.752226076388957665 ) ) ;
#10368=CIRCLE ( 'NONE', #5081, 5.000000000000000000 ) ;
#10369=CARTESIAN_POINT ( 'NONE',  ( 12.52750123246316072, 0.4973700281276248192, -11.98968819674306374 ) ) ;
#10372=CARTESIAN_POINT ( 'NONE',  ( 7.283637096917835230, -6.822343376425546779, 11.65715530555193347 ) ) ;
#10373=ORIENTED_EDGE ( 'NONE', *, *, #33838, .T. ) ;
#10379=CYLINDRICAL_SURFACE ( 'NONE', #40779, 4.999999999999999112 ) ;
#10380=EDGE_CURVE ( 'NONE', #12727, #15829, #39839, .T. ) ;
#10382=DIRECTION ( 'NONE',  ( -1.000000000000000000, -0.000000000000000000, 0.000000000000000000 ) ) ;
#10384=DIRECTION ( 'NONE',  ( 0.000000000000000000, -0.01356324068817998940, 0.9999080150203990547 ) ) ;
#10386=LINE ( 'NONE', #40986, #47874 ) ;
#10388=DIRECTION ( 'NONE',  ( 0.000000000000000000, 0.01356324068817998940, -0.9999080150203990547 ) ) ;
#10391=CARTESIAN_POINT ( 'NONE',  ( 47.00000000000000711, 4.705694406421931860E-17, -3.469127814946512892E-15 ) ) ;
#10393=VERTEX_POINT ( 'NONE', #48694 ) ;
#10395=VECTOR ( 'NONE', #24786, 1000.000000000000000 ) ;
#10398=AXIS2_PLACEMENT_3D ( 'NONE', #37965, #48312, #58609 ) ;
#10399=CARTESIAN_POINT ( 'NONE',  ( -35.00000000000000000, -11.78977382767499194, 4.245927698352017110 ) ) ;
#10400=DIRECTION ( 'NONE',  ( -0.000000000000000000, -0.000000000000000000, -1.000000000000000000 ) ) ;
#10401=LINE ( 'NONE', #5783, #33849 ) ;
#10402=AXIS2_PLACEMENT_3D ( 'NONE', #40726, #65643, #61016 ) ;
#10403=EDGE_LOOP ( 'NONE', ( #52241, #18499, #40685, #19672 ) ) ;
#10405=DIRECTION ( 'NONE',  ( 1.000000000000000000, 0.000000000000000000, -0.000000000000000000 ) ) ;
#10407=EDGE_CURVE ( 'NONE', #57508, #56892, #32385, .T. ) ;
#10408=AXIS2_PLACEMENT_3D ( 'NONE', #61920, #56269, #51639 ) ;
#10409=B_SPLINE_CURVE_WITH_KNOTS ( 'NONE', 3,
 ( #39266, #54897, #59562, #23331, #58604, #13026, #13350, #28640, #33635, #13996, #58938, #64222, #34282, #19974, #30926, #9651, #5348, #35898, #25619, #45249, #41224, #10003, #45912, #65198, #14631, #10635, #55885, #40242 ),
 .UNSPECIFIED., .F., .F.,
 ( 4, 2, 2, 2, 2, 2, 2, 2, 2, 2, 2, 2, 2, 4 ),
 ( 0.000000000000000000, 0.0005977287619976828954, 0.001195457523995365791, 0.001793186285993048686, 0.002390915047990731582, 0.002988643809988414477, 0.003586372571986097373, 0.004184101333983779834, 0.004781830095981463163, 0.005977287619976825485, 0.006575016381974505345, 0.007172745143972185204, 0.008368202667967547526, 0.009563660191962908980 ),
 .UNSPECIFIED. ) ;
#10410=CARTESIAN_POINT ( 'NONE',  ( 35.00000000000000000, -12.15823808070322798, -0.8294751490778934366 ) ) ;
#10413=CARTESIAN_POINT ( 'NONE',  ( 22.88594695219327235, -4.822122601967141264, -10.98850006195556261 ) ) ;
#10414=CARTESIAN_POINT ( 'NONE',  ( 0.3540037536853123390, 0.2457215634581275676, -11.99999999999999467 ) ) ;
#10415=DIRECTION ( 'NONE',  ( -1.000000000000000000, 0.000000000000000000, -0.000000000000000000 ) ) ;
#10416=ORIENTED_EDGE ( 'NONE', *, *, #58787, .F. ) ;
#10417=CARTESIAN_POINT ( 'NONE',  ( -18.58686583997219088, 4.911748662621227446, 10.95194156811396269 ) ) ;
#10418=CARTESIAN_POINT ( 'NONE',  ( -37.00000000000000711, 0.000000000000000000, 0.000000000000000000 ) ) ;
#10419=ORIENTED_EDGE ( 'NONE', *, *, #35354, .T. ) ;
#10421=EDGE_CURVE ( 'NONE', #57976, #56864, #33443, .T. ) ;
#10422=ORIENTED_EDGE ( 'NONE', *, *, #42884, .F. ) ;
#10423=VERTEX_POINT ( 'NONE', #7798 ) ;
#10424=EDGE_CURVE ( 'NONE', #60869, #8336, #63967, .T. ) ;
#10426=DIRECTION ( 'NONE',  ( 1.000000000000000000, -0.000000000000000000, 0.000000000000000000 ) ) ;
#10429=FACE_OUTER_BOUND ( 'NONE', #61644, .T. ) ;
#10430=DIRECTION ( 'NONE',  ( 0.000000000000000000, -0.01356324068817998940, 0.9999080150203990547 ) ) ;
#10431=AXIS2_PLACEMENT_3D ( 'NONE', #6553, #7868, #36798 ) ;
#10434=LINE ( 'NONE', #149, #63734 ) ;
#10436=DIRECTION ( 'NONE',  ( 1.000000000000000000, -0.000000000000000000, -0.000000000000000000 ) ) ;
#10438=FACE_OUTER_BOUND ( 'NONE', #48008, .T. ) ;
#10439=ORIENTED_EDGE ( 'NONE', *, *, #29602, .F. ) ;
#10443=ADVANCED_FACE ( 'NONE', ( #49670 ), #18451, .T. ) ;
#10444=AXIS2_PLACEMENT_3D ( 'NONE', #55786, #44809, #19221 ) ;
#10445=DIRECTION ( 'NONE',  ( 1.000000000000000000, -0.000000000000000000, 0.000000000000000000 ) ) ;
#10446=CYLINDRICAL_SURFACE ( 'NONE', #56763, 12.18649999999999878 ) ;
#10448=CARTESIAN_POINT ( 'NONE',  ( 37.00000000000000711, -11.16627499335657703, -3.645068577059991988 ) ) ;
#10451=VECTOR ( 'NONE', #4379, 1000.000000000000000 ) ;
#10452=AXIS2_PLACEMENT_3D ( 'NONE', #2114, #26087, #42649 ) ;
#10453=ORIENTED_EDGE ( 'NONE', *, *, #28790, .F. ) ;
#10455=ORIENTED_EDGE ( 'NONE', *, *, #35006, .T. ) ;
#10456=VECTOR ( 'NONE', #60861, 1000.000000000000000 ) ;
#10458=LINE ( 'NONE', #25433, #32776 ) ;
#10459=CARTESIAN_POINT ( 'NONE',  ( 9.402029343886097124, 7.266669477869928784, -9.551391452522942416 ) ) ;
#10460=VECTOR ( 'NONE', #1900, 1000.000000000000000 ) ;
#10462=CARTESIAN_POINT ( 'NONE',  ( 17.76182939893871193, -6.980167179982016634, 9.764583834413022245 ) ) ;
#10464=CARTESIAN_POINT ( 'NONE',  ( -37.00000000000000711, -7.717887834988307105, 8.854740511458828678 ) ) ;
#10466=( BOUNDED_CURVE ( )  B_SPLINE_CURVE ( 3, ( #5767, #15389, #20377, #55954 ),
 .UNSPECIFIED., .F., .F. ) 
 B_SPLINE_CURVE_WITH_KNOTS ( ( 4, 4 ),
 ( 2.228289365106484343, 2.237843681065574852 ),
 .UNSPECIFIED. ) 
 CURVE ( )  GEOMETRIC_REPRESENTATION_ITEM ( )  RATIONAL_B_SPLINE_CURVE ( ( 1.000000000000000000, 0.9999923929350129637, 0.9999923929350129637, 1.000000000000000000 ) ) 
 REPRESENTATION_ITEM ( '' )  );
#10467=ORIENTED_EDGE ( 'NONE', *, *, #56, .F. ) ;
#10471=CARTESIAN_POINT ( 'NONE',  ( 5.975816529957111101, -8.873589895540870742, 8.086295541294113320 ) ) ;
#10472=AXIS2_PLACEMENT_3D ( 'NONE', #3742, #63544, #63884 ) ;
#10473=FACE_OUTER_BOUND ( 'NONE', #21965, .T. ) ;
#10475=CIRCLE ( 'NONE', #40240, 5.000000000000001776 ) ;
#10476=DIRECTION ( 'NONE',  ( 1.000000000000000000, -0.000000000000000000, -0.000000000000000000 ) ) ;
#10478=CARTESIAN_POINT ( 'NONE',  ( 35.00000000000000000, -1.262958560998847624, -12.12087942037209665 ) ) ;
#10479=VERTEX_POINT ( 'NONE', #43348 ) ;
#10480=CARTESIAN_POINT ( 'NONE',  ( -37.00000000000000711, 2.527899948230636795, 12.49688848680885300 ) ) ;
#10482=DIRECTION ( 'NONE',  ( 0.000000000000000000, -1.000000000000000000, 0.000000000000000000 ) ) ;
#10483=CIRCLE ( 'NONE', #47673, 4.999999999999999112 ) ;
#10484=EDGE_CURVE ( 'NONE', #25959, #48365, #8126, .T. ) ;
#10487=AXIS2_PLACEMENT_3D ( 'NONE', #29, #56211, #10651 ) ;
#10488=ORIENTED_EDGE ( 'NONE', *, *, #7381, .T. ) ;
#10489=DIRECTION ( 'NONE',  ( -1.000000000000000000, 0.000000000000000000, -0.000000000000000000 ) ) ;
#10493=CARTESIAN_POINT ( 'NONE',  ( 22.88594695219327235, 3.421158645304719137, -13.05931366970166962 ) ) ;
#10494=CARTESIAN_POINT ( 'NONE',  ( 37.00000000000000711, 4.705694406421931860E-17, -3.469127814946512892E-15 ) ) ;
#10496=VECTOR ( 'NONE', #4533, 1000.000000000000000 ) ;
#10498=VERTEX_POINT ( 'NONE', #4455 ) ;
#10503=CARTESIAN_POINT ( 'NONE',  ( -8.648406403777006091, 10.29074439593462742, -8.744330510103520027 ) ) ;
#10505=FACE_OUTER_BOUND ( 'NONE', #2848, .T. ) ;
#10506=CARTESIAN_POINT ( 'NONE',  ( 0.000000000000000000, -1.734723475976807094E-15, -13.50000000000000178 ) ) ;
#10507=DIRECTION ( 'NONE',  ( 1.000000000000000000, 0.000000000000000000, 0.000000000000000000 ) ) ;
#10508=DIRECTION ( 'NONE',  ( 1.000000000000000000, 0.000000000000000000, -0.000000000000000000 ) ) ;
#10509=EDGE_LOOP ( 'NONE', ( #64100, #31033, #1428, #35788 ) ) ;
#10514=EDGE_CURVE ( 'NONE', #39567, #35917, #4796, .T. ) ;
#10517=B_SPLINE_CURVE_WITH_KNOTS ( 'NONE', 3,
 ( #13271, #40144, #34519, #3954, #50159, #39506, #24543, #44821, #65100, #39835, #24882, #65415, #60122, #48853, #14543, #18613, #3304, #9551 ),
 .UNSPECIFIED., .F., .F.,
 ( 4, 2, 2, 2, 2, 2, 2, 2, 4 ),
 ( 3.878959614448864246E-18, 0.001078534962646972685, 0.002157069925293941468, 0.003235604887940910033, 0.004314139850587879466, 0.005392674813234849332, 0.006471209775881817464, 0.007549744738528786463, 0.008628279701175755462 ),
 .UNSPECIFIED. ) ;
#10518=DIRECTION ( 'NONE',  ( 1.000000000000000000, 0.000000000000000000, 0.000000000000000000 ) ) ;
#10520=CARTESIAN_POINT ( 'NONE',  ( 37.00000000000000711, 1.903127969211351189, 11.59095880812005497 ) ) ;
#10521=VECTOR ( 'NONE', #14955, 1000.000000000000000 ) ;
#10522=DIRECTION ( 'NONE',  ( 0.000000000000000000, 0.01356324068817992522, -0.9999080150203990547 ) ) ;
#10524=ORIENTED_EDGE ( 'NONE', *, *, #36354, .T. ) ;
#10526=ORIENTED_EDGE ( 'NONE', *, *, #60566, .T. ) ;
#10527=CARTESIAN_POINT ( 'NONE',  ( 23.66565572653340510, -9.638793819117626782, -7.154491854832797593 ) ) ;
#10528=DIRECTION ( 'NONE',  ( 0.000000000000000000, 0.6943713148249588407, -0.7196168960969843154 ) ) ;
#10531=AXIS2_PLACEMENT_3D ( 'NONE', #32167, #38481, #58800 ) ;
#10532=EDGE_CURVE ( 'NONE', #60581, #16289, #1611, .T. ) ;
#10534=DIRECTION ( 'NONE',  ( -1.000000000000000000, 0.000000000000000000, 0.000000000000000000 ) ) ;
#10535=CARTESIAN_POINT ( 'NONE',  ( -14.17344535826537744, 8.096743466816491264, -10.80418385471381448 ) ) ;
#10537=ORIENTED_EDGE ( 'NONE', *, *, #61870, .T. ) ;
#10538=LINE ( 'NONE', #46150, #50868 ) ;
#10539=CARTESIAN_POINT ( 'NONE',  ( 22.11571975030548387, 11.89373260142252597, -1.635920820979222645 ) ) ;
#10541=DIRECTION ( 'NONE',  ( 1.000000000000000000, 0.000000000000000000, 0.000000000000000000 ) ) ;
#10544=DIRECTION ( 'NONE',  ( -1.000000000000000000, 0.000000000000000000, -0.000000000000000000 ) ) ;
#10545=AXIS2_PLACEMENT_3D ( 'NONE', #26683, #6095, #62252 ) ;
#10546=DIRECTION ( 'NONE',  ( 1.000000000000000000, 0.000000000000000000, 0.000000000000000000 ) ) ;
#10547=ADVANCED_FACE ( 'NONE', ( #51323 ), #65586, .T. ) ;
#10552=EDGE_CURVE ( 'NONE', #14292, #19644, #15700, .T. ) ;
#10553=DIRECTION ( 'NONE',  ( -0.000000000000000000, -0.000000000000000000, -1.000000000000000000 ) ) ;
#10556=ADVANCED_FACE ( 'NONE', ( #60617 ), #26039, .T. ) ;
#10558=ORIENTED_EDGE ( 'NONE', *, *, #62484, .F. ) ;
#10562=DIRECTION ( 'NONE',  ( 0.8914382917301157949, 0.000000000000000000, -0.4531421102008653112 ) ) ;
#10566=CARTESIAN_POINT ( 'NONE',  ( -17.15987333477080057, -7.887593880017340631, 9.050383707664092725 ) ) ;
#10568=VERTEX_POINT ( 'NONE', #35665 ) ;
#10569=AXIS2_PLACEMENT_3D ( 'NONE', #61585, #65585, #36324 ) ;
#10570=EDGE_CURVE ( 'NONE', #44077, #19066, #40323, .T. ) ;
#10575=FACE_OUTER_BOUND ( 'NONE', #37628, .T. ) ;
#10578=ORIENTED_EDGE ( 'NONE', *, *, #20439, .F. ) ;
#10579=EDGE_LOOP ( 'NONE', ( #58734, #63860, #28043, #56975 ) ) ;
#10580=CARTESIAN_POINT ( 'NONE',  ( -29.25731281466803324, 2.966737866142446833, 11.63518418675907817 ) ) ;
#10581=ADVANCED_FACE ( 'NONE', ( #35978 ), #15055, .T. ) ;
#10583=AXIS2_PLACEMENT_3D ( 'NONE', #9116, #43710, #44352 ) ;
#10584=DIRECTION ( 'NONE',  ( 1.000000000000000000, -0.000000000000000000, 0.000000000000000000 ) ) ;
#10585=CARTESIAN_POINT ( 'NONE',  ( 35.00000000000000000, 4.705694406421931860E-17, -3.469127814946512892E-15 ) ) ;
#10586=DIRECTION ( 'NONE',  ( 1.000000000000000000, 0.000000000000000000, 0.000000000000000000 ) ) ;
#10589=DIRECTION ( 'NONE',  ( -0.000000000000000000, -1.000000000000000000, -0.000000000000000000 ) ) ;
#10590=CARTESIAN_POINT ( 'NONE',  ( 35.00000000000000000, 4.705694406421931860E-17, -3.469127814946512892E-15 ) ) ;
#10591=ORIENTED_EDGE ( 'NONE', *, *, #1355, .T. ) ;
#10593=AXIS2_PLACEMENT_3D ( 'NONE', #11596, #41519, #61811 ) ;
#10596=DIRECTION ( 'NONE',  ( 1.000000000000000000, 0.000000000000000000, 0.000000000000000000 ) ) ;
#10597=DIRECTION ( 'NONE',  ( 1.000000000000000000, -0.000000000000000000, 0.000000000000000000 ) ) ;
#10600=ORIENTED_EDGE ( 'NONE', *, *, #12462, .T. ) ;
#10604=ORIENTED_EDGE ( 'NONE', *, *, #32866, .T. ) ;
#10605=ORIENTED_EDGE ( 'NONE', *, *, #7068, .F. ) ;
#10606=DIRECTION ( 'NONE',  ( -1.000000000000000000, 0.000000000000000000, -0.000000000000000000 ) ) ;
#10607=ORIENTED_EDGE ( 'NONE', *, *, #16469, .T. ) ;
#10608=DIRECTION ( 'NONE',  ( -0.000000000000000000, -0.000000000000000000, -1.000000000000000000 ) ) ;
#10611=VERTEX_POINT ( 'NONE', #65280 ) ;
#10612=DIRECTION ( 'NONE',  ( -0.000000000000000000, -0.000000000000000000, -1.000000000000000000 ) ) ;
#10616=DIRECTION ( 'NONE',  ( 0.000000000000000000, 0.3554799084908968343, 0.9346839223284540976 ) ) ;
#10617=VECTOR ( 'NONE', #47539, 1000.000000000000000 ) ;
#10618=CARTESIAN_POINT ( 'NONE',  ( 22.61491127797214062, 25.00000000000000000, 9.376349503825034404 ) ) ;
#10619=CARTESIAN_POINT ( 'NONE',  ( 37.00000000000000711, 9.926225166347027340, -6.280308599560179061 ) ) ;
#10622=ORIENTED_EDGE ( 'NONE', *, *, #28061, .T. ) ;
#10623=DIRECTION ( 'NONE',  ( -1.000000000000000000, 0.000000000000000000, 0.000000000000000000 ) ) ;
#10626=DIRECTION ( 'NONE',  ( 1.000000000000000000, 0.000000000000000000, -0.000000000000000000 ) ) ;
#10629=ADVANCED_FACE ( 'NONE', ( #9741 ), #40992, .T. ) ;
#10630=ORIENTED_EDGE ( 'NONE', *, *, #42655, .F. ) ;
#10631=CARTESIAN_POINT ( 'NONE',  ( 37.00000000000000711, 12.74921544981111055, -0.1414404973752615424 ) ) ;
#10634=ADVANCED_FACE ( 'NONE', ( #102 ), #25706, .T. ) ;
#10635=CARTESIAN_POINT ( 'NONE',  ( -25.13178613359605507, -8.065324219543505535, 10.83205263566206078 ) ) ;
#10637=CARTESIAN_POINT ( 'NONE',  ( -35.00000000000000000, 0.000000000000000000, 0.000000000000000000 ) ) ;
#10638=ADVANCED_FACE ( 'NONE', ( #20384 ), #45991, .T. ) ;
#10639=DIRECTION ( 'NONE',  ( 0.000000000000000000, -0.4698238015817425839, -0.8827602140260283337 ) ) ;
#10641=DIRECTION ( 'NONE',  ( -0.6147887355352408267, -0.7886918350401376232, 0.000000000000000000 ) ) ;
#10642=CARTESIAN_POINT ( 'NONE',  ( 37.00000000000000711, 8.366449238204499039, 9.621072037176899627 ) ) ;
#10643=AXIS2_PLACEMENT_3D ( 'NONE', #19863, #40125, #35129 ) ;
#10645=CARTESIAN_POINT ( 'NONE',  ( 22.62155329971168172, -12.20561453419441200, -5.777527435223176688 ) ) ;
#10647=EDGE_CURVE ( 'NONE', #3974, #57258, #47270, .T. ) ;
#10648=AXIS2_PLACEMENT_3D ( 'NONE', #64910, #44976, #54653 ) ;
#10651=DIRECTION ( 'NONE',  ( 0.000000000000000000, 0.01356324068817998940, -0.9999080150203990547 ) ) ;
#10652=AXIS2_PLACEMENT_3D ( 'NONE', #45770, #35458, #232 ) ;
#10653=DIRECTION ( 'NONE',  ( -1.000000000000000000, 0.000000000000000000, 0.000000000000000000 ) ) ;
#10654=FACE_OUTER_BOUND ( 'NONE', #42201, .T. ) ;
#10656=EDGE_CURVE ( 'NONE', #15829, #40279, #6915, .T. ) ;
#10657=VECTOR ( 'NONE', #7903, 1000.000000000000000 ) ;
#10659=CIRCLE ( 'NONE', #61647, 5.000000000000000000 ) ;
#10660=ORIENTED_EDGE ( 'NONE', *, *, #32319, .F. ) ;
#10661=ADVANCED_FACE ( 'NONE', ( #6406 ), #7367, .T. ) ;
#10663=( BOUNDED_CURVE ( )  B_SPLINE_CURVE ( 3, ( #11113, #4497, #5142, #30711 ),
 .UNSPECIFIED., .F., .F. ) 
 B_SPLINE_CURVE_WITH_KNOTS ( ( 4, 4 ),
 ( 2.222160218901154227, 2.254442315838258271 ),
 .UNSPECIFIED. ) 
 CURVE ( )  GEOMETRIC_REPRESENTATION_ITEM ( )  RATIONAL_B_SPLINE_CURVE ( ( 1.000000000000000000, 0.9999131574035865500, 0.9999131574035865500, 1.000000000000000000 ) ) 
 REPRESENTATION_ITEM ( '' )  );
#10664=FACE_OUTER_BOUND ( 'NONE', #54885, .T. ) ;
#10667=EDGE_CURVE ( 'NONE', #50465, #32047, #37718, .T. ) ;
#10668=CARTESIAN_POINT ( 'NONE',  ( -35.00000000000000000, 6.657191900728318679, 9.677500615117924809 ) ) ;
#10670=ORIENTED_EDGE ( 'NONE', *, *, #6516, .T. ) ;
#10673=AXIS2_PLACEMENT_3D ( 'NONE', #5821, #1132, #16434 ) ;
#10674=DIRECTION ( 'NONE',  ( -1.000000000000000000, 0.000000000000000000, 0.000000000000000000 ) ) ;
#10676=CARTESIAN_POINT ( 'NONE',  ( -17.90400865550613574, 4.131545694691102000, -11.26818433703756384 ) ) ;
#10677=VECTOR ( 'NONE', #56445, 1000.000000000000000 ) ;
#10678=VECTOR ( 'NONE', #56597, 1000.000000000000000 ) ;
#10680=ORIENTED_EDGE ( 'NONE', *, *, #25667, .T. ) ;
#10683=DIRECTION ( 'NONE',  ( -0.000000000000000000, -0.000000000000000000, -1.000000000000000000 ) ) ;
#10685=AXIS2_PLACEMENT_3D ( 'NONE', #4448, #53995, #8438 ) ;
#10686=DIRECTION ( 'NONE',  ( -0.000000000000000000, -0.000000000000000000, -1.000000000000000000 ) ) ;
#10689=AXIS2_PLACEMENT_3D ( 'NONE', #49580, #19648, #54574 ) ;
#10690=ORIENTED_EDGE ( 'NONE', *, *, #48125, .F. ) ;
#10691=CYLINDRICAL_SURFACE ( 'NONE', #12820, 4.999999999999999112 ) ;
#10694=DIRECTION ( 'NONE',  ( 0.000000000000000000, 0.8009703041134146329, 0.5987040770935705414 ) ) ;
#10696=EDGE_CURVE ( 'NONE', #44942, #58777, #50444, .T. ) ;
#10697=CARTESIAN_POINT ( 'NONE',  ( -35.00000000000000000, -1.463443770872689509, -12.09831040184925577 ) ) ;
#10698=CARTESIAN_POINT ( 'NONE',  ( 35.00000000000000000, -4.725891942574827809, -10.75351884295726101 ) ) ;
#10699=CARTESIAN_POINT ( 'NONE',  ( 35.00000000000000000, 0.1652884326465054732, -12.18537902504609427 ) ) ;
#10701=CARTESIAN_POINT ( 'NONE',  ( -17.50079231878650177, 2.685795310841043282, -13.23113775294028649 ) ) ;
#10702=ORIENTED_EDGE ( 'NONE', *, *, #46129, .T. ) ;
#10705=CYLINDRICAL_SURFACE ( 'NONE', #63517, 12.18650000000000055 ) ;
#10707=AXIS2_PLACEMENT_3D ( 'NONE', #58039, #32727, #48067 ) ;
#10709=EDGE_CURVE ( 'NONE', #54583, #15438, #51965, .T. ) ;
#10710=CYLINDRICAL_SURFACE ( 'NONE', #28575, 5.000000000000000888 ) ;
#10715=AXIS2_PLACEMENT_3D ( 'NONE', #36754, #12131, #1533 ) ;
#10716=AXIS2_PLACEMENT_3D ( 'NONE', #48133, #33479, #6581 ) ;
#10717=AXIS2_PLACEMENT_3D ( 'NONE', #21490, #42383, #12152 ) ;
#10718=ADVANCED_FACE ( 'NONE', ( #762 ), #26681, .T. ) ;
#10719=EDGE_LOOP ( 'NONE', ( #14831, #12509, #12085, #51539, #30525, #48290 ) ) ;
#10720=CARTESIAN_POINT ( 'NONE',  ( -19.32000128823278118, -3.826633625541849160, -11.37379849559869527 ) ) ;
#10721=AXIS2_PLACEMENT_3D ( 'NONE', #39083, #49099, #44389 ) ;
#10724=DIRECTION ( 'NONE',  ( 1.000000000000000000, 0.000000000000000000, 0.000000000000000000 ) ) ;
#10725=CARTESIAN_POINT ( 'NONE',  ( -2.952869152607111136, 4.384817011589738911, 11.17020052527586138 ) ) ;
#10726=EDGE_CURVE ( 'NONE', #50602, #37599, #22868, .T. ) ;
#10727=ORIENTED_EDGE ( 'NONE', *, *, #59806, .T. ) ;
#10730=CIRCLE ( 'NONE', #22410, 12.18649999999999878 ) ;
#10731=AXIS2_PLACEMENT_3D ( 'NONE', #22388, #32365, #27376 ) ;
#10732=CARTESIAN_POINT ( 'NONE',  ( 28.33327753883506261, 12.08535766013368473, 6.028296700677072906 ) ) ;
#10733=CARTESIAN_POINT ( 'NONE',  ( -29.68541646480307250, -2.179156473586586262, 11.82547580031049606 ) ) ;
#10737=DIRECTION ( 'NONE',  ( -1.000000000000000000, 0.000000000000000000, 0.000000000000000000 ) ) ;
#10738=CARTESIAN_POINT ( 'NONE',  ( 37.00000000000000711, 4.705694406421931860E-17, -3.469127814946512892E-15 ) ) ;
#10740=AXIS2_PLACEMENT_3D ( 'NONE', #46146, #10878, #36803 ) ;
#10741=EDGE_CURVE ( 'NONE', #32235, #49156, #48374, .T. ) ;
#10742=EDGE_CURVE ( 'NONE', #47877, #30464, #36970, .T. ) ;
#10744=FACE_OUTER_BOUND ( 'NONE', #41589, .T. ) ;
#10745=CIRCLE ( 'NONE', #27740, 5.000000000000000888 ) ;
#10748=DIRECTION ( 'NONE',  ( 0.000000000000000000, 0.9651210252299803338, 0.2618041379715598249 ) ) ;
#10751=EDGE_CURVE ( 'NONE', #27227, #61808, #12264, .T. ) ;
#10752=DIRECTION ( 'NONE',  ( 0.000000000000000000, -0.01356324068817999114, 0.9999080150203989437 ) ) ;
#10757=LINE ( 'NONE', #5808, #32695 ) ;
#10758=AXIS2_PLACEMENT_3D ( 'NONE', #26358, #1097, #21373 ) ;
#10759=AXIS2_PLACEMENT_3D ( 'NONE', #41739, #56739, #32405 ) ;
#10761=FACE_OUTER_BOUND ( 'NONE', #61238, .T. ) ;
#10764=DIRECTION ( 'NONE',  ( 1.000000000000000000, 0.000000000000000000, 0.000000000000000000 ) ) ;
#10765=ORIENTED_EDGE ( 'NONE', *, *, #64422, .T. ) ;
#10766=CARTESIAN_POINT ( 'NONE',  ( -35.00000000000000000, -9.752226076388847531, -6.547236723514122225 ) ) ;
#10768=CARTESIAN_POINT ( 'NONE',  ( 35.00000000000000000, 0.8294751490779324055, -12.15823808070322798 ) ) ;
#10769=CARTESIAN_POINT ( 'NONE',  ( 35.00000000000000000, 4.705694406421931860E-17, -3.469127814946512892E-15 ) ) ;
#10770=ORIENTED_EDGE ( 'NONE', *, *, #31666, .T. ) ;
#10772=ORIENTED_EDGE ( 'NONE', *, *, #6293, .T. ) ;
#10774=ORIENTED_EDGE ( 'NONE', *, *, #45243, .T. ) ;
#10775=ORIENTED_EDGE ( 'NONE', *, *, #2370, .T. ) ;
#10778=AXIS2_PLACEMENT_3D ( 'NONE', #10448, #21428, #26097 ) ;
#10781=AXIS2_PLACEMENT_3D ( 'NONE', #16323, #6033, #1697 ) ;
#10784=DIRECTION ( 'NONE',  ( 0.000000000000000000, -0.01356324068817998940, 0.9999080150203990547 ) ) ;
#10788=EDGE_CURVE ( 'NONE', #15077, #10081, #1659, .T. ) ;
#10789=VERTEX_POINT ( 'NONE', #21711 ) ;
#10790=DIRECTION ( 'NONE',  ( 0.000000000000000000, 0.01356324068817998940, -0.9999080150203990547 ) ) ;
#10791=EDGE_LOOP ( 'NONE', ( #61445, #55190, #19663, #59478 ) ) ;
#10793=AXIS2_PLACEMENT_3D ( 'NONE', #62317, #62011, #61336 ) ;
#10796=CYLINDRICAL_SURFACE ( 'NONE', #22399, 12.18649999999999878 ) ;
#10797=CARTESIAN_POINT ( 'NONE',  ( 18.62706029620522941, 2.680501531300553797, 11.70880161399673902 ) ) ;
#10799=FACE_OUTER_BOUND ( 'NONE', #6958, .T. ) ;
#10800=DIRECTION ( 'NONE',  ( 0.000000000000000000, 0.01356324068817991828, -0.9999080150203990547 ) ) ;
#10801=VECTOR ( 'NONE', #14138, 1000.000000000000000 ) ;
#10802=EDGE_LOOP ( 'NONE', ( #58935, #24867, #1545, #1034 ) ) ;
#10805=LINE ( 'NONE', #31422, #31879 ) ;
#10807=EDGE_CURVE ( 'NONE', #29673, #60341, #8054, .T. ) ;
#10811=VECTOR ( 'NONE', #5119, 1000.000000000000000 ) ;
#10813=CARTESIAN_POINT ( 'NONE',  ( 22.86325106016951736, 2.804889020532796096, -13.20736364802678509 ) ) ;
#10814=DIRECTION ( 'NONE',  ( -1.000000000000000000, 0.000000000000000000, 0.000000000000000000 ) ) ;
#10815=CARTESIAN_POINT ( 'NONE',  ( -19.69476066079020171, -4.201994156881551312, 25.00000000000000000 ) ) ;
#10816=ORIENTED_EDGE ( 'NONE', *, *, #55768, .T. ) ;
#10817=CARTESIAN_POINT ( 'NONE',  ( -36.00000000000000711, -11.96656215839366055, -4.400442035671074059 ) ) ;
#10820=AXIS2_PLACEMENT_3D ( 'NONE', #59297, #34974, #24704 ) ;
#10821=EDGE_CURVE ( 'NONE', #54202, #4686, #10133, .T. ) ;
#10822=VECTOR ( 'NONE', #2262, 1000.000000000000000 ) ;
#10823=AXIS2_PLACEMENT_3D ( 'NONE', #19753, #40010, #14720 ) ;
#10824=EDGE_CURVE ( 'NONE', #30241, #44540, #18655, .T. ) ;
#10825=CARTESIAN_POINT ( 'NONE',  ( -26.91319780901507386, 10.55334688052688819, 5.712466060832438686 ) ) ;
#10826=CARTESIAN_POINT ( 'NONE',  ( 26.08439714455133185, 11.40113243194252846, 3.743551691817327942 ) ) ;
#10828=CARTESIAN_POINT ( 'NONE',  ( -17.14251155165674234, -7.213546477669500412, -11.41604601608509562 ) ) ;
#10829=CARTESIAN_POINT ( 'NONE',  ( 11.74548640120467979, 25.00000000000000000, -8.184666801472349817 ) ) ;
#10830=AXIS2_PLACEMENT_3D ( 'NONE', #31947, #52268, #37614 ) ;
#10832=VERTEX_POINT ( 'NONE', #8700 ) ;
#10834=DIRECTION ( 'NONE',  ( 0.000000000000000000, -1.000000000000000000, 0.000000000000000000 ) ) ;
#10836=CYLINDRICAL_SURFACE ( 'NONE', #41504, 12.75000000000000178 ) ;
#10839=ORIENTED_EDGE ( 'NONE', *, *, #13510, .T. ) ;
#10841=CARTESIAN_POINT ( 'NONE',  ( -35.00000000000000000, -8.927548052240956267, 8.295159312811819063 ) ) ;
#10842=VERTEX_POINT ( 'NONE', #13352 ) ;
#10843=DIRECTION ( 'NONE',  ( -0.9015184547431841500, -0.4327406564646559262, 0.000000000000000000 ) ) ;
#10845=CARTESIAN_POINT ( 'NONE',  ( -47.00000000000000711, 0.000000000000000000, 0.000000000000000000 ) ) ;
#10848=CARTESIAN_POINT ( 'NONE',  ( -9.552061971074056856, 9.047766850818582895, -7.885493295094908817 ) ) ;
#10849=DIRECTION ( 'NONE',  ( 0.1034490876700550344, -0.000000000000000000, 0.9946347501772866417 ) ) ;
#10850=DIRECTION ( 'NONE',  ( 0.000000000000000000, -0.8169148498130213154, 0.5767582926625057782 ) ) ;
#10851=ORIENTED_EDGE ( 'NONE', *, *, #46528, .F. ) ;
#10854=ORIENTED_EDGE ( 'NONE', *, *, #30627, .F. ) ;
#10855=AXIS2_PLACEMENT_3D ( 'NONE', #62056, #11497, #32428 ) ;
#10858=CIRCLE ( 'NONE', #60801, 5.000000000000000000 ) ;
#10860=AXIS2_PLACEMENT_3D ( 'NONE', #55465, #276, #34522 ) ;
#10862=ORIENTED_EDGE ( 'NONE', *, *, #55900, .T. ) ;
#10868=VERTEX_POINT ( 'NONE', #3070 ) ;
#10874=AXIS2_PLACEMENT_3D ( 'NONE', #37519, #52512, #2284 ) ;
#10875=CARTESIAN_POINT ( 'NONE',  ( -36.00000000000000711, -4.561791185930499815, 11.90598845858532329 ) ) ;
#10876=CARTESIAN_POINT ( 'NONE',  ( -29.68541646480307250, -1.416020129149132334, 11.91616074890920451 ) ) ;
#10878=DIRECTION ( 'NONE',  ( -1.000000000000000000, 0.000000000000000000, 0.000000000000000000 ) ) ;
#10879=EDGE_CURVE ( 'NONE', #51547, #22753, #50494, .T. ) ;
#10880=DIRECTION ( 'NONE',  ( -1.000000000000000000, 0.000000000000000000, 0.000000000000000000 ) ) ;
#10885=FACE_OUTER_BOUND ( 'NONE', #29259, .T. ) ;
#10886=EDGE_CURVE ( 'NONE', #16429, #64737, #30302, .T. ) ;
#10888=CARTESIAN_POINT ( 'NONE',  ( -9.317739297035824819, 10.04120852590977186, -6.581867252412223479 ) ) ;
#10889=CARTESIAN_POINT ( 'NONE',  ( -37.00000000000000711, 0.000000000000000000, 0.000000000000000000 ) ) ;
#10890=FACE_OUTER_BOUND ( 'NONE', #25396, .T. ) ;
#10891=CARTESIAN_POINT ( 'NONE',  ( 17.27839441901508621, 10.52068335315811076, 5.771933972472480967 ) ) ;
#10893=EDGE_CURVE ( 'NONE', #37431, #2532, #33061, .T. ) ;
#10894=ORIENTED_EDGE ( 'NONE', *, *, #13397, .F. ) ;
#10896=DIRECTION ( 'NONE',  ( 0.000000000000000000, 0.9246979985058736418, 0.3807014730195186214 ) ) ;
#10897=AXIS2_PLACEMENT_3D ( 'NONE', #53175, #2665, #7623 ) ;
#10898=ORIENTED_EDGE ( 'NONE', *, *, #56497, .T. ) ;
#10899=CYLINDRICAL_SURFACE ( 'NONE', #55292, 4.000030059823568074 ) ;
#10902=FACE_OUTER_BOUND ( 'NONE', #18474, .T. ) ;
#10904=AXIS2_PLACEMENT_3D ( 'NONE', #64624, #50017, #40686 ) ;
#10905=CARTESIAN_POINT ( 'NONE',  ( -10.95212338237647920, -9.902220863987562183, -9.175839033069911110 ) ) ;
#10906=CARTESIAN_POINT ( 'NONE',  ( 37.00000000000000711, 4.705694406421931860E-17, -3.469127814946512892E-15 ) ) ;
#10907=CIRCLE ( 'NONE', #19421, 12.18650000000000055 ) ;
#10908=DIRECTION ( 'NONE',  ( 1.000000000000000000, 0.000000000000000000, 0.000000000000000000 ) ) ;
#10911=CIRCLE ( 'NONE', #11950, 12.74999999999999822 ) ;
#10912=VECTOR ( 'NONE', #64244, 1000.000000000000000 ) ;
#10914=DIRECTION ( 'NONE',  ( -0.000000000000000000, -0.000000000000000000, -1.000000000000000000 ) ) ;
#10915=ORIENTED_EDGE ( 'NONE', *, *, #13824, .T. ) ;
#10916=LINE ( 'NONE', #56469, #47718 ) ;
#10917=EDGE_LOOP ( 'NONE', ( #19690, #60843, #19941, #4006 ) ) ;
#10918=CARTESIAN_POINT ( 'NONE',  ( 35.00000000000000000, 4.705694406421931860E-17, -3.469127814946512892E-15 ) ) ;
#10919=DIRECTION ( 'NONE',  ( 0.000000000000000000, -0.2618041379715704275, 0.9651210252299774472 ) ) ;
#10923=ADVANCED_FACE ( 'NONE', ( #5350 ), #29948, .T. ) ;
#10924=CIRCLE ( 'NONE', #57648, 4.999999999999998224 ) ;
#10925=VERTEX_POINT ( 'NONE', #61200 ) ;
#10928=VERTEX_POINT ( 'NONE', #40584 ) ;
#10930=CARTESIAN_POINT ( 'NONE',  ( -37.00000000000000711, 11.68758509253248334, -1.171570255487489609 ) ) ;
#10933=CARTESIAN_POINT ( 'NONE',  ( 22.78397477906666069, 3.290341966830223175, 11.54089583822153031 ) ) ;
#10934=B_SPLINE_CURVE_WITH_KNOTS ( 'NONE', 3,
 ( #52433, #6871, #42741, #27142, #17160, #12480, #37437, #57748, #12167, #37772, #58066, #8487, #48743, #28771, #58388, #3860, #54719, #63354, #38759, #8168 ),
 .UNSPECIFIED., .F., .F.,
 ( 4, 2, 2, 2, 2, 2, 2, 2, 2, 4 ),
 ( 4.249187360970369464E-18, 0.001349386060196310121, 0.002024079090294461820, 0.002698772120392613737, 0.004048158180588917569, 0.004722851210687068618, 0.005397544240785222269, 0.006746930300981533908, 0.008096316361177842078, 0.01079508848157046189 ),
 .UNSPECIFIED. ) ;
#10936=DIRECTION ( 'NONE',  ( 0.000000000000000000, 0.000000000000000000, -1.000000000000000000 ) ) ;
#10938=ORIENTED_EDGE ( 'NONE', *, *, #3982, .F. ) ;
#10941=LINE ( 'NONE', #31858, #38703 ) ;
#10942=FACE_OUTER_BOUND ( 'NONE', #20676, .T. ) ;
#10943=VECTOR ( 'NONE', #39984, 1000.000000000000000 ) ;
#10945=ORIENTED_EDGE ( 'NONE', *, *, #18101, .F. ) ;
#10947=ORIENTED_EDGE ( 'NONE', *, *, #1512, .F. ) ;
#10953=ORIENTED_EDGE ( 'NONE', *, *, #45563, .F. ) ;
#10954=ORIENTED_EDGE ( 'NONE', *, *, #19020, .T. ) ;
#10955=CARTESIAN_POINT ( 'NONE',  ( 2.061095049060549744, 2.059564177347529945, 13.34611721626114189 ) ) ;
#10957=VERTEX_POINT ( 'NONE', #59903 ) ;
#10959=VERTEX_POINT ( 'NONE', #65507 ) ;
#10960=VECTOR ( 'NONE', #29116, 1000.000000000000000 ) ;
#10963=CARTESIAN_POINT ( 'NONE',  ( 6.812204945636112896, -4.138731716409435712, -11.26369831714194092 ) ) ;
#10965=AXIS2_PLACEMENT_3D ( 'NONE', #49611, #14646, #59920 ) ;
#10966=AXIS2_PLACEMENT_3D ( 'NONE', #21226, #42471, #51837 ) ;
#10969=ADVANCED_FACE ( 'NONE', ( #50256 ), #34605, .T. ) ;
#10970=DIRECTION ( 'NONE',  ( 0.000000000000000000, 0.8009703041134188517, 0.5987040770935649903 ) ) ;
#10972=DIRECTION ( 'NONE',  ( 1.000000000000000000, 0.000000000000000000, 0.000000000000000000 ) ) ;
#10975=VECTOR ( 'NONE', #27644, 1000.000000000000000 ) ;
#10976=CARTESIAN_POINT ( 'NONE',  ( -2.532614230583023041, 12.88560382747354005, 4.026315189028235153 ) ) ;
#10977=CARTESIAN_POINT ( 'NONE',  ( 35.00000000000000000, 12.18359334611896116, 0.2661492558803733588 ) ) ;
#10984=ORIENTED_EDGE ( 'NONE', *, *, #17187, .F. ) ;
#10985=FACE_OUTER_BOUND ( 'NONE', #35332, .T. ) ;
#10987=VERTEX_POINT ( 'NONE', #57534 ) ;
#10989=DIRECTION ( 'NONE',  ( 0.000000000000000000, -0.7196168960969719919, -0.6943713148249717193 ) ) ;
#10990=CIRCLE ( 'NONE', #65127, 5.000000000000000000 ) ;
#10992=DIRECTION ( 'NONE',  ( -1.000000000000000000, 0.000000000000000000, 0.000000000000000000 ) ) ;
#10994=ORIENTED_EDGE ( 'NONE', *, *, #23326, .T. ) ;
#10995=DIRECTION ( 'NONE',  ( 0.000000000000000000, -0.01356324068817992175, 0.9999080150203990547 ) ) ;
#10998=AXIS2_PLACEMENT_3D ( 'NONE', #32196, #2294, #11594 ) ;
#11002=LINE ( 'NONE', #38132, #65159 ) ;
#11003=FACE_BOUND ( 'NONE', #13857, .T. ) ;
#11006=AXIS2_PLACEMENT_3D ( 'NONE', #19833, #35093, #19516 ) ;
#11009=EDGE_LOOP ( 'NONE', ( #141, #19135, #62848, #49453 ) ) ;
#11011=VECTOR ( 'NONE', #43446, 1000.000000000000000 ) ;
#11012=DIRECTION ( 'NONE',  ( 1.000000000000000000, 0.000000000000000000, 0.000000000000000000 ) ) ;
#11013=CARTESIAN_POINT ( 'NONE',  ( 37.00000000000000711, -9.512294188640847636, 6.891188680298922620 ) ) ;
#11017=CIRCLE ( 'NONE', #48218, 4.999999999999999112 ) ;
#11021=AXIS2_PLACEMENT_3D ( 'NONE', #55007, #57312, #36016 ) ;
#11026=DIRECTION ( 'NONE',  ( 0.000000000000000000, -0.01356324068817991828, 0.9999080150203990547 ) ) ;
#11029=EDGE_CURVE ( 'NONE', #39390, #58474, #32421, .T. ) ;
#11032=CARTESIAN_POINT ( 'NONE',  ( 23.20038713279159026, 3.176051149014137653, 11.57489057894666651 ) ) ;
#11033=ORIENTED_EDGE ( 'NONE', *, *, #60960, .F. ) ;
#11034=CARTESIAN_POINT ( 'NONE',  ( -37.00000000000000711, 0.8294751490781091530, -12.15823808070321910 ) ) ;
#11036=ORIENTED_EDGE ( 'NONE', *, *, #17449, .F. ) ;
#11039=CARTESIAN_POINT ( 'NONE',  ( -18.25006854224444908, -9.443202773001939221, 9.647586298549914119 ) ) ;
#11041=DIRECTION ( 'NONE',  ( -1.000000000000000000, 0.000000000000000000, 0.000000000000000000 ) ) ;
#11042=CARTESIAN_POINT ( 'NONE',  ( -35.00000000000000000, -11.66664283989676321, -5.143145423404402727 ) ) ;
#11043=DIRECTION ( 'NONE',  ( -1.000000000000000000, 0.000000000000000000, 0.000000000000000000 ) ) ;
#11044=DIRECTION ( 'NONE',  ( -1.000000000000000000, 0.000000000000000000, 0.000000000000000000 ) ) ;
#11045=ADVANCED_FACE ( 'NONE', ( #26937 ), #6984, .T. ) ;
#11046=DIRECTION ( 'NONE',  ( -1.000000000000000000, 0.000000000000000000, 0.000000000000000000 ) ) ;
#11048=CARTESIAN_POINT ( 'NONE',  ( 3.865165140261278331, -11.00552270324296700, 7.820176569034111402 ) ) ;
#11049=ORIENTED_EDGE ( 'NONE', *, *, #35267, .F. ) ;
#11054=FACE_OUTER_BOUND ( 'NONE', #44230, .T. ) ;
#11055=AXIS2_PLACEMENT_3D ( 'NONE', #4894, #50448, #51756 ) ;
#11057=DIRECTION ( 'NONE',  ( 1.000000000000000000, 0.000000000000000000, 0.000000000000000000 ) ) ;
#11058=AXIS2_PLACEMENT_3D ( 'NONE', #51820, #11887, #7224 ) ;
#11064=ORIENTED_EDGE ( 'NONE', *, *, #39016, .F. ) ;
#11065=CARTESIAN_POINT ( 'NONE',  ( -17.19897187406723305, -8.155961655565807433, -8.809094555608780297 ) ) ;
#11066=EDGE_CURVE ( 'NONE', #46955, #55862, #35418, .T. ) ;
#11068=ORIENTED_EDGE ( 'NONE', *, *, #19601, .T. ) ;
#11070=EDGE_CURVE ( 'NONE', #31482, #60850, #43194, .T. ) ;
#11071=CARTESIAN_POINT ( 'NONE',  ( 37.00000000000000711, 4.705694406421931860E-17, -3.469127814946512892E-15 ) ) ;
#11072=CARTESIAN_POINT ( 'NONE',  ( 35.00000000000000000, 12.12087942037209842, -1.262958560998807656 ) ) ;
#11076=CIRCLE ( 'NONE', #17442, 12.18650000000000233 ) ;
#11079=CARTESIAN_POINT ( 'NONE',  ( -35.00000000000000000, -10.62137734850264614, -5.015831474386418520 ) ) ;
#11081=CARTESIAN_POINT ( 'NONE',  ( 8.437200413559443390, 4.861907246157027629, 12.60074865033406688 ) ) ;
#11082=CARTESIAN_POINT ( 'NONE',  ( -28.41827485489077532, 3.509237424706436403, 13.03592162821792222 ) ) ;
#11084=DIRECTION ( 'NONE',  ( 1.000000000000000000, 0.000000000000000000, -0.000000000000000000 ) ) ;
#11085=ADVANCED_FACE ( 'NONE', ( #53189 ), #42874, .T. ) ;
#11087=LINE ( 'NONE', #11398, #18292 ) ;
#11090=EDGE_CURVE ( 'NONE', #24439, #30430, #56905, .T. ) ;
#11091=CARTESIAN_POINT ( 'NONE',  ( 35.00000000000000000, 5.428340790341703581, -10.91072401419412685 ) ) ;
#11092=DIRECTION ( 'NONE',  ( 0.000000000000000000, -0.01356324068817999114, 0.9999080150203989437 ) ) ;
#11093=CARTESIAN_POINT ( 'NONE',  ( -37.00000000000000711, 11.73463472867576129, 3.287724142101457137 ) ) ;
#11094=ORIENTED_EDGE ( 'NONE', *, *, #37797, .F. ) ;
#11096=CARTESIAN_POINT ( 'NONE',  ( 47.00000000000000711, 4.705694406421931860E-17, -3.469127814946512892E-15 ) ) ;
#11097=ORIENTED_EDGE ( 'NONE', *, *, #27086, .F. ) ;
#11098=EDGE_CURVE ( 'NONE', #53717, #25218, #3663, .T. ) ;
#11099=AXIS2_PLACEMENT_3D ( 'NONE', #10918, #47805, #41830 ) ;
#11103=DIRECTION ( 'NONE',  ( 0.000000000000000000, -1.000000000000000000, 0.000000000000000000 ) ) ;
#11104=EDGE_CURVE ( 'NONE', #44042, #44597, #16497, .T. ) ;
#11105=ORIENTED_EDGE ( 'NONE', *, *, #37462, .F. ) ;
#11106=CARTESIAN_POINT ( 'NONE',  ( -24.90342394282648186, -7.521682070300208522, 9.357467395294243317 ) ) ;
#11107=DIRECTION ( 'NONE',  ( 1.000000000000000000, 0.000000000000000000, -0.000000000000000000 ) ) ;
#11108=DIRECTION ( 'NONE',  ( -1.000000000000000000, -0.000000000000000000, -0.000000000000000000 ) ) ;
#11109=CARTESIAN_POINT ( 'NONE',  ( 10.21897715134382700, 7.428883895067158960, 9.428733153766255981 ) ) ;
#11111=CARTESIAN_POINT ( 'NONE',  ( 37.00000000000000711, 2.216820770815085773, -11.53507381115584529 ) ) ;
#11113=CARTESIAN_POINT ( 'NONE',  ( 11.74548640120467979, -10.73597826697111124, -8.184666801472349817 ) ) ;
#11116=LINE ( 'NONE', #20432, #35223 ) ;
#11117=ADVANCED_FACE ( 'NONE', ( #7637 ), #64454, .T. ) ;
#11119=CARTESIAN_POINT ( 'NONE',  ( -37.00000000000000711, 2.497432891017006718, -11.47758908105691766 ) ) ;
#11121=ORIENTED_EDGE ( 'NONE', *, *, #18776, .T. ) ;
#11122=CARTESIAN_POINT ( 'NONE',  ( -35.00000000000000000, 10.92721691015462149, -4.309077947445535628 ) ) ;
#11123=CARTESIAN_POINT ( 'NONE',  ( -35.00000000000000000, 3.093009498344089447, -11.78745411414836930 ) ) ;
#11124=AXIS2_PLACEMENT_3D ( 'NONE', #18799, #38410, #8477 ) ;
#11125=FACE_OUTER_BOUND ( 'NONE', #26136, .T. ) ;
#11126=ORIENTED_EDGE ( 'NONE', *, *, #23872, .F. ) ;
#11127=LINE ( 'NONE', #16446, #37609 ) ;
#11130=VERTEX_POINT ( 'NONE', #37889 ) ;
#11131=ORIENTED_EDGE ( 'NONE', *, *, #33005, .F. ) ;
#11134=EDGE_CURVE ( 'NONE', #33743, #38347, #35609, .T. ) ;
#11136=ORIENTED_EDGE ( 'NONE', *, *, #54987, .T. ) ;
#11139=CYLINDRICAL_SURFACE ( 'NONE', #8590, 4.999999999999999112 ) ;
#11141=DIRECTION ( 'NONE',  ( -1.000000000000000000, 0.000000000000000000, -0.000000000000000000 ) ) ;
#11142=EDGE_CURVE ( 'NONE', #10138, #58567, #64147, .T. ) ;
#11143=CARTESIAN_POINT ( 'NONE',  ( -37.00000000000000711, 0.2661492558805056974, -12.18359334611896116 ) ) ;
#11144=CARTESIAN_POINT ( 'NONE',  ( -37.00000000000000711, 0.000000000000000000, 0.000000000000000000 ) ) ;
#11146=CARTESIAN_POINT ( 'NONE',  ( 22.57855258442565116, 3.026812727784649493, -11.61199400236326973 ) ) ;
#11152=DIRECTION ( 'NONE',  ( -1.000000000000000000, 0.000000000000000000, 0.000000000000000000 ) ) ;
#11153=DIRECTION ( 'NONE',  ( 1.000000000000000000, 0.000000000000000000, 0.000000000000000000 ) ) ;
#11154=CARTESIAN_POINT ( 'NONE',  ( 3.734305248975252400, 4.620446052658566671, -11.08365692675047498 ) ) ;
#11156=ORIENTED_EDGE ( 'NONE', *, *, #23529, .T. ) ;
#11159=DIRECTION ( 'NONE',  ( 1.000000000000000000, 0.000000000000000000, 0.000000000000000000 ) ) ;
#11161=CIRCLE ( 'NONE', #49402, 12.18649999999999878 ) ;
#11166=FACE_OUTER_BOUND ( 'NONE', #21386, .T. ) ;
#11167=CARTESIAN_POINT ( 'NONE',  ( -18.58686583997218378, 5.151216734910788908, 25.00000000000000000 ) ) ;
#11169=ORIENTED_EDGE ( 'NONE', *, *, #61174, .T. ) ;
#11170=DIRECTION ( 'NONE',  ( 0.000000000000000000, -0.01356324068817998940, 0.9999080150203990547 ) ) ;
#11171=CARTESIAN_POINT ( 'NONE',  ( -18.06081662158740642, 5.589072243798248074, -10.62163489563124763 ) ) ;
#11172=CARTESIAN_POINT ( 'NONE',  ( 35.00000000000000000, 4.705694406421931860E-17, -3.469127814946512892E-15 ) ) ;
#11173=EDGE_CURVE ( 'NONE', #33373, #16971, #17602, .T. ) ;
#11175=EDGE_LOOP ( 'NONE', ( #25756, #65718, #62624, #47304 ) ) ;
#11176=LINE ( 'NONE', #41753, #38440 ) ;
#11177=AXIS2_PLACEMENT_3D ( 'NONE', #57942, #41305, #37645 ) ;
#11182=CARTESIAN_POINT ( 'NONE',  ( 23.74704636295951587, -3.121621105806414498, -11.59142313195714635 ) ) ;
#11187=VERTEX_POINT ( 'NONE', #54828 ) ;
#11188=EDGE_CURVE ( 'NONE', #44435, #49368, #65112, .T. ) ;
#11189=ORIENTED_EDGE ( 'NONE', *, *, #45323, .F. ) ;
#11191=ORIENTED_EDGE ( 'NONE', *, *, #63463, .F. ) ;
#11194=DIRECTION ( 'NONE',  ( 0.000000000000000000, 0.9937233664769756780, -0.1118654143051654171 ) ) ;
#11195=CARTESIAN_POINT ( 'NONE',  ( -16.98800322446194855, 2.922502605998049674, 11.63868456991315625 ) ) ;
#11197=ORIENTED_EDGE ( 'NONE', *, *, #9349, .T. ) ;
#11199=CIRCLE ( 'NONE', #48386, 12.74999999999999822 ) ;
#11201=FACE_OUTER_BOUND ( 'NONE', #24798, .T. ) ;
#11203=ORIENTED_EDGE ( 'NONE', *, *, #44402, .T. ) ;
#11205=ORIENTED_EDGE ( 'NONE', *, *, #65077, .T. ) ;
#11206=CARTESIAN_POINT ( 'NONE',  ( 21.99454477296592714, -11.37209199534426318, -3.835509361899974046 ) ) ;
#11208=DIRECTION ( 'NONE',  ( -1.000000000000000000, 0.000000000000000000, 0.000000000000000000 ) ) ;
#11209=EDGE_CURVE ( 'NONE', #40162, #1597, #39847, .T. ) ;
#11210=CIRCLE ( 'NONE', #34547, 12.18650000000000055 ) ;
#11211=DIRECTION ( 'NONE',  ( -0.000000000000000000, -1.000000000000000000, -0.000000000000000000 ) ) ;
#11212=FACE_OUTER_BOUND ( 'NONE', #37202, .T. ) ;
#11213=DIRECTION ( 'NONE',  ( 0.000000000000000000, 0.9999080150203989437, 0.01356324068817649567 ) ) ;
#11214=EDGE_CURVE ( 'NONE', #23613, #14430, #24995, .T. ) ;
#11216=ORIENTED_EDGE ( 'NONE', *, *, #51506, .F. ) ;
#11218=ADVANCED_FACE ( 'NONE', ( #29529 ), #9565, .T. ) ;
#11219=CARTESIAN_POINT ( 'NONE',  ( 25.05309951391468459, 8.823569016628493245, -8.132934882857099979 ) ) ;
#11220=CARTESIAN_POINT ( 'NONE',  ( -18.49080574448680991, -12.00000000000057909, -4.407108900774715188E-13 ) ) ;
#11222=CARTESIAN_POINT ( 'NONE',  ( 37.00000000000000711, -10.99909370905160699, -5.246972444133983338 ) ) ;
#11225=EDGE_LOOP ( 'NONE', ( #27801, #54857, #64465, #20701 ) ) ;
#11227=ORIENTED_EDGE ( 'NONE', *, *, #15126, .F. ) ;
#11228=LINE ( 'NONE', #65742, #56705 ) ;
#11229=EDGE_CURVE ( 'NONE', #47974, #4532, #29859, .T. ) ;
#11231=VERTEX_POINT ( 'NONE', #19895 ) ;
#11233=CARTESIAN_POINT ( 'NONE',  ( 35.00000000000000000, -9.506317355798429958, -8.496612874013125705 ) ) ;
#11235=ORIENTED_EDGE ( 'NONE', *, *, #55133, .F. ) ;
#11236=LINE ( 'NONE', #55814, #64301 ) ;
#11238=LINE ( 'NONE', #61430, #25833 ) ;
#11241=DIRECTION ( 'NONE',  ( 0.000000000000000000, -0.01356324068817998940, 0.9999080150203989437 ) ) ;
#11242=EDGE_CURVE ( 'NONE', #1249, #153, #9262, .T. ) ;
#11243=DIRECTION ( 'NONE',  ( -1.000000000000000000, 0.000000000000000000, 0.000000000000000000 ) ) ;
#11244=AXIS2_PLACEMENT_3D ( 'NONE', #57125, #16224, #20222 ) ;
#11248=FACE_OUTER_BOUND ( 'NONE', #19854, .T. ) ;
#11252=B_SPLINE_CURVE_WITH_KNOTS ( 'NONE', 3,
 ( #23134, #59700, #19469, #43399, #54055, #44706, #8829, #14128, #9142, #29425, #29118, #64343, #49721, #64657, #59366, #3861, #33751, #24119, #24433, #39400, #63675, #7857 ),
 .UNSPECIFIED., .F., .F.,
 ( 4, 2, 2, 2, 2, 2, 2, 2, 2, 2, 4 ),
 ( 8.673617379884035472E-19, 0.001081624167374303650, 0.002163248334748606432, 0.003244872502122908564, 0.004326496669497210262, 0.004867308753184361111, 0.005408120836871511961, 0.005948932920558663677, 0.006489745004245815393, 0.007571369171620122296, 0.008652993338994427464 ),
 .UNSPECIFIED. ) ;
#11254=CARTESIAN_POINT ( 'NONE',  ( -9.842799140981188799, -4.069970586457803741, 11.29001410203253108 ) ) ;
#11256=ORIENTED_EDGE ( 'NONE', *, *, #12025, .F. ) ;
#11257=VERTEX_POINT ( 'NONE', #21874 ) ;
#11259=ORIENTED_EDGE ( 'NONE', *, *, #55830, .F. ) ;
#11260=CARTESIAN_POINT ( 'NONE',  ( 35.00000000000000000, -8.954052073409666690, -9.076753354953966735 ) ) ;
#11261=( BOUNDED_CURVE ( )  B_SPLINE_CURVE ( 3, ( #5096, #45641, #35660, #56623 ),
 .UNSPECIFIED., .F., .F. ) 
 B_SPLINE_CURVE_WITH_KNOTS ( ( 4, 4 ),
 ( 2.321366128334107160, 2.361114018676058635 ),
 .UNSPECIFIED. ) 
 CURVE ( )  GEOMETRIC_REPRESENTATION_ITEM ( )  RATIONAL_B_SPLINE_CURVE ( ( 1.000000000000000000, 0.9998683464345071714, 0.9998683464345071714, 1.000000000000000000 ) ) 
 REPRESENTATION_ITEM ( '' )  );
#11263=DIRECTION ( 'NONE',  ( 0.000000000000000000, -0.9651210252299822212, -0.2618041379715529970 ) ) ;
#11264=CARTESIAN_POINT ( 'NONE',  ( -27.16343335735464493, 10.63351257863160981, -8.317934404008967775 ) ) ;
#11267=CARTESIAN_POINT ( 'NONE',  ( -10.87446691779126695, -4.893491060116321734, 10.96515481982397766 ) ) ;
#11268=ORIENTED_EDGE ( 'NONE', *, *, #57452, .F. ) ;
#11269=EDGE_CURVE ( 'NONE', #8493, #59819, #43055, .T. ) ;
#11270=EDGE_CURVE ( 'NONE', #25074, #50979, #60066, .T. ) ;
#11272=VERTEX_POINT ( 'NONE', #6906 ) ;
#11274=DIRECTION ( 'NONE',  ( 1.000000000000000000, 0.000000000000000000, 0.000000000000000000 ) ) ;
#11276=ORIENTED_EDGE ( 'NONE', *, *, #11581, .F. ) ;
#11277=FACE_OUTER_BOUND ( 'NONE', #55749, .T. ) ;
#11278=EDGE_LOOP ( 'NONE', ( #20895, #9724, #33905, #33593 ) ) ;
#11279=CARTESIAN_POINT ( 'NONE',  ( -35.00000000000000000, 2.527899948230635907, 12.49688848680885123 ) ) ;
#11281=DIRECTION ( 'NONE',  ( 1.000000000000000000, -0.000000000000000000, 0.000000000000000000 ) ) ;
#11282=VERTEX_POINT ( 'NONE', #21194 ) ;
#11285=ORIENTED_EDGE ( 'NONE', *, *, #50914, .F. ) ;
#11286=CARTESIAN_POINT ( 'NONE',  ( -35.00000000000000000, -0.2661492558804205988, 12.18359334611896472 ) ) ;
#11287=ORIENTED_EDGE ( 'NONE', *, *, #46751, .T. ) ;
#11288=VERTEX_POINT ( 'NONE', #27177 ) ;
#11289=ORIENTED_EDGE ( 'NONE', *, *, #39024, .T. ) ;
#11295=CYLINDRICAL_SURFACE ( 'NONE', #18958, 12.18649999999999878 ) ;
#11298=CARTESIAN_POINT ( 'NONE',  ( 16.78263030916553689, 12.17295508002146320, 5.836879698929895888 ) ) ;
#11301=CARTESIAN_POINT ( 'NONE',  ( 12.47628546223243617, 0.000000000000000000, -11.99999999999998224 ) ) ;
#11302=FACE_OUTER_BOUND ( 'NONE', #22913, .T. ) ;
#11303=CARTESIAN_POINT ( 'NONE',  ( 37.00000000000000711, 12.63095688309029008, -1.738225594540043772 ) ) ;
#11304=CARTESIAN_POINT ( 'NONE',  ( 36.00000000000000711, 0.1414404973753900230, 12.74921544981110522 ) ) ;
#11306=CYLINDRICAL_SURFACE ( 'NONE', #19647, 13.50000000000000178 ) ;
#11308=EDGE_CURVE ( 'NONE', #35397, #25443, #46166, .T. ) ;
#11309=ORIENTED_EDGE ( 'NONE', *, *, #28671, .F. ) ;
#11311=ORIENTED_EDGE ( 'NONE', *, *, #63633, .F. ) ;
#11315=DIRECTION ( 'NONE',  ( 0.000000000000000000, -0.01356324068817999114, 0.9999080150203989437 ) ) ;
#11316=ORIENTED_EDGE ( 'NONE', *, *, #38114, .F. ) ;
#11317=CARTESIAN_POINT ( 'NONE',  ( -35.00000000000000000, 0.000000000000000000, 0.000000000000000000 ) ) ;
#11318=LINE ( 'NONE', #37225, #435 ) ;
#11319=CARTESIAN_POINT ( 'NONE',  ( 21.74395625310401314, 11.95369699707849165, -1.122435266587093139 ) ) ;
#11321=ADVANCED_FACE ( 'NONE', ( #21544 ), #612, .T. ) ;
#11322=CARTESIAN_POINT ( 'NONE',  ( 47.00000000000000711, 4.705694406421931860E-17, -3.469127814946512892E-15 ) ) ;
#11329=AXIS2_PLACEMENT_3D ( 'NONE', #20091, #9778, #59683 ) ;
#11330=ORIENTED_EDGE ( 'NONE', *, *, #49457, .T. ) ;
#11331=ORIENTED_EDGE ( 'NONE', *, *, #45730, .T. ) ;
#11332=DIRECTION ( 'NONE',  ( 1.000000000000000000, -0.000000000000000000, 0.000000000000000000 ) ) ;
#11334=DIRECTION ( 'NONE',  ( 1.000000000000000000, 0.000000000000000000, 0.000000000000000000 ) ) ;
#11336=ORIENTED_EDGE ( 'NONE', *, *, #54192, .T. ) ;
#11337=EDGE_CURVE ( 'NONE', #54245, #48534, #53716, .T. ) ;
#11338=ADVANCED_FACE ( 'NONE', ( #20559 ), #62403, .T. ) ;
#11339=VERTEX_POINT ( 'NONE', #11233 ) ;
#11340=EDGE_LOOP ( 'NONE', ( #21274, #61112, #23396, #64478 ) ) ;
#11341=DIRECTION ( 'NONE',  ( 0.000000000000000000, 0.01356324068817992175, -0.9999080150203990547 ) ) ;
#11344=DIRECTION ( 'NONE',  ( 0.000000000000000000, 0.01356324068817998940, -0.9999080150203990547 ) ) ;
#11345=DIRECTION ( 'NONE',  ( -1.000000000000000000, -0.000000000000000000, -0.000000000000000000 ) ) ;
#11349=CARTESIAN_POINT ( 'NONE',  ( 24.70884604468378498, -2.111405277004652969, 11.81439423874797257 ) ) ;
#11350=EDGE_LOOP ( 'NONE', ( #309, #13698, #40033, #4175 ) ) ;
#11351=FACE_OUTER_BOUND ( 'NONE', #50388, .T. ) ;
#11352=ORIENTED_EDGE ( 'NONE', *, *, #50230, .F. ) ;
#11356=DIRECTION ( 'NONE',  ( 1.000000000000000000, 0.000000000000000000, 0.000000000000000000 ) ) ;
#11358=CARTESIAN_POINT ( 'NONE',  ( 35.00000000000000000, 9.621072037176993774, -8.366449238204399563 ) ) ;
#11360=CARTESIAN_POINT ( 'NONE',  ( 47.00000000000000711, 4.705694406421931860E-17, -3.469127814946512892E-15 ) ) ;
#11361=ORIENTED_EDGE ( 'NONE', *, *, #1424, .T. ) ;
#11362=DIRECTION ( 'NONE',  ( -1.000000000000000000, 0.000000000000000000, 0.000000000000000000 ) ) ;
#11363=EDGE_LOOP ( 'NONE', ( #52916, #16375, #28528, #54466 ) ) ;
#11364=CIRCLE ( 'NONE', #24137, 12.75000000000000178 ) ;
#11366=CARTESIAN_POINT ( 'NONE',  ( 35.00000000000000000, -2.216820770815006725, 11.53507381115585417 ) ) ;
#11369=CARTESIAN_POINT ( 'NONE',  ( -18.43818118241833659, 6.164186468232681904, 10.29965514685089367 ) ) ;
#11370=CYLINDRICAL_SURFACE ( 'NONE', #56335, 7.011478057721953761 ) ;
#11371=DIRECTION ( 'NONE',  ( 1.000000000000000000, 0.000000000000000000, 0.000000000000000000 ) ) ;
#11372=CIRCLE ( 'NONE', #41116, 12.18650000000000055 ) ;
#11374=EDGE_CURVE ( 'NONE', #61765, #48935, #52781, .T. ) ;
#11376=VERTEX_POINT ( 'NONE', #32793 ) ;
#11378=CARTESIAN_POINT ( 'NONE',  ( -17.34002536255959015, -6.190470376513365736, -10.28142836167298135 ) ) ;
#11379=EDGE_LOOP ( 'NONE', ( #53958, #41932, #9944, #26194 ) ) ;
#11381=DIRECTION ( 'NONE',  ( 1.000000000000000000, 0.000000000000000000, -0.000000000000000000 ) ) ;
#11382=FACE_OUTER_BOUND ( 'NONE', #25042, .T. ) ;
#11383=VERTEX_POINT ( 'NONE', #64054 ) ;
#11385=EDGE_CURVE ( 'NONE', #50140, #34717, #47362, .T. ) ;
#11386=EDGE_CURVE ( 'NONE', #16455, #40131, #20348, .T. ) ;
#11387=CARTESIAN_POINT ( 'NONE',  ( 26.77130308255667401, 12.82903357082578921, 4.213245553477073635 ) ) ;
#11388=CARTESIAN_POINT ( 'NONE',  ( -15.27729454824424948, 5.151216734910788908, 25.00000000000000000 ) ) ;
#11389=LINE ( 'NONE', #460, #2356 ) ;
#11390=CYLINDRICAL_SURFACE ( 'NONE', #37030, 4.999999999999999112 ) ;
#11391=EDGE_CURVE ( 'NONE', #31684, #41765, #47789, .T. ) ;
#11392=DIRECTION ( 'NONE',  ( 0.000000000000000000, -0.01356324068817991828, 0.9999080150203990547 ) ) ;
#11395=AXIS2_PLACEMENT_3D ( 'NONE', #26648, #16994, #42242 ) ;
#11396=EDGE_CURVE ( 'NONE', #51437, #11726, #19591, .T. ) ;
#11397=ORIENTED_EDGE ( 'NONE', *, *, #40669, .F. ) ;
#11398=CARTESIAN_POINT ( 'NONE',  ( 6.812204945636112896, -4.138731716409435712, 25.00000000000000000 ) ) ;
#11400=ORIENTED_EDGE ( 'NONE', *, *, #19514, .T. ) ;
#11403=CARTESIAN_POINT ( 'NONE',  ( 1.299397328467618129, 1.108794299602723132, -11.95234461178691276 ) ) ;
#11404=DIRECTION ( 'NONE',  ( -1.000000000000000000, -0.000000000000000000, -0.000000000000000000 ) ) ;
#11406=CARTESIAN_POINT ( 'NONE',  ( -35.00000000000000000, 11.95840593935201213, 2.346765782874477679 ) ) ;
#11408=DIRECTION ( 'NONE',  ( 0.000000000000000000, 0.9987865678893278476, -0.04924826701374234589 ) ) ;
#11409=EDGE_LOOP ( 'NONE', ( #18806, #41643, #27731, #2081 ) ) ;
#11410=AXIS2_PLACEMENT_3D ( 'NONE', #34506, #54807, #9226 ) ;
#11411=VERTEX_POINT ( 'NONE', #33783 ) ;
#11413=AXIS2_PLACEMENT_3D ( 'NONE', #9451, #15752, #36032 ) ;
#11416=CARTESIAN_POINT ( 'NONE',  ( -25.54554785668764438, -5.744669996086663843, 10.54128946422876290 ) ) ;
#11419=DIRECTION ( 'NONE',  ( -1.000000000000000000, 0.000000000000000000, -0.000000000000000000 ) ) ;
#11421=CYLINDRICAL_SURFACE ( 'NONE', #38525, 6.511478057721953761 ) ;
#11426=CYLINDRICAL_SURFACE ( 'NONE', #44759, 5.000000000000000888 ) ;
#11428=VERTEX_POINT ( 'NONE', #8518 ) ;
#11429=CARTESIAN_POINT ( 'NONE',  ( -37.00000000000000711, 0.000000000000000000, 0.000000000000000000 ) ) ;
#11432=CARTESIAN_POINT ( 'NONE',  ( 47.00000000000000711, 4.705694406421931860E-17, -3.469127814946512892E-15 ) ) ;
#11436=DIRECTION ( 'NONE',  ( 0.000000000000000000, 0.04924826701374598187, 0.9987865678893278476 ) ) ;
#11438=ORIENTED_EDGE ( 'NONE', *, *, #24628, .T. ) ;
#11441=CARTESIAN_POINT ( 'NONE',  ( 35.00000000000000000, -4.725891942574827809, -10.75351884295726101 ) ) ;
#11443=ORIENTED_EDGE ( 'NONE', *, *, #27126, .F. ) ;
#11444=DIRECTION ( 'NONE',  ( 0.000000000000000000, 0.01356324068817998940, -0.9999080150203990547 ) ) ;
#11449=CIRCLE ( 'NONE', #1917, 12.18649999999999878 ) ;
#11450=EDGE_CURVE ( 'NONE', #30305, #12197, #18278, .T. ) ;
#11452=DIRECTION ( 'NONE',  ( 0.000000000000000000, 0.01356324068817998940, -0.9999080150203990547 ) ) ;
#11453=CIRCLE ( 'NONE', #28446, 12.18649999999999700 ) ;
#11456=DIRECTION ( 'NONE',  ( 0.000000000000000000, 0.000000000000000000, -1.000000000000000000 ) ) ;
#11457=CARTESIAN_POINT ( 'NONE',  ( 37.00000000000000711, 11.35427606708806003, -4.426194442447284771 ) ) ;
#11458=EDGE_CURVE ( 'NONE', #34717, #28861, #65229, .T. ) ;
#11464=EDGE_CURVE ( 'NONE', #61567, #35169, #8206, .T. ) ;
#11467=CARTESIAN_POINT ( 'NONE',  ( -35.00000000000000000, 11.47758908105694786, 2.497432891016883261 ) ) ;
#11468=CARTESIAN_POINT ( 'NONE',  ( -19.47984447937493613, -1.416020129149132334, 25.00000000000000000 ) ) ;
#11469=CARTESIAN_POINT ( 'NONE',  ( 35.00000000000000000, 4.705694406421931860E-17, -3.469127814946512892E-15 ) ) ;
#11470=CARTESIAN_POINT ( 'NONE',  ( 10.10599715024921963, 1.639952862261359501, -13.40131696041721909 ) ) ;
#11472=ORIENTED_EDGE ( 'NONE', *, *, #48508, .T. ) ;
#11473=AXIS2_PLACEMENT_3D ( 'NONE', #50062, #4520, #33457 ) ;
#11474=LINE ( 'NONE', #4878, #48257 ) ;
#11475=LINE ( 'NONE', #26781, #52464 ) ;
#11476=EDGE_CURVE ( 'NONE', #14758, #44370, #14152, .T. ) ;
#11478=ORIENTED_EDGE ( 'NONE', *, *, #12834, .T. ) ;
#11480=CARTESIAN_POINT ( 'NONE',  ( 35.00000000000000000, -0.01609748574436820068, 11.74614673114903596 ) ) ;
#11483=CARTESIAN_POINT ( 'NONE',  ( 35.00000000000000000, 4.705694406421931860E-17, -3.469127814946512892E-15 ) ) ;
#11485=CARTESIAN_POINT ( 'NONE',  ( 37.00000000000000711, -5.428340790341627198, 10.91072401419415883 ) ) ;
#11486=ADVANCED_FACE ( 'NONE', ( #49449 ), #19819, .T. ) ;
#11490=EDGE_CURVE ( 'NONE', #63372, #7682, #55055, .T. ) ;
#11491=CYLINDRICAL_SURFACE ( 'NONE', #4721, 12.75000000000000178 ) ;
#11493=AXIS2_PLACEMENT_3D ( 'NONE', #59252, #65209, #64860 ) ;
#11494=CARTESIAN_POINT ( 'NONE',  ( 24.20270661733482953, 0.6951122250270121983, -11.98503915607300208 ) ) ;
#11495=VECTOR ( 'NONE', #35382, 1000.000000000000000 ) ;
#11497=DIRECTION ( 'NONE',  ( 1.000000000000000000, -0.000000000000000000, 0.000000000000000000 ) ) ;
#11499=DIRECTION ( 'NONE',  ( 0.000000000000000000, 0.6745969609292663538, 0.7381862504171952111 ) ) ;
#11501=ORIENTED_EDGE ( 'NONE', *, *, #3810, .T. ) ;
#11502=AXIS2_PLACEMENT_3D ( 'NONE', #24963, #24625, #39588 ) ;
#11505=VERTEX_POINT ( 'NONE', #28808 ) ;
#11508=CARTESIAN_POINT ( 'NONE',  ( 37.00000000000000711, 6.265926637539651622, 11.10408318471052347 ) ) ;
#11511=ORIENTED_EDGE ( 'NONE', *, *, #3144, .T. ) ;
#11512=DIRECTION ( 'NONE',  ( -1.000000000000000000, 0.000000000000000000, -0.000000000000000000 ) ) ;
#11514=FACE_BOUND ( 'NONE', #28244, .T. ) ;
#11515=ORIENTED_EDGE ( 'NONE', *, *, #48571, .F. ) ;
#11516=VERTEX_POINT ( 'NONE', #9170 ) ;
#11518=ORIENTED_EDGE ( 'NONE', *, *, #45855, .T. ) ;
#11520=LINE ( 'NONE', #41785, #35248 ) ;
#11521=LINE ( 'NONE', #52102, #53291 ) ;
#11522=DIRECTION ( 'NONE',  ( 0.000000000000000000, 0.01356324068817998940, -0.9999080150203990547 ) ) ;
#11525=AXIS2_PLACEMENT_3D ( 'NONE', #8607, #33562, #38544 ) ;
#11526=DIRECTION ( 'NONE',  ( 1.000000000000000000, 0.000000000000000000, 0.000000000000000000 ) ) ;
#11528=DIRECTION ( 'NONE',  ( 1.000000000000000000, 0.000000000000000000, 0.000000000000000000 ) ) ;
#11529=AXIS2_PLACEMENT_3D ( 'NONE', #43018, #52027, #48024 ) ;
#11530=ORIENTED_EDGE ( 'NONE', *, *, #21895, .T. ) ;
#11531=DIRECTION ( 'NONE',  ( 1.000000000000000000, 0.000000000000000000, -0.000000000000000000 ) ) ;
#11532=CARTESIAN_POINT ( 'NONE',  ( 35.00000000000000000, 7.474872387601131152, 9.060822531525964507 ) ) ;
#11533=DIRECTION ( 'NONE',  ( 0.000000000000000000, -0.01356324068817998940, 0.9999080150203990547 ) ) ;
#11534=DIRECTION ( 'NONE',  ( 1.000000000000000000, 0.000000000000000000, -0.000000000000000000 ) ) ;
#11536=EDGE_CURVE ( 'NONE', #62548, #33917, #27940, .T. ) ;
#11537=CARTESIAN_POINT ( 'NONE',  ( -37.00000000000000711, -11.78745411414837818, -3.093009498344053032 ) ) ;
#11540=ORIENTED_EDGE ( 'NONE', *, *, #58947, .T. ) ;
#11541=EDGE_CURVE ( 'NONE', #46746, #43998, #19497, .T. ) ;
#11543=B_SPLINE_CURVE_WITH_KNOTS ( 'NONE', 3,
 ( #24449, #65012, #30429, #14464, #40393, #9471, #30103, #65656, #12709, #48648, #29016, #23362, #23707, #2785, #32994, #63919, #3770, #58968, #53956, #19032, #18397, #33664 ),
 .UNSPECIFIED., .F., .F.,
 ( 4, 2, 2, 2, 2, 2, 2, 2, 2, 2, 4 ),
 ( 0.000000000000000000, 0.001345449967898921465, 0.002018174951848381981, 0.002690899935797842930, 0.004036349903696756156, 0.004709074887646215804, 0.005381799871595674585, 0.006727249839494598219, 0.008072699807393519250, 0.009418149775292443751, 0.01076359974319136478 ),
 .UNSPECIFIED. ) ;
#11545=ORIENTED_EDGE ( 'NONE', *, *, #61493, .F. ) ;
#11546=CARTESIAN_POINT ( 'NONE',  ( -35.00000000000000000, -6.917234959366895808, 9.493370459201672773 ) ) ;
#11547=DIRECTION ( 'NONE',  ( -1.000000000000000000, 0.000000000000000000, 0.000000000000000000 ) ) ;
#11548=CIRCLE ( 'NONE', #40211, 4.999999999999998224 ) ;
#11551=ADVANCED_FACE ( 'NONE', ( #24809 ), #45092, .T. ) ;
#11553=CARTESIAN_POINT ( 'NONE',  ( 34.00000000000000000, -14.99999999999997513, 0.000000000000000000 ) ) ;
#11556=AXIS2_PLACEMENT_3D ( 'NONE', #65349, #40070, #35416 ) ;
#11558=CYLINDRICAL_SURFACE ( 'NONE', #56433, 5.000000000000000888 ) ;
#11560=VERTEX_POINT ( 'NONE', #40080 ) ;
#11563=DIRECTION ( 'NONE',  ( -1.000000000000000000, 0.000000000000000000, 0.000000000000000000 ) ) ;
#11564=FACE_OUTER_BOUND ( 'NONE', #44710, .T. ) ;
#11565=CARTESIAN_POINT ( 'NONE',  ( -37.00000000000000711, 9.926225166347114381, -6.280308599560036065 ) ) ;
#11567=CARTESIAN_POINT ( 'NONE',  ( -9.480571072184686088, -3.591719512060966402, 11.45094271422924415 ) ) ;
#11568=EDGE_CURVE ( 'NONE', #10423, #9409, #3570, .T. ) ;
#11569=CIRCLE ( 'NONE', #34905, 5.000000000000000000 ) ;
#11571=EDGE_LOOP ( 'NONE', ( #57072, #57301, #51841, #14954, #43242, #9353 ) ) ;
#11572=CARTESIAN_POINT ( 'NONE',  ( -30.14922989771758566, -0.5076506010579284744, 11.99141041789170892 ) ) ;
#11573=EDGE_CURVE ( 'NONE', #16668, #41187, #7775, .T. ) ;
#11574=ORIENTED_EDGE ( 'NONE', *, *, #21521, .T. ) ;
#11575=CARTESIAN_POINT ( 'NONE',  ( 3.441315431463302765, 6.040220126836617354, 10.37118595071527594 ) ) ;
#11577=DIRECTION ( 'NONE',  ( 0.000000000000000000, 0.4698238015817302604, 0.8827602140260348840 ) ) ;
#11581=EDGE_CURVE ( 'NONE', #17960, #61044, #4543, .T. ) ;
#11582=DIRECTION ( 'NONE',  ( 1.000000000000000000, 0.000000000000000000, 0.000000000000000000 ) ) ;
#11583=CARTESIAN_POINT ( 'NONE',  ( -6.748373723087907727, -1.202078537604638342, 11.93986841932145104 ) ) ;
#11584=VERTEX_POINT ( 'NONE', #39103 ) ;
#11586=VERTEX_POINT ( 'NONE', #4197 ) ;
#11587=LINE ( 'NONE', #65237, #523 ) ;
#11589=CARTESIAN_POINT ( 'NONE',  ( -47.00000000000000711, 0.000000000000000000, 0.000000000000000000 ) ) ;
#11591=CARTESIAN_POINT ( 'NONE',  ( 37.00000000000000711, 10.23119532541072552, -7.608228585767763619 ) ) ;
#11592=AXIS2_PLACEMENT_3D ( 'NONE', #29542, #8958, #19263 ) ;
#11593=ORIENTED_EDGE ( 'NONE', *, *, #43608, .F. ) ;
#11594=DIRECTION ( 'NONE',  ( 0.000000000000000000, -0.4380125133593850140, 0.8989688749565217796 ) ) ;
#11596=CARTESIAN_POINT ( 'NONE',  ( 35.00000000000000000, -10.43555801961471552, 5.391785509271064925 ) ) ;
#11598=ORIENTED_EDGE ( 'NONE', *, *, #61393, .F. ) ;
#11599=DIRECTION ( 'NONE',  ( -1.000000000000000000, -0.000000000000000000, 0.000000000000000000 ) ) ;
#11600=ORIENTED_EDGE ( 'NONE', *, *, #44574, .F. ) ;
#11601=ORIENTED_EDGE ( 'NONE', *, *, #47085, .F. ) ;
#11605=ORIENTED_EDGE ( 'NONE', *, *, #22826, .T. ) ;
#11607=FACE_OUTER_BOUND ( 'NONE', #4558, .T. ) ;
#11608=ADVANCED_FACE ( 'NONE', ( #39767 ), #60710, .T. ) ;
#11610=LINE ( 'NONE', #31880, #12830 ) ;
#11611=CARTESIAN_POINT ( 'NONE',  ( 37.00000000000000711, 4.705694406421931860E-17, -3.469127814946512892E-15 ) ) ;
#11613=CARTESIAN_POINT ( 'NONE',  ( -37.00000000000000711, 0.000000000000000000, 0.000000000000000000 ) ) ;
#11616=CARTESIAN_POINT ( 'NONE',  ( -10.79842706929647989, -9.842369975612385247, -9.240427863961665267 ) ) ;
#11623=CIRCLE ( 'NONE', #23310, 12.75000000000000178 ) ;
#11626=AXIS2_PLACEMENT_3D ( 'NONE', #21350, #7355, #27312 ) ;
#11627=ORIENTED_EDGE ( 'NONE', *, *, #48794, .T. ) ;
#11628=CARTESIAN_POINT ( 'NONE',  ( -35.00000000000000000, 12.63095688309031495, -1.738225594539862584 ) ) ;
#11634=VERTEX_POINT ( 'NONE', #533 ) ;
#11635=CYLINDRICAL_SURFACE ( 'NONE', #30282, 5.000000000000000888 ) ;
#11636=LINE ( 'NONE', #6672, #55671 ) ;
#11637=CARTESIAN_POINT ( 'NONE',  ( 24.82652845881425208, 8.390869743685042792, -8.578654028722157321 ) ) ;
#11638=DIRECTION ( 'NONE',  ( 0.000000000000000000, 0.9105187689795969375, -0.4134677391718481476 ) ) ;
#11639=EDGE_CURVE ( 'NONE', #61418, #24889, #61345, .T. ) ;
#11640=AXIS2_PLACEMENT_3D ( 'NONE', #44947, #29326, #14658 ) ;
#11643=( BOUNDED_CURVE ( )  B_SPLINE_CURVE ( 3, ( #46877, #62167, #11616, #31886 ),
 .UNSPECIFIED., .F., .F. ) 
 B_SPLINE_CURVE_WITH_KNOTS ( ( 4, 4 ),
 ( 5.516275288668797572, 5.535842959799285090 ),
 .UNSPECIFIED. ) 
 CURVE ( )  GEOMETRIC_REPRESENTATION_ITEM ( )  RATIONAL_B_SPLINE_CURVE ( ( 1.000000000000000000, 0.9999680924417370109, 0.9999680924417370109, 1.000000000000000000 ) ) 
 REPRESENTATION_ITEM ( '' )  );
#11644=VERTEX_POINT ( 'NONE', #46718 ) ;
#11646=FACE_OUTER_BOUND ( 'NONE', #10791, .T. ) ;
#11647=CIRCLE ( 'NONE', #49922, 12.18649999999999878 ) ;
#11648=EDGE_CURVE ( 'NONE', #63071, #16758, #2514, .T. ) ;
#11649=ORIENTED_EDGE ( 'NONE', *, *, #34099, .T. ) ;
#11651=ORIENTED_EDGE ( 'NONE', *, *, #38039, .F. ) ;
#11653=CARTESIAN_POINT ( 'NONE',  ( 37.00000000000000711, -7.376655759824808811, 9.700295462048739381 ) ) ;
#11654=CYLINDRICAL_SURFACE ( 'NONE', #19468, 12.18650000000000055 ) ;
#11655=DIRECTION ( 'NONE',  ( -1.000000000000000000, 0.000000000000000000, -0.000000000000000000 ) ) ;
#11656=ORIENTED_EDGE ( 'NONE', *, *, #47928, .F. ) ;
#11658=EDGE_LOOP ( 'NONE', ( #36696, #64405, #44353, #10488 ) ) ;
#11659=LINE ( 'NONE', #52256, #2610 ) ;
#11661=CARTESIAN_POINT ( 'NONE',  ( -27.01437459610461644, 13.31613970204373132, -2.220455681983952267 ) ) ;
#11662=ORIENTED_EDGE ( 'NONE', *, *, #38114, .T. ) ;
#11664=DIRECTION ( 'NONE',  ( 1.000000000000000000, 0.000000000000000000, 0.000000000000000000 ) ) ;
#11665=FACE_OUTER_BOUND ( 'NONE', #35589, .T. ) ;
#11666=ORIENTED_EDGE ( 'NONE', *, *, #39350, .T. ) ;
#11668=CYLINDRICAL_SURFACE ( 'NONE', #55175, 12.18650000000000055 ) ;
#11670=ORIENTED_EDGE ( 'NONE', *, *, #48480, .F. ) ;
#11671=CARTESIAN_POINT ( 'NONE',  ( -35.00000000000000000, 11.61175578952786047, 1.771820996347196697 ) ) ;
#11672=ORIENTED_EDGE ( 'NONE', *, *, #42860, .T. ) ;
#11676=DIRECTION ( 'NONE',  ( 1.000000000000000000, 0.000000000000000000, 0.000000000000000000 ) ) ;
#11677=CYLINDRICAL_SURFACE ( 'NONE', #60583, 5.000000000000000888 ) ;
#11678=FACE_OUTER_BOUND ( 'NONE', #61004, .T. ) ;
#11680=ORIENTED_EDGE ( 'NONE', *, *, #17039, .T. ) ;
#11682=DIRECTION ( 'NONE',  ( 0.000000000000000000, -0.01356324068817991828, 0.9999080150203990547 ) ) ;
#11683=EDGE_CURVE ( 'NONE', #64921, #29384, #16357, .T. ) ;
#11684=VERTEX_POINT ( 'NONE', #56036 ) ;
#11686=CARTESIAN_POINT ( 'NONE',  ( -35.00000000000000000, 3.614449339633491576, 11.17622378668007777 ) ) ;
#11687=ORIENTED_EDGE ( 'NONE', *, *, #28170, .T. ) ;
#11688=CARTESIAN_POINT ( 'NONE',  ( -18.58686583997218378, 5.413691226207714813, 10.71337495308983634 ) ) ;
#11690=AXIS2_PLACEMENT_3D ( 'NONE', #30251, #60175, #29914 ) ;
#11691=CARTESIAN_POINT ( 'NONE',  ( -37.00000000000000711, 12.42372387097882580, 2.865935305911671449 ) ) ;
#11692=ORIENTED_EDGE ( 'NONE', *, *, #18030, .F. ) ;
#11693=ADVANCED_FACE ( 'NONE', ( #20800 ), #30346, .T. ) ;
#11694=ORIENTED_EDGE ( 'NONE', *, *, #63719, .F. ) ;
#11695=DIRECTION ( 'NONE',  ( 0.000000000000000000, -0.3554799084908835116, -0.9346839223284592046 ) ) ;
#11696=VERTEX_POINT ( 'NONE', #9380 ) ;
#11697=DIRECTION ( 'NONE',  ( -1.000000000000000000, 0.000000000000000000, -0.000000000000000000 ) ) ;
#11701=ORIENTED_EDGE ( 'NONE', *, *, #22336, .F. ) ;
#11704=VECTOR ( 'NONE', #10914, 1000.000000000000000 ) ;
#11705=CIRCLE ( 'NONE', #31882, 12.18650000000000055 ) ;
#11706=CARTESIAN_POINT ( 'NONE',  ( 26.08439714455133185, 12.97057518889166516, 3.743551691817328386 ) ) ;
#11708=CARTESIAN_POINT ( 'NONE',  ( 11.86852745065355208, 10.64790170674535474, -8.300198448557052799 ) ) ;
#11709=DIRECTION ( 'NONE',  ( 0.000000000000000000, -0.01356324068817992175, 0.9999080150203990547 ) ) ;
#11710=CARTESIAN_POINT ( 'NONE',  ( -47.00000000000000711, 0.000000000000000000, 0.000000000000000000 ) ) ;
#11711=DIRECTION ( 'NONE',  ( 0.000000000000000000, 0.01356324068817998940, -0.9999080150203990547 ) ) ;
#11713=AXIS2_PLACEMENT_3D ( 'NONE', #26083, #41688, #60662 ) ;
#11714=EDGE_CURVE ( 'NONE', #16892, #41673, #61922, .T. ) ;
#11715=ORIENTED_EDGE ( 'NONE', *, *, #53495, .F. ) ;
#11718=ORIENTED_EDGE ( 'NONE', *, *, #35490, .T. ) ;
#11724=VECTOR ( 'NONE', #52754, 1000.000000000000000 ) ;
#11725=CARTESIAN_POINT ( 'NONE',  ( 37.00000000000000711, -8.854740511458901508, -7.717887834988215623 ) ) ;
#11726=VERTEX_POINT ( 'NONE', #44982 ) ;
#11728=EDGE_CURVE ( 'NONE', #34225, #786, #19728, .T. ) ;
#11730=ORIENTED_EDGE ( 'NONE', *, *, #30714, .F. ) ;
#11733=CARTESIAN_POINT ( 'NONE',  ( 35.00000000000000000, 8.699265615723106748, 8.534258022645994757 ) ) ;
#11734=VECTOR ( 'NONE', #15025, 1000.000000000000000 ) ;
#11737=CARTESIAN_POINT ( 'NONE',  ( -4.984431264850669230, -1.083143072858141487, -11.95218935805936056 ) ) ;
#11740=CARTESIAN_POINT ( 'NONE',  ( -26.75731680663163559, 10.79779643724861593, 5.235948385342425127 ) ) ;
#11741=ORIENTED_EDGE ( 'NONE', *, *, #23124, .F. ) ;
#11743=CIRCLE ( 'NONE', #20250, 12.18650000000000055 ) ;
#11744=EDGE_LOOP ( 'NONE', ( #39629, #508, #9611, #45062 ) ) ;
#11746=VERTEX_POINT ( 'NONE', #20037 ) ;
#11747=CARTESIAN_POINT ( 'NONE',  ( -35.00000000000000000, -8.766823244862047559, 7.817610399097479679 ) ) ;
#11748=DIRECTION ( 'NONE',  ( 0.000000000000000000, 0.01356324068817998940, -0.9999080150203990547 ) ) ;
#11750=CIRCLE ( 'NONE', #56375, 5.000000000000000000 ) ;
#11751=ORIENTED_EDGE ( 'NONE', *, *, #55046, .T. ) ;
#11752=CARTESIAN_POINT ( 'NONE',  ( -35.00000000000000000, 11.86701198550360203, -2.772148766915989881 ) ) ;
#11753=CIRCLE ( 'NONE', #14921, 12.18650000000000055 ) ;
#11755=CARTESIAN_POINT ( 'NONE',  ( 36.00000000000000711, 9.506317355798490354, 8.496612874013054650 ) ) ;
#11756=ORIENTED_EDGE ( 'NONE', *, *, #18933, .F. ) ;
#11758=VERTEX_POINT ( 'NONE', #65262 ) ;
#11761=ORIENTED_EDGE ( 'NONE', *, *, #19065, .F. ) ;
#11763=ORIENTED_EDGE ( 'NONE', *, *, #46297, .F. ) ;
#11764=CARTESIAN_POINT ( 'NONE',  ( 19.28625800530497258, -6.413918128308385036, 11.87904264843581537 ) ) ;
#11765=CARTESIAN_POINT ( 'NONE',  ( -35.00000000000000000, -7.499679039484122178, 9.040300684349668714 ) ) ;
#11769=DIRECTION ( 'NONE',  ( 1.000000000000000000, 0.000000000000000000, -0.000000000000000000 ) ) ;
#11770=EDGE_CURVE ( 'NONE', #25415, #55675, #34344, .T. ) ;
#11771=CARTESIAN_POINT ( 'NONE',  ( -35.00000000000000000, 0.000000000000000000, 0.000000000000000000 ) ) ;
#11772=VECTOR ( 'NONE', #50257, 1000.000000000000000 ) ;
#11773=AXIS2_PLACEMENT_3D ( 'NONE', #944, #21565, #27195 ) ;
#11775=AXIS2_PLACEMENT_3D ( 'NONE', #65783, #5303, #45866 ) ;
#11777=EDGE_CURVE ( 'NONE', #18204, #26747, #50319, .T. ) ;
#11778=DIRECTION ( 'NONE',  ( 1.000000000000000000, 0.000000000000000000, 0.000000000000000000 ) ) ;
#11779=VECTOR ( 'NONE', #47931, 1000.000000000000000 ) ;
#11780=CARTESIAN_POINT ( 'NONE',  ( 35.00000000000000000, -12.16632754454236043, 0.7008968033240018380 ) ) ;
#11781=FACE_OUTER_BOUND ( 'NONE', #15660, .T. ) ;
#11783=AXIS2_PLACEMENT_3D ( 'NONE', #39578, #34579, #4692 ) ;
#11784=FACE_OUTER_BOUND ( 'NONE', #55099, .T. ) ;
#11785=AXIS2_PLACEMENT_3D ( 'NONE', #38734, #54368, #2525 ) ;
#11786=ORIENTED_EDGE ( 'NONE', *, *, #43914, .T. ) ;
#11788=CARTESIAN_POINT ( 'NONE',  ( 47.00000000000000711, 4.705694406421931860E-17, -3.469127814946512892E-15 ) ) ;
#11790=CARTESIAN_POINT ( 'NONE',  ( -25.86628395826706850, -5.139808748864358456, 10.84354029019568522 ) ) ;
#11791=AXIS2_PLACEMENT_3D ( 'NONE', #40338, #35680, #36348 ) ;
#11792=AXIS2_PLACEMENT_3D ( 'NONE', #52636, #2073, #7374 ) ;
#11793=CIRCLE ( 'NONE', #57492, 5.000000000000000888 ) ;
#11794=CARTESIAN_POINT ( 'NONE',  ( -25.10197438393668889, 9.577105551445603382, 7.239297392635676509 ) ) ;
#11795=CARTESIAN_POINT ( 'NONE',  ( -25.13764408299829256, -11.42471432779190188, 7.193830867856458866 ) ) ;
#11796=EDGE_LOOP ( 'NONE', ( #3766, #16075, #61722, #4036 ) ) ;
#11797=CARTESIAN_POINT ( 'NONE',  ( 35.00000000000000000, -7.971186206369405447, 9.217970097227802029 ) ) ;
#11798=DIRECTION ( 'NONE',  ( 0.000000000000000000, 0.9847383929261623869, -0.1740410799127578845 ) ) ;
#11801=ORIENTED_EDGE ( 'NONE', *, *, #63896, .T. ) ;
#11803=CARTESIAN_POINT ( 'NONE',  ( -35.00000000000000000, 0.000000000000000000, 0.000000000000000000 ) ) ;
#11805=ORIENTED_EDGE ( 'NONE', *, *, #4975, .F. ) ;
#11806=CARTESIAN_POINT ( 'NONE',  ( 37.00000000000000711, 5.246972444134017977, -10.99909370905159101 ) ) ;
#11807=AXIS2_PLACEMENT_3D ( 'NONE', #18509, #7501, #43742 ) ;
#11808=ADVANCED_FACE ( 'NONE', ( #34973 ), #4775, .F. ) ;
#11809=VECTOR ( 'NONE', #36984, 1000.000000000000000 ) ;
#11811=ORIENTED_EDGE ( 'NONE', *, *, #7151, .F. ) ;
#11812=CIRCLE ( 'NONE', #5497, 4.999999999999999112 ) ;
#11813=CARTESIAN_POINT ( 'NONE',  ( 35.00000000000000000, -4.946702696913249042, -11.13736569743272753 ) ) ;
#11814=CYLINDRICAL_SURFACE ( 'NONE', #64380, 5.000000000000000888 ) ;
#11816=DIRECTION ( 'NONE',  ( 0.000000000000000000, -0.01356324068817999114, 0.9999080150203989437 ) ) ;
#11817=CARTESIAN_POINT ( 'NONE',  ( -3.570318967459569226, -9.097864018429371313, 9.981632988681457874 ) ) ;
#11820=DIRECTION ( 'NONE',  ( -1.000000000000000000, 0.000000000000000000, 0.000000000000000000 ) ) ;
#11821=DIRECTION ( 'NONE',  ( -1.000000000000000000, -0.000000000000000000, 0.000000000000000000 ) ) ;
#11822=ORIENTED_EDGE ( 'NONE', *, *, #28978, .F. ) ;
#11824=EDGE_LOOP ( 'NONE', ( #5612, #29734, #54369, #3560 ) ) ;
#11825=CARTESIAN_POINT ( 'NONE',  ( -35.00000000000000000, 1.771820996347319710, -11.61175578952784448 ) ) ;
#11826=EDGE_LOOP ( 'NONE', ( #22579, #19529, #4422, #48621 ) ) ;
#11828=DIRECTION ( 'NONE',  ( 0.000000000000000000, -0.01356324068817991828, 0.9999080150203990547 ) ) ;
#11829=DIRECTION ( 'NONE',  ( -1.000000000000000000, -0.000000000000000000, -0.000000000000000000 ) ) ;
#11830=ADVANCED_FACE ( 'NONE', ( #35315 ), #55627, .T. ) ;
#11831=DIRECTION ( 'NONE',  ( 0.000000000000000000, 0.9105187689795940509, -0.4134677391718546424 ) ) ;
#11832=ORIENTED_EDGE ( 'NONE', *, *, #41570, .T. ) ;
#11834=CARTESIAN_POINT ( 'NONE',  ( -36.00000000000000711, 12.68495603654572079, 1.286231064351356368 ) ) ;
#11836=ADVANCED_FACE ( 'NONE', ( #25328 ), #21322, .T. ) ;
#11837=DIRECTION ( 'NONE',  ( -1.000000000000000000, 0.000000000000000000, 0.000000000000000000 ) ) ;
#11838=ORIENTED_EDGE ( 'NONE', *, *, #16393, .F. ) ;
#11839=ORIENTED_EDGE ( 'NONE', *, *, #13570, .F. ) ;
#11841=CIRCLE ( 'NONE', #40511, 5.000000000000000000 ) ;
#11844=DIRECTION ( 'NONE',  ( 0.000000000000000000, -0.9987865678893282917, 0.04924826701373502535 ) ) ;
#11846=CARTESIAN_POINT ( 'NONE',  ( 12.03537186402451731, 0.5714996694917733322, 13.48808163914964808 ) ) ;
#11847=CARTESIAN_POINT ( 'NONE',  ( -37.00000000000000711, -1.457575200925635528, 12.66641127287625501 ) ) ;
#11848=CIRCLE ( 'NONE', #62835, 12.18649999999999878 ) ;
#11851=CARTESIAN_POINT ( 'NONE',  ( 26.08439714455133185, -11.40113243194250359, 3.743551691817327942 ) ) ;
#11854=ORIENTED_EDGE ( 'NONE', *, *, #60423, .T. ) ;
#11858=CARTESIAN_POINT ( 'NONE',  ( 36.00000000000000711, 10.59380114696469910, -7.094637218249395971 ) ) ;
#11860=FACE_OUTER_BOUND ( 'NONE', #25125, .T. ) ;
#11861=CARTESIAN_POINT ( 'NONE',  ( -37.00000000000000711, -9.908974237959601084, -6.307491713049132365 ) ) ;
#11862=CARTESIAN_POINT ( 'NONE',  ( -17.71317172853713373, 11.35466418304649139, 3.882258812239216095 ) ) ;
#11863=CYLINDRICAL_SURFACE ( 'NONE', #37216, 12.18650000000000055 ) ;
#11864=ORIENTED_EDGE ( 'NONE', *, *, #4744, .F. ) ;
#11865=CIRCLE ( 'NONE', #205, 5.000000000000000000 ) ;
#11866=EDGE_LOOP ( 'NONE', ( #47189, #2003, #16445, #35869 ) ) ;
#11867=CARTESIAN_POINT ( 'NONE',  ( -35.00000000000000000, 1.171570255487447643, 11.68758509253248867 ) ) ;
#11868=VECTOR ( 'NONE', #22427, 1000.000000000000000 ) ;
#11869=EDGE_CURVE ( 'NONE', #12850, #10311, #13085, .T. ) ;
#11870=ORIENTED_EDGE ( 'NONE', *, *, #53758, .F. ) ;
#11872=DIRECTION ( 'NONE',  ( -1.000000000000000000, 0.000000000000000000, -0.000000000000000000 ) ) ;
#11874=EDGE_CURVE ( 'NONE', #9962, #47648, #10354, .T. ) ;
#11878=DIRECTION ( 'NONE',  ( 0.000000000000000000, -0.01356324068817998940, 0.9999080150203990547 ) ) ;
#11879=DIRECTION ( 'NONE',  ( 1.000000000000000000, 0.000000000000000000, 0.000000000000000000 ) ) ;
#11882=DIRECTION ( 'NONE',  ( -0.000000000000000000, -1.000000000000000000, -0.000000000000000000 ) ) ;
#11883=CARTESIAN_POINT ( 'NONE',  ( 9.687175622948609899, -11.98570860552670325, -0.5854820436212360146 ) ) ;
#11884=EDGE_LOOP ( 'NONE', ( #51710, #58521, #29911, #45842 ) ) ;
#11886=ORIENTED_EDGE ( 'NONE', *, *, #14272, .F. ) ;
#11887=DIRECTION ( 'NONE',  ( 1.000000000000000000, 0.000000000000000000, 0.000000000000000000 ) ) ;
#11888=DIRECTION ( 'NONE',  ( -1.000000000000000000, 0.000000000000000000, 0.000000000000000000 ) ) ;
#11891=CARTESIAN_POINT ( 'NONE',  ( -29.73183716147547173, 1.699799061024255264, -13.39970470410835368 ) ) ;
#11892=DIRECTION ( 'NONE',  ( -0.000000000000000000, -1.000000000000000000, -0.000000000000000000 ) ) ;
#11896=AXIS2_PLACEMENT_3D ( 'NONE', #19237, #9554, #10228 ) ;
#11897=EDGE_LOOP ( 'NONE', ( #7877, #25535, #38672, #14922 ) ) ;
#11898=VERTEX_POINT ( 'NONE', #37266 ) ;
#11899=DIRECTION ( 'NONE',  ( -1.000000000000000000, 0.000000000000000000, 0.000000000000000000 ) ) ;
#11900=ORIENTED_EDGE ( 'NONE', *, *, #47778, .T. ) ;
#11902=FACE_OUTER_BOUND ( 'NONE', #2379, .T. ) ;
#11903=CARTESIAN_POINT ( 'NONE',  ( -35.00000000000000000, -2.544412758415929066, 11.91791701451265340 ) ) ;
#11905=CYLINDRICAL_SURFACE ( 'NONE', #7794, 5.000000000000000888 ) ;
#11907=CARTESIAN_POINT ( 'NONE',  ( -4.989057617119011745, -0.9162120371760335003, 11.96497202265570259 ) ) ;
#11909=ADVANCED_FACE ( 'NONE', ( #2720 ), #47582, .T. ) ;
#11910=LINE ( 'NONE', #57825, #7654 ) ;
#11912=CARTESIAN_POINT ( 'NONE',  ( 35.00000000000000000, 4.705694406421931860E-17, -3.469127814946512892E-15 ) ) ;
#11913=CIRCLE ( 'NONE', #46966, 4.999999999999999112 ) ;
#11915=EDGE_CURVE ( 'NONE', #19302, #47299, #63511, .T. ) ;
#11917=VERTEX_POINT ( 'NONE', #47916 ) ;
#11918=DIRECTION ( 'NONE',  ( 0.000000000000000000, 0.01356324068817998940, -0.9999080150203990547 ) ) ;
#11919=AXIS2_PLACEMENT_3D ( 'NONE', #29910, #50216, #65786 ) ;
#11922=ORIENTED_EDGE ( 'NONE', *, *, #8273, .T. ) ;
#11924=VERTEX_POINT ( 'NONE', #26980 ) ;
#11925=CARTESIAN_POINT ( 'NONE',  ( -17.08907783926314394, 2.790822428529209809, -11.67174978956914089 ) ) ;
#11933=FACE_OUTER_BOUND ( 'NONE', #12681, .T. ) ;
#11935=CARTESIAN_POINT ( 'NONE',  ( -7.489022030332961322, 25.00000000000000000, -10.84914964302385521 ) ) ;
#11938=AXIS2_PLACEMENT_3D ( 'NONE', #39676, #16295, #1339 ) ;
#11940=LINE ( 'NONE', #37550, #2016 ) ;
#11941=ADVANCED_FACE ( 'NONE', ( #17981 ), #57240, .T. ) ;
#11944=EDGE_CURVE ( 'NONE', #30241, #23572, #63197, .T. ) ;
#11946=CARTESIAN_POINT ( 'NONE',  ( -35.00000000000000000, 8.854740511458851770, 7.717887834988275131 ) ) ;
#11947=CARTESIAN_POINT ( 'NONE',  ( -35.00000000000000000, 5.672855678558835102, -10.28547182238001767 ) ) ;
#11950=AXIS2_PLACEMENT_3D ( 'NONE', #10906, #17209, #6258 ) ;
#11951=EDGE_LOOP ( 'NONE', ( #38503, #63863, #6623, #46467 ) ) ;
#11953=EDGE_CURVE ( 'NONE', #23142, #58933, #58218, .T. ) ;
#11954=EDGE_LOOP ( 'NONE', ( #64322, #17310, #24125, #25529 ) ) ;
#11955=DIRECTION ( 'NONE',  ( 1.000000000000000000, 0.000000000000000000, 0.000000000000000000 ) ) ;
#11956=CARTESIAN_POINT ( 'NONE',  ( 37.00000000000000711, -1.488153103996881610, 11.65150730582935701 ) ) ;
#11959=DIRECTION ( 'NONE',  ( 1.000000000000000000, 0.000000000000000000, 0.000000000000000000 ) ) ;
#11960=CARTESIAN_POINT ( 'NONE',  ( 37.00000000000000711, -12.31350058095520339, 3.307597835713371737 ) ) ;
#11961=ORIENTED_EDGE ( 'NONE', *, *, #8732, .T. ) ;
#11963=DIRECTION ( 'NONE',  ( -1.000000000000000000, 0.000000000000000000, 0.000000000000000000 ) ) ;
#11965=CARTESIAN_POINT ( 'NONE',  ( -3.229081750799087214, 8.212677051982280929, 10.74170107049143397 ) ) ;
#11966=AXIS2_PLACEMENT_3D ( 'NONE', #50199, #55165, #10262 ) ;
#11968=AXIS2_PLACEMENT_3D ( 'NONE', #52261, #13317, #57907 ) ;
#11973=B_SPLINE_CURVE_WITH_KNOTS ( 'NONE', 3,
 ( #61450, #31218, #17235, #1298, #26881, #5971, #1627, #21901, #37509, #26227, #62434, #16896 ),
 .UNSPECIFIED., .F., .F.,
 ( 4, 2, 2, 2, 2, 4 ),
 ( 0.000000000000000000, 0.002493599491187762762, 0.004987198982375525523, 0.006233998727969406253, 0.007480798473563286116, 0.009974397964751049311 ),
 .UNSPECIFIED. ) ;
#11974=ADVANCED_FACE ( 'NONE', ( #58563 ), #12989, .T. ) ;
#11975=VERTEX_POINT ( 'NONE', #21674 ) ;
#11976=EDGE_CURVE ( 'NONE', #40181, #55613, #41929, .T. ) ;
#11977=VERTEX_POINT ( 'NONE', #59865 ) ;
#11978=CARTESIAN_POINT ( 'NONE',  ( 36.00000000000000711, 12.68495603654573500, 1.286231064351171627 ) ) ;
#11980=CARTESIAN_POINT ( 'NONE',  ( -35.00000000000000000, 0.000000000000000000, 0.000000000000000000 ) ) ;
#11981=FACE_OUTER_BOUND ( 'NONE', #25147, .T. ) ;
#11982=ORIENTED_EDGE ( 'NONE', *, *, #7833, .T. ) ;
#11984=EDGE_CURVE ( 'NONE', #56228, #18427, #8902, .T. ) ;
#11985=AXIS2_PLACEMENT_3D ( 'NONE', #55767, #55433, #40452 ) ;
#11987=ORIENTED_EDGE ( 'NONE', *, *, #59862, .F. ) ;
#11989=AXIS2_PLACEMENT_3D ( 'NONE', #849, #21115, #41391 ) ;
#11990=CYLINDRICAL_SURFACE ( 'NONE', #61880, 12.74999999999999822 ) ;
#11991=VECTOR ( 'NONE', #41915, 1000.000000000000000 ) ;
#11992=ORIENTED_EDGE ( 'NONE', *, *, #33780, .T. ) ;
#11993=DIRECTION ( 'NONE',  ( -1.000000000000000000, 0.000000000000000000, 0.000000000000000000 ) ) ;
#11995=ORIENTED_EDGE ( 'NONE', *, *, #6724, .T. ) ;
#11997=DIRECTION ( 'NONE',  ( 1.000000000000000000, 0.000000000000000000, 0.000000000000000000 ) ) ;
#11998=CARTESIAN_POINT ( 'NONE',  ( 23.97867415005905656, 2.287513683784789364, 11.78413097500964746 ) ) ;
#11999=ORIENTED_EDGE ( 'NONE', *, *, #19251, .F. ) ;
#12000=AXIS2_PLACEMENT_3D ( 'NONE', #3814, #44645, #65583 ) ;
#12001=CARTESIAN_POINT ( 'NONE',  ( 37.00000000000000711, 4.705694406421931860E-17, -3.469127814946512892E-15 ) ) ;
#12005=CIRCLE ( 'NONE', #20466, 5.000000000000000888 ) ;
#12006=CARTESIAN_POINT ( 'NONE',  ( -18.54402015049394237, -5.053814502618243942, 12.52063007984827614 ) ) ;
#12007=EDGE_CURVE ( 'NONE', #24100, #65334, #44881, .T. ) ;
#12008=DIRECTION ( 'NONE',  ( 0.000000000000000000, -0.01356324068817991828, 0.9999080150203990547 ) ) ;
#12010=CARTESIAN_POINT ( 'NONE',  ( -35.00000000000000000, 12.02534193257726791, -4.237174932027097718 ) ) ;
#12011=CARTESIAN_POINT ( 'NONE',  ( -35.00000000000000000, -11.72397916322012890, 0.7214809346828189307 ) ) ;
#12012=CARTESIAN_POINT ( 'NONE',  ( 8.623514385631457557, 3.166471940042038025, 11.57766326477777064 ) ) ;
#12014=DIRECTION ( 'NONE',  ( 0.000000000000000000, 0.01356324068817998940, -0.9999080150203990547 ) ) ;
#12015=ORIENTED_EDGE ( 'NONE', *, *, #53413, .T. ) ;
#12017=ORIENTED_EDGE ( 'NONE', *, *, #46388, .F. ) ;
#12019=AXIS2_PLACEMENT_3D ( 'NONE', #38181, #28542, #43177 ) ;
#12020=DIRECTION ( 'NONE',  ( -1.000000000000000000, -0.000000000000000000, 0.000000000000000000 ) ) ;
#12024=CARTESIAN_POINT ( 'NONE',  ( -37.00000000000000711, -11.61175578952785159, -1.771820996347277966 ) ) ;
#12025=EDGE_CURVE ( 'NONE', #29943, #26384, #13630, .T. ) ;
#12026=ORIENTED_EDGE ( 'NONE', *, *, #57047, .F. ) ;
#12029=EDGE_CURVE ( 'NONE', #50930, #25928, #14289, .T. ) ;
#12031=ORIENTED_EDGE ( 'NONE', *, *, #18484, .F. ) ;
#12032=CYLINDRICAL_SURFACE ( 'NONE', #47651, 13.50000000000000178 ) ;
#12033=DIRECTION ( 'NONE',  ( 1.000000000000000000, -0.000000000000000000, 0.000000000000000000 ) ) ;
#12035=CARTESIAN_POINT ( 'NONE',  ( 35.00000000000000000, 5.246972444134017977, -10.99909370905159101 ) ) ;
#12039=CIRCLE ( 'NONE', #58781, 4.999999999999999112 ) ;
#12041=AXIS2_PLACEMENT_3D ( 'NONE', #47712, #59023, #23772 ) ;
#12042=CIRCLE ( 'NONE', #20551, 5.000000000000000888 ) ;
#12044=CARTESIAN_POINT ( 'NONE',  ( -27.30975859563925212, -13.34112994997249579, -2.066478916269102406 ) ) ;
#12045=CARTESIAN_POINT ( 'NONE',  ( -37.00000000000000711, -11.66664283989676321, -5.143145423404404504 ) ) ;
#12047=LINE ( 'NONE', #52638, #21122 ) ;
#12048=CARTESIAN_POINT ( 'NONE',  ( 37.00000000000000711, 7.379373053628868639, -10.39746860227893421 ) ) ;
#12051=CIRCLE ( 'NONE', #21620, 12.75000000000000178 ) ;
#12054=CARTESIAN_POINT ( 'NONE',  ( 4.913901985660861449, -9.916373276759339106, 9.161512742702274892 ) ) ;
#12056=ORIENTED_EDGE ( 'NONE', *, *, #3552, .F. ) ;
#12057=LINE ( 'NONE', #42624, #8917 ) ;
#12059=VECTOR ( 'NONE', #23154, 1000.000000000000000 ) ;
#12060=ORIENTED_EDGE ( 'NONE', *, *, #20942, .T. ) ;
#12061=CARTESIAN_POINT ( 'NONE',  ( 35.00000000000000000, 4.705694406421931860E-17, -3.469127814946512892E-15 ) ) ;
#12062=ORIENTED_EDGE ( 'NONE', *, *, #18707, .F. ) ;
#12063=DIRECTION ( 'NONE',  ( -1.000000000000000000, 0.000000000000000000, 0.000000000000000000 ) ) ;
#12064=ORIENTED_EDGE ( 'NONE', *, *, #58178, .F. ) ;
#12065=ORIENTED_EDGE ( 'NONE', *, *, #61498, .F. ) ;
#12067=AXIS2_PLACEMENT_3D ( 'NONE', #6371, #46933, #1394 ) ;
#12069=CARTESIAN_POINT ( 'NONE',  ( -27.09195336418143540, -10.57949983636788716, 5.663524655488941129 ) ) ;
#12071=CARTESIAN_POINT ( 'NONE',  ( 35.00000000000000000, -12.74068829017554094, -0.4871980014161064743 ) ) ;
#12072=CARTESIAN_POINT ( 'NONE',  ( 35.00000000000000000, 4.705694406421931860E-17, -3.469127814946512892E-15 ) ) ;
#12073=ORIENTED_EDGE ( 'NONE', *, *, #49188, .T. ) ;
#12077=DIRECTION ( 'NONE',  ( 0.000000000000000000, -0.07632122047557189648, 0.9970832820307033995 ) ) ;
#12078=ORIENTED_EDGE ( 'NONE', *, *, #40451, .T. ) ;
#12079=DIRECTION ( 'NONE',  ( -1.000000000000000000, -0.000000000000000000, 0.000000000000000000 ) ) ;
#12080=EDGE_CURVE ( 'NONE', #55105, #25248, #20584, .T. ) ;
#12082=AXIS2_PLACEMENT_3D ( 'NONE', #31763, #47423, #32093 ) ;
#12084=CIRCLE ( 'NONE', #26954, 12.74999999999999822 ) ;
#12085=ORIENTED_EDGE ( 'NONE', *, *, #49283, .T. ) ;
#12089=CIRCLE ( 'NONE', #21651, 4.999999999999998224 ) ;
#12091=VERTEX_POINT ( 'NONE', #39562 ) ;
#12094=LINE ( 'NONE', #11755, #47960 ) ;
#12096=ORIENTED_EDGE ( 'NONE', *, *, #41396, .T. ) ;
#12098=VERTEX_POINT ( 'NONE', #48911 ) ;
#12099=CIRCLE ( 'NONE', #49301, 5.000000000000000888 ) ;
#12101=CARTESIAN_POINT ( 'NONE',  ( -36.00000000000000711, -10.12742074351902311, 7.745827850122975811 ) ) ;
#12104=DIRECTION ( 'NONE',  ( -1.000000000000000000, 0.000000000000000000, -0.000000000000000000 ) ) ;
#12107=ADVANCED_FACE ( 'NONE', ( #54865 ), #9288, .T. ) ;
#12108=CIRCLE ( 'NONE', #453, 12.74999999999999822 ) ;
#12109=DIRECTION ( 'NONE',  ( 0.000000000000000000, 0.9718671068226452103, -0.2355298848897551256 ) ) ;
#12110=FACE_OUTER_BOUND ( 'NONE', #59932, .T. ) ;
#12111=ORIENTED_EDGE ( 'NONE', *, *, #29388, .F. ) ;
#12115=EDGE_CURVE ( 'NONE', #10957, #35285, #30249, .T. ) ;
#12117=CARTESIAN_POINT ( 'NONE',  ( 35.00000000000000000, -9.733281772932100395, 8.235637554476742395 ) ) ;
#12119=CARTESIAN_POINT ( 'NONE',  ( 35.00000000000000000, 9.677500615117898164, -6.657191900728355094 ) ) ;
#12120=CARTESIAN_POINT ( 'NONE',  ( 37.00000000000000711, 12.71517666308947980, -0.9416912585474888076 ) ) ;
#12121=CARTESIAN_POINT ( 'NONE',  ( 9.376909970675686878, 1.710254508811689389, -11.87935414277131230 ) ) ;
#12123=VERTEX_POINT ( 'NONE', #40543 ) ;
#12124=CARTESIAN_POINT ( 'NONE',  ( 37.00000000000000711, -9.908974237959688125, -6.307491713048997362 ) ) ;
#12126=DIRECTION ( 'NONE',  ( 0.000000000000000000, 0.5987040770935676548, -0.8009703041134167423 ) ) ;
#12128=AXIS2_PLACEMENT_3D ( 'NONE', #65043, #55406, #19836 ) ;
#12130=CARTESIAN_POINT ( 'NONE',  ( 9.105565894490755596, 3.302923352347424402, -13.09178073503522910 ) ) ;
#12131=DIRECTION ( 'NONE',  ( -1.000000000000000000, 0.000000000000000000, 0.000000000000000000 ) ) ;
#12132=ADVANCED_FACE ( 'NONE', ( #21241 ), #34876, .T. ) ;
#12133=CIRCLE ( 'NONE', #45042, 5.000000000000000888 ) ;
#12135=CYLINDRICAL_SURFACE ( 'NONE', #6804, 12.74999999999999822 ) ;
#12139=EDGE_LOOP ( 'NONE', ( #23301, #7768, #49176, #46433 ) ) ;
#12140=EDGE_CURVE ( 'NONE', #1113, #43258, #4649, .T. ) ;
#12143=VECTOR ( 'NONE', #50339, 1000.000000000000000 ) ;
#12145=VERTEX_POINT ( 'NONE', #24939 ) ;
#12147=VECTOR ( 'NONE', #51880, 1000.000000000000000 ) ;
#12148=ADVANCED_FACE ( 'NONE', ( #51542 ), #50862, .T. ) ;
#12149=PLANE ( 'NONE',  #15990 ) ;
#12150=ORIENTED_EDGE ( 'NONE', *, *, #50672, .F. ) ;
#12152=DIRECTION ( 'NONE',  ( 0.000000000000000000, 0.01356324068817998940, -0.9999080150203990547 ) ) ;
#12153=DIRECTION ( 'NONE',  ( 1.000000000000000000, 0.000000000000000000, 0.000000000000000000 ) ) ;
#12155=CARTESIAN_POINT ( 'NONE',  ( -8.975844149139822647, 7.740763930099402224, -9.178461504936025861 ) ) ;
#12158=CARTESIAN_POINT ( 'NONE',  ( 16.78263030916553333, 10.48479066935627202, 5.836879698929882565 ) ) ;
#12159=EDGE_LOOP ( 'NONE', ( #43513, #4594, #20185, #50163, #30589, #2120 ) ) ;
#12161=EDGE_CURVE ( 'NONE', #58976, #39860, #51874, .T. ) ;
#12163=CARTESIAN_POINT ( 'NONE',  ( 23.95927305399629859, -3.715110391582095328, -11.41482587237507929 ) ) ;
#12164=VERTEX_POINT ( 'NONE', #15276 ) ;
#12166=CARTESIAN_POINT ( 'NONE',  ( -34.00000000000000000, 11.99999999999999822, 0.000000000000000000 ) ) ;
#12167=CARTESIAN_POINT ( 'NONE',  ( -4.023199085832738220, 9.887175217721903664, 6.815337405083463196 ) ) ;
#12171=VERTEX_POINT ( 'NONE', #45526 ) ;
#12173=CARTESIAN_POINT ( 'NONE',  ( 35.00000000000000000, -3.916263239775270577, 11.07407352312216453 ) ) ;
#12177=CIRCLE ( 'NONE', #37674, 12.18649999999999878 ) ;
#12178=VERTEX_POINT ( 'NONE', #51204 ) ;
#12181=CARTESIAN_POINT ( 'NONE',  ( 12.51043786959929704, 0.3316631525046854212, 11.99656223984053760 ) ) ;
#12184=DIRECTION ( 'NONE',  ( -1.000000000000000000, 0.000000000000000000, 0.000000000000000000 ) ) ;
#12188=DIRECTION ( 'NONE',  ( 1.000000000000000000, 0.000000000000000000, 0.000000000000000000 ) ) ;
#12191=CYLINDRICAL_SURFACE ( 'NONE', #44830, 13.50000000000000178 ) ;
#12193=AXIS2_PLACEMENT_3D ( 'NONE', #23653, #13647, #33931 ) ;
#12195=CARTESIAN_POINT ( 'NONE',  ( -27.01437459610461644, 13.31613970204373132, -2.220455681983952267 ) ) ;
#12197=VERTEX_POINT ( 'NONE', #20607 ) ;
#12198=EDGE_CURVE ( 'NONE', #45280, #167, #5989, .T. ) ;
#12199=VERTEX_POINT ( 'NONE', #55851 ) ;
#12203=CARTESIAN_POINT ( 'NONE',  ( 8.437200413559441614, 4.476360154859203355, 11.13383131558893346 ) ) ;
#12206=VERTEX_POINT ( 'NONE', #60836 ) ;
#12207=DIRECTION ( 'NONE',  ( 0.000000000000000000, 0.2960891610144510966, 0.9551603052523478521 ) ) ;
#12209=CARTESIAN_POINT ( 'NONE',  ( -28.41827485489077532, 3.509237424706437292, -13.03592162821790801 ) ) ;
#12211=AXIS2_PLACEMENT_3D ( 'NONE', #5433, #29686, #30365 ) ;
#12212=EDGE_CURVE ( 'NONE', #10842, #19771, #26245, .T. ) ;
#12215=( BOUNDED_CURVE ( )  B_SPLINE_CURVE ( 3, ( #52482, #54439, #64700, #34762 ),
 .UNSPECIFIED., .F., .F. ) 
 B_SPLINE_CURVE_WITH_KNOTS ( ( 4, 4 ),
 ( 4.045341626114011824, 4.054895942073102333 ),
 .UNSPECIFIED. ) 
 CURVE ( )  GEOMETRIC_REPRESENTATION_ITEM ( )  RATIONAL_B_SPLINE_CURVE ( ( 1.000000000000000000, 0.9999923929350129637, 0.9999923929350129637, 1.000000000000000000 ) ) 
 REPRESENTATION_ITEM ( '' )  );
#12216=ADVANCED_FACE ( 'NONE', ( #14595 ), #46519, .T. ) ;
#12220=ORIENTED_EDGE ( 'NONE', *, *, #34931, .T. ) ;
#12221=EDGE_CURVE ( 'NONE', #59141, #40799, #50315, .T. ) ;
#12222=CARTESIAN_POINT ( 'NONE',  ( -6.726017918545671215, -1.195345798906086277, -13.44716762434733681 ) ) ;
#12223=CARTESIAN_POINT ( 'NONE',  ( 37.00000000000000711, -4.946702696913249930, -11.13736569743272931 ) ) ;
#12226=FACE_OUTER_BOUND ( 'NONE', #41959, .T. ) ;
#12228=ORIENTED_EDGE ( 'NONE', *, *, #51005, .F. ) ;
#12229=ADVANCED_FACE ( 'NONE', ( #25923 ), #56504, .T. ) ;
#12230=ORIENTED_EDGE ( 'NONE', *, *, #59724, .F. ) ;
#12235=AXIS2_PLACEMENT_3D ( 'NONE', #42202, #27580, #27261 ) ;
#12236=CARTESIAN_POINT ( 'NONE',  ( 35.00000000000000000, -10.43555801961471552, 5.391785509271064925 ) ) ;
#12238=CARTESIAN_POINT ( 'NONE',  ( 37.00000000000000711, 4.705694406421931860E-17, -3.469127814946512892E-15 ) ) ;
#12243=ORIENTED_EDGE ( 'NONE', *, *, #39840, .F. ) ;
#12245=ORIENTED_EDGE ( 'NONE', *, *, #22517, .T. ) ;
#12247=CARTESIAN_POINT ( 'NONE',  ( -35.00000000000000000, 10.12742074351907462, -7.745827850122902092 ) ) ;
#12248=CARTESIAN_POINT ( 'NONE',  ( 35.00000000000000000, -3.213188559034160452, 11.29812557209479706 ) ) ;
#12253=CARTESIAN_POINT ( 'NONE',  ( 35.00000000000000000, -10.28547182238011715, -5.672855678558653914 ) ) ;
#12254=ORIENTED_EDGE ( 'NONE', *, *, #20797, .F. ) ;
#12255=ORIENTED_EDGE ( 'NONE', *, *, #31359, .F. ) ;
#12256=CARTESIAN_POINT ( 'NONE',  ( 35.00000000000000000, 4.705694406421931860E-17, -3.469127814946512892E-15 ) ) ;
#12257=ORIENTED_EDGE ( 'NONE', *, *, #7061, .T. ) ;
#12258=ORIENTED_EDGE ( 'NONE', *, *, #3565, .T. ) ;
#12261=ORIENTED_EDGE ( 'NONE', *, *, #16220, .F. ) ;
#12264=CIRCLE ( 'NONE', #38803, 12.18649999999999878 ) ;
#12265=DIRECTION ( 'NONE',  ( -1.000000000000000000, -0.000000000000000000, 0.000000000000000000 ) ) ;
#12266=CARTESIAN_POINT ( 'NONE',  ( 35.00000000000000000, -12.12087942037208776, 1.262958560998883595 ) ) ;
#12267=FACE_OUTER_BOUND ( 'NONE', #33248, .T. ) ;
#12268=LINE ( 'NONE', #37203, #2507 ) ;
#12276=EDGE_CURVE ( 'NONE', #57461, #17645, #33304, .T. ) ;
#12278=DIRECTION ( 'NONE',  ( -1.000000000000000000, 0.000000000000000000, 0.000000000000000000 ) ) ;
#12280=VERTEX_POINT ( 'NONE', #12560 ) ;
#12282=DIRECTION ( 'NONE',  ( 1.000000000000000000, -0.000000000000000000, 0.000000000000000000 ) ) ;
#12283=CARTESIAN_POINT ( 'NONE',  ( -35.00000000000000000, 0.000000000000000000, 0.000000000000000000 ) ) ;
#12285=VERTEX_POINT ( 'NONE', #1315 ) ;
#12286=EDGE_CURVE ( 'NONE', #39344, #34948, #32514, .T. ) ;
#12287=CARTESIAN_POINT ( 'NONE',  ( 37.00000000000000711, -11.73555825188272905, 4.983891302653699285 ) ) ;
#12289=CARTESIAN_POINT ( 'NONE',  ( -19.02967556479643463, -13.50000000000023803, -2.066764320408402454E-13 ) ) ;
#12290=CARTESIAN_POINT ( 'NONE',  ( -35.00000000000000000, 7.817610399097512541, 8.766823244862019138 ) ) ;
#12291=AXIS2_PLACEMENT_3D ( 'NONE', #53333, #32677, #11436 ) ;
#12294=ORIENTED_EDGE ( 'NONE', *, *, #37073, .F. ) ;
#12295=EDGE_CURVE ( 'NONE', #56700, #27528, #46081, .T. ) ;
#12297=EDGE_CURVE ( 'NONE', #36193, #64644, #27882, .T. ) ;
#12299=ORIENTED_EDGE ( 'NONE', *, *, #8566, .F. ) ;
#12300=VERTEX_POINT ( 'NONE', #57832 ) ;
#12305=EDGE_CURVE ( 'NONE', #266, #7420, #16917, .T. ) ;
#12307=ORIENTED_EDGE ( 'NONE', *, *, #37969, .T. ) ;
#12308=EDGE_CURVE ( 'NONE', #27547, #54995, #47131, .T. ) ;
#12312=DIRECTION ( 'NONE',  ( 0.000000000000000000, 0.8369827122275325104, 0.5472293298355300761 ) ) ;
#12313=ADVANCED_FACE ( 'NONE', ( #53150 ), #22227, .T. ) ;
#12317=DIRECTION ( 'NONE',  ( 0.000000000000000000, -0.01356324068817991828, 0.9999080150203990547 ) ) ;
#12318=ADVANCED_FACE ( 'NONE', ( #17252 ), #37527, .T. ) ;
#12320=ORIENTED_EDGE ( 'NONE', *, *, #16255, .F. ) ;
#12321=AXIS2_PLACEMENT_3D ( 'NONE', #46007, #35991, #15069 ) ;
#12327=EDGE_LOOP ( 'NONE', ( #64513, #40676, #57571, #30622 ) ) ;
#12330=ORIENTED_EDGE ( 'NONE', *, *, #49325, .F. ) ;
#12331=LINE ( 'NONE', #44233, #45525 ) ;
#12332=ORIENTED_EDGE ( 'NONE', *, *, #61600, .F. ) ;
#12335=CYLINDRICAL_SURFACE ( 'NONE', #44306, 5.000000000000000888 ) ;
#12336=DIRECTION ( 'NONE',  ( 0.000000000000000000, -1.000000000000000000, 0.000000000000000000 ) ) ;
#12337=CARTESIAN_POINT ( 'NONE',  ( 8.812247137149384457, 2.657441218557111906, 11.70499198588243850 ) ) ;
#12339=DIRECTION ( 'NONE',  ( -1.000000000000000000, 0.000000000000000000, 0.000000000000000000 ) ) ;
#12340=ORIENTED_EDGE ( 'NONE', *, *, #12295, .T. ) ;
#12341=CARTESIAN_POINT ( 'NONE',  ( -35.00000000000000000, 0.000000000000000000, 0.000000000000000000 ) ) ;
#12342=ORIENTED_EDGE ( 'NONE', *, *, #12955, .T. ) ;
#12345=EDGE_LOOP ( 'NONE', ( #35920, #60567, #41456, #56165 ) ) ;
#12347=DIRECTION ( 'NONE',  ( -1.000000000000000000, 0.000000000000000000, -0.000000000000000000 ) ) ;
#12349=ORIENTED_EDGE ( 'NONE', *, *, #36763, .F. ) ;
#12353=ORIENTED_EDGE ( 'NONE', *, *, #48623, .F. ) ;
#12354=DIRECTION ( 'NONE',  ( -1.000000000000000000, 0.000000000000000000, 0.000000000000000000 ) ) ;
#12357=CARTESIAN_POINT ( 'NONE',  ( -19.41624570965199581, -4.334582023309537568, 11.19068518931768352 ) ) ;
#12359=EDGE_CURVE ( 'NONE', #6959, #38911, #7816, .T. ) ;
#12360=AXIS2_PLACEMENT_3D ( 'NONE', #59619, #14682, #20350 ) ;
#12361=DIRECTION ( 'NONE',  ( -1.000000000000000000, 0.000000000000000000, 0.000000000000000000 ) ) ;
#12363=CARTESIAN_POINT ( 'NONE',  ( -2.952869152607107139, -12.96714474214480717, 3.755417052241487585 ) ) ;
#12367=CYLINDRICAL_SURFACE ( 'NONE', #28817, 5.000000000000000888 ) ;
#12370=VERTEX_POINT ( 'NONE', #11279 ) ;
#12372=FACE_OUTER_BOUND ( 'NONE', #27192, .T. ) ;
#12373=ORIENTED_EDGE ( 'NONE', *, *, #42927, .F. ) ;
#12375=DIRECTION ( 'NONE',  ( 1.000000000000000000, 0.000000000000000000, 0.000000000000000000 ) ) ;
#12376=ORIENTED_EDGE ( 'NONE', *, *, #28603, .T. ) ;
#12377=UNCERTAINTY_MEASURE_WITH_UNIT (LENGTH_MEASURE( 1.000000000000000082E-05 ), #22659, 'distance_accuracy_value', 'NONE');
#12379=EDGE_LOOP ( 'NONE', ( #17395, #7469, #22139, #6567 ) ) ;
#12380=CARTESIAN_POINT ( 'NONE',  ( 35.00000000000000000, 4.705694406421931860E-17, -3.469127814946512892E-15 ) ) ;
#12381=ORIENTED_EDGE ( 'NONE', *, *, #5872, .T. ) ;
#12383=EDGE_CURVE ( 'NONE', #19103, #14524, #57166, .T. ) ;
#12385=VERTEX_POINT ( 'NONE', #62144 ) ;
#12386=EDGE_CURVE ( 'NONE', #27171, #36886, #37580, .T. ) ;
#12387=DIRECTION ( 'NONE',  ( 1.000000000000000000, 0.000000000000000000, 0.000000000000000000 ) ) ;
#12388=CARTESIAN_POINT ( 'NONE',  ( 1.637652121266425231, 0.7383001981046479756, 13.48328331344350062 ) ) ;
#12389=CARTESIAN_POINT ( 'NONE',  ( 32.00000000000000000, 1.230770033143089974E-14, 0.000000000000000000 ) ) ;
#12390=DIRECTION ( 'NONE',  ( -1.000000000000000000, 0.000000000000000000, 0.000000000000000000 ) ) ;
#12391=ORIENTED_EDGE ( 'NONE', *, *, #58580, .F. ) ;
#12394=DIRECTION ( 'NONE',  ( 0.000000000000000000, 0.01356324068817991481, -0.9999080150203990547 ) ) ;
#12396=ADVANCED_FACE ( 'NONE', ( #8570 ), #49797, .T. ) ;
#12397=LINE ( 'NONE', #27371, #6583 ) ;
#12398=ORIENTED_EDGE ( 'NONE', *, *, #56528, .T. ) ;
#12399=CARTESIAN_POINT ( 'NONE',  ( -37.00000000000000711, 3.805206332242643263, -12.16893194857546412 ) ) ;
#12400=VERTEX_POINT ( 'NONE', #33831 ) ;
#12401=CIRCLE ( 'NONE', #49603, 12.18650000000000055 ) ;
#12402=FACE_OUTER_BOUND ( 'NONE', #17763, .T. ) ;
#12403=DIRECTION ( 'NONE',  ( -1.000000000000000000, 0.000000000000000000, -0.000000000000000000 ) ) ;
#12404=DIRECTION ( 'NONE',  ( -1.000000000000000000, 0.000000000000000000, 0.000000000000000000 ) ) ;
#12406=DIRECTION ( 'NONE',  ( 0.000000000000000000, 0.01356324068817998940, -0.9999080150203990547 ) ) ;
#12407=AXIS2_PLACEMENT_3D ( 'NONE', #63838, #18320, #38587 ) ;
#12410=ORIENTED_EDGE ( 'NONE', *, *, #47772, .F. ) ;
#12411=( BOUNDED_CURVE ( )  B_SPLINE_CURVE ( 3, ( #43814, #22212, #64096, #18575 ),
 .UNSPECIFIED., .F., .F. ) 
 B_SPLINE_CURVE_WITH_KNOTS ( ( 4, 4 ),
 ( 4.494179741888913782, 4.524178010218698809 ),
 .UNSPECIFIED. ) 
 CURVE ( )  GEOMETRIC_REPRESENTATION_ITEM ( )  RATIONAL_B_SPLINE_CURVE ( ( 1.000000000000000000, 0.9999250100640160177, 0.9999250100640160177, 1.000000000000000000 ) ) 
 REPRESENTATION_ITEM ( '' )  );
#12412=ORIENTED_EDGE ( 'NONE', *, *, #36734, .T. ) ;
#12416=CARTESIAN_POINT ( 'NONE',  ( 35.00000000000000000, 11.98254675519227952, -2.220215194441947482 ) ) ;
#12422=EDGE_CURVE ( 'NONE', #55363, #23613, #17402, .T. ) ;
#12423=DIRECTION ( 'NONE',  ( -1.000000000000000000, -1.836970198721029688E-16, 0.000000000000000000 ) ) ;
#12426=LINE ( 'NONE', #36133, #25995 ) ;
#12427=CYLINDRICAL_SURFACE ( 'NONE', #6309, 12.74999999999999822 ) ;
#12428=EDGE_CURVE ( 'NONE', #64891, #61666, #35421, .T. ) ;
#12431=DIRECTION ( 'NONE',  ( 0.000000000000000000, 0.01356324068817998940, -0.9999080150203990547 ) ) ;
#12433=DIRECTION ( 'NONE',  ( 1.000000000000000000, 0.000000000000000000, 0.000000000000000000 ) ) ;
#12434=CARTESIAN_POINT ( 'NONE',  ( 8.937200413559445167, 4.247489200464594994, -11.22584895011355144 ) ) ;
#12436=EDGE_CURVE ( 'NONE', #25992, #51508, #54589, .T. ) ;
#12437=ORIENTED_EDGE ( 'NONE', *, *, #4717, .T. ) ;
#12439=CARTESIAN_POINT ( 'NONE',  ( -35.00000000000000000, 0.000000000000000000, 0.000000000000000000 ) ) ;
#12440=DIRECTION ( 'NONE',  ( -0.000000000000000000, -0.000000000000000000, -1.000000000000000000 ) ) ;
#12442=AXIS2_PLACEMENT_3D ( 'NONE', #39160, #59455, #23904 ) ;
#12443=EDGE_CURVE ( 'NONE', #60039, #21190, #59443, .T. ) ;
#12445=CIRCLE ( 'NONE', #49651, 12.18650000000000055 ) ;
#12447=CARTESIAN_POINT ( 'NONE',  ( -26.94662368254203244, -12.23618042240103243, 5.703482483425735161 ) ) ;
#12448=ORIENTED_EDGE ( 'NONE', *, *, #43979, .T. ) ;
#12453=VERTEX_POINT ( 'NONE', #58475 ) ;
#12459=EDGE_CURVE ( 'NONE', #53266, #9626, #14203, .T. ) ;
#12460=LINE ( 'NONE', #38063, #29800 ) ;
#12461=EDGE_LOOP ( 'NONE', ( #13686, #14662, #41948, #42061 ) ) ;
#12462=EDGE_CURVE ( 'NONE', #39298, #55512, #62715, .T. ) ;
#12466=CARTESIAN_POINT ( 'NONE',  ( -4.049490757281464681, -11.39905423463014777, 7.243820352457140288 ) ) ;
#12468=CARTESIAN_POINT ( 'NONE',  ( 37.00000000000000711, 5.300372733891642874, -11.59605747147788790 ) ) ;
#12469=CARTESIAN_POINT ( 'NONE',  ( -37.00000000000000711, -1.903127969211109383, -11.59095880812010471 ) ) ;
#12470=ORIENTED_EDGE ( 'NONE', *, *, #16294, .F. ) ;
#12471=DIRECTION ( 'NONE',  ( -1.000000000000000000, 0.000000000000000000, 0.000000000000000000 ) ) ;
#12472=EDGE_LOOP ( 'NONE', ( #11672, #39089, #55615, #18502 ) ) ;
#12473=CARTESIAN_POINT ( 'NONE',  ( 22.88594695219327235, 3.421158645304719137, -11.50198563395279194 ) ) ;
#12474=ORIENTED_EDGE ( 'NONE', *, *, #6986, .T. ) ;
#12475=ORIENTED_EDGE ( 'NONE', *, *, #26458, .F. ) ;
#12479=AXIS2_PLACEMENT_3D ( 'NONE', #19474, #2884, #23141 ) ;
#12480=CARTESIAN_POINT ( 'NONE',  ( -3.807799651111238859, 10.57930927450194503, 5.668006617322318696 ) ) ;
#12483=ORIENTED_EDGE ( 'NONE', *, *, #4193, .F. ) ;
#12485=CARTESIAN_POINT ( 'NONE',  ( 145.1370849898475797, 3.309064568108273190E-14, 0.000000000000000000 ) ) ;
#12486=CARTESIAN_POINT ( 'NONE',  ( 3.780834652287974773, 8.352030633203074927, -10.60629927458383470 ) ) ;
#12488=ORIENTED_EDGE ( 'NONE', *, *, #2691, .T. ) ;
#12489=VERTEX_POINT ( 'NONE', #33527 ) ;
#12490=CYLINDRICAL_SURFACE ( 'NONE', #24749, 12.18650000000000055 ) ;
#12492=DIRECTION ( 'NONE',  ( 0.000000000000000000, -0.7617968321374946061, -0.6478160128811867313 ) ) ;
#12493=AXIS2_PLACEMENT_3D ( 'NONE', #3873, #44391, #45074 ) ;
#12497=CARTESIAN_POINT ( 'NONE',  ( -29.41386513404535208, 0.9325270014138739016, 13.46939172307182275 ) ) ;
#12498=CIRCLE ( 'NONE', #7191, 12.18649999999999878 ) ;
#12499=CARTESIAN_POINT ( 'NONE',  ( -35.00000000000000000, 5.814360711498290257, 10.70999494708494559 ) ) ;
#12500=EDGE_CURVE ( 'NONE', #22430, #40555, #64795, .T. ) ;
#12502=CARTESIAN_POINT ( 'NONE',  ( 37.00000000000000711, 4.705694406421931860E-17, -3.469127814946512892E-15 ) ) ;
#12505=CARTESIAN_POINT ( 'NONE',  ( -7.636043109944020024, -8.974902109404503392, -10.10026812394724338 ) ) ;
#12509=ORIENTED_EDGE ( 'NONE', *, *, #13852, .T. ) ;
#12511=DIRECTION ( 'NONE',  ( -1.000000000000000000, 0.000000000000000000, 0.000000000000000000 ) ) ;
#12512=EDGE_LOOP ( 'NONE', ( #17971, #7537, #31637, #16524 ) ) ;
#12513=LINE ( 'NONE', #26848, #25575 ) ;
#12514=CARTESIAN_POINT ( 'NONE',  ( 37.00000000000000711, -5.644643009979139592, -10.30098186818248074 ) ) ;
#12517=EDGE_LOOP ( 'NONE', ( #55732, #32418, #62125, #58295 ) ) ;
#12520=CARTESIAN_POINT ( 'NONE',  ( -28.80358531978833625, 2.755772354643147182, -13.22187685252809253 ) ) ;
#12522=AXIS2_PLACEMENT_3D ( 'NONE', #34177, #27899, #13881 ) ;
#12527=CARTESIAN_POINT ( 'NONE',  ( -18.77295711560618940, -11.99999999999997513, -0.7162851318434579895 ) ) ;
#12528=FACE_OUTER_BOUND ( 'NONE', #1637, .T. ) ;
#12530=ORIENTED_EDGE ( 'NONE', *, *, #37814, .F. ) ;
#12531=AXIS2_PLACEMENT_3D ( 'NONE', #17091, #57335, #61998 ) ;
#12532=CARTESIAN_POINT ( 'NONE',  ( -17.32166409804204577, 3.211681732051251625, -13.11356909678292126 ) ) ;
#12533=CARTESIAN_POINT ( 'NONE',  ( 34.38695973621796043, 25.00000000000000000, 3.530690241644829364 ) ) ;
#12536=CIRCLE ( 'NONE', #49734, 12.18649999999999878 ) ;
#12538=CYLINDRICAL_SURFACE ( 'NONE', #61736, 6.094511299047803199 ) ;
#12540=ORIENTED_EDGE ( 'NONE', *, *, #36009, .T. ) ;
#12541=ORIENTED_EDGE ( 'NONE', *, *, #36566, .F. ) ;
#12543=EDGE_LOOP ( 'NONE', ( #34637, #6505, #63272, #45569 ) ) ;
#12545=CARTESIAN_POINT ( 'NONE',  ( 37.00000000000000711, 4.705694406421931860E-17, -3.469127814946512892E-15 ) ) ;
#12546=CARTESIAN_POINT ( 'NONE',  ( 35.00000000000000000, -7.499679039483992504, 9.040300684349768190 ) ) ;
#12550=DIRECTION ( 'NONE',  ( -1.000000000000000000, -1.836970198721029688E-16, 0.000000000000000000 ) ) ;
#12551=ORIENTED_EDGE ( 'NONE', *, *, #22512, .T. ) ;
#12553=DIRECTION ( 'NONE',  ( -1.000000000000000000, 0.000000000000000000, 0.000000000000000000 ) ) ;
#12555=CARTESIAN_POINT ( 'NONE',  ( 35.00000000000000000, 4.983891302653744582, 11.73555825188270596 ) ) ;
#12556=EDGE_CURVE ( 'NONE', #6306, #21596, #35075, .T. ) ;
#12558=DIRECTION ( 'NONE',  ( 1.000000000000000000, 0.000000000000000000, 0.000000000000000000 ) ) ;
#12560=CARTESIAN_POINT ( 'NONE',  ( -35.00000000000000000, -6.946017217729864690, -10.01317267707894310 ) ) ;
#12562=AXIS2_PLACEMENT_3D ( 'NONE', #28619, #63526, #2390 ) ;
#12566=CARTESIAN_POINT ( 'NONE',  ( 0.000000000000000000, -1.734723475976807094E-15, 13.50000000000000178 ) ) ;
#12568=ORIENTED_EDGE ( 'NONE', *, *, #52981, .T. ) ;
#12569=LINE ( 'NONE', #62793, #21699 ) ;
#12570=VERTEX_POINT ( 'NONE', #25170 ) ;
#12571=ORIENTED_EDGE ( 'NONE', *, *, #51289, .F. ) ;
#12572=DIRECTION ( 'NONE',  ( 0.000000000000000000, 0.01356324068817998940, -0.9999080150203989437 ) ) ;
#12573=CARTESIAN_POINT ( 'NONE',  ( 35.00000000000000000, 11.07407352312218052, 3.916263239775223504 ) ) ;
#12574=AXIS2_PLACEMENT_3D ( 'NONE', #44166, #29209, #49182 ) ;
#12579=AXIS2_PLACEMENT_3D ( 'NONE', #18417, #38994, #59617 ) ;
#12581=EDGE_LOOP ( 'NONE', ( #42223, #5775, #11189, #15269 ) ) ;
#12584=VECTOR ( 'NONE', #10623, 1000.000000000000000 ) ;
#12586=CARTESIAN_POINT ( 'NONE',  ( 35.00000000000000000, -11.78745411414841726, -3.093009498343884722 ) ) ;
#12588=CARTESIAN_POINT ( 'NONE',  ( 26.34661844826604593, 11.53221627053869369, 3.317828791472333005 ) ) ;
#12590=CYLINDRICAL_SURFACE ( 'NONE', #34036, 4.999999999999998224 ) ;
#12594=ADVANCED_FACE ( 'NONE', ( #4912 ), #51461, .T. ) ;
#12598=CARTESIAN_POINT ( 'NONE',  ( -11.40165637462999904, -7.508992741355383416, 9.360289953322597611 ) ) ;
#12599=DIRECTION ( 'NONE',  ( 0.000000000000000000, -0.07632122047557185485, 0.9970832820307033995 ) ) ;
#12601=CARTESIAN_POINT ( 'NONE',  ( -35.00000000000000000, 7.251710744571578715, 9.240395740215660680 ) ) ;
#12603=EDGE_CURVE ( 'NONE', #59191, #39378, #31912, .T. ) ;
#12604=ORIENTED_EDGE ( 'NONE', *, *, #818, .F. ) ;
#12605=CARTESIAN_POINT ( 'NONE',  ( -35.00000000000000000, 8.551552972817082932, 8.052525312709914118 ) ) ;
#12609=CIRCLE ( 'NONE', #25342, 5.000000000000000000 ) ;
#12610=ADVANCED_FACE ( 'NONE', ( #39813 ), #31152, .T. ) ;
#12612=CARTESIAN_POINT ( 'NONE',  ( -4.984433189575353751, -1.083073623696801935, -13.45752292036589637 ) ) ;
#12613=ORIENTED_EDGE ( 'NONE', *, *, #51398, .T. ) ;
#12616=CARTESIAN_POINT ( 'NONE',  ( -35.00000000000000000, 0.000000000000000000, 0.000000000000000000 ) ) ;
#12617=CARTESIAN_POINT ( 'NONE',  ( -37.00000000000000711, 4.946702696913171771, 11.13736569743276306 ) ) ;
#12618=VECTOR ( 'NONE', #53302, 1000.000000000000000 ) ;
#12619=VERTEX_POINT ( 'NONE', #40122 ) ;
#12620=DIRECTION ( 'NONE',  ( -1.000000000000000000, 0.000000000000000000, 0.000000000000000000 ) ) ;
#12621=AXIS2_PLACEMENT_3D ( 'NONE', #16708, #26694, #46004 ) ;
#12622=ORIENTED_EDGE ( 'NONE', *, *, #19383, .T. ) ;
#12625=CYLINDRICAL_SURFACE ( 'NONE', #59798, 4.999999999999999112 ) ;
#12626=DIRECTION ( 'NONE',  ( -1.000000000000000000, 0.000000000000000000, 0.000000000000000000 ) ) ;
#12629=ORIENTED_EDGE ( 'NONE', *, *, #19697, .F. ) ;
#12630=VECTOR ( 'NONE', #38368, 1000.000000000000000 ) ;
#12631=ORIENTED_EDGE ( 'NONE', *, *, #24987, .T. ) ;
#12633=ADVANCED_FACE ( 'NONE', ( #19549 ), #35474, .T. ) ;
#12635=VERTEX_POINT ( 'NONE', #30163 ) ;
#12640=CARTESIAN_POINT ( 'NONE',  ( 22.36482863261543486, -11.96441317219524514, -0.9234811557364158707 ) ) ;
#12641=LINE ( 'NONE', #3367, #47342 ) ;
#12643=EDGE_LOOP ( 'NONE', ( #42867, #46131, #398, #55193 ) ) ;
#12644=CARTESIAN_POINT ( 'NONE',  ( -35.00000000000000000, -2.080187960898651767, 12.57916205664480458 ) ) ;
#12645=ORIENTED_EDGE ( 'NONE', *, *, #58000, .T. ) ;
#12646=DIRECTION ( 'NONE',  ( 0.000000000000000000, -0.01356324068817998940, 0.9999080150203990547 ) ) ;
#12647=VERTEX_POINT ( 'NONE', #60415 ) ;
#12653=EDGE_CURVE ( 'NONE', #48935, #4396, #23428, .T. ) ;
#12654=CARTESIAN_POINT ( 'NONE',  ( 16.78263030916553333, 25.00000000000000000, 5.836879698929882565 ) ) ;
#12656=CARTESIAN_POINT ( 'NONE',  ( 5.373297959932116896, -9.555382238011333129, -7.266535920493700118 ) ) ;
#12657=EDGE_LOOP ( 'NONE', ( #26399, #30108, #45231, #62764 ) ) ;
#12659=ORIENTED_EDGE ( 'NONE', *, *, #37969, .F. ) ;
#12660=AXIS2_PLACEMENT_3D ( 'NONE', #43584, #23989, #18353 ) ;
#12661=CARTESIAN_POINT ( 'NONE',  ( 145.1370849898475797, 3.309064568108273190E-14, 0.000000000000000000 ) ) ;
#12662=EDGE_CURVE ( 'NONE', #61808, #46276, #55100, .T. ) ;
#12663=CARTESIAN_POINT ( 'NONE',  ( -37.00000000000000711, -8.352657516904613999, -8.258652103341526995 ) ) ;
#12664=ADVANCED_FACE ( 'NONE', ( #50466 ), #65394, .F. ) ;
#12666=CARTESIAN_POINT ( 'NONE',  ( -15.52273868740600626, 8.454822416089735171, 8.515633660947054651 ) ) ;
#12670=VERTEX_POINT ( 'NONE', #50133 ) ;
#12671=ORIENTED_EDGE ( 'NONE', *, *, #3563, .T. ) ;
#12674=VECTOR ( 'NONE', #61437, 1000.000000000000000 ) ;
#12679=CARTESIAN_POINT ( 'NONE',  ( -2.894288433085122847, -12.68055345927033706, 4.644490739423512871 ) ) ;
#12680=CARTESIAN_POINT ( 'NONE',  ( -7.393613020821582005, 5.386680228572950035, -10.72686196631679323 ) ) ;
#12681=EDGE_LOOP ( 'NONE', ( #3911, #31941, #48349, #46666 ) ) ;
#12682=VECTOR ( 'NONE', #16918, 1000.000000000000000 ) ;
#12684=EDGE_CURVE ( 'NONE', #60345, #12453, #31781, .T. ) ;
#12688=ADVANCED_FACE ( 'NONE', ( #33685 ), #33018, .T. ) ;
#12689=CARTESIAN_POINT ( 'NONE',  ( 21.94582960821244555, 13.05933372330677500, -3.441589981846832291 ) ) ;
#12691=CARTESIAN_POINT ( 'NONE',  ( 145.1370849898475797, 3.309064568108273190E-14, 0.000000000000000000 ) ) ;
#12692=CARTESIAN_POINT ( 'NONE',  ( 6.211465341154163156, -9.377354143557047550, -7.490490949957647970 ) ) ;
#12694=AXIS2_PLACEMENT_3D ( 'NONE', #43435, #43781, #29452 ) ;
#12695=CIRCLE ( 'NONE', #16983, 4.999999999999999112 ) ;
#12697=CARTESIAN_POINT ( 'NONE',  ( 12.49808451655605879, -9.686563543903927709, -7.085704797288028267 ) ) ;
#12698=ORIENTED_EDGE ( 'NONE', *, *, #54178, .T. ) ;
#12703=ORIENTED_EDGE ( 'NONE', *, *, #24729, .F. ) ;
#12706=CARTESIAN_POINT ( 'NONE',  ( -35.00000000000000000, -11.99999999999999289, 0.000000000000000000 ) ) ;
#12709=CARTESIAN_POINT ( 'NONE',  ( 28.76862497509140226, -12.20680944158938175, 5.780333286781263347 ) ) ;
#12710=AXIS2_PLACEMENT_3D ( 'NONE', #65226, #19695, #29975 ) ;
#12712=EDGE_CURVE ( 'NONE', #10987, #22527, #45733, .T. ) ;
#12713=ADVANCED_FACE ( 'NONE', ( #23387 ), #48357, .T. ) ;
#12714=ORIENTED_EDGE ( 'NONE', *, *, #16913, .T. ) ;
#12715=DIRECTION ( 'NONE',  ( 0.000000000000000000, -0.7196168960969719919, -0.6943713148249714973 ) ) ;
#12717=VECTOR ( 'NONE', #20587, 1000.000000000000000 ) ;
#12718=LINE ( 'NONE', #2451, #24834 ) ;
#12720=ORIENTED_EDGE ( 'NONE', *, *, #38002, .F. ) ;
#12721=CARTESIAN_POINT ( 'NONE',  ( -35.00000000000000000, -11.74226168163341022, -0.3025107581132430723 ) ) ;
#12724=LINE ( 'NONE', #37015, #21314 ) ;
#12726=LINE ( 'NONE', #2112, #43682 ) ;
#12727=VERTEX_POINT ( 'NONE', #41432 ) ;
#12730=VECTOR ( 'NONE', #38846, 1000.000000000000000 ) ;
#12731=ORIENTED_EDGE ( 'NONE', *, *, #32185, .F. ) ;
#12735=DIRECTION ( 'NONE',  ( 0.000000000000000000, 0.9246979985058736418, 0.3807014730195186214 ) ) ;
#12736=DIRECTION ( 'NONE',  ( 1.000000000000000000, 0.000000000000000000, 0.000000000000000000 ) ) ;
#12740=EDGE_LOOP ( 'NONE', ( #42636, #41582, #39293, #58772 ) ) ;
#12743=EDGE_LOOP ( 'NONE', ( #4857, #3287, #42976, #50402 ) ) ;
#12744=EDGE_CURVE ( 'NONE', #27033, #7491, #18421, .T. ) ;
#12745=EDGE_LOOP ( 'NONE', ( #36552, #52048, #46552, #48132 ) ) ;
#12746=FACE_OUTER_BOUND ( 'NONE', #47587, .T. ) ;
#12747=CARTESIAN_POINT ( 'NONE',  ( -35.00000000000000000, -2.185196060783795691, -11.54110654723651486 ) ) ;
#12748=LINE ( 'NONE', #13733, #1191 ) ;
#12750=DIRECTION ( 'NONE',  ( -1.000000000000000000, -1.836970198721029688E-16, 0.000000000000000000 ) ) ;
#12753=DIRECTION ( 'NONE',  ( -1.000000000000000000, 0.000000000000000000, 0.000000000000000000 ) ) ;
#12755=EDGE_CURVE ( 'NONE', #18737, #51616, #3277, .T. ) ;
#12759=ADVANCED_FACE ( 'NONE', ( #26168 ), #7773, .T. ) ;
#12760=CIRCLE ( 'NONE', #59490, 4.999999999999999112 ) ;
#12764=CIRCLE ( 'NONE', #14838, 12.74999999999999822 ) ;
#12766=ADVANCED_FACE ( 'NONE', ( #33367 ), #8102, .T. ) ;
#12769=FACE_OUTER_BOUND ( 'NONE', #23271, .T. ) ;
#12772=CARTESIAN_POINT ( 'NONE',  ( -18.49080574448724690, -13.49999999999999822, -2.827202046691532642E-15 ) ) ;
#12773=AXIS2_PLACEMENT_3D ( 'NONE', #56254, #51299, #18512 ) ;
#12776=ORIENTED_EDGE ( 'NONE', *, *, #7668, .T. ) ;
#12777=CARTESIAN_POINT ( 'NONE',  ( 37.00000000000000711, 10.28547182238015978, 5.672855678558568648 ) ) ;
#12778=DIRECTION ( 'NONE',  ( 0.000000000000000000, -0.01356324068817998940, 0.9999080150203990547 ) ) ;
#12779=DIRECTION ( 'NONE',  ( 1.000000000000000000, 0.000000000000000000, 0.000000000000000000 ) ) ;
#12781=ORIENTED_EDGE ( 'NONE', *, *, #49324, .F. ) ;
#12785=VERTEX_POINT ( 'NONE', #887 ) ;
#12786=APPLICATION_CONTEXT ( 'automotive_design' ) ;
#12787=B_SPLINE_CURVE_WITH_KNOTS ( 'NONE', 3,
 ( #10876, #60430, #35139, #30177, #35487, #35793, #31167, #60110, #10214, #25855, #46145, #65086 ),
 .UNSPECIFIED., .F., .F.,
 ( 4, 2, 2, 2, 2, 4 ),
 ( 0.002289549871878519133, 0.002934044320523027626, 0.003578538769167536118, 0.004867527666456550502, 0.006156516563745564885, 0.007445505461034578401 ),
 .UNSPECIFIED. ) ;
#12788=ORIENTED_EDGE ( 'NONE', *, *, #37449, .F. ) ;
#12789=CARTESIAN_POINT ( 'NONE',  ( -35.00000000000000000, 0.000000000000000000, 0.000000000000000000 ) ) ;
#12790=CIRCLE ( 'NONE', #43553, 12.74999999999999822 ) ;
#12792=AXIS2_PLACEMENT_3D ( 'NONE', #47470, #52469, #22858 ) ;
#12793=AXIS2_PLACEMENT_3D ( 'NONE', #53711, #8144, #28415 ) ;
#12794=ORIENTED_EDGE ( 'NONE', *, *, #37716, .F. ) ;
#12795=CARTESIAN_POINT ( 'NONE',  ( 35.00000000000000000, -10.75351884295723970, 4.725891942574862448 ) ) ;
#12796=EDGE_CURVE ( 'NONE', #21512, #1348, #41447, .T. ) ;
#12803=DIRECTION ( 'NONE',  ( 0.000000000000000000, -0.9651210252299767811, -0.2618041379715732586 ) ) ;
#12808=EDGE_LOOP ( 'NONE', ( #7001, #8985, #24915, #36943 ) ) ;
#12809=EDGE_CURVE ( 'NONE', #27449, #429, #9375, .T. ) ;
#12810=EDGE_LOOP ( 'NONE', ( #38304, #42430, #47866, #36379 ) ) ;
#12811=PLANE ( 'NONE',  #40078 ) ;
#12812=CIRCLE ( 'NONE', #61661, 12.74999999999999822 ) ;
#12814=CARTESIAN_POINT ( 'NONE',  ( -25.13384719747249108, 8.062265727243834945, 10.83424663242000996 ) ) ;
#12815=AXIS2_PLACEMENT_3D ( 'NONE', #8043, #22004, #28307 ) ;
#12816=DIRECTION ( 'NONE',  ( 1.000000000000000000, 0.000000000000000000, 0.000000000000000000 ) ) ;
#12817=CARTESIAN_POINT ( 'NONE',  ( -35.00000000000000000, 0.000000000000000000, 0.000000000000000000 ) ) ;
#12818=VECTOR ( 'NONE', #21188, 1000.000000000000000 ) ;
#12820=AXIS2_PLACEMENT_3D ( 'NONE', #16358, #2038, #21682 ) ;
#12821=CARTESIAN_POINT ( 'NONE',  ( -26.14336630348346091, -10.67021403765777521, 5.492080489366163221 ) ) ;
#12822=DIRECTION ( 'NONE',  ( 0.000000000000000000, -0.01356324068817991828, 0.9999080150203990547 ) ) ;
#12824=EDGE_LOOP ( 'NONE', ( #46856, #31375, #19803, #10984 ) ) ;
#12825=ORIENTED_EDGE ( 'NONE', *, *, #28726, .T. ) ;
#12826=AXIS2_PLACEMENT_3D ( 'NONE', #41454, #26840, #61414 ) ;
#12828=EDGE_CURVE ( 'NONE', #32047, #10423, #18744, .T. ) ;
#12829=EDGE_LOOP ( 'NONE', ( #15361, #42845, #37345, #20044 ) ) ;
#12830=VECTOR ( 'NONE', #52199, 1000.000000000000000 ) ;
#12831=CARTESIAN_POINT ( 'NONE',  ( 29.35982233226166471, -7.748204631658793140, 11.05532493772648550 ) ) ;
#12834=EDGE_CURVE ( 'NONE', #7231, #56666, #48943, .T. ) ;
#12836=CARTESIAN_POINT ( 'NONE',  ( 37.00000000000000711, 4.705694406421931860E-17, -3.469127814946512892E-15 ) ) ;
#12838=CARTESIAN_POINT ( 'NONE',  ( -9.351388602708162523, 12.99278190472488248, -3.665735721005250358 ) ) ;
#12839=AXIS2_PLACEMENT_3D ( 'NONE', #39657, #39977, #60587 ) ;
#12841=CARTESIAN_POINT ( 'NONE',  ( -17.71314213125373627, 12.92974920937838768, 3.882255733911251117 ) ) ;
#12842=VERTEX_POINT ( 'NONE', #8421 ) ;
#12843=AXIS2_PLACEMENT_3D ( 'NONE', #45029, #40693, #65303 ) ;
#12847=ADVANCED_FACE ( 'NONE', ( #14378 ), #49967, .T. ) ;
#12850=VERTEX_POINT ( 'NONE', #34650 ) ;
#12852=EDGE_CURVE ( 'NONE', #36872, #65779, #24356, .T. ) ;
#12853=VERTEX_POINT ( 'NONE', #39318 ) ;
#12856=CARTESIAN_POINT ( 'NONE',  ( 8.691781497961200031, 5.979943475656228635, 10.40578628523820015 ) ) ;
#12857=EDGE_CURVE ( 'NONE', #37109, #27716, #25029, .T. ) ;
#12861=DIRECTION ( 'NONE',  ( 1.000000000000000000, 0.000000000000000000, 0.000000000000000000 ) ) ;
#12863=DIRECTION ( 'NONE',  ( -0.000000000000000000, -1.000000000000000000, -0.000000000000000000 ) ) ;
#12865=VECTOR ( 'NONE', #5039, 1000.000000000000000 ) ;
#12869=AXIS2_PLACEMENT_3D ( 'NONE', #33017, #23066, #28371 ) ;
#12871=ORIENTED_EDGE ( 'NONE', *, *, #47646, .T. ) ;
#12872=DIRECTION ( 'NONE',  ( 1.000000000000000000, 0.000000000000000000, 0.000000000000000000 ) ) ;
#12873=CARTESIAN_POINT ( 'NONE',  ( 29.73200328305864204, 9.106906332337908694, 10.00596268623472263 ) ) ;
#12877=CARTESIAN_POINT ( 'NONE',  ( -11.08084578044607582, -9.571663398071640572, -7.261247739973540227 ) ) ;
#12881=CARTESIAN_POINT ( 'NONE',  ( -29.59036887715360464, 2.131711947223947412, -13.33733930595583494 ) ) ;
#12883=ORIENTED_EDGE ( 'NONE', *, *, #15651, .F. ) ;
#12884=DIRECTION ( 'NONE',  ( 1.000000000000000000, 0.000000000000000000, 0.000000000000000000 ) ) ;
#12886=AXIS2_PLACEMENT_3D ( 'NONE', #34807, #59454, #60109 ) ;
#12887=EDGE_CURVE ( 'NONE', #23433, #38220, #39326, .T. ) ;
#12892=FACE_OUTER_BOUND ( 'NONE', #44531, .T. ) ;
#12894=DIRECTION ( 'NONE',  ( 1.000000000000000000, 0.000000000000000000, 0.000000000000000000 ) ) ;
#12895=AXIS2_PLACEMENT_3D ( 'NONE', #22377, #57982, #17740 ) ;
#12896=ORIENTED_EDGE ( 'NONE', *, *, #15643, .F. ) ;
#12897=VECTOR ( 'NONE', #52652, 1000.000000000000000 ) ;
#12899=CARTESIAN_POINT ( 'NONE',  ( -37.00000000000000711, -3.645068577060105230, 11.16627499335654150 ) ) ;
#12900=EDGE_LOOP ( 'NONE', ( #39816, #6766, #5375, #4354 ) ) ;
#12905=CIRCLE ( 'NONE', #27751, 4.999999999999999112 ) ;
#12907=ORIENTED_EDGE ( 'NONE', *, *, #60060, .F. ) ;
#12908=CARTESIAN_POINT ( 'NONE',  ( -37.00000000000000711, 11.73808581813437968, -0.4353888892048790038 ) ) ;
#12910=CARTESIAN_POINT ( 'NONE',  ( 37.00000000000000711, -1.791059740004337097, 12.05416472667166872 ) ) ;
#12913=LINE ( 'NONE', #33837, #51255 ) ;
#12914=EDGE_CURVE ( 'NONE', #44234, #17999, #56315, .T. ) ;
#12915=EDGE_LOOP ( 'NONE', ( #61458, #14171, #53661, #29563 ) ) ;
#12918=EDGE_LOOP ( 'NONE', ( #43931, #44348, #22885, #1513 ) ) ;
#12919=VECTOR ( 'NONE', #64346, 1000.000000000000000 ) ;
#12920=CARTESIAN_POINT ( 'NONE',  ( 34.00000000000000000, 11.99999999999999822, 0.000000000000000000 ) ) ;
#12921=ADVANCED_FACE ( 'NONE', ( #3793 ), #44308, .T. ) ;
#12923=AXIS2_PLACEMENT_3D ( 'NONE', #33499, #53790, #23190 ) ;
#12926=CARTESIAN_POINT ( 'NONE',  ( -35.00000000000000000, -3.213188559034318992, 11.29812557209475798 ) ) ;
#12927=VECTOR ( 'NONE', #9829, 1000.000000000000000 ) ;
#12930=DIRECTION ( 'NONE',  ( -1.000000000000000000, 0.000000000000000000, -0.000000000000000000 ) ) ;
#12934=CARTESIAN_POINT ( 'NONE',  ( 37.00000000000000711, -6.265926637539569910, -11.10408318471057676 ) ) ;
#12935=CARTESIAN_POINT ( 'NONE',  ( 36.00000000000000711, -10.59380114696464581, 7.094637218249467914 ) ) ;
#12939=CARTESIAN_POINT ( 'NONE',  ( -37.00000000000000711, -8.830544224262881770, -9.196955404009390378 ) ) ;
#12941=VERTEX_POINT ( 'NONE', #19724 ) ;
#12943=AXIS2_PLACEMENT_3D ( 'NONE', #44723, #39084, #4178 ) ;
#12944=ORIENTED_EDGE ( 'NONE', *, *, #5, .F. ) ;
#12947=CARTESIAN_POINT ( 'NONE',  ( 37.00000000000000711, -11.37311665002365579, -2.936739658819832677 ) ) ;
#12950=ORIENTED_EDGE ( 'NONE', *, *, #45655, .T. ) ;
#12951=DIRECTION ( 'NONE',  ( 1.000000000000000000, 0.000000000000000000, 0.000000000000000000 ) ) ;
#12952=CARTESIAN_POINT ( 'NONE',  ( -35.00000000000000000, -11.30684963584386082, -4.545979934229532837 ) ) ;
#12953=CARTESIAN_POINT ( 'NONE',  ( -18.76942114191558275, -13.50000000000000355, 0.6346529038414141510 ) ) ;
#12955=EDGE_CURVE ( 'NONE', #16089, #54132, #3332, .T. ) ;
#12956=AXIS2_PLACEMENT_3D ( 'NONE', #63138, #52535, #7958 ) ;
#12957=CARTESIAN_POINT ( 'NONE',  ( 35.00000000000000000, 8.295159312811978936, 8.927548052240801724 ) ) ;
#12958=ORIENTED_EDGE ( 'NONE', *, *, #5488, .T. ) ;
#12962=CARTESIAN_POINT ( 'NONE',  ( 36.00000000000000711, -7.094637218249427946, -10.59380114696467778 ) ) ;
#12963=CIRCLE ( 'NONE', #45867, 4.999999999999999112 ) ;
#12964=VECTOR ( 'NONE', #219, 1000.000000000000000 ) ;
#12965=ORIENTED_EDGE ( 'NONE', *, *, #57118, .F. ) ;
#12967=CARTESIAN_POINT ( 'NONE',  ( -9.824774371450907040, 12.26007224129469897, -5.655028462584398952 ) ) ;
#12968=EDGE_CURVE ( 'NONE', #30390, #29592, #9648, .T. ) ;
#12970=FACE_OUTER_BOUND ( 'NONE', #60912, .T. ) ;
#12971=DIRECTION ( 'NONE',  ( -1.000000000000000000, -0.000000000000000000, 0.000000000000000000 ) ) ;
#12972=CARTESIAN_POINT ( 'NONE',  ( 35.00000000000000000, 7.717887834988244045, -8.854740511458876639 ) ) ;
#12973=DIRECTION ( 'NONE',  ( 1.000000000000000000, 0.000000000000000000, 0.000000000000000000 ) ) ;
#12976=EDGE_CURVE ( 'NONE', #19103, #28220, #61671, .T. ) ;
#12978=VERTEX_POINT ( 'NONE', #68 ) ;
#12979=VERTEX_POINT ( 'NONE', #16006 ) ;
#12982=B_SPLINE_CURVE_WITH_KNOTS ( 'NONE', 3,
 ( #15022, #66, #50310, #39316, #29349, #65557, #54651, #14045, #19388, #29998 ),
 .UNSPECIFIED., .F., .F.,
 ( 4, 2, 2, 2, 4 ),
 ( 3.469446951953614189E-18, 0.002586846717445558108, 0.003233558396806946768, 0.003880270076168335427, 0.005173693434891112747 ),
 .UNSPECIFIED. ) ;
#12983=ADVANCED_FACE ( 'NONE', ( #1404 ), #55934, .T. ) ;
#12984=EDGE_LOOP ( 'NONE', ( #24887, #62933, #18845, #36420 ) ) ;
#12985=DIRECTION ( 'NONE',  ( 0.000000000000000000, 0.01356324068817998940, -0.9999080150203990547 ) ) ;
#12986=AXIS2_PLACEMENT_3D ( 'NONE', #19569, #60119, #14539 ) ;
#12989=CYLINDRICAL_SURFACE ( 'NONE', #12067, 5.225920239717171789 ) ;
#12991=DIRECTION ( 'NONE',  ( 0.000000000000000000, -0.9847383929261598334, 0.1740410799127720121 ) ) ;
#12992=EDGE_LOOP ( 'NONE', ( #39076, #48914, #24410, #722 ) ) ;
#12994=CARTESIAN_POINT ( 'NONE',  ( 35.00000000000000000, -8.146229107149464355, -9.063649021438928699 ) ) ;
#12996=FACE_OUTER_BOUND ( 'NONE', #23597, .T. ) ;
#12997=VERTEX_POINT ( 'NONE', #15672 ) ;
#13002=AXIS2_PLACEMENT_3D ( 'NONE', #48547, #58523, #22950 ) ;
#13004=CIRCLE ( 'NONE', #29983, 12.18650000000000055 ) ;
#13009=EDGE_LOOP ( 'NONE', ( #22397, #39701, #20987, #32851 ) ) ;
#13012=ORIENTED_EDGE ( 'NONE', *, *, #60060, .T. ) ;
#13015=VERTEX_POINT ( 'NONE', #20352 ) ;
#13017=DIRECTION ( 'NONE',  ( 0.000000000000000000, -0.01356324068817998940, 0.9999080150203990547 ) ) ;
#13021=VECTOR ( 'NONE', #17966, 1000.000000000000000 ) ;
#13022=ORIENTED_EDGE ( 'NONE', *, *, #56697, .T. ) ;
#13023=CARTESIAN_POINT ( 'NONE',  ( 35.00000000000000000, -3.614449339633571512, -11.17622378668005290 ) ) ;
#13024=AXIS2_PLACEMENT_3D ( 'NONE', #16348, #26638, #406 ) ;
#13025=ORIENTED_EDGE ( 'NONE', *, *, #22545, .T. ) ;
#13026=CARTESIAN_POINT ( 'NONE',  ( -25.90770972894546276, -12.26982202440151681, 5.631397833353792848 ) ) ;
#13027=LINE ( 'NONE', #28320, #60549 ) ;
#13028=VECTOR ( 'NONE', #44798, 1000.000000000000000 ) ;
#13030=CARTESIAN_POINT ( 'NONE',  ( -37.00000000000000711, 12.60630747491665993, -1.908798535168240607 ) ) ;
#13031=LINE ( 'NONE', #7055, #41657 ) ;
#13033=FACE_OUTER_BOUND ( 'NONE', #2257, .T. ) ;
#13034=EDGE_CURVE ( 'NONE', #19643, #6845, #63810, .T. ) ;
#13036=CARTESIAN_POINT ( 'NONE',  ( -35.00000000000000000, 0.000000000000000000, 0.000000000000000000 ) ) ;
#13037=DIRECTION ( 'NONE',  ( 1.000000000000000000, 0.000000000000000000, 0.000000000000000000 ) ) ;
#13039=CARTESIAN_POINT ( 'NONE',  ( 6.313836040153129936, -9.245614688376601720, -7.652703899474847304 ) ) ;
#13040=DIRECTION ( 'NONE',  ( 0.000000000000000000, 0.01356324068817991828, -0.9999080150203990547 ) ) ;
#13041=CIRCLE ( 'NONE', #51422, 5.000000000000000000 ) ;
#13042=CIRCLE ( 'NONE', #56574, 4.999999999999999112 ) ;
#13045=ORIENTED_EDGE ( 'NONE', *, *, #40864, .F. ) ;
#13046=CARTESIAN_POINT ( 'NONE',  ( 12.89197382821344107, -10.53456990936045656, -5.760929614845139213 ) ) ;
#13054=EDGE_CURVE ( 'NONE', #39894, #53714, #27690, .T. ) ;
#13055=ORIENTED_EDGE ( 'NONE', *, *, #43453, .F. ) ;
#13056=VECTOR ( 'NONE', #7130, 1000.000000000000000 ) ;
#13057=DIRECTION ( 'NONE',  ( 1.000000000000000000, 0.000000000000000000, 0.000000000000000000 ) ) ;
#13058=ORIENTED_EDGE ( 'NONE', *, *, #54480, .F. ) ;
#13060=FACE_OUTER_BOUND ( 'NONE', #30363, .T. ) ;
#13065=DIRECTION ( 'NONE',  ( 0.000000000000000000, 0.9718671068226450993, -0.2355298848897551256 ) ) ;
#13066=CARTESIAN_POINT ( 'NONE',  ( 3.780834652287974773, 8.352030633203080257, 10.60629927458383115 ) ) ;
#13067=LINE ( 'NONE', #2103, #16343 ) ;
#13068=CARTESIAN_POINT ( 'NONE',  ( 17.82326783675071624, 8.603617134778573927, 8.377922036602647893 ) ) ;
#13069=ORIENTED_EDGE ( 'NONE', *, *, #18400, .T. ) ;
#13070=CARTESIAN_POINT ( 'NONE',  ( -15.27729454824424948, 5.151216734910788908, 25.00000000000000000 ) ) ;
#13072=VECTOR ( 'NONE', #61910, 1000.000000000000000 ) ;
#13075=CARTESIAN_POINT ( 'NONE',  ( -24.43712776614061610, 9.284275035674196985, 7.605845515126569367 ) ) ;
#13077=CARTESIAN_POINT ( 'NONE',  ( -35.00000000000000000, 12.74613886779085270, -0.3137578094507860738 ) ) ;
#13079=DIRECTION ( 'NONE',  ( 1.000000000000000000, 0.000000000000000000, 0.000000000000000000 ) ) ;
#13080=VERTEX_POINT ( 'NONE', #31628 ) ;
#13081=DIRECTION ( 'NONE',  ( 1.000000000000000000, -0.000000000000000000, 0.000000000000000000 ) ) ;
#13084=CARTESIAN_POINT ( 'NONE',  ( 35.00000000000000000, 8.573591947375318156, -8.029056188533719052 ) ) ;
#13085=CIRCLE ( 'NONE', #65089, 5.000000000000001776 ) ;
#13089=EDGE_CURVE ( 'NONE', #38600, #52675, #46829, .T. ) ;
#13090=ORIENTED_EDGE ( 'NONE', *, *, #35185, .T. ) ;
#13091=CARTESIAN_POINT ( 'NONE',  ( 35.00000000000000000, 4.705694406421931860E-17, -3.469127814946512892E-15 ) ) ;
#13094=ORIENTED_EDGE ( 'NONE', *, *, #35778, .T. ) ;
#13096=AXIS2_PLACEMENT_3D ( 'NONE', #52177, #27218, #47510 ) ;
#13097=CARTESIAN_POINT ( 'NONE',  ( 35.00000000000000000, 4.705694406421931860E-17, -3.469127814946512892E-15 ) ) ;
#13098=DIRECTION ( 'NONE',  ( 0.000000000000000000, 0.01356324068817998940, -0.9999080150203989437 ) ) ;
#13100=LINE ( 'NONE', #28388, #8299 ) ;
#13101=CARTESIAN_POINT ( 'NONE',  ( -35.00000000000000000, -1.591260454995328866, 12.08216339958900321 ) ) ;
#13102=AXIS2_PLACEMENT_3D ( 'NONE', #12238, #32502, #27868 ) ;
#13104=EDGE_LOOP ( 'NONE', ( #3976, #16122, #4237, #25353 ) ) ;
#13106=AXIS2_PLACEMENT_3D ( 'NONE', #2407, #18359, #22686 ) ;
#13109=AXIS2_PLACEMENT_3D ( 'NONE', #18488, #18135, #38407 ) ;
#13111=DIRECTION ( 'NONE',  ( 0.000000000000000000, 0.7196168960969766548, 0.6943713148249667233 ) ) ;
#13112=DIRECTION ( 'NONE',  ( 1.000000000000000000, 0.000000000000000000, 0.000000000000000000 ) ) ;
#13114=CARTESIAN_POINT ( 'NONE',  ( 12.27732682522752583, 0.5231312807845712731, -11.98861953884736131 ) ) ;
#13115=ORIENTED_EDGE ( 'NONE', *, *, #53199, .F. ) ;
#13116=FACE_OUTER_BOUND ( 'NONE', #29597, .T. ) ;
#13117=CARTESIAN_POINT ( 'NONE',  ( -36.00000000000000711, -11.80185301892984562, 4.824807283154076920 ) ) ;
#13118=CARTESIAN_POINT ( 'NONE',  ( 35.00000000000000000, 4.705694406421931860E-17, -3.469127814946512892E-15 ) ) ;
#13120=AXIS2_PLACEMENT_3D ( 'NONE', #7597, #48189, #16265 ) ;
#13123=CARTESIAN_POINT ( 'NONE',  ( 35.00000000000000000, 4.339012074899953220, -10.91536515067649660 ) ) ;
#13125=DIRECTION ( 'NONE',  ( 0.000000000000000000, 0.01356324068817998940, -0.9999080150203989437 ) ) ;
#13127=DIRECTION ( 'NONE',  ( 1.000000000000000000, 0.000000000000000000, 0.000000000000000000 ) ) ;
#13128=VERTEX_POINT ( 'NONE', #48592 ) ;
#13129=CARTESIAN_POINT ( 'NONE',  ( -14.11589373245165469, 8.250315036047107142, -8.713914264323175729 ) ) ;
#13130=CYLINDRICAL_SURFACE ( 'NONE', #9655, 4.999999999999999112 ) ;
#13131=ADVANCED_FACE ( 'NONE', ( #31953 ), #57248, .T. ) ;
#13133=VECTOR ( 'NONE', #35905, 1000.000000000000000 ) ;
#13134=AXIS2_PLACEMENT_3D ( 'NONE', #2119, #42654, #43326 ) ;
#13135=ORIENTED_EDGE ( 'NONE', *, *, #21369, .T. ) ;
#13136=LINE ( 'NONE', #2854, #51178 ) ;
#13137=AXIS2_PLACEMENT_3D ( 'NONE', #34124, #58791, #44420 ) ;
#13138=B_SPLINE_CURVE_WITH_KNOTS ( 'NONE', 3,
 ( #38798, #59097, #33144, #63085, #17544, #37811, #22865, #28173, #50426, #50742, #8864, #50090 ),
 .UNSPECIFIED., .F., .F.,
 ( 4, 2, 2, 2, 2, 4 ),
 ( 2.096074351170153978E-17, 0.002188339370024745302, 0.004376678740049471522, 0.005470848425061835933, 0.006565018110074198610, 0.008753357480098915289 ),
 .UNSPECIFIED. ) ;
#13139=ORIENTED_EDGE ( 'NONE', *, *, #13976, .T. ) ;
#13140=CARTESIAN_POINT ( 'NONE',  ( -37.00000000000000711, 11.61175578952786047, 1.771820996347196697 ) ) ;
#13142=DIRECTION ( 'NONE',  ( -1.000000000000000000, 0.000000000000000000, 0.000000000000000000 ) ) ;
#13143=CYLINDRICAL_SURFACE ( 'NONE', #18124, 5.000000000000000888 ) ;
#13144=CARTESIAN_POINT ( 'NONE',  ( -27.22416769087903532, 9.103615227035337654, -7.837773337750173930 ) ) ;
#13145=ADVANCED_FACE ( 'NONE', ( #62535 ), #17676, .T. ) ;
#13146=AXIS2_PLACEMENT_3D ( 'NONE', #37215, #7287, #48226 ) ;
#13147=DIRECTION ( 'NONE',  ( 0.000000000000000000, 0.8989688749565172277, 0.4380125133593943398 ) ) ;
#13148=DIRECTION ( 'NONE',  ( -1.000000000000000000, 0.000000000000000000, -0.000000000000000000 ) ) ;
#13149=ORIENTED_EDGE ( 'NONE', *, *, #21369, .F. ) ;
#13150=DIRECTION ( 'NONE',  ( 0.000000000000000000, -0.9987865678893271815, 0.04924826701375693838 ) ) ;
#13151=EDGE_CURVE ( 'NONE', #55517, #16276, #4366, .T. ) ;
#13152=ORIENTED_EDGE ( 'NONE', *, *, #4902, .T. ) ;
#13153=DIRECTION ( 'NONE',  ( 0.000000000000000000, -0.01356324068817998940, 0.9999080150203990547 ) ) ;
#13154=VECTOR ( 'NONE', #20145, 1000.000000000000000 ) ;
#13155=ORIENTED_EDGE ( 'NONE', *, *, #1761, .F. ) ;
#13157=CARTESIAN_POINT ( 'NONE',  ( -18.12415734164024883, 6.857820005957854015, 11.63132115085990570 ) ) ;
#13160=CARTESIAN_POINT ( 'NONE',  ( -25.43923780825302572, 12.11207825353047518, 5.970565962100374158 ) ) ;
#13161=CARTESIAN_POINT ( 'NONE',  ( 36.00000000000000711, -8.235637554476713973, -9.733281772932135922 ) ) ;
#13165=EDGE_CURVE ( 'NONE', #27716, #10498, #56111, .T. ) ;
#13166=VERTEX_POINT ( 'NONE', #33283 ) ;
#13170=AXIS2_PLACEMENT_3D ( 'NONE', #5590, #595, #35145 ) ;
#13172=EDGE_CURVE ( 'NONE', #29748, #48808, #23484, .T. ) ;
#13174=ORIENTED_EDGE ( 'NONE', *, *, #43987, .F. ) ;
#13178=CARTESIAN_POINT ( 'NONE',  ( -35.00000000000000000, 0.2661492558805056974, -12.18359334611896116 ) ) ;
#13179=DIRECTION ( 'NONE',  ( -1.000000000000000000, -0.000000000000000000, 0.000000000000000000 ) ) ;
#13182=DIRECTION ( 'NONE',  ( 0.000000000000000000, -0.8515178078024921993, 0.5243256840888473880 ) ) ;
#13183=ORIENTED_EDGE ( 'NONE', *, *, #55933, .T. ) ;
#13187=AXIS2_PLACEMENT_3D ( 'NONE', #44436, #49146, #59421 ) ;
#13190=EDGE_CURVE ( 'NONE', #61135, #42299, #64203, .T. ) ;
#13191=ORIENTED_EDGE ( 'NONE', *, *, #39564, .T. ) ;
#13192=LINE ( 'NONE', #9167, #54610 ) ;
#13193=ORIENTED_EDGE ( 'NONE', *, *, #65060, .T. ) ;
#13195=DIRECTION ( 'NONE',  ( 1.000000000000000000, 0.000000000000000000, 0.000000000000000000 ) ) ;
#13196=CARTESIAN_POINT ( 'NONE',  ( -35.00000000000000000, 8.830544224262945718, 9.196955404009328205 ) ) ;
#13197=DIRECTION ( 'NONE',  ( 0.000000000000000000, 0.5987040770935676548, -0.8009703041134168533 ) ) ;
#13198=ORIENTED_EDGE ( 'NONE', *, *, #27374, .T. ) ;
#13201=DIRECTION ( 'NONE',  ( 1.000000000000000000, 0.000000000000000000, 0.000000000000000000 ) ) ;
#13204=CARTESIAN_POINT ( 'NONE',  ( -35.00000000000000000, -2.216820770815165265, 11.53507381115582575 ) ) ;
#13207=( BOUNDED_CURVE ( )  B_SPLINE_CURVE ( 3, ( #45399, #40749, #61037, #35074 ),
 .UNSPECIFIED., .F., .F. ) 
 B_SPLINE_CURVE_WITH_KNOTS ( ( 4, 4 ),
 ( 3.531674309133673528, 3.627469539221107375 ),
 .UNSPECIFIED. ) 
 CURVE ( )  GEOMETRIC_REPRESENTATION_ITEM ( )  RATIONAL_B_SPLINE_CURVE ( ( 1.000000000000000000, 0.9992354190151078175, 0.9992354190151078175, 1.000000000000000000 ) ) 
 REPRESENTATION_ITEM ( '' )  );
#13208=ORIENTED_EDGE ( 'NONE', *, *, #23204, .T. ) ;
#13212=ORIENTED_EDGE ( 'NONE', *, *, #18430, .F. ) ;
#13213=CARTESIAN_POINT ( 'NONE',  ( 37.00000000000000711, 10.02106554660720050, 7.882940143791662635 ) ) ;
#13215=DIRECTION ( 'NONE',  ( 0.000000000000000000, -0.9651210252299767811, -0.2618041379715732586 ) ) ;
#13216=EDGE_CURVE ( 'NONE', #63114, #1051, #62765, .T. ) ;
#13217=DIRECTION ( 'NONE',  ( 0.000000000000000000, -0.01356324068817998940, 0.9999080150203990547 ) ) ;
#13218=EDGE_CURVE ( 'NONE', #33743, #34466, #31962, .T. ) ;
#13220=ORIENTED_EDGE ( 'NONE', *, *, #47009, .F. ) ;
#13221=CARTESIAN_POINT ( 'NONE',  ( 47.00000000000000711, 4.705694406421931860E-17, -3.469127814946512892E-15 ) ) ;
#13224=DIRECTION ( 'NONE',  ( 0.000000000000000000, 0.9987865678893275145, -0.04924826701374940968 ) ) ;
#13227=DIRECTION ( 'NONE',  ( 0.000000000000000000, 0.000000000000000000, -1.000000000000000000 ) ) ;
#13228=DIRECTION ( 'NONE',  ( 0.000000000000000000, 0.9999080150203989437, 0.01356324068817649567 ) ) ;
#13229=DIRECTION ( 'NONE',  ( -1.000000000000000000, 0.000000000000000000, -0.000000000000000000 ) ) ;
#13232=AXIS2_PLACEMENT_3D ( 'NONE', #27772, #48075, #2533 ) ;
#13233=EDGE_LOOP ( 'NONE', ( #11361, #48491, #5622, #48455 ) ) ;
#13235=EDGE_LOOP ( 'NONE', ( #51989, #22687, #5207, #29399 ) ) ;
#13236=EDGE_CURVE ( 'NONE', #61588, #29827, #39364, .T. ) ;
#13239=CARTESIAN_POINT ( 'NONE',  ( -35.00000000000000000, 12.14284015767850100, 1.030638227056609679 ) ) ;
#13241=EDGE_CURVE ( 'NONE', #54831, #32188, #28616, .T. ) ;
#13243=VERTEX_POINT ( 'NONE', #24617 ) ;
#13245=AXIS2_PLACEMENT_3D ( 'NONE', #5029, #40248, #19674 ) ;
#13248=ORIENTED_EDGE ( 'NONE', *, *, #65711, .T. ) ;
#13249=VERTEX_POINT ( 'NONE', #8997 ) ;
#13251=CARTESIAN_POINT ( 'NONE',  ( 34.00000000000000000, -11.99999999999997335, 0.000000000000000000 ) ) ;
#13252=AXIS2_PLACEMENT_3D ( 'NONE', #24620, #15612, #44900 ) ;
#13255=ORIENTED_EDGE ( 'NONE', *, *, #53823, .F. ) ;
#13256=ORIENTED_EDGE ( 'NONE', *, *, #34718, .F. ) ;
#13257=CARTESIAN_POINT ( 'NONE',  ( 12.49336221634852429, 0.1658369216508863153, 13.50000000000000355 ) ) ;
#13260=CARTESIAN_POINT ( 'NONE',  ( -35.00000000000000000, -0.4871980014162358152, 12.74068829017553739 ) ) ;
#13261=DIRECTION ( 'NONE',  ( -1.000000000000000000, 0.000000000000000000, 0.000000000000000000 ) ) ;
#13262=FACE_OUTER_BOUND ( 'NONE', #27646, .T. ) ;
#13263=ADVANCED_FACE ( 'NONE', ( #9628 ), #58916, .T. ) ;
#13264=DIRECTION ( 'NONE',  ( -1.000000000000000000, 0.000000000000000000, 0.000000000000000000 ) ) ;
#13265=VERTEX_POINT ( 'NONE', #9300 ) ;
#13266=DIRECTION ( 'NONE',  ( -1.000000000000000000, -0.000000000000000000, -0.000000000000000000 ) ) ;
#13268=DIRECTION ( 'NONE',  ( 1.000000000000000000, 0.000000000000000000, -0.000000000000000000 ) ) ;
#13270=CARTESIAN_POINT ( 'NONE',  ( -18.11422852383967452, 13.12233133686801345, 3.247147390179137449 ) ) ;
#13271=CARTESIAN_POINT ( 'NONE',  ( 22.57855258442564761, -4.427776684447072952, 12.75322679295976691 ) ) ;
#13273=CARTESIAN_POINT ( 'NONE',  ( -37.00000000000000711, 11.10408318471068689, -6.265926637539373623 ) ) ;
#13275=AXIS2_PLACEMENT_3D ( 'NONE', #46636, #32622, #1090 ) ;
#13279=ORIENTED_EDGE ( 'NONE', *, *, #3641, .T. ) ;
#13281=CARTESIAN_POINT ( 'NONE',  ( 37.00000000000000711, 2.185196060784047045, 11.54110654723646157 ) ) ;
#13282=CARTESIAN_POINT ( 'NONE',  ( 11.98523602762309537, -10.93063363335638272, -7.929333770360376121 ) ) ;
#13286=LINE ( 'NONE', #18929, #32112 ) ;
#13287=ADVANCED_FACE ( 'NONE', ( #3378 ), #44896, .T. ) ;
#13288=DIRECTION ( 'NONE',  ( -1.000000000000000000, 0.000000000000000000, -0.000000000000000000 ) ) ;
#13289=CARTESIAN_POINT ( 'NONE',  ( 47.00000000000000711, 4.705694406421931860E-17, -3.469127814946512892E-15 ) ) ;
#13291=EDGE_LOOP ( 'NONE', ( #58125, #44885, #28268, #48181 ) ) ;
#13294=DIRECTION ( 'NONE',  ( 1.000000000000000000, 0.000000000000000000, 0.000000000000000000 ) ) ;
#13295=ADVANCED_FACE ( 'NONE', ( #13643 ), #19645, .T. ) ;
#13296=EDGE_CURVE ( 'NONE', #22914, #1326, #21343, .T. ) ;
#13297=EDGE_CURVE ( 'NONE', #50524, #21944, #20298, .T. ) ;
#13298=ORIENTED_EDGE ( 'NONE', *, *, #51785, .T. ) ;
#13299=ORIENTED_EDGE ( 'NONE', *, *, #4744, .T. ) ;
#13300=CARTESIAN_POINT ( 'NONE',  ( -9.502271734863095176, 12.89234648065891875, -4.021717619241973907 ) ) ;
#13301=ORIENTED_EDGE ( 'NONE', *, *, #51893, .F. ) ;
#13302=CARTESIAN_POINT ( 'NONE',  ( -37.00000000000000711, -6.584150480049622445, 10.25474254703950905 ) ) ;
#13303=DIRECTION ( 'NONE',  ( 0.000000000000000000, -0.3554799084908832896, -0.9346839223284592046 ) ) ;
#13304=DIRECTION ( 'NONE',  ( 0.000000000000000000, 0.01356324068817992175, -0.9999080150203990547 ) ) ;
#13305=CYLINDRICAL_SURFACE ( 'NONE', #29001, 12.18649999999999878 ) ;
#13307=EDGE_LOOP ( 'NONE', ( #30891, #47911, #37853, #34978 ) ) ;
#13311=EDGE_CURVE ( 'NONE', #32907, #12370, #124, .T. ) ;
#13312=AXIS2_PLACEMENT_3D ( 'NONE', #25287, #24978, #14633 ) ;
#13314=ORIENTED_EDGE ( 'NONE', *, *, #53865, .T. ) ;
#13317=DIRECTION ( 'NONE',  ( -1.000000000000000000, -1.836970198721029688E-16, 0.000000000000000000 ) ) ;
#13318=EDGE_LOOP ( 'NONE', ( #35936, #58497, #13355, #22755 ) ) ;
#13320=DIRECTION ( 'NONE',  ( -1.000000000000000000, 0.000000000000000000, 0.000000000000000000 ) ) ;
#13321=CARTESIAN_POINT ( 'NONE',  ( 35.00000000000000000, -12.17626345777663310, 0.4993900848168664752 ) ) ;
#13325=ORIENTED_EDGE ( 'NONE', *, *, #8383, .F. ) ;
#13326=DIRECTION ( 'NONE',  ( 0.000000000000000000, 0.4380125133593912312, -0.8989688749565187820 ) ) ;
#13329=DIRECTION ( 'NONE',  ( 0.000000000000000000, 0.01356324068817991828, -0.9999080150203990547 ) ) ;
#13331=CARTESIAN_POINT ( 'NONE',  ( 37.00000000000000711, 12.14284015767851344, 1.030638227056429157 ) ) ;
#13332=DIRECTION ( 'NONE',  ( 0.000000000000000000, -0.01356324068817998940, 0.9999080150203990547 ) ) ;
#13333=CYLINDRICAL_SURFACE ( 'NONE', #35545, 5.000000000000000888 ) ;
#13334=ORIENTED_EDGE ( 'NONE', *, *, #8018, .F. ) ;
#13335=CARTESIAN_POINT ( 'NONE',  ( -36.00000000000000711, 4.237174932027226504, 12.02534193257722528 ) ) ;
#13336=AXIS2_PLACEMENT_3D ( 'NONE', #44839, #65118, #14879 ) ;
#13339=DIRECTION ( 'NONE',  ( -1.000000000000000000, 0.000000000000000000, -0.000000000000000000 ) ) ;
#13341=CARTESIAN_POINT ( 'NONE',  ( -14.11589373245165469, 8.250315036047107142, 8.713914264323175729 ) ) ;
#13344=CIRCLE ( 'NONE', #20749, 12.18650000000000055 ) ;
#13345=EDGE_LOOP ( 'NONE', ( #52255, #51777, #36537, #13314 ) ) ;
#13346=VERTEX_POINT ( 'NONE', #20621 ) ;
#13350=CARTESIAN_POINT ( 'NONE',  ( -25.74809257979862309, -12.21955862071013676, 5.740220618591444612 ) ) ;
#13351=CARTESIAN_POINT ( 'NONE',  ( -37.00000000000000711, 0.000000000000000000, 0.000000000000000000 ) ) ;
#13352=CARTESIAN_POINT ( 'NONE',  ( 18.84867683979355846, 5.944105725974518251, 12.12095735156415088 ) ) ;
#13353=CARTESIAN_POINT ( 'NONE',  ( -35.00000000000000000, 0.000000000000000000, 0.000000000000000000 ) ) ;
#13355=ORIENTED_EDGE ( 'NONE', *, *, #50683, .F. ) ;
#13358=EDGE_CURVE ( 'NONE', #49507, #36860, #35177, .T. ) ;
#13359=CARTESIAN_POINT ( 'NONE',  ( -27.01437459610461644, -13.31613970204372421, -2.220455681983950935 ) ) ;
#13360=CARTESIAN_POINT ( 'NONE',  ( 23.90122759429952026, 11.31311706520687288, -7.370651591097819200 ) ) ;
#13361=LINE ( 'NONE', #18374, #47680 ) ;
#13362=CARTESIAN_POINT ( 'NONE',  ( 35.00000000000000000, -12.15823808070322798, -0.8294751490778934366 ) ) ;
#13363=CARTESIAN_POINT ( 'NONE',  ( 6.598188397287249707, -8.822549351475428736, -8.136977447280584030 ) ) ;
#13365=VECTOR ( 'NONE', #11043, 1000.000000000000000 ) ;
#13366=ORIENTED_EDGE ( 'NONE', *, *, #65726, .F. ) ;
#13367=DIRECTION ( 'NONE',  ( -0.000000000000000000, -1.000000000000000000, -0.000000000000000000 ) ) ;
#13368=CIRCLE ( 'NONE', #53783, 5.000000000000000888 ) ;
#13372=DIRECTION ( 'NONE',  ( -1.000000000000000000, -0.000000000000000000, 0.000000000000000000 ) ) ;
#13373=ORIENTED_EDGE ( 'NONE', *, *, #52480, .F. ) ;
#13374=FACE_OUTER_BOUND ( 'NONE', #22044, .T. ) ;
#13375=VERTEX_POINT ( 'NONE', #20278 ) ;
#13376=ORIENTED_EDGE ( 'NONE', *, *, #27283, .F. ) ;
#13377=ORIENTED_EDGE ( 'NONE', *, *, #1969, .T. ) ;
#13379=CYLINDRICAL_SURFACE ( 'NONE', #62057, 12.18650000000000055 ) ;
#13380=CIRCLE ( 'NONE', #9109, 12.74999999999999822 ) ;
#13382=ORIENTED_EDGE ( 'NONE', *, *, #21731, .T. ) ;
#13384=DIRECTION ( 'NONE',  ( 0.000000000000000000, 0.9937233664769765662, -0.1118654143051580896 ) ) ;
#13385=CARTESIAN_POINT ( 'NONE',  ( -35.00000000000000000, 4.018060380616562455, -11.50504120060938718 ) ) ;
#13386=CARTESIAN_POINT ( 'NONE',  ( 19.21199004881496109, 2.638489798294652022, 11.74470497263192748 ) ) ;
#13387=ORIENTED_EDGE ( 'NONE', *, *, #45974, .T. ) ;
#13389=CARTESIAN_POINT ( 'NONE',  ( -35.00000000000000000, 6.547236723514155976, -9.752226076388824438 ) ) ;
#13391=CARTESIAN_POINT ( 'NONE',  ( -29.60271627082680368, -3.677907232733512721, 11.42254165076253614 ) ) ;
#13392=DIRECTION ( 'NONE',  ( 0.000000000000000000, -0.8369827122275401710, -0.5472293298355184188 ) ) ;
#13395=VERTEX_POINT ( 'NONE', #41530 ) ;
#13396=DIRECTION ( 'NONE',  ( 0.000000000000000000, -0.01356324068817998940, 0.9999080150203990547 ) ) ;
#13397=EDGE_CURVE ( 'NONE', #395, #37649, #30262, .T. ) ;
#13398=ORIENTED_EDGE ( 'NONE', *, *, #50647, .F. ) ;
#13399=DIRECTION ( 'NONE',  ( 0.000000000000000000, -0.01356324068818000328, 0.9999080150203990547 ) ) ;
#13402=DIRECTION ( 'NONE',  ( 0.000000000000000000, -0.3554799084908833451, -0.9346839223284592046 ) ) ;
#13403=EDGE_CURVE ( 'NONE', #29231, #12206, #37325, .T. ) ;
#13406=DIRECTION ( 'NONE',  ( 0.000000000000000000, -0.01356324068817998940, 0.9999080150203990547 ) ) ;
#13407=VERTEX_POINT ( 'NONE', #65485 ) ;
#13408=CARTESIAN_POINT ( 'NONE',  ( 35.00000000000000000, 1.908798535168558352, 12.60630747491660664 ) ) ;
#13410=ORIENTED_EDGE ( 'NONE', *, *, #28389, .T. ) ;
#13413=CARTESIAN_POINT ( 'NONE',  ( 37.00000000000000711, -12.38385022362083987, -3.033604067594535714 ) ) ;
#13416=DIRECTION ( 'NONE',  ( -1.000000000000000000, 0.000000000000000000, -0.000000000000000000 ) ) ;
#13418=CYLINDRICAL_SURFACE ( 'NONE', #52528, 13.50000000000000178 ) ;
#13422=DIRECTION ( 'NONE',  ( -1.000000000000000000, 0.000000000000000000, -0.000000000000000000 ) ) ;
#13424=ADVANCED_FACE ( 'NONE', ( #342 ), #56176, .F. ) ;
#13425=CARTESIAN_POINT ( 'NONE',  ( -35.00000000000000000, 0.000000000000000000, 0.000000000000000000 ) ) ;
#13427=CARTESIAN_POINT ( 'NONE',  ( 37.00000000000000711, -12.08151691381187298, 4.074242145636131518 ) ) ;
#13430=EDGE_CURVE ( 'NONE', #22711, #21005, #2327, .T. ) ;
#13431=CARTESIAN_POINT ( 'NONE',  ( -8.737571515103036646, -2.833124800313057801, 13.20164519060687347 ) ) ;
#13432=VERTEX_POINT ( 'NONE', #55535 ) ;
#13433=DIRECTION ( 'NONE',  ( -1.000000000000000000, 0.000000000000000000, 0.000000000000000000 ) ) ;
#13437=DIRECTION ( 'NONE',  ( -1.000000000000000000, -0.000000000000000000, 0.000000000000000000 ) ) ;
#13439=ORIENTED_EDGE ( 'NONE', *, *, #18793, .T. ) ;
#13441=CARTESIAN_POINT ( 'NONE',  ( -9.806951085677328095, -9.949905073136244837, -6.721768133878152085 ) ) ;
#13442=CARTESIAN_POINT ( 'NONE',  ( -18.01809167125681910, 3.277815084079592989, -11.54557337376306769 ) ) ;
#13443=ORIENTED_EDGE ( 'NONE', *, *, #15551, .T. ) ;
#13444=CARTESIAN_POINT ( 'NONE',  ( 24.82652845881425208, 10.42385221765396608, -8.578654028722157321 ) ) ;
#13445=LINE ( 'NONE', #28746, #19212 ) ;
#13447=ORIENTED_EDGE ( 'NONE', *, *, #62441, .F. ) ;
#13448=AXIS2_PLACEMENT_3D ( 'NONE', #53247, #58577, #47286 ) ;
#13455=DIRECTION ( 'NONE',  ( 0.000000000000000000, -0.8169148498130213154, 0.5767582926625057782 ) ) ;
#13457=DIRECTION ( 'NONE',  ( 0.000000000000000000, -0.01356324068817991828, 0.9999080150203990547 ) ) ;
#13458=VERTEX_POINT ( 'NONE', #10963 ) ;
#13459=FACE_OUTER_BOUND ( 'NONE', #27049, .T. ) ;
#13461=DIRECTION ( 'NONE',  ( 1.000000000000000000, 0.000000000000000000, -0.000000000000000000 ) ) ;
#13462=ORIENTED_EDGE ( 'NONE', *, *, #10269, .F. ) ;
#13465=CARTESIAN_POINT ( 'NONE',  ( -36.00000000000000711, -12.74068829017553561, -0.4871980014162809458 ) ) ;
#13467=LINE ( 'NONE', #18506, #56634 ) ;
#13470=CARTESIAN_POINT ( 'NONE',  ( -37.00000000000000711, 0.000000000000000000, 0.000000000000000000 ) ) ;
#13474=DIRECTION ( 'NONE',  ( 1.000000000000000000, 0.000000000000000000, 0.000000000000000000 ) ) ;
#13475=CARTESIAN_POINT ( 'NONE',  ( 37.00000000000000711, 4.705694406421931860E-17, -3.469127814946512892E-15 ) ) ;
#13477=DIRECTION ( 'NONE',  ( 0.000000000000000000, -0.01356324068817999114, 0.9999080150203989437 ) ) ;
#13482=LINE ( 'NONE', #64667, #60259 ) ;
#13483=CARTESIAN_POINT ( 'NONE',  ( -36.00000000000000711, -9.913596905230058098, -8.017674001891890612 ) ) ;
#13484=CARTESIAN_POINT ( 'NONE',  ( -29.46184535117399150, 0.7194508147655768182, 13.48249488223129688 ) ) ;
#13485=EDGE_CURVE ( 'NONE', #62894, #58300, #59653, .T. ) ;
#13487=EDGE_LOOP ( 'NONE', ( #55194, #39584, #58210, #49716 ) ) ;
#13489=ORIENTED_EDGE ( 'NONE', *, *, #22545, .F. ) ;
#13490=ADVANCED_FACE ( 'NONE', ( #1657, #21926 ), #42498, .F. ) ;
#13491=CARTESIAN_POINT ( 'NONE',  ( 12.47628546223243617, 0.000000000000000000, 25.00000000000000000 ) ) ;
#13493=VECTOR ( 'NONE', #8032, 1000.000000000000000 ) ;
#13496=DIRECTION ( 'NONE',  ( 1.000000000000000000, -0.000000000000000000, 0.000000000000000000 ) ) ;
#13497=CARTESIAN_POINT ( 'NONE',  ( -35.00000000000000000, 0.000000000000000000, 0.000000000000000000 ) ) ;
#13498=AXIS2_PLACEMENT_3D ( 'NONE', #33911, #30476, #54213 ) ;
#13499=ADVANCED_FACE ( 'NONE', ( #42847 ), #63135, .T. ) ;
#13500=CARTESIAN_POINT ( 'NONE',  ( 7.273419175973108608, -6.815651482458461530, -11.65514903918486311 ) ) ;
#13503=CARTESIAN_POINT ( 'NONE',  ( -35.00000000000000000, 9.217970097227725645, 7.971186206369506699 ) ) ;
#13504=DIRECTION ( 'NONE',  ( 1.000000000000000000, -0.000000000000000000, 0.000000000000000000 ) ) ;
#13505=EDGE_CURVE ( 'NONE', #54151, #24707, #58585, .T. ) ;
#13507=DIRECTION ( 'NONE',  ( -1.000000000000000000, -0.000000000000000000, 0.000000000000000000 ) ) ;
#13509=DIRECTION ( 'NONE',  ( 1.000000000000000000, 0.000000000000000000, 0.000000000000000000 ) ) ;
#13510=EDGE_CURVE ( 'NONE', #51925, #65451, #41552, .T. ) ;
#13514=ORIENTED_EDGE ( 'NONE', *, *, #49573, .T. ) ;
#13515=DIRECTION ( 'NONE',  ( 0.000000000000000000, 0.01356324068817992175, -0.9999080150203990547 ) ) ;
#13519=EDGE_LOOP ( 'NONE', ( #17356, #2872, #17326, #23361 ) ) ;
#13522=LINE ( 'NONE', #48477, #8417 ) ;
#13523=DIRECTION ( 'NONE',  ( -1.000000000000000000, 0.000000000000000000, 0.000000000000000000 ) ) ;
#13525=DIRECTION ( 'NONE',  ( 0.000000000000000000, 0.04924826701374583615, 0.9987865678893277366 ) ) ;
#13526=AXIS2_PLACEMENT_3D ( 'NONE', #24045, #23728, #43996 ) ;
#13527=CARTESIAN_POINT ( 'NONE',  ( 37.00000000000000711, -5.015831474386232891, 10.62137734850272786 ) ) ;
#13528=ORIENTED_EDGE ( 'NONE', *, *, #59174, .T. ) ;
#13530=CARTESIAN_POINT ( 'NONE',  ( -35.00000000000000000, 7.971186206369601734, -9.217970097227642157 ) ) ;
#13533=CARTESIAN_POINT ( 'NONE',  ( -36.00000000000000711, 1.738225594539995589, 12.63095688309029718 ) ) ;
#13536=DIRECTION ( 'NONE',  ( 1.000000000000000000, 0.000000000000000000, 0.000000000000000000 ) ) ;
#13538=VERTEX_POINT ( 'NONE', #49501 ) ;
#13541=EDGE_LOOP ( 'NONE', ( #40958, #44770, #9537, #38428 ) ) ;
#13542=VECTOR ( 'NONE', #55784, 1000.000000000000000 ) ;
#13544=CARTESIAN_POINT ( 'NONE',  ( -35.00000000000000000, -11.56998259273174945, -3.827046518385204266 ) ) ;
#13547=CIRCLE ( 'NONE', #49557, 12.75000000000000178 ) ;
#13549=ORIENTED_EDGE ( 'NONE', *, *, #6461, .T. ) ;
#13550=CARTESIAN_POINT ( 'NONE',  ( 35.00000000000000000, 3.645068577060024850, -11.16627499335656815 ) ) ;
#13552=FACE_OUTER_BOUND ( 'NONE', #26376, .T. ) ;
#13553=ORIENTED_EDGE ( 'NONE', *, *, #27265, .F. ) ;
#13554=VERTEX_POINT ( 'NONE', #18598 ) ;
#13555=CARTESIAN_POINT ( 'NONE',  ( -35.00000000000000000, -12.42372387097880271, -2.865935305911757602 ) ) ;
#13556=DIRECTION ( 'NONE',  ( -1.000000000000000000, 0.000000000000000000, 0.000000000000000000 ) ) ;
#13557=ADVANCED_FACE ( 'NONE', ( #64428 ), #65085, .T. ) ;
#13559=ORIENTED_EDGE ( 'NONE', *, *, #37716, .T. ) ;
#13562=CARTESIAN_POINT ( 'NONE',  ( -37.00000000000000711, 6.036400161834567513, 10.07641281632180075 ) ) ;
#13563=CYLINDRICAL_SURFACE ( 'NONE', #12574, 5.000000000000000888 ) ;
#13566=ORIENTED_EDGE ( 'NONE', *, *, #58206, .F. ) ;
#13568=CARTESIAN_POINT ( 'NONE',  ( -17.31370294542102428, 7.098634700851768287, 9.677313122349437080 ) ) ;
#13569=CARTESIAN_POINT ( 'NONE',  ( -20.73706235180480562, -13.15925562679262306, -3.065506255066365426 ) ) ;
#13570=EDGE_CURVE ( 'NONE', #57717, #60184, #43291, .T. ) ;
#13573=CYLINDRICAL_SURFACE ( 'NONE', #31826, 12.75000000000000178 ) ;
#13576=CARTESIAN_POINT ( 'NONE',  ( -17.29244623348158783, 2.525873743887551814, 13.26159725786978960 ) ) ;
#13577=CIRCLE ( 'NONE', #27396, 12.75000000000000178 ) ;
#13579=CARTESIAN_POINT ( 'NONE',  ( -35.00000000000000000, -6.547236723514086698, 9.752226076388870624 ) ) ;
#13580=AXIS2_PLACEMENT_3D ( 'NONE', #63062, #37793, #22843 ) ;
#13583=CARTESIAN_POINT ( 'NONE',  ( 37.00000000000000711, 2.865935305911624376, -12.42372387097883646 ) ) ;
#13584=DIRECTION ( 'NONE',  ( -1.000000000000000000, 0.000000000000000000, 0.000000000000000000 ) ) ;
#13586=AXIS2_PLACEMENT_3D ( 'NONE', #28380, #49355, #55283 ) ;
#13588=DIRECTION ( 'NONE',  ( 1.000000000000000000, 0.000000000000000000, -0.000000000000000000 ) ) ;
#13589=ORIENTED_EDGE ( 'NONE', *, *, #19448, .T. ) ;
#13590=CARTESIAN_POINT ( 'NONE',  ( 35.00000000000000000, 2.497432891016841960, -11.47758908105695319 ) ) ;
#13592=CARTESIAN_POINT ( 'NONE',  ( 9.376659010705683528, 2.637162270932692731, 11.70861080908859364 ) ) ;
#13593=VECTOR ( 'NONE', #60949, 1000.000000000000000 ) ;
#13595=B_SPLINE_CURVE_WITH_KNOTS ( 'NONE', 3,
 ( #12598, #2678, #33872, #32878, #7635, #63796 ),
 .UNSPECIFIED., .F., .F.,
 ( 4, 2, 4 ),
 ( 0.01068930494538425542, 0.01246789317672156866, 0.01424648140805888016 ),
 .UNSPECIFIED. ) ;
#13596=ADVANCED_FACE ( 'NONE', ( #34504 ), #18252, .T. ) ;
#13599=ORIENTED_EDGE ( 'NONE', *, *, #54448, .T. ) ;
#13601=EDGE_CURVE ( 'NONE', #9962, #31780, #20391, .T. ) ;
#13602=ORIENTED_EDGE ( 'NONE', *, *, #49116, .F. ) ;
#13603=DIRECTION ( 'NONE',  ( 0.000000000000000000, -0.01356324068817999114, 0.9999080150203989437 ) ) ;
#13604=FACE_OUTER_BOUND ( 'NONE', #10207, .T. ) ;
#13610=DIRECTION ( 'NONE',  ( -1.000000000000000000, 0.000000000000000000, 0.000000000000000000 ) ) ;
#13612=CIRCLE ( 'NONE', #3066, 12.18649999999999878 ) ;
#13614=B_SPLINE_CURVE_WITH_KNOTS ( 'NONE', 3,
 ( #44795, #34165, #44458, #39815, #55440, #19208, #65076, #3627, #44154, #39151, #54474, #39481, #19551, #50469, #60102, #34798, #55103, #9532 ),
 .UNSPECIFIED., .F., .F.,
 ( 4, 2, 2, 2, 2, 2, 2, 2, 4 ),
 ( 0.000000000000000000, 0.001195117733165457262, 0.002390235466330913657, 0.003585353199496369835, 0.004780470932661826447, 0.005975588665827281758, 0.007170706398992739670, 0.008365824132158196716, 0.009560941865323654629 ),
 .UNSPECIFIED. ) ;
#13616=EDGE_LOOP ( 'NONE', ( #35772, #38314, #53222, #26450 ) ) ;
#13617=ORIENTED_EDGE ( 'NONE', *, *, #33160, .F. ) ;
#13618=ORIENTED_EDGE ( 'NONE', *, *, #56355, .T. ) ;
#13621=DIRECTION ( 'NONE',  ( 0.000000000000000000, -0.01356324068817999114, 0.9999080150203989437 ) ) ;
#13622=ADVANCED_FACE ( 'NONE', ( #3288 ), #4258, .T. ) ;
#13623=ORIENTED_EDGE ( 'NONE', *, *, #52240, .T. ) ;
#13624=DIRECTION ( 'NONE',  ( 0.000000000000000000, -0.01356324068817998940, 0.9999080150203990547 ) ) ;
#13626=EDGE_CURVE ( 'NONE', #41918, #52756, #38517, .T. ) ;
#13627=AXIS2_PLACEMENT_3D ( 'NONE', #42881, #52232, #47246 ) ;
#13628=VERTEX_POINT ( 'NONE', #43837 ) ;
#13629=CIRCLE ( 'NONE', #10452, 12.18650000000000411 ) ;
#13630=LINE ( 'NONE', #34568, #38621 ) ;
#13632=DIRECTION ( 'NONE',  ( -1.000000000000000000, 0.000000000000000000, 0.000000000000000000 ) ) ;
#13633=ORIENTED_EDGE ( 'NONE', *, *, #16749, .T. ) ;
#13634=ORIENTED_EDGE ( 'NONE', *, *, #25589, .T. ) ;
#13636=VERTEX_POINT ( 'NONE', #64118 ) ;
#13641=VECTOR ( 'NONE', #56440, 1000.000000000000000 ) ;
#13643=FACE_OUTER_BOUND ( 'NONE', #6056, .T. ) ;
#13647=DIRECTION ( 'NONE',  ( 1.000000000000000000, 0.000000000000000000, 0.000000000000000000 ) ) ;
#13648=ORIENTED_EDGE ( 'NONE', *, *, #33177, .T. ) ;
#13649=FACE_OUTER_BOUND ( 'NONE', #50783, .T. ) ;
#13650=ORIENTED_EDGE ( 'NONE', *, *, #56308, .F. ) ;
#13651=CARTESIAN_POINT ( 'NONE',  ( -35.00000000000000000, 0.000000000000000000, 0.000000000000000000 ) ) ;
#13653=EDGE_CURVE ( 'NONE', #65068, #64141, #65404, .T. ) ;
#13655=CARTESIAN_POINT ( 'NONE',  ( -14.65407954714387451, 8.414523573697247016, 8.555553591160615312 ) ) ;
#13656=DIRECTION ( 'NONE',  ( 0.000000000000000000, -0.01356324068817998940, 0.9999080150203990547 ) ) ;
#13658=EDGE_CURVE ( 'NONE', #50699, #60788, #15007, .T. ) ;
#13660=VECTOR ( 'NONE', #19247, 1000.000000000000000 ) ;
#13661=ORIENTED_EDGE ( 'NONE', *, *, #19704, .F. ) ;
#13662=CARTESIAN_POINT ( 'NONE',  ( 37.00000000000000711, 4.705694406421931860E-17, -3.469127814946512892E-15 ) ) ;
#13663=CIRCLE ( 'NONE', #21108, 12.75000000000000178 ) ;
#13667=CARTESIAN_POINT ( 'NONE',  ( -29.61524753723641012, 2.148738662487795992, 13.35711602759049654 ) ) ;
#13668=DIRECTION ( 'NONE',  ( 0.000000000000000000, -0.8696919319575129315, -0.4935949184179356242 ) ) ;
#13672=DIRECTION ( 'NONE',  ( 0.000000000000000000, -0.01356324068817999114, 0.9999080150203989437 ) ) ;
#13675=AXIS2_PLACEMENT_3D ( 'NONE', #52654, #27352, #22364 ) ;
#13676=EDGE_CURVE ( 'NONE', #10290, #11977, #10745, .T. ) ;
#13679=CARTESIAN_POINT ( 'NONE',  ( 35.00000000000000000, 12.12087942037209842, -1.262958560998807656 ) ) ;
#13680=CARTESIAN_POINT ( 'NONE',  ( 35.00000000000000000, 8.839356091080166067, 8.389074212634184846 ) ) ;
#13683=CARTESIAN_POINT ( 'NONE',  ( 37.00000000000000711, 5.710938531231874116, 11.39945968423464784 ) ) ;
#13684=CARTESIAN_POINT ( 'NONE',  ( -37.00000000000000711, 8.766823244862097297, -7.817610399097422835 ) ) ;
#13685=CIRCLE ( 'NONE', #39180, 12.18649999999999878 ) ;
#13686=ORIENTED_EDGE ( 'NONE', *, *, #39630, .F. ) ;
#13687=DIRECTION ( 'NONE',  ( 0.000000000000000000, -0.04924826701373161142, -0.9987865678893286248 ) ) ;
#13689=CARTESIAN_POINT ( 'NONE',  ( -14.29135464769095520, 7.782112657557433089, -9.134479874907182051 ) ) ;
#13691=CYLINDRICAL_SURFACE ( 'NONE', #48096, 12.18649999999999878 ) ;
#13692=CARTESIAN_POINT ( 'NONE',  ( 35.00000000000000000, -12.74921544981110699, 0.1414404973753423111 ) ) ;
#13693=ORIENTED_EDGE ( 'NONE', *, *, #5635, .F. ) ;
#13694=VERTEX_POINT ( 'NONE', #46449 ) ;
#13695=VERTEX_POINT ( 'NONE', #50788 ) ;
#13698=ORIENTED_EDGE ( 'NONE', *, *, #42763, .F. ) ;
#13700=CARTESIAN_POINT ( 'NONE',  ( 37.00000000000000711, -6.102719229070595830, 10.54834585426226390 ) ) ;
#13705=CARTESIAN_POINT ( 'NONE',  ( -27.27855387000350262, -10.59660315834921107, 5.631341004100471892 ) ) ;
#13709=CARTESIAN_POINT ( 'NONE',  ( 11.74548640120467979, -8.775604215601116920, -8.184666801472349817 ) ) ;
#13710=EDGE_LOOP ( 'NONE', ( #58094, #29153, #36874, #1933 ) ) ;
#13711=ORIENTED_EDGE ( 'NONE', *, *, #9196, .F. ) ;
#13715=CIRCLE ( 'NONE', #59389, 12.18649999999999878 ) ;
#13716=DIRECTION ( 'NONE',  ( 1.000000000000000000, -0.000000000000000000, 0.000000000000000000 ) ) ;
#13717=CIRCLE ( 'NONE', #39207, 4.999999999999999112 ) ;
#13718=CARTESIAN_POINT ( 'NONE',  ( -35.00000000000000000, 10.80631716521666874, 4.603882218679588689 ) ) ;
#13719=CARTESIAN_POINT ( 'NONE',  ( -11.40165637462999904, -7.508992741355383416, 9.360289953322597611 ) ) ;
#13720=ADVANCED_FACE ( 'NONE', ( #61092 ), #24870, .T. ) ;
#13722=CARTESIAN_POINT ( 'NONE',  ( 35.00000000000000000, 11.78745411414844035, 3.093009498343795460 ) ) ;
#13723=CARTESIAN_POINT ( 'NONE',  ( -37.00000000000000711, -7.251710744571512102, -9.240395740215712195 ) ) ;
#13724=VECTOR ( 'NONE', #62418, 1000.000000000000000 ) ;
#13725=VERTEX_POINT ( 'NONE', #5238 ) ;
#13726=CARTESIAN_POINT ( 'NONE',  ( -4.989057617119008192, -0.9162120371760335003, 13.46887357958837406 ) ) ;
#13730=FACE_OUTER_BOUND ( 'NONE', #12992, .T. ) ;
#13733=CARTESIAN_POINT ( 'NONE',  ( 35.00000000000000000, -11.67026961469347768, -4.564151185897032725 ) ) ;
#13735=CYLINDRICAL_SURFACE ( 'NONE', #51823, 12.74999999999999822 ) ;
#13739=ORIENTED_EDGE ( 'NONE', *, *, #34777, .F. ) ;
#13740=LINE ( 'NONE', #19078, #2085 ) ;
#13742=CARTESIAN_POINT ( 'NONE',  ( -17.55122397361593656, -9.296840455340431575, 9.807752914019381763 ) ) ;
#13743=ORIENTED_EDGE ( 'NONE', *, *, #43880, .T. ) ;
#13744=EDGE_CURVE ( 'NONE', #5815, #40304, #20335, .T. ) ;
#13746=CIRCLE ( 'NONE', #26527, 12.75000000000000178 ) ;
#13748=CARTESIAN_POINT ( 'NONE',  ( -10.22406655687136023, -4.688833681473150605, 12.66448649920025993 ) ) ;
#13752=FACE_OUTER_BOUND ( 'NONE', #11897, .T. ) ;
#13753=AXIS2_PLACEMENT_3D ( 'NONE', #31927, #15649, #22282 ) ;
#13754=EDGE_CURVE ( 'NONE', #266, #54167, #28838, .T. ) ;
#13755=CARTESIAN_POINT ( 'NONE',  ( -25.86628395826706850, 5.139808748864376220, 10.84354029019568522 ) ) ;
#13756=CARTESIAN_POINT ( 'NONE',  ( -35.00000000000000000, -8.352657516904613999, -8.258652103341526995 ) ) ;
#13760=CARTESIAN_POINT ( 'NONE',  ( -9.830496058488753519, -10.61724537947942260, -5.608865105245247840 ) ) ;
#13762=ORIENTED_EDGE ( 'NONE', *, *, #48526, .F. ) ;
#13763=DIRECTION ( 'NONE',  ( 0.000000000000000000, 0.01356324068817992175, -0.9999080150203990547 ) ) ;
#13764=CARTESIAN_POINT ( 'NONE',  ( -37.00000000000000711, -12.71517666308948691, 0.9416912585473986574 ) ) ;
#13765=VERTEX_POINT ( 'NONE', #27467 ) ;
#13768=CARTESIAN_POINT ( 'NONE',  ( 35.00000000000000000, 11.02904044024202967, -4.041347439436060007 ) ) ;
#13769=ORIENTED_EDGE ( 'NONE', *, *, #7929, .F. ) ;
#13770=DIRECTION ( 'NONE',  ( -1.000000000000000000, 0.000000000000000000, -0.000000000000000000 ) ) ;
#13774=EDGE_CURVE ( 'NONE', #32833, #60184, #36628, .T. ) ;
#13775=CARTESIAN_POINT ( 'NONE',  ( 35.00000000000000000, -7.376655759824808811, 9.700295462048739381 ) ) ;
#13779=CARTESIAN_POINT ( 'NONE',  ( -35.00000000000000000, 11.61976888909158490, 3.827969819614504221 ) ) ;
#13780=ORIENTED_EDGE ( 'NONE', *, *, #56771, .F. ) ;
#13781=DIRECTION ( 'NONE',  ( -1.000000000000000000, -1.836970198721029688E-16, -0.000000000000000000 ) ) ;
#13782=EDGE_LOOP ( 'NONE', ( #10141, #30381, #65082, #31714 ) ) ;
#13783=ORIENTED_EDGE ( 'NONE', *, *, #13883, .T. ) ;
#13784=CARTESIAN_POINT ( 'NONE',  ( -25.66858381519323018, 8.266157983362676376, 10.67702105760074183 ) ) ;
#13786=DIRECTION ( 'NONE',  ( 1.000000000000000000, 0.000000000000000000, -0.000000000000000000 ) ) ;
#13787=AXIS2_PLACEMENT_3D ( 'NONE', #48876, #37232, #22620 ) ;
#13788=AXIS2_PLACEMENT_3D ( 'NONE', #62395, #52460, #65016 ) ;
#13789=EDGE_CURVE ( 'NONE', #25348, #65337, #34140, .T. ) ;
#13791=CARTESIAN_POINT ( 'NONE',  ( 3.459614771489464946, -11.09853614738469396, -4.563167253695070258 ) ) ;
#13793=ORIENTED_EDGE ( 'NONE', *, *, #4514, .T. ) ;
#13796=LINE ( 'NONE', #15375, #62948 ) ;
#13797=ORIENTED_EDGE ( 'NONE', *, *, #34242, .T. ) ;
#13800=DIRECTION ( 'NONE',  ( 1.000000000000000000, 0.000000000000000000, 0.000000000000000000 ) ) ;
#13801=CARTESIAN_POINT ( 'NONE',  ( 35.00000000000000000, -5.273331777780263074, 10.49591321039685887 ) ) ;
#13802=CIRCLE ( 'NONE', #41426, 5.000000000000001776 ) ;
#13803=CARTESIAN_POINT ( 'NONE',  ( 37.00000000000000711, 2.497432891016841960, -11.47758908105695319 ) ) ;
#13804=EDGE_CURVE ( 'NONE', #21959, #63611, #5512, .T. ) ;
#13806=CIRCLE ( 'NONE', #59491, 5.000000000000000888 ) ;
#13807=ORIENTED_EDGE ( 'NONE', *, *, #20024, .T. ) ;
#13808=ORIENTED_EDGE ( 'NONE', *, *, #134, .T. ) ;
#13809=DIRECTION ( 'NONE',  ( 0.000000000000000000, -0.01356324068817998940, 0.9999080150203990547 ) ) ;
#13810=CYLINDRICAL_SURFACE ( 'NONE', #28713, 4.999999999999999112 ) ;
#13811=CIRCLE ( 'NONE', #20234, 12.75000000000000178 ) ;
#13814=CARTESIAN_POINT ( 'NONE',  ( -28.13819771402047820, 11.82670130915983719, -6.517207649538970138 ) ) ;
#13815=CIRCLE ( 'NONE', #12895, 4.999999999999999112 ) ;
#13816=DIRECTION ( 'NONE',  ( 0.000000000000000000, -0.01356324068817998940, 0.9999080150203990547 ) ) ;
#13817=DIRECTION ( 'NONE',  ( -1.000000000000000000, -1.836970198721029688E-16, 0.000000000000000000 ) ) ;
#13819=DIRECTION ( 'NONE',  ( 0.000000000000000000, 0.01356324068817992175, -0.9999080150203990547 ) ) ;
#13820=ORIENTED_EDGE ( 'NONE', *, *, #8664, .F. ) ;
#13823=FACE_OUTER_BOUND ( 'NONE', #17350, .T. ) ;
#13824=EDGE_CURVE ( 'NONE', #44305, #16743, #58080, .T. ) ;
#13825=AXIS2_PLACEMENT_3D ( 'NONE', #13351, #53927, #60531 ) ;
#13826=AXIS2_PLACEMENT_3D ( 'NONE', #59892, #24969, #18688 ) ;
#13827=AXIS2_PLACEMENT_3D ( 'NONE', #45194, #35197, #55502 ) ;
#13828=DIRECTION ( 'NONE',  ( -0.000000000000000000, -0.000000000000000000, -1.000000000000000000 ) ) ;
#13829=CARTESIAN_POINT ( 'NONE',  ( -28.15365128295566421, -11.30992368511472890, -4.022759283342765002 ) ) ;
#13831=DIRECTION ( 'NONE',  ( 1.000000000000000000, 0.000000000000000000, -0.000000000000000000 ) ) ;
#13835=CARTESIAN_POINT ( 'NONE',  ( -18.06443652845103642, 4.738606707596126455, -12.64292522309443001 ) ) ;
#13836=DIRECTION ( 'NONE',  ( 1.000000000000000000, 0.000000000000000000, 0.000000000000000000 ) ) ;
#13837=CARTESIAN_POINT ( 'NONE',  ( -15.27729454824424948, 5.151216734910788908, 25.00000000000000000 ) ) ;
#13838=CARTESIAN_POINT ( 'NONE',  ( -35.00000000000000000, 4.309077947445652867, 10.92721691015457708 ) ) ;
#13839=CARTESIAN_POINT ( 'NONE',  ( -7.489022030332961322, -8.034049540753116503, -10.84914964302385521 ) ) ;
#13841=EDGE_CURVE ( 'NONE', #44679, #43286, #56416, .T. ) ;
#13842=CARTESIAN_POINT ( 'NONE',  ( 35.00000000000000000, 5.300372733891642874, -11.59605747147788435 ) ) ;
#13843=ORIENTED_EDGE ( 'NONE', *, *, #2350, .F. ) ;
#13844=VECTOR ( 'NONE', #26841, 1000.000000000000000 ) ;
#13847=DIRECTION ( 'NONE',  ( -1.000000000000000000, 0.000000000000000000, 0.000000000000000000 ) ) ;
#13848=CARTESIAN_POINT ( 'NONE',  ( 37.00000000000000711, 11.66953048682399441, -3.511814412392164186 ) ) ;
#13849=LINE ( 'NONE', #53481, #53298 ) ;
#13851=DIRECTION ( 'NONE',  ( 1.000000000000000000, 0.000000000000000000, -0.000000000000000000 ) ) ;
#13852=EDGE_CURVE ( 'NONE', #817, #61894, #40377, .T. ) ;
#13856=EDGE_CURVE ( 'NONE', #28250, #4710, #19260, .T. ) ;
#13857=EDGE_LOOP ( 'NONE', ( #39044, #9398 ) ) ;
#13859=CIRCLE ( 'NONE', #62706, 5.000000000000000000 ) ;
#13860=ORIENTED_EDGE ( 'NONE', *, *, #16439, .T. ) ;
#13861=CARTESIAN_POINT ( 'NONE',  ( 37.00000000000000711, -11.47758908105696207, -2.497432891016804657 ) ) ;
#13863=CYLINDRICAL_SURFACE ( 'NONE', #38358, 4.999999999999998224 ) ;
#13868=EDGE_CURVE ( 'NONE', #8648, #57089, #63054, .T. ) ;
#13869=VERTEX_POINT ( 'NONE', #31792 ) ;
#13872=CIRCLE ( 'NONE', #30816, 4.999999999999999112 ) ;
#13873=LINE ( 'NONE', #48837, #35432 ) ;
#13874=ORIENTED_EDGE ( 'NONE', *, *, #33005, .T. ) ;
#13876=CARTESIAN_POINT ( 'NONE',  ( -35.00000000000000000, 11.73808581813437968, -0.4353888892048790038 ) ) ;
#13877=CYLINDRICAL_SURFACE ( 'NONE', #9263, 12.18649999999999878 ) ;
#13879=DIRECTION ( 'NONE',  ( 1.000000000000000000, 0.000000000000000000, 0.000000000000000000 ) ) ;
#13880=DIRECTION ( 'NONE',  ( 1.000000000000000000, 0.000000000000000000, -0.000000000000000000 ) ) ;
#13881=DIRECTION ( 'NONE',  ( 0.000000000000000000, -0.01356324068817991828, 0.9999080150203990547 ) ) ;
#13882=AXIS2_PLACEMENT_3D ( 'NONE', #15176, #35456, #55755 ) ;
#13883=EDGE_CURVE ( 'NONE', #44716, #54679, #27809, .T. ) ;
#13888=CARTESIAN_POINT ( 'NONE',  ( -16.50484331857675002, 7.681086090980186576, 9.219792269895048520 ) ) ;
#13889=EDGE_CURVE ( 'NONE', #4651, #52994, #11521, .T. ) ;
#13890=CARTESIAN_POINT ( 'NONE',  ( -20.33691237604007540, -13.28109756591637947, -2.496095192331454715 ) ) ;
#13891=DIRECTION ( 'NONE',  ( 0.000000000000000000, 0.9999080150203989437, 0.01356324068818348313 ) ) ;
#13893=CARTESIAN_POINT ( 'NONE',  ( 26.76876439064266222, 11.45740883406175570, 3.577846890752803155 ) ) ;
#13894=CARTESIAN_POINT ( 'NONE',  ( 37.00000000000000711, -8.235637554476713973, -9.733281772932137699 ) ) ;
#13895=CYLINDRICAL_SURFACE ( 'NONE', #5547, 12.18649999999999878 ) ;
#13896=CARTESIAN_POINT ( 'NONE',  ( -35.00000000000000000, -5.015831474386382105, 10.62137734850266391 ) ) ;
#13898=AXIS2_PLACEMENT_3D ( 'NONE', #9528, #65708, #25168 ) ;
#13899=CIRCLE ( 'NONE', #107, 5.000000000000000000 ) ;
#13900=ORIENTED_EDGE ( 'NONE', *, *, #57346, .T. ) ;
#13901=CARTESIAN_POINT ( 'NONE',  ( 37.00000000000000711, -12.70128625845191728, 1.113475361586618195 ) ) ;
#13902=AXIS2_PLACEMENT_3D ( 'NONE', #42601, #37647, #57943 ) ;
#13903=EDGE_LOOP ( 'NONE', ( #15745, #18905, #24981, #28900 ) ) ;
#13906=EDGE_CURVE ( 'NONE', #35917, #1946, #26825, .T. ) ;
#13908=CARTESIAN_POINT ( 'NONE',  ( -10.71762586082606639, -9.042033845899357658, 10.03605433748208853 ) ) ;
#13910=VERTEX_POINT ( 'NONE', #64358 ) ;
#13911=LINE ( 'NONE', #60138, #45136 ) ;
#13913=AXIS2_PLACEMENT_3D ( 'NONE', #2569, #2222, #17180 ) ;
#13914=CARTESIAN_POINT ( 'NONE',  ( 8.937200413559443390, 4.476360154859203355, 11.13383131558893346 ) ) ;
#13918=CARTESIAN_POINT ( 'NONE',  ( 35.00000000000000000, 10.43555801961475282, -5.391785509271000087 ) ) ;
#13919=ORIENTED_EDGE ( 'NONE', *, *, #56106, .T. ) ;
#13921=VERTEX_POINT ( 'NONE', #23825 ) ;
#13923=CARTESIAN_POINT ( 'NONE',  ( -35.00000000000000000, -7.094637218249277844, -10.59380114696477726 ) ) ;
#13925=EDGE_CURVE ( 'NONE', #28701, #34574, #34431, .T. ) ;
#13927=CARTESIAN_POINT ( 'NONE',  ( 6.633584127423891807, -5.026838569920903055, 12.53474721772208511 ) ) ;
#13932=ORIENTED_EDGE ( 'NONE', *, *, #28499, .F. ) ;
#13933=CYLINDRICAL_SURFACE ( 'NONE', #41385, 5.000000000000000888 ) ;
#13934=DIRECTION ( 'NONE',  ( -0.1699641022377680333, 0.000000000000000000, 0.9854502544271371844 ) ) ;
#13938=CYLINDRICAL_SURFACE ( 'NONE', #56249, 4.500030059823568074 ) ;
#13939=ORIENTED_EDGE ( 'NONE', *, *, #65051, .T. ) ;
#13940=ADVANCED_FACE ( 'NONE', ( #63690 ), #33460, .F. ) ;
#13941=B_SPLINE_CURVE_WITH_KNOTS ( 'NONE', 3,
 ( #48619, #8055, #59566, #28643, #29610, #14326, #49919, #24307, #34606, #18020, #3071, #23334, #44572, #43597, #18367, #38628 ),
 .UNSPECIFIED., .F., .F.,
 ( 4, 2, 2, 2, 2, 2, 2, 4 ),
 ( 4.091337135425211056E-18, 0.001225059573319686778, 0.001837589359979528107, 0.002450119146639369219, 0.003675178719959051876, 0.004900238293278734968, 0.007350357439918100283, 0.009800476586557464731 ),
 .UNSPECIFIED. ) ;
#13942=ORIENTED_EDGE ( 'NONE', *, *, #43442, .F. ) ;
#13943=ORIENTED_EDGE ( 'NONE', *, *, #25974, .T. ) ;
#13944=LINE ( 'NONE', #7320, #41543 ) ;
#13945=VECTOR ( 'NONE', #39741, 1000.000000000000000 ) ;
#13946=AXIS2_PLACEMENT_3D ( 'NONE', #35990, #10737, #41652 ) ;
#13947=CARTESIAN_POINT ( 'NONE',  ( 145.1370849898475797, 3.309064568108273190E-14, 0.000000000000000000 ) ) ;
#13948=ORIENTED_EDGE ( 'NONE', *, *, #25264, .T. ) ;
#13950=VECTOR ( 'NONE', #2993, 1000.000000000000000 ) ;
#13951=DIRECTION ( 'NONE',  ( 0.000000000000000000, 0.01356324068817998940, -0.9999080150203990547 ) ) ;
#13952=VERTEX_POINT ( 'NONE', #33116 ) ;
#13956=ADVANCED_FACE ( 'NONE', ( #44390 ), #43756, .T. ) ;
#13959=AXIS2_PLACEMENT_3D ( 'NONE', #50700, #5146, #25412 ) ;
#13962=EDGE_CURVE ( 'NONE', #56170, #15952, #57573, .T. ) ;
#13964=DIRECTION ( 'NONE',  ( 0.000000000000000000, -0.6745969609292717939, -0.7381862504171902151 ) ) ;
#13965=ORIENTED_EDGE ( 'NONE', *, *, #31100, .T. ) ;
#13968=ORIENTED_EDGE ( 'NONE', *, *, #16861, .T. ) ;
#13969=ADVANCED_FACE ( 'NONE', ( #9155 ), #64036, .T. ) ;
#13970=DIRECTION ( 'NONE',  ( 0.000000000000000000, -1.000000000000000000, 0.000000000000000000 ) ) ;
#13974=LINE ( 'NONE', #53593, #49399 ) ;
#13975=ORIENTED_EDGE ( 'NONE', *, *, #48450, .T. ) ;
#13976=EDGE_CURVE ( 'NONE', #13694, #47279, #64666, .T. ) ;
#13978=AXIS2_PLACEMENT_3D ( 'NONE', #2220, #6227, #16840 ) ;
#13981=DIRECTION ( 'NONE',  ( 0.000000000000000000, -0.01356324068817998940, 0.9999080150203990547 ) ) ;
#13982=CARTESIAN_POINT ( 'NONE',  ( -37.00000000000000711, 6.711949091238296639, -10.84030624090599559 ) ) ;
#13984=AXIS2_PLACEMENT_3D ( 'NONE', #17724, #47644, #42978 ) ;
#13987=DIRECTION ( 'NONE',  ( 1.000000000000000000, 0.000000000000000000, 0.000000000000000000 ) ) ;
#13988=CARTESIAN_POINT ( 'NONE',  ( -35.00000000000000000, 0.000000000000000000, 0.000000000000000000 ) ) ;
#13990=CIRCLE ( 'NONE', #192, 12.74999999999999822 ) ;
#13992=CIRCLE ( 'NONE', #30986, 4.999999999999999112 ) ;
#13994=DIRECTION ( 'NONE',  ( -0.000000000000000000, -0.000000000000000000, -1.000000000000000000 ) ) ;
#13995=ORIENTED_EDGE ( 'NONE', *, *, #41941, .T. ) ;
#13996=CARTESIAN_POINT ( 'NONE',  ( -25.06355223964699874, -11.89192422770156021, 6.391943611169346617 ) ) ;
#13998=CARTESIAN_POINT ( 'NONE',  ( -30.15699386792130454, -0.5151376480018481363, 13.49760124941971462 ) ) ;
#13999=CARTESIAN_POINT ( 'NONE',  ( -37.00000000000000711, 7.094637218249358668, 10.59380114696472752 ) ) ;
#14001=VERTEX_POINT ( 'NONE', #18520 ) ;
#14006=EDGE_CURVE ( 'NONE', #27622, #28103, #23149, .T. ) ;
#14010=CYLINDRICAL_SURFACE ( 'NONE', #45817, 13.50000000000000178 ) ;
#14011=CARTESIAN_POINT ( 'NONE',  ( 7.292875064767452287, -5.787367871520388007, -10.52247668536931435 ) ) ;
#14013=VECTOR ( 'NONE', #49025, 1000.000000000000000 ) ;
#14016=CARTESIAN_POINT ( 'NONE',  ( 37.00000000000000711, 9.896810808925392777, -7.110831038798317572 ) ) ;
#14017=CIRCLE ( 'NONE', #32058, 12.74999999999999822 ) ;
#14019=DIRECTION ( 'NONE',  ( -0.000000000000000000, -1.000000000000000000, -0.000000000000000000 ) ) ;
#14021=CARTESIAN_POINT ( 'NONE',  ( -27.01437459610461644, 11.79277645698183363, -2.220455681983952267 ) ) ;
#14028=EDGE_CURVE ( 'NONE', #26931, #2058, #33454, .T. ) ;
#14029=AXIS2_PLACEMENT_3D ( 'NONE', #43717, #24098, #44358 ) ;
#14030=VERTEX_POINT ( 'NONE', #45717 ) ;
#14032=CYLINDRICAL_SURFACE ( 'NONE', #64433, 13.50000000000000178 ) ;
#14034=DIRECTION ( 'NONE',  ( 0.000000000000000000, -0.9796553971857721033, -0.2006870767258996657 ) ) ;
#14036=LINE ( 'NONE', #34638, #25512 ) ;
#14044=ORIENTED_EDGE ( 'NONE', *, *, #42347, .T. ) ;
#14045=CARTESIAN_POINT ( 'NONE',  ( -29.65824816215590687, -0.5562943748163905466, -11.99470473606822907 ) ) ;
#14048=EDGE_CURVE ( 'NONE', #19224, #35366, #39513, .T. ) ;
#14049=DIRECTION ( 'NONE',  ( -1.000000000000000000, 0.000000000000000000, 0.000000000000000000 ) ) ;
#14051=AXIS2_PLACEMENT_3D ( 'NONE', #19997, #24999, #50603 ) ;
#14053=DIRECTION ( 'NONE',  ( 0.000000000000000000, -0.01356324068817998940, 0.9999080150203990547 ) ) ;
#14055=CARTESIAN_POINT ( 'NONE',  ( -37.00000000000000711, 8.854740511458851770, 7.717887834988275131 ) ) ;
#14056=ORIENTED_EDGE ( 'NONE', *, *, #22214, .F. ) ;
#14058=AXIS2_PLACEMENT_3D ( 'NONE', #27611, #32584, #17328 ) ;
#14059=ORIENTED_EDGE ( 'NONE', *, *, #65582, .F. ) ;
#14062=CIRCLE ( 'NONE', #43831, 4.999999999999999112 ) ;
#14065=CYLINDRICAL_SURFACE ( 'NONE', #2004, 12.74999999999999822 ) ;
#14067=CARTESIAN_POINT ( 'NONE',  ( 32.00000000000000000, 1.230770033143089974E-14, 0.000000000000000000 ) ) ;
#14070=DIRECTION ( 'NONE',  ( 0.000000000000000000, -0.01356324068817998940, 0.9999080150203990547 ) ) ;
#14071=EDGE_CURVE ( 'NONE', #29408, #16453, #47977, .T. ) ;
#14073=VECTOR ( 'NONE', #13268, 1000.000000000000000 ) ;
#14074=ORIENTED_EDGE ( 'NONE', *, *, #59555, .F. ) ;
#14076=DIRECTION ( 'NONE',  ( 0.000000000000000000, 0.01356324068817998940, -0.9999080150203989437 ) ) ;
#14079=VECTOR ( 'NONE', #19360, 1000.000000000000000 ) ;
#14080=CIRCLE ( 'NONE', #20454, 12.18650000000000055 ) ;
#14083=AXIS2_PLACEMENT_3D ( 'NONE', #21045, #36351, #11092 ) ;
#14087=ORIENTED_EDGE ( 'NONE', *, *, #37919, .T. ) ;
#14089=DIRECTION ( 'NONE',  ( -1.000000000000000000, 0.000000000000000000, 0.000000000000000000 ) ) ;
#14090=CARTESIAN_POINT ( 'NONE',  ( -35.00000000000000000, 0.000000000000000000, 0.000000000000000000 ) ) ;
#14091=VECTOR ( 'NONE', #11152, 1000.000000000000000 ) ;
#14092=CIRCLE ( 'NONE', #11966, 12.74999999999999822 ) ;
#14093=CARTESIAN_POINT ( 'NONE',  ( -18.04458733766117362, 25.00000000000000000, 3.916728392552376370 ) ) ;
#14094=LINE ( 'NONE', #24399, #63817 ) ;
#14096=DIRECTION ( 'NONE',  ( -1.000000000000000000, 0.000000000000000000, -0.000000000000000000 ) ) ;
#14098=AXIS2_PLACEMENT_3D ( 'NONE', #64030, #53423, #48436 ) ;
#14099=CYLINDRICAL_SURFACE ( 'NONE', #18058, 5.000000000000000888 ) ;
#14100=ORIENTED_EDGE ( 'NONE', *, *, #5551, .T. ) ;
#14101=DIRECTION ( 'NONE',  ( -0.8405098440481674205, 0.000000000000000000, -0.5417962735734949131 ) ) ;
#14102=DIRECTION ( 'NONE',  ( 0.000000000000000000, -0.01356324068817998940, 0.9999080150203990547 ) ) ;
#14104=EDGE_CURVE ( 'NONE', #7512, #42983, #4461, .T. ) ;
#14105=ORIENTED_EDGE ( 'NONE', *, *, #11337, .T. ) ;
#14109=DIRECTION ( 'NONE',  ( -1.000000000000000000, 0.000000000000000000, 0.000000000000000000 ) ) ;
#14114=ORIENTED_EDGE ( 'NONE', *, *, #39350, .F. ) ;
#14118=CYLINDRICAL_SURFACE ( 'NONE', #49762, 4.999999999999999112 ) ;
#14119=ORIENTED_EDGE ( 'NONE', *, *, #47441, .T. ) ;
#14120=VECTOR ( 'NONE', #14202, 1000.000000000000000 ) ;
#14121=EDGE_LOOP ( 'NONE', ( #11397, #64964, #27280, #64348 ) ) ;
#14122=CARTESIAN_POINT ( 'NONE',  ( -24.80569231367726246, 10.34937607735212772, 8.670028611839507349 ) ) ;
#14125=AXIS2_PLACEMENT_3D ( 'NONE', #8136, #3499, #27416 ) ;
#14126=CARTESIAN_POINT ( 'NONE',  ( -26.79516877879233050, 12.45549024775193736, 5.207329862939345411 ) ) ;
#14127=AXIS2_PLACEMENT_3D ( 'NONE', #11980, #12626, #31603 ) ;
#14128=CARTESIAN_POINT ( 'NONE',  ( 24.36182730707165689, -0.005113602571830759905, 12.00528096431153280 ) ) ;
#14131=ORIENTED_EDGE ( 'NONE', *, *, #35056, .T. ) ;
#14133=DIRECTION ( 'NONE',  ( 0.000000000000000000, -0.8989688749565111214, -0.4380125133594070519 ) ) ;
#14134=ORIENTED_EDGE ( 'NONE', *, *, #54277, .F. ) ;
#14135=AXIS2_PLACEMENT_3D ( 'NONE', #63169, #22266, #7989 ) ;
#14136=CARTESIAN_POINT ( 'NONE',  ( 35.00000000000000000, -7.474872387601069867, -9.060822531526026680 ) ) ;
#14138=DIRECTION ( 'NONE',  ( 1.000000000000000000, 0.000000000000000000, 0.000000000000000000 ) ) ;
#14140=EDGE_CURVE ( 'NONE', #22570, #5722, #64944, .T. ) ;
#14141=CIRCLE ( 'NONE', #42811, 12.18650000000000055 ) ;
#14145=CIRCLE ( 'NONE', #55607, 5.000000000000000888 ) ;
#14148=DIRECTION ( 'NONE',  ( -1.000000000000000000, -0.000000000000000000, 0.000000000000000000 ) ) ;
#14149=CARTESIAN_POINT ( 'NONE',  ( 35.00000000000000000, 11.65150730582934635, 1.488153103997001514 ) ) ;
#14150=CYLINDRICAL_SURFACE ( 'NONE', #21318, 12.18650000000000055 ) ;
#14151=ORIENTED_EDGE ( 'NONE', *, *, #15337, .F. ) ;
#14152=CIRCLE ( 'NONE', #18423, 4.999999999999999112 ) ;
#14154=EDGE_CURVE ( 'NONE', #32398, #28276, #828, .T. ) ;
#14155=( BOUNDED_CURVE ( )  B_SPLINE_CURVE ( 3, ( #621, #14885, #35821, #55819 ),
 .UNSPECIFIED., .F., .F. ) 
 B_SPLINE_CURVE_WITH_KNOTS ( ( 4, 4 ),
 ( 2.725141476405820384, 2.750767380661962136 ),
 .UNSPECIFIED. ) 
 CURVE ( )  GEOMETRIC_REPRESENTATION_ITEM ( )  RATIONAL_B_SPLINE_CURVE ( ( 1.000000000000000000, 0.9999452768345937770, 0.9999452768345937770, 1.000000000000000000 ) ) 
 REPRESENTATION_ITEM ( '' )  );
#14156=CARTESIAN_POINT ( 'NONE',  ( -5.394281107717450396, -1.427634444718381079, -11.91478059761895558 ) ) ;
#14157=CARTESIAN_POINT ( 'NONE',  ( 145.1370849898475797, 3.309064568108273190E-14, 0.000000000000000000 ) ) ;
#14159=ADVANCED_FACE ( 'NONE', ( #46702 ), #27394, .T. ) ;
#14160=CARTESIAN_POINT ( 'NONE',  ( -2.532614230583022152, -11.30437021680553222, 4.026315189028233377 ) ) ;
#14161=ORIENTED_EDGE ( 'NONE', *, *, #34060, .F. ) ;
#14162=AXIS2_PLACEMENT_3D ( 'NONE', #52704, #7802, #12431 ) ;
#14163=CARTESIAN_POINT ( 'NONE',  ( -21.04906020170784942, 11.41231286973902925, -3.710994071045396137 ) ) ;
#14165=CIRCLE ( 'NONE', #28008, 5.000000000000000888 ) ;
#14166=DIRECTION ( 'NONE',  ( 0.000000000000000000, 0.01356324068817992522, -0.9999080150203990547 ) ) ;
#14171=ORIENTED_EDGE ( 'NONE', *, *, #65639, .F. ) ;
#14174=VECTOR ( 'NONE', #36141, 1000.000000000000000 ) ;
#14176=EDGE_LOOP ( 'NONE', ( #38171, #53730, #61482, #31810 ) ) ;
#14178=CARTESIAN_POINT ( 'NONE',  ( -28.21837939661944006, -12.11352702982830642, -5.967125770076286528 ) ) ;
#14180=ADVANCED_FACE ( 'NONE', ( #21784 ), #32690, .T. ) ;
#14181=AXIS2_PLACEMENT_3D ( 'NONE', #20481, #36070, #40762 ) ;
#14182=CYLINDRICAL_SURFACE ( 'NONE', #59390, 12.75000000000000178 ) ;
#14183=FACE_OUTER_BOUND ( 'NONE', #32408, .T. ) ;
#14184=AXIS2_PLACEMENT_3D ( 'NONE', #5813, #6126, #62281 ) ;
#14186=ORIENTED_EDGE ( 'NONE', *, *, #29761, .T. ) ;
#14188=CARTESIAN_POINT ( 'NONE',  ( -8.018618887729799027, 9.418346547213671371, -9.692888119526816837 ) ) ;
#14189=CARTESIAN_POINT ( 'NONE',  ( 37.00000000000000711, 4.705694406421931860E-17, -3.469127814946512892E-15 ) ) ;
#14190=VECTOR ( 'NONE', #4073, 1000.000000000000000 ) ;
#14193=CARTESIAN_POINT ( 'NONE',  ( 35.00000000000000000, 4.705694406421931860E-17, -3.469127814946512892E-15 ) ) ;
#14197=VERTEX_POINT ( 'NONE', #61659 ) ;
#14198=ORIENTED_EDGE ( 'NONE', *, *, #18298, .F. ) ;
#14199=CARTESIAN_POINT ( 'NONE',  ( -17.65540486153495792, -7.075472138365880070, -9.696984679443399813 ) ) ;
#14200=VERTEX_POINT ( 'NONE', #16115 ) ;
#14202=DIRECTION ( 'NONE',  ( -1.000000000000000000, -0.000000000000000000, 0.000000000000000000 ) ) ;
#14203=CIRCLE ( 'NONE', #14901, 12.75000000000000178 ) ;
#14205=ORIENTED_EDGE ( 'NONE', *, *, #39194, .F. ) ;
#14212=CIRCLE ( 'NONE', #51417, 12.18650000000000055 ) ;
#14215=AXIS2_PLACEMENT_3D ( 'NONE', #53822, #24521, #28863 ) ;
#14216=ORIENTED_EDGE ( 'NONE', *, *, #45552, .F. ) ;
#14217=CARTESIAN_POINT ( 'NONE',  ( 35.00000000000000000, -11.24036214326524608, -6.018036132182126963 ) ) ;
#14218=ORIENTED_EDGE ( 'NONE', *, *, #28541, .T. ) ;
#14221=AXIS2_PLACEMENT_3D ( 'NONE', #1193, #41744, #13125 ) ;
#14224=LINE ( 'NONE', #29835, #16805 ) ;
#14225=LINE ( 'NONE', #9230, #7864 ) ;
#14228=CARTESIAN_POINT ( 'NONE',  ( 35.00000000000000000, -11.59095880812006385, 1.903127969211307224 ) ) ;
#14230=CYLINDRICAL_SURFACE ( 'NONE', #51921, 4.999999999999999112 ) ;
#14232=CIRCLE ( 'NONE', #22758, 4.999999999999999112 ) ;
#14235=LINE ( 'NONE', #19574, #27032 ) ;
#14243=ORIENTED_EDGE ( 'NONE', *, *, #43041, .F. ) ;
#14245=DIRECTION ( 'NONE',  ( 0.000000000000000000, -0.01356324068817991828, 0.9999080150203990547 ) ) ;
#14249=CARTESIAN_POINT ( 'NONE',  ( -37.00000000000000711, 0.000000000000000000, 0.000000000000000000 ) ) ;
#14253=CARTESIAN_POINT ( 'NONE',  ( -27.16408673750833103, 8.649729821182791767, -8.318274995791208326 ) ) ;
#14254=LINE ( 'NONE', #10241, #243 ) ;
#14255=DIRECTION ( 'NONE',  ( -1.000000000000000000, -0.000000000000000000, 0.000000000000000000 ) ) ;
#14258=LINE ( 'NONE', #34841, #22335 ) ;
#14259=ORIENTED_EDGE ( 'NONE', *, *, #13172, .T. ) ;
#14260=EDGE_CURVE ( 'NONE', #5091, #10987, #42677, .T. ) ;
#14262=ORIENTED_EDGE ( 'NONE', *, *, #50149, .T. ) ;
#14264=CARTESIAN_POINT ( 'NONE',  ( -36.00000000000000711, -6.018036132182241538, 11.24036214326518390 ) ) ;
#14266=AXIS2_PLACEMENT_3D ( 'NONE', #4214, #45417, #25148 ) ;
#14267=DIRECTION ( 'NONE',  ( 1.000000000000000000, -0.000000000000000000, 0.000000000000000000 ) ) ;
#14268=DIRECTION ( 'NONE',  ( 0.000000000000000000, -0.9970832820307030664, -0.07632122047557567124 ) ) ;
#14269=EDGE_LOOP ( 'NONE', ( #17456, #21591, #45881, #686 ) ) ;
#14270=ORIENTED_EDGE ( 'NONE', *, *, #15999, .F. ) ;
#14272=EDGE_CURVE ( 'NONE', #59596, #25928, #14017, .T. ) ;
#14273=CARTESIAN_POINT ( 'NONE',  ( 35.00000000000000000, 4.705694406421931860E-17, -3.469127814946512892E-15 ) ) ;
#14275=CYLINDRICAL_SURFACE ( 'NONE', #51172, 6.094511299047803199 ) ;
#14283=DIRECTION ( 'NONE',  ( 1.000000000000000000, 0.000000000000000000, 0.000000000000000000 ) ) ;
#14284=CIRCLE ( 'NONE', #22800, 12.18650000000000233 ) ;
#14286=VERTEX_POINT ( 'NONE', #29369 ) ;
#14287=CARTESIAN_POINT ( 'NONE',  ( -4.806344283790351390, -7.508992741355383416, 25.00000000000000000 ) ) ;
#14288=VERTEX_POINT ( 'NONE', #11303 ) ;
#14289=LINE ( 'NONE', #39891, #34382 ) ;
#14292=VERTEX_POINT ( 'NONE', #10977 ) ;
#14293=ORIENTED_EDGE ( 'NONE', *, *, #25264, .F. ) ;
#14294=DIRECTION ( 'NONE',  ( 0.000000000000000000, -0.01356324068817998940, 0.9999080150203990547 ) ) ;
#14296=CARTESIAN_POINT ( 'NONE',  ( -37.00000000000000711, 0.000000000000000000, 0.000000000000000000 ) ) ;
#14297=ORIENTED_EDGE ( 'NONE', *, *, #33691, .F. ) ;
#14299=ORIENTED_EDGE ( 'NONE', *, *, #44678, .F. ) ;
#14301=DIRECTION ( 'NONE',  ( -1.000000000000000000, 0.000000000000000000, 0.000000000000000000 ) ) ;
#14303=VECTOR ( 'NONE', #37380, 1000.000000000000000 ) ;
#14309=ADVANCED_FACE ( 'NONE', ( #29678 ), #4104, .T. ) ;
#14310=DIRECTION ( 'NONE',  ( -0.000000000000000000, -0.000000000000000000, -1.000000000000000000 ) ) ;
#14311=CYLINDRICAL_SURFACE ( 'NONE', #27726, 5.000000000000000888 ) ;
#14312=CIRCLE ( 'NONE', #52559, 4.999999999999999112 ) ;
#14313=ORIENTED_EDGE ( 'NONE', *, *, #47247, .T. ) ;
#14315=FACE_OUTER_BOUND ( 'NONE', #47675, .T. ) ;
#14318=EDGE_CURVE ( 'NONE', #56626, #15788, #3429, .T. ) ;
#14319=EDGE_LOOP ( 'NONE', ( #36363, #58750, #19588, #6197 ) ) ;
#14321=ORIENTED_EDGE ( 'NONE', *, *, #62553, .F. ) ;
#14322=EDGE_CURVE ( 'NONE', #51071, #24932, #36893, .T. ) ;
#14323=CYLINDRICAL_SURFACE ( 'NONE', #37003, 6.511478057721953761 ) ;
#14324=DIRECTION ( 'NONE',  ( 0.000000000000000000, -0.01356324068817998940, 0.9999080150203990547 ) ) ;
#14326=CARTESIAN_POINT ( 'NONE',  ( -3.311295734053511630, 10.53467347881536398, 5.749784130745220878 ) ) ;
#14327=EDGE_CURVE ( 'NONE', #49219, #34799, #41601, .T. ) ;
#14328=CARTESIAN_POINT ( 'NONE',  ( 13.37455928674113714, 10.48515777575467744, -5.840559289581060298 ) ) ;
#14331=DIRECTION ( 'NONE',  ( 1.000000000000000000, -0.000000000000000000, 0.000000000000000000 ) ) ;
#14333=VECTOR ( 'NONE', #56998, 1000.000000000000000 ) ;
#14335=EDGE_CURVE ( 'NONE', #29968, #48838, #60736, .T. ) ;
#14337=EDGE_CURVE ( 'NONE', #12300, #50867, #229, .T. ) ;
#14338=DIRECTION ( 'NONE',  ( 0.000000000000000000, -0.01356324068817992175, 0.9999080150203990547 ) ) ;
#14339=DIRECTION ( 'NONE',  ( 0.000000000000000000, -0.2355298848897586506, -0.9718671068226442111 ) ) ;
#14343=ORIENTED_EDGE ( 'NONE', *, *, #45442, .F. ) ;
#14344=DIRECTION ( 'NONE',  ( 1.000000000000000000, 0.000000000000000000, 0.000000000000000000 ) ) ;
#14345=ADVANCED_FACE ( 'NONE', ( #31261 ), #6014, .T. ) ;
#14347=ORIENTED_EDGE ( 'NONE', *, *, #10300, .T. ) ;
#14350=CYLINDRICAL_SURFACE ( 'NONE', #16229, 4.094603870727468120 ) ;
#14358=DIRECTION ( 'NONE',  ( -1.000000000000000000, -0.000000000000000000, -0.000000000000000000 ) ) ;
#14360=DIRECTION ( 'NONE',  ( 0.000000000000000000, -0.7196168960969868689, -0.6943713148249562872 ) ) ;
#14363=DIRECTION ( 'NONE',  ( -1.000000000000000000, 0.000000000000000000, -0.000000000000000000 ) ) ;
#14364=EDGE_LOOP ( 'NONE', ( #792, #23636, #44107, #62001 ) ) ;
#14365=CIRCLE ( 'NONE', #35588, 12.18649999999999878 ) ;
#14366=LINE ( 'NONE', #49635, #29874 ) ;
#14369=DIRECTION ( 'NONE',  ( 0.000000000000000000, 0.01356324068817998940, -0.9999080150203990547 ) ) ;
#14370=ORIENTED_EDGE ( 'NONE', *, *, #47928, .T. ) ;
#14372=ORIENTED_EDGE ( 'NONE', *, *, #26109, .F. ) ;
#14377=VECTOR ( 'NONE', #63844, 1000.000000000000000 ) ;
#14378=FACE_OUTER_BOUND ( 'NONE', #45594, .T. ) ;
#14379=DIRECTION ( 'NONE',  ( 0.000000000000000000, -0.9847383929261599445, 0.1740410799127720953 ) ) ;
#14380=ADVANCED_FACE ( 'NONE', ( #41544 ), #64928, .T. ) ;
#14381=CARTESIAN_POINT ( 'NONE',  ( -37.00000000000000711, 0.000000000000000000, 0.000000000000000000 ) ) ;
#14386=ORIENTED_EDGE ( 'NONE', *, *, #4648, .F. ) ;
#14387=CARTESIAN_POINT ( 'NONE',  ( 13.21690730856285434, -12.92645890715633250, -3.899147611715625850 ) ) ;
#14388=ORIENTED_EDGE ( 'NONE', *, *, #34731, .T. ) ;
#14389=ORIENTED_EDGE ( 'NONE', *, *, #22013, .T. ) ;
#14393=FACE_OUTER_BOUND ( 'NONE', #55912, .T. ) ;
#14394=DIRECTION ( 'NONE',  ( 0.000000000000000000, 0.01356324068817998940, -0.9999080150203990547 ) ) ;
#14400=CARTESIAN_POINT ( 'NONE',  ( -37.00000000000000711, 3.645068577060182946, -11.16627499335651130 ) ) ;
#14403=ORIENTED_EDGE ( 'NONE', *, *, #33201, .T. ) ;
#14404=AXIS2_PLACEMENT_3D ( 'NONE', #21461, #16785, #2155 ) ;
#14406=CARTESIAN_POINT ( 'NONE',  ( -10.90165637463000614, -7.508992741355389633, -11.21895841913464764 ) ) ;
#14407=CARTESIAN_POINT ( 'NONE',  ( -37.00000000000000711, 0.000000000000000000, 0.000000000000000000 ) ) ;
#14408=EDGE_LOOP ( 'NONE', ( #30431, #23452, #63766, #33907 ) ) ;
#14413=EDGE_CURVE ( 'NONE', #38595, #6117, #43182, .T. ) ;
#14416=DIRECTION ( 'NONE',  ( 0.000000000000000000, 0.01356324068817991828, -0.9999080150203990547 ) ) ;
#14418=ORIENTED_EDGE ( 'NONE', *, *, #15174, .F. ) ;
#14419=DIRECTION ( 'NONE',  ( 0.000000000000000000, 0.01356324068817991828, -0.9999080150203990547 ) ) ;
#14422=VERTEX_POINT ( 'NONE', #28233 ) ;
#14424=CARTESIAN_POINT ( 'NONE',  ( 9.751598139935644838, 1.285911471645831528, 13.44024205703445851 ) ) ;
#14425=FACE_OUTER_BOUND ( 'NONE', #27055, .T. ) ;
#14426=ORIENTED_EDGE ( 'NONE', *, *, #61850, .F. ) ;
#14430=VERTEX_POINT ( 'NONE', #37877 ) ;
#14431=DIRECTION ( 'NONE',  ( 0.000000000000000000, -0.01356324068817998940, 0.9999080150203990547 ) ) ;
#14434=DIRECTION ( 'NONE',  ( 1.000000000000000000, 0.000000000000000000, 0.000000000000000000 ) ) ;
#14437=ORIENTED_EDGE ( 'NONE', *, *, #5187, .T. ) ;
#14438=DIRECTION ( 'NONE',  ( 0.000000000000000000, 0.8696919319575201479, 0.4935949184179230786 ) ) ;
#14441=ORIENTED_EDGE ( 'NONE', *, *, #64378, .F. ) ;
#14445=DIRECTION ( 'NONE',  ( -1.000000000000000000, 0.000000000000000000, 0.000000000000000000 ) ) ;
#14447=DIRECTION ( 'NONE',  ( 0.000000000000000000, -0.01356324068817998940, 0.9999080150203990547 ) ) ;
#14448=DIRECTION ( 'NONE',  ( 1.000000000000000000, 0.000000000000000000, 0.000000000000000000 ) ) ;
#14450=EDGE_LOOP ( 'NONE', ( #62956, #15305, #10299, #50207 ) ) ;
#14457=EDGE_CURVE ( 'NONE', #45219, #55881, #17614, .T. ) ;
#14458=CARTESIAN_POINT ( 'NONE',  ( -35.00000000000000000, 4.074242145636004508, 12.08151691381191739 ) ) ;
#14460=B_SPLINE_CURVE_WITH_KNOTS ( 'NONE', 3,
 ( #47023, #33357, #11740, #22058, #7094, #1794, #42315, #2798, #58651, #17067, #28047, #13075, #52346, #62951, #27059, #1478, #27369, #47664, #53655, #22734, #57985, #16742, #26728, #42997 ),
 .UNSPECIFIED., .F., .F.,
 ( 4, 2, 2, 2, 2, 2, 2, 2, 2, 2, 2, 4 ),
 ( 0.000000000000000000, 0.0006693376636140126916, 0.001338675327228025383, 0.002008012990842038183, 0.002677350654456050767, 0.004016025981684075499, 0.004685363645298088950, 0.005354701308912100666, 0.006024038972526111514, 0.006693376636140124097, 0.008032051963368149264, 0.01070940261782419439 ),
 .UNSPECIFIED. ) ;
#14461=CARTESIAN_POINT ( 'NONE',  ( 17.52955304423989347, 7.823381130471544154, 9.114384484749823656 ) ) ;
#14462=CARTESIAN_POINT ( 'NONE',  ( 37.00000000000000711, -1.771820996347075017, 11.61175578952787113 ) ) ;
#14464=CARTESIAN_POINT ( 'NONE',  ( 27.57023587884935978, -12.80946526384611239, 4.265168728770441398 ) ) ;
#14467=EDGE_CURVE ( 'NONE', #45445, #35395, #48076, .T. ) ;
#14470=CYLINDRICAL_SURFACE ( 'NONE', #56283, 12.18650000000000055 ) ;
#14471=DIRECTION ( 'NONE',  ( 1.000000000000000000, 0.000000000000000000, 0.000000000000000000 ) ) ;
#14472=EDGE_CURVE ( 'NONE', #11505, #18081, #34243, .T. ) ;
#14473=CARTESIAN_POINT ( 'NONE',  ( -35.00000000000000000, -4.309077947445573820, -10.92721691015460550 ) ) ;
#14475=DIRECTION ( 'NONE',  ( 0.000000000000000000, 0.01356324068818000848, -0.9999080150203990547 ) ) ;
#14480=DIRECTION ( 'NONE',  ( 1.000000000000000000, 0.000000000000000000, 0.000000000000000000 ) ) ;
#14481=CARTESIAN_POINT ( 'NONE',  ( 35.00000000000000000, -11.01837265713068525, 6.415447294506815723 ) ) ;
#14483=EDGE_CURVE ( 'NONE', #62155, #45280, #2420, .T. ) ;
#14484=AXIS2_PLACEMENT_3D ( 'NONE', #24033, #50616, #49329 ) ;
#14485=ADVANCED_FACE ( 'NONE', ( #64131 ), #43847, .T. ) ;
#14487=CARTESIAN_POINT ( 'NONE',  ( -18.04458733766117362, -12.91933584589293282, 3.916728392552376370 ) ) ;
#14488=VERTEX_POINT ( 'NONE', #8272 ) ;
#14492=ORIENTED_EDGE ( 'NONE', *, *, #27322, .F. ) ;
#14495=DIRECTION ( 'NONE',  ( 1.000000000000000000, 0.000000000000000000, 0.000000000000000000 ) ) ;
#14496=DIRECTION ( 'NONE',  ( -1.000000000000000000, -0.000000000000000000, -0.000000000000000000 ) ) ;
#14500=ORIENTED_EDGE ( 'NONE', *, *, #61374, .F. ) ;
#14501=CARTESIAN_POINT ( 'NONE',  ( 47.00000000000000711, 4.705694406421931860E-17, -3.469127814946512892E-15 ) ) ;
#14507=CARTESIAN_POINT ( 'NONE',  ( -37.00000000000000711, 0.000000000000000000, 0.000000000000000000 ) ) ;
#14509=ORIENTED_EDGE ( 'NONE', *, *, #12386, .T. ) ;
#14510=EDGE_LOOP ( 'NONE', ( #19040, #50043, #55455, #57184 ) ) ;
#14511=DIRECTION ( 'NONE',  ( -1.000000000000000000, 0.000000000000000000, 0.000000000000000000 ) ) ;
#14514=FACE_OUTER_BOUND ( 'NONE', #58902, .T. ) ;
#14515=VERTEX_POINT ( 'NONE', #34184 ) ;
#14516=CARTESIAN_POINT ( 'NONE',  ( 35.00000000000000000, -11.91791701451267826, -2.544412758415803388 ) ) ;
#14517=EDGE_CURVE ( 'NONE', #3037, #38770, #8929, .T. ) ;
#14518=CARTESIAN_POINT ( 'NONE',  ( 12.70977043081474989, 11.35156634708707379, -3.911303883136926896 ) ) ;
#14519=CIRCLE ( 'NONE', #5020, 12.74999999999999822 ) ;
#14521=ORIENTED_EDGE ( 'NONE', *, *, #60296, .T. ) ;
#14522=EDGE_LOOP ( 'NONE', ( #17230, #23640, #55225, #43418 ) ) ;
#14524=VERTEX_POINT ( 'NONE', #38864 ) ;
#14527=ORIENTED_EDGE ( 'NONE', *, *, #9491, .F. ) ;
#14528=DIRECTION ( 'NONE',  ( -1.000000000000000000, -0.000000000000000000, 0.000000000000000000 ) ) ;
#14531=EDGE_CURVE ( 'NONE', #21703, #57924, #49189, .T. ) ;
#14534=DIRECTION ( 'NONE',  ( 0.000000000000000000, 0.01356324068817998940, -0.9999080150203990547 ) ) ;
#14535=VERTEX_POINT ( 'NONE', #64438 ) ;
#14539=DIRECTION ( 'NONE',  ( 0.000000000000000000, 0.1387779952735747890, -0.9903235168508558450 ) ) ;
#14542=DIRECTION ( 'NONE',  ( 1.000000000000000000, 0.000000000000000000, 0.000000000000000000 ) ) ;
#14543=CARTESIAN_POINT ( 'NONE',  ( 23.57283587138365988, 1.992978007930514606, 13.35506794274939857 ) ) ;
#14545=CARTESIAN_POINT ( 'NONE',  ( 37.00000000000000711, -8.830544224263011444, -9.196955404009264257 ) ) ;
#14546=DIRECTION ( 'NONE',  ( 0.000000000000000000, 0.9999080150203990547, 0.01356324068817645230 ) ) ;
#14548=EDGE_CURVE ( 'NONE', #14197, #4304, #42858, .T. ) ;
#14549=ORIENTED_EDGE ( 'NONE', *, *, #25978, .T. ) ;
#14550=CARTESIAN_POINT ( 'NONE',  ( -18.58686583997218378, 5.151216734910788908, -10.83812558286602012 ) ) ;
#14551=VERTEX_POINT ( 'NONE', #3951 ) ;
#14552=CARTESIAN_POINT ( 'NONE',  ( -3.518363822661491280, -9.894611242992905176, 6.801870020365760716 ) ) ;
#14558=CARTESIAN_POINT ( 'NONE',  ( -11.34824676872795379, -8.373158424984243453, -10.59295273223004585 ) ) ;
#14562=B_SPLINE_CURVE_WITH_KNOTS ( 'NONE', 3,
 ( #5962, #56829, #46185, #17881, #7568, #11891, #12881, #27855, #48161, #62427 ),
 .UNSPECIFIED., .F., .F.,
 ( 4, 2, 2, 2, 4 ),
 ( 0.002391677032556851785, 0.003742148321009147044, 0.005092619609461442737, 0.006443090897913736695, 0.007793562186366032388 ),
 .UNSPECIFIED. ) ;
#14564=CARTESIAN_POINT ( 'NONE',  ( 37.00000000000000711, -4.545979934229326780, 11.30684963584393543 ) ) ;
#14565=ORIENTED_EDGE ( 'NONE', *, *, #55887, .T. ) ;
#14569=DIRECTION ( 'NONE',  ( 0.000000000000000000, 0.8515178078024849828, -0.5243256840888592674 ) ) ;
#14574=ORIENTED_EDGE ( 'NONE', *, *, #19970, .T. ) ;
#14575=CIRCLE ( 'NONE', #29448, 12.75000000000000178 ) ;
#14576=ORIENTED_EDGE ( 'NONE', *, *, #8657, .F. ) ;
#14578=ORIENTED_EDGE ( 'NONE', *, *, #55095, .T. ) ;
#14580=CARTESIAN_POINT ( 'NONE',  ( -37.00000000000000711, -10.80631716521663854, -4.603882218679666849 ) ) ;
#14582=CARTESIAN_POINT ( 'NONE',  ( -37.00000000000000711, 8.295159312811854591, 8.927548052240926069 ) ) ;
#14583=CARTESIAN_POINT ( 'NONE',  ( -10.90165637463000614, -7.508992741355389633, -11.21895841913464764 ) ) ;
#14584=PLANE ( 'NONE',  #31794 ) ;
#14587=ORIENTED_EDGE ( 'NONE', *, *, #18549, .F. ) ;
#14590=CARTESIAN_POINT ( 'NONE',  ( -37.00000000000000711, 5.865551165831237590, -11.32068061209289134 ) ) ;
#14591=DIRECTION ( 'NONE',  ( 1.000000000000000000, -0.000000000000000000, -0.000000000000000000 ) ) ;
#14592=VERTEX_POINT ( 'NONE', #9234 ) ;
#14593=FACE_OUTER_BOUND ( 'NONE', #26034, .T. ) ;
#14594=ORIENTED_EDGE ( 'NONE', *, *, #8449, .T. ) ;
#14595=FACE_OUTER_BOUND ( 'NONE', #28513, .T. ) ;
#14596=EDGE_CURVE ( 'NONE', #42404, #43631, #56527, .T. ) ;
#14597=CARTESIAN_POINT ( 'NONE',  ( 6.022218414405385190, -8.808464729627129230, -10.23561391756376260 ) ) ;
#14598=EDGE_CURVE ( 'NONE', #45277, #22627, #43790, .T. ) ;
#14599=DIRECTION ( 'NONE',  ( -1.000000000000000000, 0.000000000000000000, 0.000000000000000000 ) ) ;
#14602=ORIENTED_EDGE ( 'NONE', *, *, #38518, .T. ) ;
#14604=EDGE_CURVE ( 'NONE', #52645, #34279, #23630, .T. ) ;
#14607=VERTEX_POINT ( 'NONE', #34816 ) ;
#14608=ORIENTED_EDGE ( 'NONE', *, *, #53276, .F. ) ;
#14609=VERTEX_POINT ( 'NONE', #55123 ) ;
#14613=EDGE_CURVE ( 'NONE', #797, #58290, #56566, .T. ) ;
#14614=DIRECTION ( 'NONE',  ( -1.000000000000000000, -0.000000000000000000, 0.000000000000000000 ) ) ;
#14615=ORIENTED_EDGE ( 'NONE', *, *, #2001, .T. ) ;
#14617=AXIS2_PLACEMENT_3D ( 'NONE', #16072, #31682, #47650 ) ;
#14619=CARTESIAN_POINT ( 'NONE',  ( -35.00000000000000000, 0.000000000000000000, 0.000000000000000000 ) ) ;
#14620=CARTESIAN_POINT ( 'NONE',  ( -18.01437271360181924, -9.050680068142952450, -10.02063192642447298 ) ) ;
#14621=ADVANCED_FACE ( 'NONE', ( #10885 ), #909, .T. ) ;
#14622=ORIENTED_EDGE ( 'NONE', *, *, #61613, .T. ) ;
#14623=CARTESIAN_POINT ( 'NONE',  ( -27.40895923133352596, 11.32254584181078449, -7.372712543863383594 ) ) ;
#14624=DIRECTION ( 'NONE',  ( 0.000000000000000000, -0.01356324068817998940, 0.9999080150203990547 ) ) ;
#14625=DIRECTION ( 'NONE',  ( 0.000000000000000000, -0.01356324068817998940, 0.9999080150203990547 ) ) ;
#14627=VERTEX_POINT ( 'NONE', #5250 ) ;
#14628=CARTESIAN_POINT ( 'NONE',  ( -18.58686583997218378, 5.151216734910788908, 25.00000000000000000 ) ) ;
#14629=EDGE_CURVE ( 'NONE', #40447, #24291, #54438, .T. ) ;
#14631=CARTESIAN_POINT ( 'NONE',  ( -24.80504806300548637, -8.637991458312614057, 10.38113301303026326 ) ) ;
#14633=DIRECTION ( 'NONE',  ( 0.000000000000000000, -0.01356324068817998940, 0.9999080150203990547 ) ) ;
#14635=DIRECTION ( 'NONE',  ( 0.000000000000000000, 0.1387779952735818667, -0.9903235168508549569 ) ) ;
#14637=CARTESIAN_POINT ( 'NONE',  ( 35.00000000000000000, 11.53507381115583108, 2.216820770815121744 ) ) ;
#14640=DIRECTION ( 'NONE',  ( 1.000000000000000000, 0.000000000000000000, 0.000000000000000000 ) ) ;
#14645=CYLINDRICAL_SURFACE ( 'NONE', #18762, 12.18650000000000055 ) ;
#14646=DIRECTION ( 'NONE',  ( -1.000000000000000000, 0.000000000000000000, 0.000000000000000000 ) ) ;
#14647=AXIS2_PLACEMENT_3D ( 'NONE', #6315, #37547, #26578 ) ;
#14648=ADVANCED_FACE ( 'NONE', ( #20541 ), #15534, .F. ) ;
#14649=ORIENTED_EDGE ( 'NONE', *, *, #35354, .F. ) ;
#14650=CARTESIAN_POINT ( 'NONE',  ( -30.09644976052020482, -2.995659101710075767, 11.64721265447471943 ) ) ;
#14651=AXIS2_PLACEMENT_3D ( 'NONE', #374, #41566, #55573 ) ;
#14652=CIRCLE ( 'NONE', #59314, 12.18649999999999878 ) ;
#14653=VERTEX_POINT ( 'NONE', #4928 ) ;
#14654=FACE_OUTER_BOUND ( 'NONE', #6370, .T. ) ;
#14655=DIRECTION ( 'NONE',  ( 1.000000000000000000, 0.000000000000000000, 0.000000000000000000 ) ) ;
#14656=LINE ( 'NONE', #8074, #10912 ) ;
#14657=VECTOR ( 'NONE', #51708, 1000.000000000000000 ) ;
#14658=DIRECTION ( 'NONE',  ( 0.000000000000000000, -0.4380125133594037767, 0.8989688749565126757 ) ) ;
#14659=ORIENTED_EDGE ( 'NONE', *, *, #20332, .F. ) ;
#14660=EDGE_LOOP ( 'NONE', ( #3616, #56767, #52327, #58323 ) ) ;
#14661=AXIS2_PLACEMENT_3D ( 'NONE', #59159, #53840, #29216 ) ;
#14662=ORIENTED_EDGE ( 'NONE', *, *, #2718, .F. ) ;
#14665=ADVANCED_FACE ( 'NONE', ( #65731 ), #56797, .T. ) ;
#14667=DIRECTION ( 'NONE',  ( 1.000000000000000000, 0.000000000000000000, 0.000000000000000000 ) ) ;
#14668=FACE_OUTER_BOUND ( 'NONE', #37161, .T. ) ;
#14669=CARTESIAN_POINT ( 'NONE',  ( -19.02967556479643463, -13.50000000000023803, -2.066764320408402454E-13 ) ) ;
#14670=ORIENTED_EDGE ( 'NONE', *, *, #16909, .F. ) ;
#14672=EDGE_CURVE ( 'NONE', #25281, #43014, #32094, .T. ) ;
#14674=DIRECTION ( 'NONE',  ( 0.000000000000000000, 0.01356324068817992175, -0.9999080150203990547 ) ) ;
#14675=CARTESIAN_POINT ( 'NONE',  ( 12.10998784662220729, -8.443435280036764468, -8.526922110106905706 ) ) ;
#14677=CARTESIAN_POINT ( 'NONE',  ( -35.00000000000000000, 12.49688848680887965, -2.527899948230500460 ) ) ;
#14678=EDGE_CURVE ( 'NONE', #18084, #52024, #8837, .T. ) ;
#14681=ORIENTED_EDGE ( 'NONE', *, *, #54073, .T. ) ;
#14682=DIRECTION ( 'NONE',  ( -1.000000000000000000, 0.000000000000000000, 0.000000000000000000 ) ) ;
#14684=DIRECTION ( 'NONE',  ( -1.000000000000000000, 0.000000000000000000, -0.000000000000000000 ) ) ;
#14688=DIRECTION ( 'NONE',  ( 0.000000000000000000, 0.9999080150203989437, 0.01356324068817649567 ) ) ;
#14689=EDGE_CURVE ( 'NONE', #17729, #8204, #50165, .T. ) ;
#14692=CARTESIAN_POINT ( 'NONE',  ( -35.00000000000000000, -3.287724142101498437, 11.73463472867575064 ) ) ;
#14693=ORIENTED_EDGE ( 'NONE', *, *, #52853, .F. ) ;
#14694=VERTEX_POINT ( 'NONE', #20859 ) ;
#14695=CARTESIAN_POINT ( 'NONE',  ( 13.33811086919980582, -12.02507490806326906, -6.151199329268367322 ) ) ;
#14696=ORIENTED_EDGE ( 'NONE', *, *, #20519, .F. ) ;
#14697=EDGE_CURVE ( 'NONE', #16833, #1585, #15849, .T. ) ;
#14700=CARTESIAN_POINT ( 'NONE',  ( 37.00000000000000711, 4.705694406421931860E-17, -3.469127814946512892E-15 ) ) ;
#14701=CARTESIAN_POINT ( 'NONE',  ( 22.88594695219327235, -4.822122601967141264, 10.98850006195556261 ) ) ;
#14703=CARTESIAN_POINT ( 'NONE',  ( 35.00000000000000000, 4.705694406421931860E-17, -3.469127814946512892E-15 ) ) ;
#14704=VECTOR ( 'NONE', #42418, 1000.000000000000000 ) ;
#14707=EDGE_CURVE ( 'NONE', #64752, #52828, #22847, .T. ) ;
#14708=CIRCLE ( 'NONE', #27488, 5.000000000000000000 ) ;
#14709=AXIS2_PLACEMENT_3D ( 'NONE', #45050, #55689, #45367 ) ;
#14710=ORIENTED_EDGE ( 'NONE', *, *, #46809, .T. ) ;
#14712=ADVANCED_FACE ( 'NONE', ( #21531 ), #12191, .T. ) ;
#14715=CARTESIAN_POINT ( 'NONE',  ( -19.47984447937493613, -3.750539801530005768, 12.96855624952674724 ) ) ;
#14716=ORIENTED_EDGE ( 'NONE', *, *, #25004, .F. ) ;
#14717=CIRCLE ( 'NONE', #14661, 4.999999999999999112 ) ;
#14718=( BOUNDED_CURVE ( )  B_SPLINE_CURVE ( 3, ( #48917, #23638, #43913, #43565 ),
 .UNSPECIFIED., .F., .F. ) 
 B_SPLINE_CURVE_WITH_KNOTS ( ( 4, 4 ),
 ( 3.768125045480501978, 3.806565460767492581 ),
 .UNSPECIFIED. ) 
 CURVE ( )  GEOMETRIC_REPRESENTATION_ITEM ( )  RATIONAL_B_SPLINE_CURVE ( ( 1.000000000000000000, 0.9998768649967908484, 0.9998768649967908484, 1.000000000000000000 ) ) 
 REPRESENTATION_ITEM ( '' )  );
#14720=DIRECTION ( 'NONE',  ( 0.000000000000000000, -0.2960891610144378849, -0.9551603052523519599 ) ) ;
#14725=DIRECTION ( 'NONE',  ( 0.000000000000000000, 0.01356324068817998940, -0.9999080150203989437 ) ) ;
#14726=ADVANCED_FACE ( 'NONE', ( #52114 ), #22168, .T. ) ;
#14727=EDGE_CURVE ( 'NONE', #58914, #325, #16162, .T. ) ;
#14729=CARTESIAN_POINT ( 'NONE',  ( -37.00000000000000711, 11.65554240571059275, -1.456211999474221086 ) ) ;
#14730=DIRECTION ( 'NONE',  ( 0.000000000000000000, -0.01356324068817998940, 0.9999080150203990547 ) ) ;
#14731=ORIENTED_EDGE ( 'NONE', *, *, #64087, .F. ) ;
#14732=VECTOR ( 'NONE', #56346, 1000.000000000000000 ) ;
#14733=CARTESIAN_POINT ( 'NONE',  ( -37.00000000000000711, 2.143131898507868297E-16, 1.750000000000000000 ) ) ;
#14734=CARTESIAN_POINT ( 'NONE',  ( -9.387807931906369419, -8.620866317596876272, -8.357905562734071481 ) ) ;
#14737=CARTESIAN_POINT ( 'NONE',  ( -35.00000000000000000, -1.039216533672986387, 11.70009620280411333 ) ) ;
#14738=CYLINDRICAL_SURFACE ( 'NONE', #28797, 12.18649999999999878 ) ;
#14740=EDGE_CURVE ( 'NONE', #41139, #56080, #16850, .T. ) ;
#14743=AXIS2_PLACEMENT_3D ( 'NONE', #11765, #36400, #57339 ) ;
#14744=CIRCLE ( 'NONE', #51957, 12.75000000000000178 ) ;
#14745=EDGE_CURVE ( 'NONE', #53954, #64447, #15114, .T. ) ;
#14746=ORIENTED_EDGE ( 'NONE', *, *, #56534, .T. ) ;
#14747=CARTESIAN_POINT ( 'NONE',  ( -35.00000000000000000, 12.18632975068353019, 0.06441628369840693424 ) ) ;
#14750=DIRECTION ( 'NONE',  ( 0.000000000000000000, -0.01356324068817998940, 0.9999080150203990547 ) ) ;
#14753=CARTESIAN_POINT ( 'NONE',  ( 24.89813668873049934, -0.9220755465451354604, -13.46995378289207856 ) ) ;
#14756=CYLINDRICAL_SURFACE ( 'NONE', #30954, 12.74999999999999822 ) ;
#14757=ADVANCED_FACE ( 'NONE', ( #42424 ), #37125, .T. ) ;
#14758=VERTEX_POINT ( 'NONE', #62392 ) ;
#14759=VERTEX_POINT ( 'NONE', #57426 ) ;
#14765=DIRECTION ( 'NONE',  ( 1.000000000000000000, 0.000000000000000000, 0.000000000000000000 ) ) ;
#14766=DIRECTION ( 'NONE',  ( 1.000000000000000000, -0.000000000000000000, -0.000000000000000000 ) ) ;
#14767=ORIENTED_EDGE ( 'NONE', *, *, #32039, .F. ) ;
#14768=ORIENTED_EDGE ( 'NONE', *, *, #2894, .F. ) ;
#14769=CYLINDRICAL_SURFACE ( 'NONE', #60299, 12.74999999999999822 ) ;
#14771=EDGE_CURVE ( 'NONE', #28779, #11257, #16542, .T. ) ;
#14772=EDGE_CURVE ( 'NONE', #27274, #44068, #47136, .T. ) ;
#14773=ORIENTED_EDGE ( 'NONE', *, *, #10742, .T. ) ;
#14776=CARTESIAN_POINT ( 'NONE',  ( 18.20196009002823345, 5.188642410960312645, 10.83342377252405164 ) ) ;
#14780=CIRCLE ( 'NONE', #2079, 12.74999999999999822 ) ;
#14781=ADVANCED_FACE ( 'NONE', ( #5817 ), #47019, .T. ) ;
#14782=FACE_OUTER_BOUND ( 'NONE', #48600, .T. ) ;
#14784=CIRCLE ( 'NONE', #27522, 5.000000000000001776 ) ;
#14785=VERTEX_POINT ( 'NONE', #31690 ) ;
#14786=EDGE_CURVE ( 'NONE', #35230, #10928, #44878, .T. ) ;
#14790=AXIS2_PLACEMENT_3D ( 'NONE', #36085, #51436, #41406 ) ;
#14792=DIRECTION ( 'NONE',  ( 1.000000000000000000, 0.000000000000000000, 0.000000000000000000 ) ) ;
#14793=AXIS2_PLACEMENT_3D ( 'NONE', #30692, #40024, #24750 ) ;
#14794=CARTESIAN_POINT ( 'NONE',  ( -7.761246313398307173, -2.161858718264055401, -11.80499000202248894 ) ) ;
#14796=CARTESIAN_POINT ( 'NONE',  ( -37.00000000000000711, 0.000000000000000000, 0.000000000000000000 ) ) ;
#14797=VERTEX_POINT ( 'NONE', #30397 ) ;
#14799=CARTESIAN_POINT ( 'NONE',  ( 37.00000000000000711, 12.16632754454236398, -0.7008968033239244555 ) ) ;
#14800=FACE_OUTER_BOUND ( 'NONE', #10802, .T. ) ;
#14801=AXIS2_PLACEMENT_3D ( 'NONE', #35219, #4991, #55522 ) ;
#14805=DIRECTION ( 'NONE',  ( -1.000000000000000000, 0.000000000000000000, -0.000000000000000000 ) ) ;
#14806=ORIENTED_EDGE ( 'NONE', *, *, #22409, .T. ) ;
#14807=LINE ( 'NONE', #19515, #55644 ) ;
#14810=EDGE_LOOP ( 'NONE', ( #42926, #11438, #5955, #34561 ) ) ;
#14812=DIRECTION ( 'NONE',  ( 0.000000000000000000, 0.01356324068817998940, -0.9999080150203990547 ) ) ;
#14816=ORIENTED_EDGE ( 'NONE', *, *, #23504, .F. ) ;
#14819=VECTOR ( 'NONE', #26503, 1000.000000000000000 ) ;
#14820=DIRECTION ( 'NONE',  ( 0.000000000000000000, 0.01356324068817998940, -0.9999080150203990547 ) ) ;
#14822=DIRECTION ( 'NONE',  ( 0.000000000000000000, -0.9246979985058680906, -0.3807014730195321661 ) ) ;
#14823=CARTESIAN_POINT ( 'NONE',  ( -35.00000000000000000, -12.31350058095525668, 3.307597835713200762 ) ) ;
#14825=CARTESIAN_POINT ( 'NONE',  ( -35.00000000000000000, -10.91072401419407001, -5.428340790341820821 ) ) ;
#14828=CARTESIAN_POINT ( 'NONE',  ( 35.00000000000000000, 0.3025107581131208367, -11.74226168163341555 ) ) ;
#14829=DIRECTION ( 'NONE',  ( 1.000000000000000000, -0.000000000000000000, 0.000000000000000000 ) ) ;
#14831=ORIENTED_EDGE ( 'NONE', *, *, #17708, .F. ) ;
#14832=DIRECTION ( 'NONE',  ( 1.000000000000000000, -0.000000000000000000, 0.000000000000000000 ) ) ;
#14833=ORIENTED_EDGE ( 'NONE', *, *, #9479, .F. ) ;
#14834=EDGE_CURVE ( 'NONE', #29699, #25796, #61871, .T. ) ;
#14838=AXIS2_PLACEMENT_3D ( 'NONE', #43805, #19842, #14820 ) ;
#14839=ORIENTED_EDGE ( 'NONE', *, *, #56669, .F. ) ;
#14840=CARTESIAN_POINT ( 'NONE',  ( -32.16141091265169649, 25.00000000000000000, 5.384978440493686236 ) ) ;
#14841=DIRECTION ( 'NONE',  ( 1.000000000000000000, 0.000000000000000000, 0.000000000000000000 ) ) ;
#14842=CYLINDRICAL_SURFACE ( 'NONE', #10643, 4.999999999999999112 ) ;
#14844=ORIENTED_EDGE ( 'NONE', *, *, #26557, .F. ) ;
#14845=CARTESIAN_POINT ( 'NONE',  ( -2.532614230583022152, 25.00000000000000000, 4.026315189028233377 ) ) ;
#14849=ORIENTED_EDGE ( 'NONE', *, *, #38568, .T. ) ;
#14854=CARTESIAN_POINT ( 'NONE',  ( 26.08439714455133185, 25.00000000000000000, 3.743551691817327942 ) ) ;
#14859=EDGE_CURVE ( 'NONE', #2844, #28276, #41704, .T. ) ;
#14860=DIRECTION ( 'NONE',  ( -1.000000000000000000, 0.000000000000000000, 0.000000000000000000 ) ) ;
#14861=DIRECTION ( 'NONE',  ( -1.000000000000000000, 0.000000000000000000, 0.000000000000000000 ) ) ;
#14862=CARTESIAN_POINT ( 'NONE',  ( 35.00000000000000000, 11.30684963584395675, 4.545979934229284147 ) ) ;
#14864=CARTESIAN_POINT ( 'NONE',  ( 37.00000000000000711, 11.78977382767499549, -4.245927698352105928 ) ) ;
#14865=CARTESIAN_POINT ( 'NONE',  ( -35.00000000000000000, 0.000000000000000000, 0.000000000000000000 ) ) ;
#14867=CIRCLE ( 'NONE', #55239, 5.000000000000000888 ) ;
#14868=VECTOR ( 'NONE', #15689, 1000.000000000000000 ) ;
#14869=ORIENTED_EDGE ( 'NONE', *, *, #7803, .T. ) ;
#14870=AXIS2_PLACEMENT_3D ( 'NONE', #60002, #9424, #13763 ) ;
#14872=VERTEX_POINT ( 'NONE', #15430 ) ;
#14873=DIRECTION ( 'NONE',  ( 0.000000000000000000, -0.4698238015817428059, -0.8827602140260282226 ) ) ;
#14875=DIRECTION ( 'NONE',  ( -1.000000000000000000, -0.000000000000000000, 0.000000000000000000 ) ) ;
#14878=EDGE_LOOP ( 'NONE', ( #1105, #6841, #11501, #24933 ) ) ;
#14879=DIRECTION ( 'NONE',  ( 0.000000000000000000, -0.7381862504171877726, 0.6745969609292743474 ) ) ;
#14881=DIRECTION ( 'NONE',  ( 0.000000000000000000, 0.01356324068817998940, -0.9999080150203990547 ) ) ;
#14882=PLANE ( 'NONE',  #61421 ) ;
#14885=CARTESIAN_POINT ( 'NONE',  ( 29.20115507325780868, -4.760464791327672529, 11.01582872674790892 ) ) ;
#14886=ADVANCED_FACE ( 'NONE', ( #36370 ), #11421, .F. ) ;
#14895=FACE_OUTER_BOUND ( 'NONE', #36781, .T. ) ;
#14897=VERTEX_POINT ( 'NONE', #490 ) ;
#14898=VERTEX_POINT ( 'NONE', #31385 ) ;
#14900=VERTEX_POINT ( 'NONE', #5479 ) ;
#14901=AXIS2_PLACEMENT_3D ( 'NONE', #18587, #59137, #54795 ) ;
#14902=CARTESIAN_POINT ( 'NONE',  ( 35.00000000000000000, 10.91072401419418014, 5.428340790341585453 ) ) ;
#14903=CARTESIAN_POINT ( 'NONE',  ( -35.00000000000000000, 1.171570255487447643, 11.68758509253248867 ) ) ;
#14907=CARTESIAN_POINT ( 'NONE',  ( -16.98800322446194855, 2.922502605998049674, 11.63868456991315625 ) ) ;
#14908=DIRECTION ( 'NONE',  ( -0.9790892447477997917, -0.2034311943119418153, 0.000000000000000000 ) ) ;
#14909=VERTEX_POINT ( 'NONE', #51687 ) ;
#14913=CARTESIAN_POINT ( 'NONE',  ( -8.891032880924177206, -11.36194426013948444, -3.860857758255646921 ) ) ;
#14914=ORIENTED_EDGE ( 'NONE', *, *, #11070, .F. ) ;
#14915=VERTEX_POINT ( 'NONE', #6446 ) ;
#14921=AXIS2_PLACEMENT_3D ( 'NONE', #26796, #47424, #2183 ) ;
#14922=ORIENTED_EDGE ( 'NONE', *, *, #46727, .F. ) ;
#14924=EDGE_LOOP ( 'NONE', ( #18348, #45193, #44553, #39138 ) ) ;
#14925=CARTESIAN_POINT ( 'NONE',  ( -2.812214508280797887, -11.36735472963161087, 3.846083643116571693 ) ) ;
#14926=( BOUNDED_CURVE ( )  B_SPLINE_CURVE ( 3, ( #25492, #59776, #45783, #24513 ),
 .UNSPECIFIED., .F., .F. ) 
 B_SPLINE_CURVE_WITH_KNOTS ( ( 4, 4 ),
 ( 2.345489028160348877, 2.374682635079008008 ),
 .UNSPECIFIED. ) 
 CURVE ( )  GEOMETRIC_REPRESENTATION_ITEM ( )  RATIONAL_B_SPLINE_CURVE ( ( 1.000000000000000000, 0.9999289790372866138, 0.9999289790372866138, 1.000000000000000000 ) ) 
 REPRESENTATION_ITEM ( '' )  );
#14928=DIRECTION ( 'NONE',  ( 1.000000000000000000, 0.000000000000000000, -0.000000000000000000 ) ) ;
#14930=EDGE_LOOP ( 'NONE', ( #26889, #8349, #62035, #48732 ) ) ;
#14932=DIRECTION ( 'NONE',  ( -1.000000000000000000, 0.000000000000000000, 0.000000000000000000 ) ) ;
#14933=ORIENTED_EDGE ( 'NONE', *, *, #2267, .T. ) ;
#14936=ORIENTED_EDGE ( 'NONE', *, *, #50923, .F. ) ;
#14937=ORIENTED_EDGE ( 'NONE', *, *, #33773, .F. ) ;
#14938=CIRCLE ( 'NONE', #57453, 12.75000000000000178 ) ;
#14939=CARTESIAN_POINT ( 'NONE',  ( -21.23983773598477498, -7.447593303288433830, 25.00000000000000000 ) ) ;
#14940=EDGE_CURVE ( 'NONE', #37122, #20190, #47039, .T. ) ;
#14942=AXIS2_PLACEMENT_3D ( 'NONE', #33401, #38718, #8790 ) ;
#14944=CARTESIAN_POINT ( 'NONE',  ( 22.61491127797214062, 25.00000000000000000, 9.376349503825034404 ) ) ;
#14947=AXIS2_PLACEMENT_3D ( 'NONE', #2759, #40745, #61035 ) ;
#14948=PLANE ( 'NONE',  #23766 ) ;
#14949=CIRCLE ( 'NONE', #52144, 12.74999999999999822 ) ;
#14951=CARTESIAN_POINT ( 'NONE',  ( 37.00000000000000711, 3.827046518385079032, -11.56998259273179386 ) ) ;
#14952=CARTESIAN_POINT ( 'NONE',  ( -37.00000000000000711, 0.000000000000000000, 0.000000000000000000 ) ) ;
#14953=AXIS2_PLACEMENT_3D ( 'NONE', #48657, #7407, #17741 ) ;
#14954=ORIENTED_EDGE ( 'NONE', *, *, #2419, .T. ) ;
#14955=DIRECTION ( 'NONE',  ( 1.000000000000000000, 0.000000000000000000, 0.000000000000000000 ) ) ;
#14958=PLANE ( 'NONE',  #17452 ) ;
#14960=ORIENTED_EDGE ( 'NONE', *, *, #20580, .T. ) ;
#14961=CARTESIAN_POINT ( 'NONE',  ( 37.00000000000000711, 8.624332853796058629, -9.390600770288022758 ) ) ;
#14964=LINE ( 'NONE', #15947, #38102 ) ;
#14968=CIRCLE ( 'NONE', #52169, 12.74999999999999822 ) ;
#14969=CARTESIAN_POINT ( 'NONE',  ( 12.95271867950812528, 9.518344588336780987, -7.319468597748340244 ) ) ;
#14970=ORIENTED_EDGE ( 'NONE', *, *, #17308, .F. ) ;
#14971=LINE ( 'NONE', #9658, #21798 ) ;
#14973=CYLINDRICAL_SURFACE ( 'NONE', #53425, 5.000000000000000888 ) ;
#14976=AXIS2_PLACEMENT_3D ( 'NONE', #46001, #40009, #457 ) ;
#14977=AXIS2_PLACEMENT_3D ( 'NONE', #15709, #31024, #6418 ) ;
#14978=ADVANCED_FACE ( 'NONE', ( #7091 ), #42004, .F. ) ;
#14983=DIRECTION ( 'NONE',  ( -1.000000000000000000, 0.000000000000000000, -0.000000000000000000 ) ) ;
#14985=VECTOR ( 'NONE', #53738, 1000.000000000000000 ) ;
#14987=EDGE_CURVE ( 'NONE', #61588, #22166, #13815, .T. ) ;
#14998=EDGE_CURVE ( 'NONE', #23816, #61226, #47221, .T. ) ;
#15001=VERTEX_POINT ( 'NONE', #52342 ) ;
#15005=( NAMED_UNIT ( * ) PLANE_ANGLE_UNIT ( ) SI_UNIT ( $, .RADIAN. ) );
#15006=CARTESIAN_POINT ( 'NONE',  ( -35.00000000000000000, -1.903127969211109383, -11.59095880812010471 ) ) ;
#15007=CIRCLE ( 'NONE', #52218, 12.18650000000000233 ) ;
#15013=DIRECTION ( 'NONE',  ( -1.000000000000000000, -0.000000000000000000, -0.000000000000000000 ) ) ;
#15014=VERTEX_POINT ( 'NONE', #32662 ) ;
#15015=AXIS2_PLACEMENT_3D ( 'NONE', #25272, #61189, #15304 ) ;
#15016=DIRECTION ( 'NONE',  ( -1.000000000000000000, -0.000000000000000000, 0.000000000000000000 ) ) ;
#15017=AXIS2_PLACEMENT_3D ( 'NONE', #11096, #47337, #46660 ) ;
#15021=ORIENTED_EDGE ( 'NONE', *, *, #20628, .F. ) ;
#15022=CARTESIAN_POINT ( 'NONE',  ( -28.41827485489077532, 3.509237424706437292, -11.47541949982828413 ) ) ;
#15025=DIRECTION ( 'NONE',  ( 1.000000000000000000, 0.000000000000000000, 0.000000000000000000 ) ) ;
#15027=DIRECTION ( 'NONE',  ( -1.000000000000000000, 0.000000000000000000, 0.000000000000000000 ) ) ;
#15028=AXIS2_PLACEMENT_3D ( 'NONE', #36170, #36523, #5964 ) ;
#15030=DIRECTION ( 'NONE',  ( 1.000000000000000000, 0.000000000000000000, 0.000000000000000000 ) ) ;
#15031=AXIS2_PLACEMENT_3D ( 'NONE', #34043, #29082, #49388 ) ;
#15035=CARTESIAN_POINT ( 'NONE',  ( 5.978762125391987148, -9.660146724424269138, 9.437723523674879544 ) ) ;
#15039=CARTESIAN_POINT ( 'NONE',  ( 13.31844906986379939, -12.79504830355194578, -4.310850366937079237 ) ) ;
#15040=ORIENTED_EDGE ( 'NONE', *, *, #33257, .T. ) ;
#15046=CIRCLE ( 'NONE', #4487, 15.00000000000000000 ) ;
#15047=ADVANCED_FACE ( 'NONE', ( #6782 ), #2106, .T. ) ;
#15048=AXIS2_PLACEMENT_3D ( 'NONE', #6600, #30854, #61779 ) ;
#15049=CARTESIAN_POINT ( 'NONE',  ( 37.00000000000000711, -11.60979404548631777, 3.704519465651427534 ) ) ;
#15051=AXIS2_PLACEMENT_3D ( 'NONE', #48781, #23846, #54430 ) ;
#15052=ORIENTED_EDGE ( 'NONE', *, *, #58682, .F. ) ;
#15055=CYLINDRICAL_SURFACE ( 'NONE', #3758, 12.74999999999999822 ) ;
#15057=ORIENTED_EDGE ( 'NONE', *, *, #27094, .T. ) ;
#15058=VECTOR ( 'NONE', #62631, 1000.000000000000000 ) ;
#15060=ADVANCED_FACE ( 'NONE', ( #33004 ), #18063, .T. ) ;
#15061=VECTOR ( 'NONE', #43411, 1000.000000000000000 ) ;
#15062=CARTESIAN_POINT ( 'NONE',  ( -29.43980975494970309, -3.641506875706030488, 11.43413432115373318 ) ) ;
#15063=ADVANCED_FACE ( 'NONE', ( #7405 ), #37998, .T. ) ;
#15064=CARTESIAN_POINT ( 'NONE',  ( -10.85292393035418002, -8.302656004634402009, -10.64777333369827694 ) ) ;
#15065=CARTESIAN_POINT ( 'NONE',  ( 29.03457606387295087, 25.00000000000000000, 10.97436308512422265 ) ) ;
#15069=DIRECTION ( 'NONE',  ( 0.000000000000000000, -0.01356324068817999114, 0.9999080150203989437 ) ) ;
#15070=DIRECTION ( 'NONE',  ( 0.000000000000000000, 0.4380125133593974485, -0.8989688749565157844 ) ) ;
#15072=AXIS2_PLACEMENT_3D ( 'NONE', #34805, #5582, #25852 ) ;
#15073=AXIS2_PLACEMENT_3D ( 'NONE', #8936, #43188, #2324 ) ;
#15074=EDGE_CURVE ( 'NONE', #34975, #48767, #17171, .T. ) ;
#15077=VERTEX_POINT ( 'NONE', #48994 ) ;
#15081=CARTESIAN_POINT ( 'NONE',  ( 35.00000000000000000, 6.917234959366825642, -9.493370459201726064 ) ) ;
#15083=LINE ( 'NONE', #49694, #28714 ) ;
#15084=CARTESIAN_POINT ( 'NONE',  ( -35.00000000000000000, 0.000000000000000000, 0.000000000000000000 ) ) ;
#15085=ORIENTED_EDGE ( 'NONE', *, *, #7755, .F. ) ;
#15087=VERTEX_POINT ( 'NONE', #19041 ) ;
#15088=CIRCLE ( 'NONE', #49064, 12.18649999999999878 ) ;
#15089=VERTEX_POINT ( 'NONE', #59282 ) ;
#15090=EDGE_CURVE ( 'NONE', #63404, #3635, #47982, .T. ) ;
#15091=DIRECTION ( 'NONE',  ( 0.000000000000000000, -0.01356324068817998940, 0.9999080150203990547 ) ) ;
#15092=CYLINDRICAL_SURFACE ( 'NONE', #15544, 6.183183579532408380 ) ;
#15095=DIRECTION ( 'NONE',  ( 0.000000000000000000, -0.8515178078024924213, 0.5243256840888473880 ) ) ;
#15098=EDGE_CURVE ( 'NONE', #36353, #29968, #54196, .T. ) ;
#15099=CARTESIAN_POINT ( 'NONE',  ( 24.19622822648017646, 1.946907465358852951, -13.36368882268028635 ) ) ;
#15100=CARTESIAN_POINT ( 'NONE',  ( 35.00000000000000000, 3.827046518385079032, -11.56998259273179386 ) ) ;
#15102=FACE_OUTER_BOUND ( 'NONE', #46734, .T. ) ;
#15103=ORIENTED_EDGE ( 'NONE', *, *, #42335, .T. ) ;
#15104=DIRECTION ( 'NONE',  ( 1.000000000000000000, 0.000000000000000000, 0.000000000000000000 ) ) ;
#15105=ORIENTED_EDGE ( 'NONE', *, *, #48826, .T. ) ;
#15106=ORIENTED_EDGE ( 'NONE', *, *, #60444, .T. ) ;
#15109=CARTESIAN_POINT ( 'NONE',  ( -27.45775109278351067, 25.00000000000000000, -1.989333891161980894 ) ) ;
#15112=LINE ( 'NONE', #45376, #60672 ) ;
#15113=ORIENTED_EDGE ( 'NONE', *, *, #22945, .F. ) ;
#15114=CIRCLE ( 'NONE', #60785, 12.18650000000000055 ) ;
#15116=LINE ( 'NONE', #168, #57137 ) ;
#15119=DIRECTION ( 'NONE',  ( -1.000000000000000000, 0.000000000000000000, -0.000000000000000000 ) ) ;
#15123=CARTESIAN_POINT ( 'NONE',  ( 18.48387936547513277, 3.702729101149824675, 11.42676336058183217 ) ) ;
#15125=AXIS2_PLACEMENT_3D ( 'NONE', #63888, #33312, #37306 ) ;
#15126=EDGE_CURVE ( 'NONE', #17960, #12171, #52224, .T. ) ;
#15129=CARTESIAN_POINT ( 'NONE',  ( -32.00000000000000000, -15.00000000000000000, 0.000000000000000000 ) ) ;
#15130=ORIENTED_EDGE ( 'NONE', *, *, #26646, .T. ) ;
#15132=ORIENTED_EDGE ( 'NONE', *, *, #39087, .F. ) ;
#15135=ADVANCED_FACE ( 'NONE', ( #38673 ), #58978, .T. ) ;
#15136=CARTESIAN_POINT ( 'NONE',  ( 37.00000000000000711, -10.43555801961471552, 5.391785509271064925 ) ) ;
#15137=DIRECTION ( 'NONE',  ( 0.000000000000000000, -0.1740410799127686259, -0.9847383929261604996 ) ) ;
#15138=EDGE_CURVE ( 'NONE', #62542, #46560, #14036, .T. ) ;
#15139=CARTESIAN_POINT ( 'NONE',  ( -35.00000000000000000, 9.240395740215735287, -7.251710744571480127 ) ) ;
#15140=CIRCLE ( 'NONE', #48058, 12.74999999999999822 ) ;
#15141=CARTESIAN_POINT ( 'NONE',  ( 24.19857423850153566, 0.7091544454727191082, -13.48603582285567271 ) ) ;
#15142=DIRECTION ( 'NONE',  ( -1.000000000000000000, -0.000000000000000000, 0.000000000000000000 ) ) ;
#15143=CIRCLE ( 'NONE', #27887, 5.000000000000000000 ) ;
#15145=EDGE_CURVE ( 'NONE', #797, #33730, #58590, .T. ) ;
#15146=ORIENTED_EDGE ( 'NONE', *, *, #4608, .T. ) ;
#15148=CARTESIAN_POINT ( 'NONE',  ( 37.00000000000000711, 10.39746860227901060, 7.379373053628750512 ) ) ;
#15149=CARTESIAN_POINT ( 'NONE',  ( -18.25006854224444908, -9.443202773001939221, 7.404452808139724063 ) ) ;
#15153=ORIENTED_EDGE ( 'NONE', *, *, #23759, .F. ) ;
#15156=EDGE_CURVE ( 'NONE', #24950, #36705, #53999, .T. ) ;
#15158=ORIENTED_EDGE ( 'NONE', *, *, #58934, .F. ) ;
#15159=CARTESIAN_POINT ( 'NONE',  ( -35.00000000000000000, 0.000000000000000000, 0.000000000000000000 ) ) ;
#15160=DIRECTION ( 'NONE',  ( -1.000000000000000000, 0.000000000000000000, 0.000000000000000000 ) ) ;
#15161=CARTESIAN_POINT ( 'NONE',  ( 17.27839441901508621, -10.52068335315807524, 5.771933972472480967 ) ) ;
#15162=EDGE_CURVE ( 'NONE', #27103, #8013, #6550, .T. ) ;
#15163=AXIS2_PLACEMENT_3D ( 'NONE', #43140, #33171, #42149 ) ;
#15164=AXIS2_PLACEMENT_3D ( 'NONE', #13861, #34156, #54469 ) ;
#15168=EDGE_CURVE ( 'NONE', #31395, #1816, #14366, .T. ) ;
#15170=VECTOR ( 'NONE', #61223, 1000.000000000000000 ) ;
#15171=CARTESIAN_POINT ( 'NONE',  ( -35.00000000000000000, -11.29812557209474733, -3.213188559034363401 ) ) ;
#15174=EDGE_CURVE ( 'NONE', #37272, #29699, #38378, .T. ) ;
#15176=CARTESIAN_POINT ( 'NONE',  ( 37.00000000000000711, 11.73808581813437080, -0.4353888892050498116 ) ) ;
#15177=CARTESIAN_POINT ( 'NONE',  ( -14.11589373245165469, 8.250315036047107142, -10.68561190601526256 ) ) ;
#15178=DIRECTION ( 'NONE',  ( 0.000000000000000000, 0.9987865678893277366, -0.04924826701374931254 ) ) ;
#15180=B_SPLINE_CURVE_WITH_KNOTS ( 'NONE', 3,
 ( #65299, #9421, #34387, #64962, #63991, #50018, #14734, #59030, #49056, #13441, #54364, #13760, #3834, #8800, #35013, #64625 ),
 .UNSPECIFIED., .F., .F.,
 ( 4, 2, 2, 2, 2, 2, 2, 4 ),
 ( 4.249187360970369464E-18, 0.002558063192038479913, 0.003837094788057715533, 0.005116126384076951153, 0.006395157980096183303, 0.007674189576115417188, 0.008953221172134649339, 0.01023225276815388322 ),
 .UNSPECIFIED. ) ;
#15181=CIRCLE ( 'NONE', #6750, 5.000000000000000000 ) ;
#15182=EDGE_CURVE ( 'NONE', #49437, #5514, #27, .T. ) ;
#15184=CARTESIAN_POINT ( 'NONE',  ( 47.00000000000000711, 4.705694406421931860E-17, -3.469127814946512892E-15 ) ) ;
#15187=CIRCLE ( 'NONE', #23704, 5.000000000000000888 ) ;
#15188=ORIENTED_EDGE ( 'NONE', *, *, #51041, .T. ) ;
#15191=CYLINDRICAL_SURFACE ( 'NONE', #31932, 12.74999999999999822 ) ;
#15193=DIRECTION ( 'NONE',  ( -1.000000000000000000, 0.000000000000000000, -0.000000000000000000 ) ) ;
#15195=FACE_BOUND ( 'NONE', #29578, .T. ) ;
#15196=ORIENTED_EDGE ( 'NONE', *, *, #45596, .F. ) ;
#15198=ORIENTED_EDGE ( 'NONE', *, *, #63346, .T. ) ;
#15206=CARTESIAN_POINT ( 'NONE',  ( -14.23194138997495273, 7.940651831586622578, 10.91941811743712876 ) ) ;
#15207=CARTESIAN_POINT ( 'NONE',  ( 37.00000000000000711, -12.15823808070322798, -0.8294751490778934366 ) ) ;
#15208=EDGE_LOOP ( 'NONE', ( #17630, #30352, #2260, #32898 ) ) ;
#15210=CARTESIAN_POINT ( 'NONE',  ( 21.98520202802499668, 11.37898758322522852, -3.828589025987038319 ) ) ;
#15212=CARTESIAN_POINT ( 'NONE',  ( 11.03672806164797215, 13.39240040767147555, -1.705299592209642556 ) ) ;
#15213=CARTESIAN_POINT ( 'NONE',  ( -10.48620311856347875, -9.720786832536937538, 25.00000000000000000 ) ) ;
#15214=LINE ( 'NONE', #45812, #39354 ) ;
#15215=CARTESIAN_POINT ( 'NONE',  ( -47.00000000000000711, 0.000000000000000000, 0.000000000000000000 ) ) ;
#15216=EDGE_CURVE ( 'NONE', #62620, #8491, #42627, .T. ) ;
#15217=CIRCLE ( 'NONE', #37538, 4.999999999999999112 ) ;
#15218=DIRECTION ( 'NONE',  ( 1.000000000000000000, 0.000000000000000000, 0.000000000000000000 ) ) ;
#15220=ORIENTED_EDGE ( 'NONE', *, *, #6976, .F. ) ;
#15222=CARTESIAN_POINT ( 'NONE',  ( -35.00000000000000000, 7.561043153947966999, 9.557269938331581116 ) ) ;
#15224=ORIENTED_EDGE ( 'NONE', *, *, #29636, .T. ) ;
#15225=LINE ( 'NONE', #55807, #27512 ) ;
#15227=CARTESIAN_POINT ( 'NONE',  ( -17.13652129973968741, 7.269150443694792685, -11.37692447958999864 ) ) ;
#15228=AXIS2_PLACEMENT_3D ( 'NONE', #38542, #1678, #33225 ) ;
#15231=ADVANCED_FACE ( 'NONE', ( #4415 ), #49955, .T. ) ;
#15232=ORIENTED_EDGE ( 'NONE', *, *, #24083, .T. ) ;
#15233=CIRCLE ( 'NONE', #56649, 12.75000000000000178 ) ;
#15235=DIRECTION ( 'NONE',  ( -1.000000000000000000, 0.000000000000000000, 0.000000000000000000 ) ) ;
#15236=CARTESIAN_POINT ( 'NONE',  ( -37.00000000000000711, 10.12742074351907817, -7.745827850122903868 ) ) ;
#15238=CIRCLE ( 'NONE', #1450, 5.000000000000000888 ) ;
#15239=CARTESIAN_POINT ( 'NONE',  ( 10.21737588954345100, 7.427574052226248114, -11.27660933775315755 ) ) ;
#15242=AXIS2_PLACEMENT_3D ( 'NONE', #3296, #23233, #53834 ) ;
#15244=ORIENTED_EDGE ( 'NONE', *, *, #11683, .T. ) ;
#15247=CARTESIAN_POINT ( 'NONE',  ( 29.22756163550774033, -7.948250717091969619, 9.002011177893463056 ) ) ;
#15248=EDGE_CURVE ( 'NONE', #28155, #52774, #43693, .T. ) ;
#15249=CARTESIAN_POINT ( 'NONE',  ( -37.00000000000000711, 11.30684963584389280, 4.545979934229452901 ) ) ;
#15250=EDGE_CURVE ( 'NONE', #41694, #63262, #41195, .T. ) ;
#15251=VECTOR ( 'NONE', #62451, 1000.000000000000000 ) ;
#15255=ADVANCED_FACE ( 'NONE', ( #10305 ), #35578, .T. ) ;
#15256=ORIENTED_EDGE ( 'NONE', *, *, #62323, .T. ) ;
#15258=CYLINDRICAL_SURFACE ( 'NONE', #47010, 4.285769192180103992 ) ;
#15259=FACE_OUTER_BOUND ( 'NONE', #4305, .T. ) ;
#15260=CARTESIAN_POINT ( 'NONE',  ( 37.00000000000000711, -7.379373053628790480, 10.39746860227898395 ) ) ;
#15262=EDGE_CURVE ( 'NONE', #41856, #63348, #49042, .T. ) ;
#15269=ORIENTED_EDGE ( 'NONE', *, *, #22157, .T. ) ;
#15274=DIRECTION ( 'NONE',  ( -1.000000000000000000, 0.000000000000000000, 0.000000000000000000 ) ) ;
#15275=ORIENTED_EDGE ( 'NONE', *, *, #39691, .F. ) ;
#15276=CARTESIAN_POINT ( 'NONE',  ( 37.00000000000000711, 1.463443770872944194, 12.09831040184922024 ) ) ;
#15277=AXIS2_PLACEMENT_3D ( 'NONE', #5197, #10489, #62036 ) ;
#15282=CIRCLE ( 'NONE', #60958, 12.75000000000000178 ) ;
#15283=ORIENTED_EDGE ( 'NONE', *, *, #39709, .F. ) ;
#15288=ORIENTED_EDGE ( 'NONE', *, *, #61312, .F. ) ;
#15289=ORIENTED_EDGE ( 'NONE', *, *, #56688, .F. ) ;
#15291=CIRCLE ( 'NONE', #49310, 5.000000000000000888 ) ;
#15294=ADVANCED_FACE ( 'NONE', ( #11302 ), #9993, .T. ) ;
#15295=DIRECTION ( 'NONE',  ( 1.000000000000000000, 0.000000000000000000, 0.000000000000000000 ) ) ;
#15296=DIRECTION ( 'NONE',  ( -1.000000000000000000, 0.000000000000000000, 0.000000000000000000 ) ) ;
#15299=LINE ( 'NONE', #20933, #3562 ) ;
#15300=EDGE_CURVE ( 'NONE', #26580, #4994, #59656, .T. ) ;
#15302=CARTESIAN_POINT ( 'NONE',  ( -37.00000000000000711, -6.102719229070750373, 10.54834585426218041 ) ) ;
#15304=DIRECTION ( 'NONE',  ( 0.000000000000000000, 0.01356324068817998940, -0.9999080150203990547 ) ) ;
#15305=ORIENTED_EDGE ( 'NONE', *, *, #6981, .F. ) ;
#15310=AXIS2_PLACEMENT_3D ( 'NONE', #41630, #46626, #36314 ) ;
#15311=ORIENTED_EDGE ( 'NONE', *, *, #40086, .T. ) ;
#15312=DIRECTION ( 'NONE',  ( -1.000000000000000000, -0.000000000000000000, 0.000000000000000000 ) ) ;
#15313=ORIENTED_EDGE ( 'NONE', *, *, #695, .F. ) ;
#15321=EDGE_LOOP ( 'NONE', ( #61815, #22539, #27997, #43860 ) ) ;
#15322=CIRCLE ( 'NONE', #32304, 4.999999999999999112 ) ;
#15323=DIRECTION ( 'NONE',  ( -1.000000000000000000, 0.000000000000000000, 0.000000000000000000 ) ) ;
#15324=CYLINDRICAL_SURFACE ( 'NONE', #48247, 12.74999999999999822 ) ;
#15325=DIRECTION ( 'NONE',  ( 1.000000000000000000, 0.000000000000000000, 0.000000000000000000 ) ) ;
#15328=DIRECTION ( 'NONE',  ( -1.000000000000000000, 0.000000000000000000, 0.000000000000000000 ) ) ;
#15332=FACE_OUTER_BOUND ( 'NONE', #16054, .T. ) ;
#15333=AXIS2_PLACEMENT_3D ( 'NONE', #96, #10080, #24376 ) ;
#15334=ADVANCED_FACE ( 'NONE', ( #57191 ), #6970, .T. ) ;
#15335=CIRCLE ( 'NONE', #32318, 4.999999999999999112 ) ;
#15337=EDGE_CURVE ( 'NONE', #55606, #5144, #30972, .T. ) ;
#15338=ORIENTED_EDGE ( 'NONE', *, *, #2808, .F. ) ;
#15339=CARTESIAN_POINT ( 'NONE',  ( -35.00000000000000000, 0.000000000000000000, 0.000000000000000000 ) ) ;
#15345=EDGE_LOOP ( 'NONE', ( #10622, #49239, #5980, #33092 ) ) ;
#15346=ORIENTED_EDGE ( 'NONE', *, *, #63581, .F. ) ;
#15347=ORIENTED_EDGE ( 'NONE', *, *, #28909, .F. ) ;
#15349=VECTOR ( 'NONE', #4272, 1000.000000000000000 ) ;
#15351=ORIENTED_EDGE ( 'NONE', *, *, #44055, .T. ) ;
#15352=DIRECTION ( 'NONE',  ( 0.000000000000000000, 0.000000000000000000, 1.000000000000000000 ) ) ;
#15353=DIRECTION ( 'NONE',  ( 0.000000000000000000, -1.000000000000000000, 0.000000000000000000 ) ) ;
#15358=CARTESIAN_POINT ( 'NONE',  ( -35.00000000000000000, -6.891188680298757419, -9.512294188640973758 ) ) ;
#15359=VERTEX_POINT ( 'NONE', #17925 ) ;
#15361=ORIENTED_EDGE ( 'NONE', *, *, #58971, .F. ) ;
#15362=CARTESIAN_POINT ( 'NONE',  ( -35.00000000000000000, 12.57916205664481168, 2.080187960898605581 ) ) ;
#15363=ORIENTED_EDGE ( 'NONE', *, *, #37117, .T. ) ;
#15364=CARTESIAN_POINT ( 'NONE',  ( 13.08854576485774857, -9.765169235090553457, -6.977652523680585972 ) ) ;
#15366=DIRECTION ( 'NONE',  ( 1.000000000000000000, 0.000000000000000000, 0.000000000000000000 ) ) ;
#15368=CARTESIAN_POINT ( 'NONE',  ( 37.00000000000000711, 9.240395740215630482, -7.251710744571611578 ) ) ;
#15375=CARTESIAN_POINT ( 'NONE',  ( 35.00000000000000000, 12.08216339958902630, 1.591260454995109930 ) ) ;
#15378=ORIENTED_EDGE ( 'NONE', *, *, #51138, .F. ) ;
#15380=ORIENTED_EDGE ( 'NONE', *, *, #58557, .T. ) ;
#15381=DIRECTION ( 'NONE',  ( 0.000000000000000000, 0.9551603052523489623, -0.2960891610144475439 ) ) ;
#15382=AXIS2_PLACEMENT_3D ( 'NONE', #21688, #16678, #22668 ) ;
#15383=ORIENTED_EDGE ( 'NONE', *, *, #1855, .T. ) ;
#15386=CARTESIAN_POINT ( 'NONE',  ( 35.00000000000000000, -9.621072037176933378, 8.366449238204463512 ) ) ;
#15387=FACE_OUTER_BOUND ( 'NONE', #65421, .T. ) ;
#15388=AXIS2_PLACEMENT_3D ( 'NONE', #15358, #9366, #9702 ) ;
#15389=CARTESIAN_POINT ( 'NONE',  ( 3.455078800971986386, 8.284346402942343701, -10.65933643386987306 ) ) ;
#15393=ORIENTED_EDGE ( 'NONE', *, *, #38840, .F. ) ;
#15394=CARTESIAN_POINT ( 'NONE',  ( 9.650011408859194617, -13.48023745212356239, -0.7481333718491276485 ) ) ;
#15401=DIRECTION ( 'NONE',  ( -1.000000000000000000, 0.000000000000000000, 0.000000000000000000 ) ) ;
#15402=B_SPLINE_CURVE_WITH_KNOTS ( 'NONE', 3,
 ( #3488, #13742, #3820, #28086, #34030, #17773, #29066, #44331, #64608, #54677, #29380, #33048, #34676, #24383, #24726, #40993, #45007, #4456, #60287, #14715 ),
 .UNSPECIFIED., .F., .F.,
 ( 4, 2, 2, 2, 2, 2, 2, 2, 2, 4 ),
 ( 1.274756208291110993E-17, 0.001996908854952089522, 0.002995363282428130380, 0.003993817709904172106, 0.004992272137380212964, 0.005491499351118232959, 0.005990726564856252954, 0.006489953778594273817, 0.006989180992332292945, 0.007987635419808342477 ),
 .UNSPECIFIED. ) ;
#15404=ORIENTED_EDGE ( 'NONE', *, *, #11541, .F. ) ;
#15405=CARTESIAN_POINT ( 'NONE',  ( 35.00000000000000000, 3.287724142101414504, -11.73463472867577373 ) ) ;
#15406=AXIS2_PLACEMENT_3D ( 'NONE', #59601, #64892, #13065 ) ;
#15409=ADVANCED_FACE ( 'NONE', ( #26924 ), #28232, .T. ) ;
#15410=DIRECTION ( 'NONE',  ( 0.000000000000000000, 0.01356324068817998940, -0.9999080150203990547 ) ) ;
#15412=CIRCLE ( 'NONE', #9058, 12.18649999999999878 ) ;
#15413=VERTEX_POINT ( 'NONE', #57521 ) ;
#15417=ORIENTED_EDGE ( 'NONE', *, *, #58394, .T. ) ;
#15419=CARTESIAN_POINT ( 'NONE',  ( -2.952869152607106251, 25.00000000000000000, 3.755417052241485365 ) ) ;
#15420=EDGE_LOOP ( 'NONE', ( #7709, #51510, #15275, #46283 ) ) ;
#15423=CIRCLE ( 'NONE', #41995, 5.000000000000001776 ) ;
#15424=EDGE_CURVE ( 'NONE', #41991, #60869, #45685, .T. ) ;
#15428=DIRECTION ( 'NONE',  ( 1.000000000000000000, 0.000000000000000000, 0.000000000000000000 ) ) ;
#15429=CARTESIAN_POINT ( 'NONE',  ( 6.661406098020968614, -4.211117136771885150, 11.23710102852283299 ) ) ;
#15430=CARTESIAN_POINT ( 'NONE',  ( -35.00000000000000000, -3.093009498344009955, 11.78745411414838884 ) ) ;
#15432=CARTESIAN_POINT ( 'NONE',  ( 35.00000000000000000, 4.705694406421931860E-17, -3.469127814946512892E-15 ) ) ;
#15433=DIRECTION ( 'NONE',  ( -1.000000000000000000, 0.000000000000000000, 0.000000000000000000 ) ) ;
#15435=CARTESIAN_POINT ( 'NONE',  ( 47.00000000000000711, 4.705694406421931860E-17, -3.469127814946512892E-15 ) ) ;
#15436=ORIENTED_EDGE ( 'NONE', *, *, #46782, .T. ) ;
#15438=VERTEX_POINT ( 'NONE', #59157 ) ;
#15439=ORIENTED_EDGE ( 'NONE', *, *, #45696, .T. ) ;
#15442=DIRECTION ( 'NONE',  ( 0.000000000000000000, -0.01356324068817991828, 0.9999080150203990547 ) ) ;
#15444=EDGE_CURVE ( 'NONE', #32997, #34038, #55690, .T. ) ;
#15445=CARTESIAN_POINT ( 'NONE',  ( -11.40165637463000614, -7.508992741355387857, -11.21895841913464587 ) ) ;
#15446=LINE ( 'NONE', #45706, #62224 ) ;
#15447=LINE ( 'NONE', #6146, #17141 ) ;
#15448=ORIENTED_EDGE ( 'NONE', *, *, #14596, .F. ) ;
#15453=ADVANCED_FACE ( 'NONE', ( #8591 ), #38528, .T. ) ;
#15454=EDGE_CURVE ( 'NONE', #53805, #43974, #61033, .T. ) ;
#15456=CARTESIAN_POINT ( 'NONE',  ( 3.291290029914074378, 8.250315036047103590, 8.713914264323182834 ) ) ;
#15457=CARTESIAN_POINT ( 'NONE',  ( 9.887190305652888256, 7.804856637177040035, -9.121441579706537794 ) ) ;
#15459=CARTESIAN_POINT ( 'NONE',  ( 18.41452685719870530, -4.205716937948009715, 11.29046638959579063 ) ) ;
#15461=DIRECTION ( 'NONE',  ( 0.000000000000000000, 0.01356324068817992175, -0.9999080150203990547 ) ) ;
#15462=EDGE_CURVE ( 'NONE', #51695, #26384, #26139, .T. ) ;
#15463=EDGE_LOOP ( 'NONE', ( #58325, #55498, #47033, #26592 ) ) ;
#15465=ORIENTED_EDGE ( 'NONE', *, *, #5994, .F. ) ;
#15468=CARTESIAN_POINT ( 'NONE',  ( 37.00000000000000711, 3.307597835713414369, 12.31350058095519096 ) ) ;
#15469=AXIS2_PLACEMENT_3D ( 'NONE', #61993, #10136, #35049 ) ;
#15472=ADVANCED_FACE ( 'NONE', ( #34815 ), #53837, .T. ) ;
#15473=FACE_OUTER_BOUND ( 'NONE', #35897, .T. ) ;
#15475=DIRECTION ( 'NONE',  ( -1.000000000000000000, 0.000000000000000000, 0.000000000000000000 ) ) ;
#15476=ORIENTED_EDGE ( 'NONE', *, *, #908, .F. ) ;
#15481=DIRECTION ( 'NONE',  ( 1.000000000000000000, -0.000000000000000000, 0.000000000000000000 ) ) ;
#15483=CARTESIAN_POINT ( 'NONE',  ( -17.17991164731014564, -8.042067640992478061, -10.84821509031881526 ) ) ;
#15488=CARTESIAN_POINT ( 'NONE',  ( -17.70181089779288186, 6.586671166928411481, -10.03326520023147594 ) ) ;
#15491=ORIENTED_EDGE ( 'NONE', *, *, #9179, .T. ) ;
#15492=CYLINDRICAL_SURFACE ( 'NONE', #46945, 5.000000000000000000 ) ;
#15497=CARTESIAN_POINT ( 'NONE',  ( -9.008580248661141709, 10.91680307554687523, -7.949412954711231549 ) ) ;
#15498=LINE ( 'NONE', #36773, #32169 ) ;
#15499=AXIS2_PLACEMENT_3D ( 'NONE', #49386, #38720, #18464 ) ;
#15502=DIRECTION ( 'NONE',  ( 0.000000000000000000, 0.01356324068817998940, -0.9999080150203989437 ) ) ;
#15505=DIRECTION ( 'NONE',  ( 0.000000000000000000, -0.01356324068817991828, 0.9999080150203990547 ) ) ;
#15510=EDGE_CURVE ( 'NONE', #42839, #15077, #36733, .T. ) ;
#15511=DIRECTION ( 'NONE',  ( 0.000000000000000000, 0.9970832820307036215, 0.07632122047556835764 ) ) ;
#15515=CARTESIAN_POINT ( 'NONE',  ( -35.00000000000000000, 6.564808257521927537, -10.93004082984011482 ) ) ;
#15516=EDGE_CURVE ( 'NONE', #65388, #17474, #5776, .T. ) ;
#15517=FACE_BOUND ( 'NONE', #39262, .T. ) ;
#15518=ORIENTED_EDGE ( 'NONE', *, *, #33160, .T. ) ;
#15519=ORIENTED_EDGE ( 'NONE', *, *, #57144, .T. ) ;
#15521=ADVANCED_FACE ( 'NONE', ( #37045 ), #1165, .T. ) ;
#15522=ORIENTED_EDGE ( 'NONE', *, *, #58041, .T. ) ;
#15523=FACE_OUTER_BOUND ( 'NONE', #47028, .T. ) ;
#15525=CARTESIAN_POINT ( 'NONE',  ( -37.00000000000000711, -3.340853584269456888, -11.26103545359859304 ) ) ;
#15527=DIRECTION ( 'NONE',  ( 1.000000000000000000, 0.000000000000000000, 0.000000000000000000 ) ) ;
#15528=CARTESIAN_POINT ( 'NONE',  ( -14.17344535826537744, 8.096743466816493040, 10.80418385471381448 ) ) ;
#15529=EDGE_CURVE ( 'NONE', #54167, #59596, #54617, .T. ) ;
#15531=VERTEX_POINT ( 'NONE', #21101 ) ;
#15532=DIRECTION ( 'NONE',  ( 1.000000000000000000, 0.000000000000000000, 0.000000000000000000 ) ) ;
#15533=EDGE_CURVE ( 'NONE', #35052, #64499, #9863, .T. ) ;
#15534=CYLINDRICAL_SURFACE ( 'NONE', #62910, 6.095312090839646757 ) ;
#15536=CARTESIAN_POINT ( 'NONE',  ( -19.32298883157327296, 13.49691393547099239, -0.7062062602696702607 ) ) ;
#15537=CARTESIAN_POINT ( 'NONE',  ( -27.01437459610461644, 25.00000000000000000, -2.220455681983952267 ) ) ;
#15538=DIRECTION ( 'NONE',  ( -0.000000000000000000, -0.000000000000000000, -1.000000000000000000 ) ) ;
#15540=CARTESIAN_POINT ( 'NONE',  ( -37.00000000000000711, -10.49626516989265923, -7.238157050195740183 ) ) ;
#15541=ADVANCED_FACE ( 'NONE', ( #12110 ), #42037, .T. ) ;
#15542=ORIENTED_EDGE ( 'NONE', *, *, #38962, .T. ) ;
#15544=AXIS2_PLACEMENT_3D ( 'NONE', #35371, #29410, #19111 ) ;
#15546=VECTOR ( 'NONE', #19990, 1000.000000000000000 ) ;
#15547=ORIENTED_EDGE ( 'NONE', *, *, #47234, .T. ) ;
#15548=CARTESIAN_POINT ( 'NONE',  ( -2.748241610611773300, -11.18522623946203609, 4.360826414742480672 ) ) ;
#15550=CARTESIAN_POINT ( 'NONE',  ( -14.86395414634036882, 7.932783874389932599, -10.92342345601903908 ) ) ;
#15551=EDGE_CURVE ( 'NONE', #2297, #14551, #26425, .T. ) ;
#15554=B_SPLINE_CURVE_WITH_KNOTS ( 'NONE', 3,
 ( #2570, #17520, #22839, #12497, #13484, #63370, #58410, #49104, #58084, #48445 ),
 .UNSPECIFIED., .F., .F.,
 ( 4, 2, 2, 2, 4 ),
 ( 0.000000000000000000, 0.002581029528971738683, 0.003226286911214673245, 0.003871544293457608241, 0.005162059057943477365 ),
 .UNSPECIFIED. ) ;
#15555=ORIENTED_EDGE ( 'NONE', *, *, #29695, .T. ) ;
#15557=CARTESIAN_POINT ( 'NONE',  ( -30.16280033943767336, -2.214233674731126644, -11.80068582467317739 ) ) ;
#15564=ORIENTED_EDGE ( 'NONE', *, *, #3587, .F. ) ;
#15567=CARTESIAN_POINT ( 'NONE',  ( 29.21000934519853942, -6.487399748294825130, 10.13727455448839798 ) ) ;
#15569=EDGE_CURVE ( 'NONE', #11924, #39344, #41867, .T. ) ;
#15571=ORIENTED_EDGE ( 'NONE', *, *, #49546, .T. ) ;
#15573=ORIENTED_EDGE ( 'NONE', *, *, #14154, .T. ) ;
#15574=DIRECTION ( 'NONE',  ( -1.000000000000000000, 0.000000000000000000, 0.000000000000000000 ) ) ;
#15577=CARTESIAN_POINT ( 'NONE',  ( -27.01437459610461644, 10.69338818478080455, -8.240233560378637634 ) ) ;
#15578=CARTESIAN_POINT ( 'NONE',  ( -35.00000000000000000, -11.98254675519229906, 2.220215194441857331 ) ) ;
#15579=CYLINDRICAL_SURFACE ( 'NONE', #45575, 4.999999999999999112 ) ;
#15580=DIRECTION ( 'NONE',  ( 0.000000000000000000, -0.01356324068817998940, 0.9999080150203990547 ) ) ;
#15581=ORIENTED_EDGE ( 'NONE', *, *, #45190, .T. ) ;
#15582=EDGE_CURVE ( 'NONE', #13554, #16743, #2597, .T. ) ;
#15584=ORIENTED_EDGE ( 'NONE', *, *, #14327, .F. ) ;
#15585=AXIS2_PLACEMENT_3D ( 'NONE', #31322, #11356, #45619 ) ;
#15586=CARTESIAN_POINT ( 'NONE',  ( 37.00000000000000711, -10.12742074351890764, 7.745827850123116143 ) ) ;
#15588=CYLINDRICAL_SURFACE ( 'NONE', #21551, 12.74999999999999822 ) ;
#15589=EDGE_CURVE ( 'NONE', #43482, #58117, #49367, .T. ) ;
#15591=CIRCLE ( 'NONE', #9229, 12.18649999999999878 ) ;
#15594=DIRECTION ( 'NONE',  ( -1.000000000000000000, 0.000000000000000000, 0.000000000000000000 ) ) ;
#15595=CARTESIAN_POINT ( 'NONE',  ( 4.640500126211298593, -10.09411786235453690, -8.965292744499050670 ) ) ;
#15596=LINE ( 'NONE', #5657, #30759 ) ;
#15597=CARTESIAN_POINT ( 'NONE',  ( 6.516094201635106664, -8.971286330002193665, 7.981610909288549216 ) ) ;
#15598=ORIENTED_EDGE ( 'NONE', *, *, #31657, .T. ) ;
#15599=ORIENTED_EDGE ( 'NONE', *, *, #64780, .T. ) ;
#15601=EDGE_CURVE ( 'NONE', #476, #48664, #58895, .T. ) ;
#15602=ORIENTED_EDGE ( 'NONE', *, *, #48493, .T. ) ;
#15603=LINE ( 'NONE', #6305, #18916 ) ;
#15604=VERTEX_POINT ( 'NONE', #47055 ) ;
#15606=ORIENTED_EDGE ( 'NONE', *, *, #39577, .T. ) ;
#15612=DIRECTION ( 'NONE',  ( -1.000000000000000000, 0.000000000000000000, 0.000000000000000000 ) ) ;
#15613=ORIENTED_EDGE ( 'NONE', *, *, #61127, .T. ) ;
#15614=DIRECTION ( 'NONE',  ( -1.000000000000000000, 0.000000000000000000, 0.000000000000000000 ) ) ;
#15616=CARTESIAN_POINT ( 'NONE',  ( -17.08916676964391357, 2.790706569880187171, 13.20909463602864697 ) ) ;
#15617=DIRECTION ( 'NONE',  ( 0.000000000000000000, 0.01356324068817998940, -0.9999080150203989437 ) ) ;
#15618=CARTESIAN_POINT ( 'NONE',  ( 35.00000000000000000, 9.321877890560537949, 7.146664589317804683 ) ) ;
#15620=CARTESIAN_POINT ( 'NONE',  ( -37.00000000000000711, 1.456211999474342766, 11.65554240571057854 ) ) ;
#15621=DIRECTION ( 'NONE',  ( 0.000000000000000000, -0.8827602140260367714, 0.4698238015817268742 ) ) ;
#15622=ADVANCED_FACE ( 'NONE', ( #46387 ), #31418, .T. ) ;
#15628=DIRECTION ( 'NONE',  ( -1.000000000000000000, 0.000000000000000000, -0.000000000000000000 ) ) ;
#15642=CARTESIAN_POINT ( 'NONE',  ( -35.00000000000000000, -1.113475361586400814, -12.70128625845194215 ) ) ;
#15643=EDGE_CURVE ( 'NONE', #5805, #40836, #53349, .T. ) ;
#15646=ORIENTED_EDGE ( 'NONE', *, *, #54760, .T. ) ;
#15649=DIRECTION ( 'NONE',  ( -1.000000000000000000, 0.000000000000000000, 0.000000000000000000 ) ) ;
#15650=ORIENTED_EDGE ( 'NONE', *, *, #55768, .F. ) ;
#15651=EDGE_CURVE ( 'NONE', #31935, #44696, #27019, .T. ) ;
#15652=ORIENTED_EDGE ( 'NONE', *, *, #26567, .F. ) ;
#15653=EDGE_LOOP ( 'NONE', ( #40261, #22376, #41273, #45608 ) ) ;
#15655=AXIS2_PLACEMENT_3D ( 'NONE', #38930, #58913, #13326 ) ;
#15658=CYLINDRICAL_SURFACE ( 'NONE', #21527, 4.999999999999999112 ) ;
#15659=CIRCLE ( 'NONE', #10352, 12.74999999999999822 ) ;
#15660=EDGE_LOOP ( 'NONE', ( #11443, #29688, #29984, #44319 ) ) ;
#15661=DIRECTION ( 'NONE',  ( -0.000000000000000000, -0.000000000000000000, -1.000000000000000000 ) ) ;
#15663=FACE_OUTER_BOUND ( 'NONE', #18607, .T. ) ;
#15664=ORIENTED_EDGE ( 'NONE', *, *, #42312, .T. ) ;
#15665=FACE_OUTER_BOUND ( 'NONE', #57800, .T. ) ;
#15666=EDGE_CURVE ( 'NONE', #29924, #1294, #53996, .T. ) ;
#15667=ORIENTED_EDGE ( 'NONE', *, *, #27777, .F. ) ;
#15672=CARTESIAN_POINT ( 'NONE',  ( -35.00000000000000000, 3.805206332242643263, -12.16893194857546057 ) ) ;
#15673=DIRECTION ( 'NONE',  ( 1.000000000000000000, 0.000000000000000000, -0.000000000000000000 ) ) ;
#15674=LINE ( 'NONE', #46298, #60165 ) ;
#15675=CARTESIAN_POINT ( 'NONE',  ( 37.00000000000000711, 9.506317355798490354, 8.496612874013054650 ) ) ;
#15676=AXIS2_PLACEMENT_3D ( 'NONE', #64735, #43828, #18589 ) ;
#15677=CARTESIAN_POINT ( 'NONE',  ( 35.00000000000000000, -4.732539170486179003, 11.23004253107769124 ) ) ;
#15679=DIRECTION ( 'NONE',  ( -0.000000000000000000, -0.000000000000000000, -1.000000000000000000 ) ) ;
#15680=FACE_OUTER_BOUND ( 'NONE', #1261, .T. ) ;
#15681=ORIENTED_EDGE ( 'NONE', *, *, #25654, .T. ) ;
#15682=LINE ( 'NONE', #25039, #20474 ) ;
#15683=ORIENTED_EDGE ( 'NONE', *, *, #61763, .F. ) ;
#15684=CARTESIAN_POINT ( 'NONE',  ( 13.15144582642090754, -12.98672512126129419, -3.693064144862436837 ) ) ;
#15685=VERTEX_POINT ( 'NONE', #33385 ) ;
#15687=ORIENTED_EDGE ( 'NONE', *, *, #60542, .T. ) ;
#15689=DIRECTION ( 'NONE',  ( -0.000000000000000000, -0.000000000000000000, -1.000000000000000000 ) ) ;
#15690=LINE ( 'NONE', #22008, #56723 ) ;
#15694=VERTEX_POINT ( 'NONE', #18761 ) ;
#15695=CARTESIAN_POINT ( 'NONE',  ( 37.00000000000000711, -10.23119532541066867, 7.608228585767832897 ) ) ;
#15696=EDGE_CURVE ( 'NONE', #42832, #35285, #14232, .T. ) ;
#15697=( BOUNDED_CURVE ( )  B_SPLINE_CURVE ( 3, ( #48237, #33880, #8615, #18287 ),
 .UNSPECIFIED., .F., .F. ) 
 B_SPLINE_CURVE_WITH_KNOTS ( ( 4, 4 ),
 ( 1.904964486966213011, 1.936058588204076836 ),
 .UNSPECIFIED. ) 
 CURVE ( )  GEOMETRIC_REPRESENTATION_ITEM ( )  RATIONAL_B_SPLINE_CURVE ( ( 1.000000000000000000, 0.9999194313618959828, 0.9999194313618959828, 1.000000000000000000 ) ) 
 REPRESENTATION_ITEM ( '' )  );
#15698=ORIENTED_EDGE ( 'NONE', *, *, #44705, .F. ) ;
#15699=CARTESIAN_POINT ( 'NONE',  ( 9.612882454814815958, -13.47023598955340162, -0.9106303824545916026 ) ) ;
#15700=LINE ( 'NONE', #10083, #57903 ) ;
#15701=EDGE_CURVE ( 'NONE', #15987, #38977, #1543, .T. ) ;
#15703=ORIENTED_EDGE ( 'NONE', *, *, #39872, .T. ) ;
#15704=CARTESIAN_POINT ( 'NONE',  ( -36.00000000000000711, -1.286231064351400555, 12.68495603654571369 ) ) ;
#15706=CARTESIAN_POINT ( 'NONE',  ( 29.22869416613001547, 10.03734508462482289, 9.037510697015965988 ) ) ;
#15708=CARTESIAN_POINT ( 'NONE',  ( -29.60090551182471685, -2.920537340839129303, 11.66374641461455042 ) ) ;
#15709=CARTESIAN_POINT ( 'NONE',  ( -37.00000000000000711, 0.000000000000000000, 0.000000000000000000 ) ) ;
#15710=CARTESIAN_POINT ( 'NONE',  ( -35.00000000000000000, 9.390600770287994337, 8.624332853796092380 ) ) ;
#15712=VERTEX_POINT ( 'NONE', #37719 ) ;
#15713=LINE ( 'NONE', #5115, #22455 ) ;
#15716=VECTOR ( 'NONE', #17768, 1000.000000000000000 ) ;
#15717=B_SPLINE_CURVE_WITH_KNOTS ( 'NONE', 3,
 ( #30067, #65622, #40359, #36373, #148, #16084, #65317, #20429 ),
 .UNSPECIFIED., .F., .F.,
 ( 4, 2, 2, 4 ),
 ( 0.004604583187049208354, 0.006625549100428843735, 0.007636032057118663161, 0.008646515013808482586 ),
 .UNSPECIFIED. ) ;
#15719=CARTESIAN_POINT ( 'NONE',  ( 18.90103867708235086, -7.635891018350232429, 11.15525402366580821 ) ) ;
#15720=ADVANCED_FACE ( 'NONE', ( #53683 ), #13418, .T. ) ;
#15723=CARTESIAN_POINT ( 'NONE',  ( 3.245536480809931401, 4.729013804446176472, -11.03678433915268364 ) ) ;
#15725=VERTEX_POINT ( 'NONE', #3483 ) ;
#15727=CYLINDRICAL_SURFACE ( 'NONE', #15017, 12.74999999999999822 ) ;
#15728=ORIENTED_EDGE ( 'NONE', *, *, #16835, .T. ) ;
#15729=ORIENTED_EDGE ( 'NONE', *, *, #55900, .F. ) ;
#15732=EDGE_CURVE ( 'NONE', #43228, #12145, #23752, .T. ) ;
#15733=EDGE_LOOP ( 'NONE', ( #19246, #19772, #46554, #26508 ) ) ;
#15734=DIRECTION ( 'NONE',  ( 1.000000000000000000, -0.000000000000000000, 0.000000000000000000 ) ) ;
#15736=LINE ( 'NONE', #36366, #20570 ) ;
#15737=DIRECTION ( 'NONE',  ( 0.000000000000000000, 0.8515178078024887576, -0.5243256840888532722 ) ) ;
#15738=ORIENTED_EDGE ( 'NONE', *, *, #25616, .T. ) ;
#15740=VECTOR ( 'NONE', #65338, 1000.000000000000000 ) ;
#15741=B_SPLINE_CURVE_WITH_KNOTS ( 'NONE', 3,
 ( #3195, #49086, #12814, #24118, #9141, #17820, #59058, #28440, #29424, #34076, #18810, #39069, #59364, #53409, #43076, #63673, #59699, #18150, #23133, #13160, #33442, #23461, #14126, #2551 ),
 .UNSPECIFIED., .F., .F.,
 ( 4, 2, 2, 2, 2, 2, 2, 2, 2, 2, 2, 4 ),
 ( 6.009258394948636926E-18, 0.001190494761224138035, 0.002380989522448269998, 0.003571484283672401745, 0.004166731664284471087, 0.004761979044896539129, 0.005357226425508608038, 0.005952473806120676079, 0.006547721186732744121, 0.007142968567344811295, 0.008333463328568954318, 0.009523958089793097340 ),
 .UNSPECIFIED. ) ;
#15743=CARTESIAN_POINT ( 'NONE',  ( 37.00000000000000711, 11.60979404548634619, -3.704519465651352483 ) ) ;
#15745=ORIENTED_EDGE ( 'NONE', *, *, #28018, .T. ) ;
#15746=DIRECTION ( 'NONE',  ( -1.000000000000000000, -0.000000000000000000, 0.000000000000000000 ) ) ;
#15747=EDGE_CURVE ( 'NONE', #27703, #34385, #2826, .T. ) ;
#15749=LINE ( 'NONE', #55350, #50809 ) ;
#15751=ORIENTED_EDGE ( 'NONE', *, *, #60559, .F. ) ;
#15752=DIRECTION ( 'NONE',  ( 1.000000000000000000, 0.000000000000000000, -0.000000000000000000 ) ) ;
#15754=ADVANCED_FACE ( 'NONE', ( #64294 ), #3145, .T. ) ;
#15755=AXIS2_PLACEMENT_3D ( 'NONE', #11611, #57515, #36567 ) ;
#15759=CARTESIAN_POINT ( 'NONE',  ( 35.00000000000000000, 4.561791185930414549, -11.90598845858535526 ) ) ;
#15760=EDGE_LOOP ( 'NONE', ( #15581, #44277, #46074, #21586 ) ) ;
#15761=AXIS2_PLACEMENT_3D ( 'NONE', #2601, #57451, #26522 ) ;
#15762=ORIENTED_EDGE ( 'NONE', *, *, #63187, .F. ) ;
#15763=CARTESIAN_POINT ( 'NONE',  ( 47.00000000000000711, 4.705694406421931860E-17, -3.469127814946512892E-15 ) ) ;
#15765=AXIS2_PLACEMENT_3D ( 'NONE', #45631, #20367, #60940 ) ;
#15766=ORIENTED_EDGE ( 'NONE', *, *, #39285, .T. ) ;
#15767=CARTESIAN_POINT ( 'NONE',  ( 37.00000000000000711, 10.80478261802181805, -5.636262487437360136 ) ) ;
#15769=AXIS2_PLACEMENT_3D ( 'NONE', #18830, #43767, #13809 ) ;
#15773=EDGE_CURVE ( 'NONE', #6738, #14524, #62044, .T. ) ;
#15774=FACE_OUTER_BOUND ( 'NONE', #53172, .T. ) ;
#15776=EDGE_LOOP ( 'NONE', ( #35903, #42665, #22384, #35119 ) ) ;
#15777=DIRECTION ( 'NONE',  ( 0.000000000000000000, 0.4698238015817364777, 0.8827602140260315533 ) ) ;
#15781=CARTESIAN_POINT ( 'NONE',  ( 37.00000000000000711, -11.35427606708803161, 4.426194442447358490 ) ) ;
#15783=DIRECTION ( 'NONE',  ( 0.000000000000000000, -0.6269146997507876184, -0.7790879021242596014 ) ) ;
#15784=VECTOR ( 'NONE', #10382, 1000.000000000000000 ) ;
#15785=DIRECTION ( 'NONE',  ( 0.000000000000000000, 0.9718671068226450993, -0.2355298848897551256 ) ) ;
#15786=DIRECTION ( 'NONE',  ( 0.000000000000000000, 0.1118654143051546479, 0.9937233664769768993 ) ) ;
#15788=VERTEX_POINT ( 'NONE', #29061 ) ;
#15790=DIRECTION ( 'NONE',  ( -1.000000000000000000, -0.000000000000000000, 0.000000000000000000 ) ) ;
#15791=FACE_OUTER_BOUND ( 'NONE', #43161, .T. ) ;
#15794=CARTESIAN_POINT ( 'NONE',  ( 37.00000000000000711, 7.561043153948100226, 9.557269938331470982 ) ) ;
#15797=ORIENTED_EDGE ( 'NONE', *, *, #4016, .F. ) ;
#15798=CARTESIAN_POINT ( 'NONE',  ( -17.87896547527707014, -5.103338146098263195, -12.49897969532171160 ) ) ;
#15799=DIRECTION ( 'NONE',  ( -0.000000000000000000, -0.000000000000000000, -1.000000000000000000 ) ) ;
#15803=EDGE_CURVE ( 'NONE', #23216, #58222, #49366, .T. ) ;
#15804=CARTESIAN_POINT ( 'NONE',  ( 35.00000000000000000, 2.696588552979229725, 12.46157735505186004 ) ) ;
#15806=CARTESIAN_POINT ( 'NONE',  ( -30.18541646480390384, -1.416020129149325513, 13.42553116244798517 ) ) ;
#15807=CIRCLE ( 'NONE', #24321, 12.74999999999999822 ) ;
#15808=FACE_OUTER_BOUND ( 'NONE', #32844, .T. ) ;
#15811=EDGE_CURVE ( 'NONE', #50088, #41521, #45000, .T. ) ;
#15814=CARTESIAN_POINT ( 'NONE',  ( -36.00000000000000711, 8.017674001891920810, -9.913596905230035006 ) ) ;
#15815=DIRECTION ( 'NONE',  ( 1.000000000000000000, 0.000000000000000000, 0.000000000000000000 ) ) ;
#15817=CARTESIAN_POINT ( 'NONE',  ( 37.00000000000000711, 4.705694406421931860E-17, -3.469127814946512892E-15 ) ) ;
#15819=CARTESIAN_POINT ( 'NONE',  ( -18.45078447393003529, 4.179087011105350413, 12.83947810587989657 ) ) ;
#15821=EDGE_CURVE ( 'NONE', #6431, #38541, #10022, .T. ) ;
#15824=ORIENTED_EDGE ( 'NONE', *, *, #2071, .F. ) ;
#15827=AXIS2_PLACEMENT_3D ( 'NONE', #31583, #46895, #35594 ) ;
#15828=CARTESIAN_POINT ( 'NONE',  ( 37.00000000000000711, -3.704519465651390675, -11.60979404548633731 ) ) ;
#15829=VERTEX_POINT ( 'NONE', #55294 ) ;
#15830=DIRECTION ( 'NONE',  ( -1.000000000000000000, 0.000000000000000000, 0.000000000000000000 ) ) ;
#15831=CARTESIAN_POINT ( 'NONE',  ( -24.33291729085842192, -8.849064928703691990, 8.108208844799051462 ) ) ;
#15835=ORIENTED_EDGE ( 'NONE', *, *, #25219, .T. ) ;
#15836=CARTESIAN_POINT ( 'NONE',  ( 27.36401306237657849, -12.63164339974623829, 4.766274618149700437 ) ) ;
#15839=CARTESIAN_POINT ( 'NONE',  ( -35.00000000000000000, 6.036400161834567513, 10.07641281632180075 ) ) ;
#15840=DIRECTION ( 'NONE',  ( 0.000000000000000000, -0.9903235168508535136, -0.1387779952735919697 ) ) ;
#15842=VECTOR ( 'NONE', #56750, 1000.000000000000000 ) ;
#15846=VECTOR ( 'NONE', #30217, 1000.000000000000000 ) ;
#15847=ORIENTED_EDGE ( 'NONE', *, *, #23934, .T. ) ;
#15848=FACE_OUTER_BOUND ( 'NONE', #42491, .T. ) ;
#15849=LINE ( 'NONE', #21182, #58683 ) ;
#15850=LINE ( 'NONE', #36129, #13641 ) ;
#15852=CARTESIAN_POINT ( 'NONE',  ( 35.00000000000000000, 1.457575200925545822, -12.66641127287626567 ) ) ;
#15854=CYLINDRICAL_SURFACE ( 'NONE', #5850, 12.74999999999999822 ) ;
#15855=CIRCLE ( 'NONE', #43488, 4.999999999999999112 ) ;
#15856=LINE ( 'NONE', #51145, #10677 ) ;
#15858=ADVANCED_FACE ( 'NONE', ( #4450 ), #59644, .T. ) ;
#15861=AXIS2_PLACEMENT_3D ( 'NONE', #64845, #29294, #65191 ) ;
#15862=ORIENTED_EDGE ( 'NONE', *, *, #35585, .F. ) ;
#15864=CARTESIAN_POINT ( 'NONE',  ( -35.00000000000000000, -6.657191900728257394, -9.677500615117970995 ) ) ;
#15866=CARTESIAN_POINT ( 'NONE',  ( -35.00000000000000000, 0.000000000000000000, 0.000000000000000000 ) ) ;
#15867=VERTEX_POINT ( 'NONE', #25051 ) ;
#15872=CIRCLE ( 'NONE', #25439, 5.000000000000000000 ) ;
#15874=AXIS2_PLACEMENT_3D ( 'NONE', #37374, #37713, #6813 ) ;
#15875=CARTESIAN_POINT ( 'NONE',  ( 9.147487969233463190, 5.798649334944467881, -12.19629036017794377 ) ) ;
#15876=CARTESIAN_POINT ( 'NONE',  ( -35.00000000000000000, -6.475373545682229448, -10.32377448871674908 ) ) ;
#15879=EDGE_CURVE ( 'NONE', #54738, #22062, #35329, .T. ) ;
#15881=ORIENTED_EDGE ( 'NONE', *, *, #5156, .T. ) ;
#15882=EDGE_CURVE ( 'NONE', #41187, #36819, #54673, .T. ) ;
#15883=CARTESIAN_POINT ( 'NONE',  ( -35.00000000000000000, 12.08216339958900676, 1.591260454995285789 ) ) ;
#15885=CARTESIAN_POINT ( 'NONE',  ( 26.47593756983254210, -11.32194551905248048, 3.984718518152139399 ) ) ;
#15886=CARTESIAN_POINT ( 'NONE',  ( 35.00000000000000000, 4.705694406421931860E-17, -3.469127814946512892E-15 ) ) ;
#15887=AXIS2_PLACEMENT_3D ( 'NONE', #31296, #16336, #16653 ) ;
#15889=ADVANCED_FACE ( 'NONE', ( #49990 ), #9091, .T. ) ;
#15890=VERTEX_POINT ( 'NONE', #44327 ) ;
#15891=DIRECTION ( 'NONE',  ( 1.000000000000000000, 0.000000000000000000, 0.000000000000000000 ) ) ;
#15893=VECTOR ( 'NONE', #40343, 1000.000000000000000 ) ;
#15894=CYLINDRICAL_SURFACE ( 'NONE', #64864, 12.18649999999999878 ) ;
#15896=CARTESIAN_POINT ( 'NONE',  ( 35.00000000000000000, -0.4871980014160587347, 12.74068829017553739 ) ) ;
#15899=DIRECTION ( 'NONE',  ( -1.000000000000000000, 0.000000000000000000, 0.000000000000000000 ) ) ;
#15900=ADVANCED_FACE ( 'NONE', ( #24721 ), #64934, .T. ) ;
#15901=DIRECTION ( 'NONE',  ( -1.000000000000000000, 0.000000000000000000, 0.000000000000000000 ) ) ;
#15903=ORIENTED_EDGE ( 'NONE', *, *, #2602, .T. ) ;
#15904=CARTESIAN_POINT ( 'NONE',  ( -9.036476730761222598, -11.24534018395614154, -4.204006637871185781 ) ) ;
#15905=CIRCLE ( 'NONE', #53092, 12.18649999999999878 ) ;
#15906=VERTEX_POINT ( 'NONE', #59978 ) ;
#15908=CARTESIAN_POINT ( 'NONE',  ( 21.64317917535383984, -12.68252773215642470, -4.630549806628736498 ) ) ;
#15911=EDGE_CURVE ( 'NONE', #63611, #39378, #19075, .T. ) ;
#15912=DIRECTION ( 'NONE',  ( 1.000000000000000000, 1.836970198721029688E-16, 0.000000000000000000 ) ) ;
#15913=VERTEX_POINT ( 'NONE', #19742 ) ;
#15914=CYLINDRICAL_SURFACE ( 'NONE', #14801, 12.18649999999999878 ) ;
#15915=LINE ( 'NONE', #56857, #50972 ) ;
#15917=ORIENTED_EDGE ( 'NONE', *, *, #46413, .F. ) ;
#15919=EDGE_CURVE ( 'NONE', #59239, #62900, #20507, .T. ) ;
#15920=DIRECTION ( 'NONE',  ( -1.000000000000000000, -0.000000000000000000, 0.000000000000000000 ) ) ;
#15921=ORIENTED_EDGE ( 'NONE', *, *, #4328, .T. ) ;
#15922=CARTESIAN_POINT ( 'NONE',  ( -35.00000000000000000, -11.07407352312210058, -3.916263239775468197 ) ) ;
#15923=ORIENTED_EDGE ( 'NONE', *, *, #62272, .T. ) ;
#15924=ORIENTED_EDGE ( 'NONE', *, *, #41815, .T. ) ;
#15925=ORIENTED_EDGE ( 'NONE', *, *, #51005, .T. ) ;
#15928=AXIS2_PLACEMENT_3D ( 'NONE', #16320, #41904, #15328 ) ;
#15933=DIRECTION ( 'NONE',  ( 0.000000000000000000, -0.5767582926625031137, -0.8169148498130233138 ) ) ;
#15935=DIRECTION ( 'NONE',  ( 1.000000000000000000, 0.000000000000000000, 0.000000000000000000 ) ) ;
#15942=AXIS2_PLACEMENT_3D ( 'NONE', #32829, #52810, #7931 ) ;
#15943=ADVANCED_FACE ( 'NONE', ( #4789 ), #60613, .T. ) ;
#15944=VERTEX_POINT ( 'NONE', #26346 ) ;
#15945=DIRECTION ( 'NONE',  ( -1.000000000000000000, 0.000000000000000000, 0.000000000000000000 ) ) ;
#15947=CARTESIAN_POINT ( 'NONE',  ( 36.00000000000000711, 2.250029553613756228, -12.54989509947652060 ) ) ;
#15948=DIRECTION ( 'NONE',  ( 1.000000000000000000, 0.000000000000000000, 0.000000000000000000 ) ) ;
#15952=VERTEX_POINT ( 'NONE', #15695 ) ;
#15953=ADVANCED_FACE ( 'NONE', ( #1746 ), #41300, .T. ) ;
#15954=CARTESIAN_POINT ( 'NONE',  ( 37.00000000000000711, 4.705694406421931860E-17, -3.469127814946512892E-15 ) ) ;
#15956=VECTOR ( 'NONE', #2043, 1000.000000000000000 ) ;
#15958=CARTESIAN_POINT ( 'NONE',  ( 24.73714956085536798, -10.89644250736724729, -7.972329006067469415 ) ) ;
#15959=EDGE_CURVE ( 'NONE', #19892, #64485, #61583, .T. ) ;
#15960=AXIS2_PLACEMENT_3D ( 'NONE', #579, #15830, #44792 ) ;
#15962=CARTESIAN_POINT ( 'NONE',  ( -36.00000000000000711, -12.74613886779085270, 0.3137578094508789439 ) ) ;
#15964=EDGE_CURVE ( 'NONE', #48363, #15014, #57271, .T. ) ;
#15965=CYLINDRICAL_SURFACE ( 'NONE', #64932, 4.999999999999999112 ) ;
#15966=DIRECTION ( 'NONE',  ( 1.000000000000000000, 0.000000000000000000, -0.000000000000000000 ) ) ;
#15967=CARTESIAN_POINT ( 'NONE',  ( 25.05309951391468459, 10.77522019223767558, -8.132934882857098202 ) ) ;
#15969=AXIS2_PLACEMENT_3D ( 'NONE', #4038, #10004, #40583 ) ;
#15970=CIRCLE ( 'NONE', #36140, 4.999999999999999112 ) ;
#15971=ORIENTED_EDGE ( 'NONE', *, *, #46835, .F. ) ;
#15972=VERTEX_POINT ( 'NONE', #1086 ) ;
#15976=EDGE_CURVE ( 'NONE', #62523, #9962, #43623, .T. ) ;
#15978=EDGE_LOOP ( 'NONE', ( #49108, #53262, #3666, #20346 ) ) ;
#15979=EDGE_CURVE ( 'NONE', #56247, #36611, #54509, .T. ) ;
#15982=DIRECTION ( 'NONE',  ( 0.000000000000000000, 0.07632122047555796318, -0.9970832820307042876 ) ) ;
#15984=AXIS2_PLACEMENT_3D ( 'NONE', #63935, #54644, #29652 ) ;
#15985=CIRCLE ( 'NONE', #42556, 5.000000000000000000 ) ;
#15986=DIRECTION ( 'NONE',  ( -1.000000000000000000, 0.000000000000000000, 0.000000000000000000 ) ) ;
#15987=VERTEX_POINT ( 'NONE', #6403 ) ;
#15988=EDGE_CURVE ( 'NONE', #9912, #58567, #19476, .T. ) ;
#15990=AXIS2_PLACEMENT_3D ( 'NONE', #6517, #17801, #32422 ) ;
#15992=CARTESIAN_POINT ( 'NONE',  ( -35.00000000000000000, 8.573591947375437172, -8.029056188533592930 ) ) ;
#15993=VERTEX_POINT ( 'NONE', #36966 ) ;
#15998=CIRCLE ( 'NONE', #30850, 5.000000000000001776 ) ;
#15999=EDGE_CURVE ( 'NONE', #22166, #32661, #52297, .T. ) ;
#16001=ORIENTED_EDGE ( 'NONE', *, *, #51277, .F. ) ;
#16002=CARTESIAN_POINT ( 'NONE',  ( 37.00000000000000711, 3.093009498343925134, -11.78745411414841016 ) ) ;
#16003=CIRCLE ( 'NONE', #10689, 12.74999999999999822 ) ;
#16005=FACE_OUTER_BOUND ( 'NONE', #5395, .T. ) ;
#16006=CARTESIAN_POINT ( 'NONE',  ( -18.58686583997218378, 5.151216734910788908, -10.83812558286602012 ) ) ;
#16007=LINE ( 'NONE', #48198, #16377 ) ;
#16009=CARTESIAN_POINT ( 'NONE',  ( -37.00000000000000711, -2.968224442958319553, -11.81949347079750368 ) ) ;
#16010=CARTESIAN_POINT ( 'NONE',  ( 8.437200413559441614, 4.217676196305609970, 11.23783527720358855 ) ) ;
#16013=DIRECTION ( 'NONE',  ( 1.000000000000000000, -0.000000000000000000, 0.000000000000000000 ) ) ;
#16014=ORIENTED_EDGE ( 'NONE', *, *, #56000, .F. ) ;
#16022=DIRECTION ( 'NONE',  ( 0.000000000000000000, 0.01356324068817992175, -0.9999080150203990547 ) ) ;
#16023=CARTESIAN_POINT ( 'NONE',  ( -47.00000000000000711, 0.000000000000000000, 0.000000000000000000 ) ) ;
#16024=CIRCLE ( 'NONE', #22390, 12.75000000000000178 ) ;
#16025=ADVANCED_FACE ( 'NONE', ( #25699 ), #45988, .T. ) ;
#16026=AXIS2_PLACEMENT_3D ( 'NONE', #27256, #6983, #12599 ) ;
#16027=AXIS2_PLACEMENT_3D ( 'NONE', #61449, #20589, #30541 ) ;
#16028=ORIENTED_EDGE ( 'NONE', *, *, #13925, .F. ) ;
#16029=CARTESIAN_POINT ( 'NONE',  ( -17.57581661391215988, -5.612678105267818296, -10.60769512666424674 ) ) ;
#16030=ORIENTED_EDGE ( 'NONE', *, *, #52189, .T. ) ;
#16031=CARTESIAN_POINT ( 'NONE',  ( 9.687175622948608122, -13.48729812737142986, -0.5854820436212360146 ) ) ;
#16032=CARTESIAN_POINT ( 'NONE',  ( 35.00000000000000000, 4.705694406421931860E-17, -3.469127814946512892E-15 ) ) ;
#16033=DIRECTION ( 'NONE',  ( -1.000000000000000000, 0.000000000000000000, 0.000000000000000000 ) ) ;
#16035=EDGE_CURVE ( 'NONE', #15413, #40664, #24788, .T. ) ;
#16039=B_SPLINE_CURVE_WITH_KNOTS ( 'NONE', 3,
 ( #11907, #36183, #51529, #41175, #11583, #6619, #25567, #56489, #16253, #960, #16589, #5643, #36536, #21583, #45862, #32183, #56843, #26233, #11267, #26888, #61151, #317, #46508, #31852 ),
 .UNSPECIFIED., .F., .F.,
 ( 4, 2, 2, 2, 2, 2, 2, 2, 2, 2, 2, 4 ),
 ( 3.529906531158615134E-18, 0.001336163118173039517, 0.002004244677259556240, 0.002672326236346072963, 0.004008489354519103806, 0.004676570913605619662, 0.005344652472692135517, 0.006012734031778651372, 0.006680815590865167228, 0.008016978709038195469, 0.009353141827211225445, 0.01068930494538425542 ),
 .UNSPECIFIED. ) ;
#16040=AXIS2_PLACEMENT_3D ( 'NONE', #12283, #16311, #11315 ) ;
#16041=AXIS2_PLACEMENT_3D ( 'NONE', #61987, #31701, #53975 ) ;
#16043=DIRECTION ( 'NONE',  ( 1.000000000000000000, 0.000000000000000000, 0.000000000000000000 ) ) ;
#16045=CARTESIAN_POINT ( 'NONE',  ( 37.00000000000000711, 4.824807283154291859, 11.80185301892974969 ) ) ;
#16046=CARTESIAN_POINT ( 'NONE',  ( 8.814021188620074554, 6.315961215693210562, 11.93714002953281117 ) ) ;
#16047=EDGE_CURVE ( 'NONE', #26236, #35632, #17697, .T. ) ;
#16048=CARTESIAN_POINT ( 'NONE',  ( 37.00000000000000711, 7.376655759824882530, -9.700295462048689643 ) ) ;
#16049=CYLINDRICAL_SURFACE ( 'NONE', #50569, 12.75000000000000178 ) ;
#16050=DIRECTION ( 'NONE',  ( -1.000000000000000000, 0.000000000000000000, 0.000000000000000000 ) ) ;
#16051=AXIS2_PLACEMENT_3D ( 'NONE', #33846, #54147, #39163 ) ;
#16054=EDGE_LOOP ( 'NONE', ( #46025, #13528, #58869, #16384, #57937, #13198, #46825, #835, #510, #47934, #25270, #1458, #63700, #19964, #50557, #27527, #14849, #32485, #59226, #17063, #17154, #39911, #42507, #3355, #8481, #45944, #27485, #12245, #35385, #19048, #6000, #10727, #9204, #17771, #18787, #30540, #35451, #29637, #48589, #65571, #8178, #24599, #12410, #48715, #51629, #26549, #17812, #51859, #50854, #18072, #61275, #4435, #23882, #60161, #17106, #44596, #57106, #12340, #48573, #41851, #62253, #63173, #32596, #42823, #30013, #31073, #25947, #12871, #31607, #14259, #47146, #23457, #30570, #3727, #51028, #64811, #45346, #10702, #56514, #53601, #26366, #41780, #13808, #21496, #5013, #51765, #29979, #22238, #64317, #61355, #21737, #50964, #48929, #28511, #28865, #48065, #59055, #47104, #58153, #9269, #58208, #29584, #20249, #29978, #29872, #33260, #52613, #16928, #55192, #29002, #22960, #47588, #5353, #32276, #65181, #51317, #61999, #38329, #61017, #19215, #29627, #31450, #24169, #52395, #33409, #34601, #52083, #54846, #55267, #41114, #10357, #47281, #4503, #10765, #33823, #1454, #60435, #39416, #44190, #52793, #5279, #28430, #26582, #53477, #50381, #33955, #32668, #64529, #61528, #4184, #13069, #2062, #560, #24182, #38894, #25702, #8151, #30248, #15436, #37143, #12373, #61786, #44972, #28081, #30388, #43052, #57176, #61234, #59997, #62952, #47456, #32552, #39329, #19046, #34598, #63123, #40182, #32518, #51359, #42216, #20010, #43483, #42746, #48193, #59873, #11197, #35428, #34031, #51382, #51416, #7398, #9105, #41752, #34767, #33696, #52800, #42170, #20296, #15602, #64247, #20415, #56013, #54165, #54623, #63708, #53697, #40890, #40378, #29720, #13135, #11136, #28606, #27175, #27250, #43408, #60317, #32877, #28192, #34633, #7712, #39671, #28972, #54799, #41917, #36625, #36868, #29191, #36686, #1596, #47613, #19553, #63390, #56886, #59707, #53236, #15571, #15917, #17894, #34010, #30693, #64249, #17188, #2089, #21847, #54883, #39091, #8670, #41042, #50538, #28305, #57177, #1077, #33627, #58037, #33577, #15903, #23542, #25808, #42474, #31914, #62883, #38285, #3900, #19620, #48149, #56227, #4342, #51492, #2211, #35960, #2562, #56071, #49083, #19907, #6801, #63499, #13366, #51450, #12258, #26713, #27602, #40882, #53642, #1048, #35619, #18657, #34747, #36559, #6957, #52286, #43743, #49904, #34051, #61951, #20844, #58550, #59218, #2710, #23186, #57319, #43317, #43593, #8579, #30689, #24906, #388, #36004, #20857, #32585, #41424, #17433, #8818, #32092, #4530, #35483, #32643, #12391, #23531, #2193, #62388, #49498, #34047, #56026, #56395, #26389, #62491, #51929, #11718, #23255, #15232, #6290, #15040, #40694, #1168, #9704, #65552, #62293, #28205, #38080, #38350, #39305, #4828, #29488, #23727, #1535, #24583, #25559, #6006, #48210, #29612, #60684, #28544, #30071, #54313, #38395, #56390, #40247, #5147, #10690, #45324, #22236, #60207, #16549, #20612, #36144, #44889, #28755, #17586, #39064, #2724, #2852, #21748, #22483, #11518, #32258, #59525, #59399, #54591, #31081, #20556, #3445, #38901, #11763, #63200, #37858, #17935, #48833, #52925, #1270, #20086, #308, #33278, #32617, #5691, #61915, #37974, #59200, #19756, #45752, #62728, #45977, #8338, #64725, #37917, #33994 ) ) ;
#16055=CARTESIAN_POINT ( 'NONE',  ( -35.00000000000000000, -8.258652103341496797, 8.352657516904644197 ) ) ;
#16058=ORIENTED_EDGE ( 'NONE', *, *, #19786, .F. ) ;
#16060=DIRECTION ( 'NONE',  ( 0.000000000000000000, 0.01356324068817998940, -0.9999080150203990547 ) ) ;
#16061=CARTESIAN_POINT ( 'NONE',  ( 8.981012069803050224, 5.156238751367448359, -10.84194425323662436 ) ) ;
#16062=ORIENTED_EDGE ( 'NONE', *, *, #46056, .F. ) ;
#16065=CARTESIAN_POINT ( 'NONE',  ( -35.00000000000000000, -8.146229107149334681, -9.063649021439044162 ) ) ;
#16066=VERTEX_POINT ( 'NONE', #57939 ) ;
#16069=ORIENTED_EDGE ( 'NONE', *, *, #15138, .F. ) ;
#16070=EDGE_CURVE ( 'NONE', #19449, #55094, #2494, .T. ) ;
#16071=AXIS2_PLACEMENT_3D ( 'NONE', #57145, #51516, #55828 ) ;
#16072=CARTESIAN_POINT ( 'NONE',  ( -35.00000000000000000, 2.627174906296914525, 11.44858830469741129 ) ) ;
#16073=AXIS2_PLACEMENT_3D ( 'NONE', #30118, #35076, #62021 ) ;
#16074=AXIS2_PLACEMENT_3D ( 'NONE', #47165, #62113, #11241 ) ;
#16075=ORIENTED_EDGE ( 'NONE', *, *, #3641, .F. ) ;
#16079=LINE ( 'NONE', #55992, #49262 ) ;
#16080=DIRECTION ( 'NONE',  ( 0.000000000000000000, -0.01356324068817998940, 0.9999080150203990547 ) ) ;
#16081=ORIENTED_EDGE ( 'NONE', *, *, #17325, .T. ) ;
#16084=CARTESIAN_POINT ( 'NONE',  ( -17.62527007572664317, 11.56525963221033138, 3.218409487716447082 ) ) ;
#16086=VERTEX_POINT ( 'NONE', #28317 ) ;
#16089=VERTEX_POINT ( 'NONE', #27320 ) ;
#16090=CARTESIAN_POINT ( 'NONE',  ( 37.00000000000000711, 4.705694406421931860E-17, -3.469127814946512892E-15 ) ) ;
#16092=ORIENTED_EDGE ( 'NONE', *, *, #13852, .F. ) ;
#16093=DIRECTION ( 'NONE',  ( -1.000000000000000000, 0.000000000000000000, 0.000000000000000000 ) ) ;
#16095=CARTESIAN_POINT ( 'NONE',  ( -35.00000000000000000, 0.000000000000000000, 0.000000000000000000 ) ) ;
#16096=CARTESIAN_POINT ( 'NONE',  ( 35.00000000000000000, 8.534258022646096009, -8.699265615723016154 ) ) ;
#16097=AXIS2_PLACEMENT_3D ( 'NONE', #11710, #36669, #31993 ) ;
#16099=DIRECTION ( 'NONE',  ( 1.000000000000000000, -0.000000000000000000, 0.000000000000000000 ) ) ;
#16101=CARTESIAN_POINT ( 'NONE',  ( -21.17861794710831091, 11.44571409049744304, -3.604945070120774808 ) ) ;
#16102=CARTESIAN_POINT ( 'NONE',  ( -18.10941110424454337, -9.537088721069784114, -9.555689318548479250 ) ) ;
#16103=CIRCLE ( 'NONE', #24600, 12.18650000000000055 ) ;
#16105=( BOUNDED_CURVE ( )  B_SPLINE_CURVE ( 3, ( #5190, #29156, #4549, #44411 ),
 .UNSPECIFIED., .F., .F. ) 
 B_SPLINE_CURVE_WITH_KNOTS ( ( 4, 4 ),
 ( 1.948709165869125792, 1.984325536053276551 ),
 .UNSPECIFIED. ) 
 CURVE ( )  GEOMETRIC_REPRESENTATION_ITEM ( )  RATIONAL_B_SPLINE_CURVE ( ( 1.000000000000000000, 0.9998942923082225764, 0.9998942923082225764, 1.000000000000000000 ) ) 
 REPRESENTATION_ITEM ( '' )  );
#16106=ORIENTED_EDGE ( 'NONE', *, *, #47364, .F. ) ;
#16107=CARTESIAN_POINT ( 'NONE',  ( 37.00000000000000711, 9.040300684349800164, 7.499679039483956977 ) ) ;
#16109=AXIS2_PLACEMENT_3D ( 'NONE', #4829, #35034, #151 ) ;
#16110=ORIENTED_EDGE ( 'NONE', *, *, #43223, .F. ) ;
#16111=AXIS2_PLACEMENT_3D ( 'NONE', #22411, #11769, #57686 ) ;
#16112=DIRECTION ( 'NONE',  ( 0.000000000000000000, 0.01356324068817991828, -0.9999080150203990547 ) ) ;
#16115=CARTESIAN_POINT ( 'NONE',  ( -21.17861794710831091, 11.44571409049744304, -3.604945070120774808 ) ) ;
#16116=CARTESIAN_POINT ( 'NONE',  ( -35.00000000000000000, 0.000000000000000000, 0.000000000000000000 ) ) ;
#16117=CARTESIAN_POINT ( 'NONE',  ( -4.989057617119011745, -0.9162120371760335003, -11.96497202265568660 ) ) ;
#16119=VECTOR ( 'NONE', #4445, 1000.000000000000000 ) ;
#16120=EDGE_CURVE ( 'NONE', #52686, #38454, #35344, .T. ) ;
#16122=ORIENTED_EDGE ( 'NONE', *, *, #46727, .T. ) ;
#16125=DIRECTION ( 'NONE',  ( 1.000000000000000000, 0.000000000000000000, -0.000000000000000000 ) ) ;
#16126=AXIS2_PLACEMENT_3D ( 'NONE', #50443, #49141, #13525 ) ;
#16127=VECTOR ( 'NONE', #60855, 1000.000000000000000 ) ;
#16128=DIRECTION ( 'NONE',  ( 1.000000000000000000, 0.000000000000000000, 0.000000000000000000 ) ) ;
#16129=CIRCLE ( 'NONE', #53309, 5.000000000000000000 ) ;
#16133=CARTESIAN_POINT ( 'NONE',  ( 3.878878013157130766, 5.423588667954382103, -10.70679124709716135 ) ) ;
#16135=EDGE_CURVE ( 'NONE', #52529, #2297, #37492, .T. ) ;
#16136=EDGE_CURVE ( 'NONE', #47803, #62620, #39627, .T. ) ;
#16137=ORIENTED_EDGE ( 'NONE', *, *, #12212, .F. ) ;
#16138=CARTESIAN_POINT ( 'NONE',  ( -35.00000000000000000, -12.57916205664479925, -2.080187960898692623 ) ) ;
#16139=CARTESIAN_POINT ( 'NONE',  ( -25.74864769002726561, 4.845157721295412223, 10.98320407977279345 ) ) ;
#16140=FACE_OUTER_BOUND ( 'NONE', #51181, .T. ) ;
#16142=VECTOR ( 'NONE', #18940, 1000.000000000000000 ) ;
#16143=EDGE_CURVE ( 'NONE', #19699, #57845, #53267, .T. ) ;
#16145=CIRCLE ( 'NONE', #4491, 5.000000000000000888 ) ;
#16146=CARTESIAN_POINT ( 'NONE',  ( 10.88715743210410203, 1.032614531350164011, -13.46093288850865655 ) ) ;
#16147=FACE_OUTER_BOUND ( 'NONE', #31162, .T. ) ;
#16150=LINE ( 'NONE', #10829, #385 ) ;
#16151=VECTOR ( 'NONE', #15016, 1000.000000000000000 ) ;
#16154=CARTESIAN_POINT ( 'NONE',  ( -35.00000000000000000, -10.64792938439751246, -5.927257550915431494 ) ) ;
#16156=CYLINDRICAL_SURFACE ( 'NONE', #58408, 12.18649999999999878 ) ;
#16157=ORIENTED_EDGE ( 'NONE', *, *, #16605, .F. ) ;
#16159=ADVANCED_FACE ( 'NONE', ( #47951 ), #63541, .T. ) ;
#16162=CIRCLE ( 'NONE', #38470, 5.000000000000001776 ) ;
#16163=DIRECTION ( 'NONE',  ( 0.000000000000000000, 0.9999080150203989437, 0.01356324068818348313 ) ) ;
#16164=CARTESIAN_POINT ( 'NONE',  ( 24.35223141888314302, -1.455662175893269961, -11.91666582609157210 ) ) ;
#16166=LINE ( 'NONE', #63024, #6602 ) ;
#16167=PLANE ( 'NONE',  #2655 ) ;
#16169=ORIENTED_EDGE ( 'NONE', *, *, #5209, .T. ) ;
#16171=CARTESIAN_POINT ( 'NONE',  ( 24.17474130245189912, -3.383288635110214937, -11.51882187244559930 ) ) ;
#16173=AXIS2_PLACEMENT_3D ( 'NONE', #24176, #8237, #13228 ) ;
#16175=DIRECTION ( 'NONE',  ( -1.000000000000000000, 0.000000000000000000, 0.000000000000000000 ) ) ;
#16176=EDGE_CURVE ( 'NONE', #33730, #26919, #60862, .T. ) ;
#16177=CIRCLE ( 'NONE', #54453, 5.000000000000002665 ) ;
#16178=CARTESIAN_POINT ( 'NONE',  ( -17.32414925028539443, 3.214166590961689440, 11.56290286403455880 ) ) ;
#16179=CIRCLE ( 'NONE', #58693, 12.75000000000000178 ) ;
#16182=ORIENTED_EDGE ( 'NONE', *, *, #21254, .T. ) ;
#16185=DIRECTION ( 'NONE',  ( 1.000000000000000000, 0.000000000000000000, 0.000000000000000000 ) ) ;
#16188=DIRECTION ( 'NONE',  ( -0.000000000000000000, -0.000000000000000000, -1.000000000000000000 ) ) ;
#16189=B_SPLINE_CURVE_WITH_KNOTS ( 'NONE', 3,
 ( #48701, #12434, #42694, #49041, #64304, #23092, #27412, #2152, #53696, #52707, #47708, #48046, #8452, #18770, #22779, #62995, #13114, #17455 ),
 .UNSPECIFIED., .F., .F.,
 ( 4, 2, 2, 2, 2, 2, 2, 2, 4 ),
 ( 0.004456855160748429343, 0.005198565759172233368, 0.005940276357596038261, 0.006681986956019843153, 0.007423697554443648046, 0.008165408152867453806, 0.008907118751291256964, 0.009648829349715063591, 0.01039053994813886848 ),
 .UNSPECIFIED. ) ;
#16190=EDGE_LOOP ( 'NONE', ( #65694, #45778, #17495, #25366 ) ) ;
#16191=CARTESIAN_POINT ( 'NONE',  ( -47.00000000000000711, 0.000000000000000000, 0.000000000000000000 ) ) ;
#16192=CARTESIAN_POINT ( 'NONE',  ( 35.00000000000000000, -8.389074212634222150, 8.839356091080130540 ) ) ;
#16193=AXIS2_PLACEMENT_3D ( 'NONE', #7244, #16905, #32187 ) ;
#16198=DIRECTION ( 'NONE',  ( -1.000000000000000000, 0.000000000000000000, 0.000000000000000000 ) ) ;
#16201=VECTOR ( 'NONE', #52891, 1000.000000000000000 ) ;
#16202=DIRECTION ( 'NONE',  ( -1.000000000000000000, 0.000000000000000000, 0.000000000000000000 ) ) ;
#16203=CIRCLE ( 'NONE', #37407, 5.000000000000001776 ) ;
#16206=DIRECTION ( 'NONE',  ( 0.000000000000000000, 0.01356324068817998940, -0.9999080150203989437 ) ) ;
#16207=CYLINDRICAL_SURFACE ( 'NONE', #41376, 4.999999999999999112 ) ;
#16210=VERTEX_POINT ( 'NONE', #4365 ) ;
#16211=ORIENTED_EDGE ( 'NONE', *, *, #46413, .T. ) ;
#16213=CARTESIAN_POINT ( 'NONE',  ( -37.00000000000000711, -4.983891302653500333, -11.73555825188281787 ) ) ;
#16214=AXIS2_PLACEMENT_3D ( 'NONE', #10766, #60657, #15095 ) ;
#16215=ORIENTED_EDGE ( 'NONE', *, *, #41243, .F. ) ;
#16220=EDGE_CURVE ( 'NONE', #17445, #14898, #24300, .T. ) ;
#16222=ORIENTED_EDGE ( 'NONE', *, *, #5438, .T. ) ;
#16224=DIRECTION ( 'NONE',  ( -0.9746931518056332067, -0.2235469969004301727, 0.000000000000000000 ) ) ;
#16225=FACE_OUTER_BOUND ( 'NONE', #51191, .T. ) ;
#16229=AXIS2_PLACEMENT_3D ( 'NONE', #39953, #28664, #43625 ) ;
#16232=ORIENTED_EDGE ( 'NONE', *, *, #17590, .T. ) ;
#16233=CARTESIAN_POINT ( 'NONE',  ( -35.00000000000000000, 4.237620530777800987, 11.42599468261430928 ) ) ;
#16235=DIRECTION ( 'NONE',  ( 1.000000000000000000, 0.000000000000000000, 0.000000000000000000 ) ) ;
#16236=DIRECTION ( 'NONE',  ( -1.000000000000000000, -0.000000000000000000, 0.000000000000000000 ) ) ;
#16237=DIRECTION ( 'NONE',  ( 1.000000000000000000, 0.000000000000000000, 0.000000000000000000 ) ) ;
#16239=CARTESIAN_POINT ( 'NONE',  ( 29.10306999346632040, -8.924211771781015656, 8.035139106930564878 ) ) ;
#16240=CARTESIAN_POINT ( 'NONE',  ( -9.953223611451470276, -4.237682741712822221, 11.22833300639604204 ) ) ;
#16241=CIRCLE ( 'NONE', #36413, 12.74999999999999822 ) ;
#16244=CARTESIAN_POINT ( 'NONE',  ( -37.00000000000000711, -5.143145423404365424, 11.66664283989678275 ) ) ;
#16246=DIRECTION ( 'NONE',  ( 1.000000000000000000, 0.000000000000000000, 0.000000000000000000 ) ) ;
#16247=DIRECTION ( 'NONE',  ( 1.000000000000000000, -0.000000000000000000, 0.000000000000000000 ) ) ;
#16248=DIRECTION ( 'NONE',  ( -1.000000000000000000, 0.000000000000000000, 0.000000000000000000 ) ) ;
#16249=DIRECTION ( 'NONE',  ( -0.000000000000000000, -0.000000000000000000, -1.000000000000000000 ) ) ;
#16250=CARTESIAN_POINT ( 'NONE',  ( 35.00000000000000000, 4.705694406421931860E-17, -3.469127814946512892E-15 ) ) ;
#16251=VECTOR ( 'NONE', #21691, 1000.000000000000000 ) ;
#16253=CARTESIAN_POINT ( 'NONE',  ( -8.371944397756363898, -1.942763698273609840, 11.84475809039481931 ) ) ;
#16255=EDGE_CURVE ( 'NONE', #60814, #55613, #56642, .T. ) ;
#16256=DIRECTION ( 'NONE',  ( 0.000000000000000000, 0.01356324068817998940, -0.9999080150203990547 ) ) ;
#16257=ORIENTED_EDGE ( 'NONE', *, *, #28770, .F. ) ;
#16258=DIRECTION ( 'NONE',  ( 1.000000000000000000, 0.000000000000000000, -0.000000000000000000 ) ) ;
#16261=ORIENTED_EDGE ( 'NONE', *, *, #30602, .T. ) ;
#16265=DIRECTION ( 'NONE',  ( 0.000000000000000000, -0.01356324068817998940, 0.9999080150203990547 ) ) ;
#16266=CARTESIAN_POINT ( 'NONE',  ( 36.00000000000000711, -11.59605747147790211, -5.300372733891606458 ) ) ;
#16268=ORIENTED_EDGE ( 'NONE', *, *, #15959, .F. ) ;
#16270=DIRECTION ( 'NONE',  ( 0.000000000000000000, -0.01356324068817992175, 0.9999080150203990547 ) ) ;
#16271=EDGE_LOOP ( 'NONE', ( #14131, #41389, #6638, #39812 ) ) ;
#16272=DIRECTION ( 'NONE',  ( 0.000000000000000000, 0.01356324068817992175, -0.9999080150203990547 ) ) ;
#16273=ORIENTED_EDGE ( 'NONE', *, *, #468, .T. ) ;
#16276=VERTEX_POINT ( 'NONE', #14961 ) ;
#16277=ORIENTED_EDGE ( 'NONE', *, *, #63203, .F. ) ;
#16278=DIRECTION ( 'NONE',  ( 0.000000000000000000, -0.9105187689795911643, 0.4134677391718608597 ) ) ;
#16280=AXIS2_PLACEMENT_3D ( 'NONE', #59661, #50671, #64618 ) ;
#16281=CIRCLE ( 'NONE', #13102, 12.18649999999999878 ) ;
#16283=CARTESIAN_POINT ( 'NONE',  ( -37.00000000000000711, 6.475373545682302279, 10.32377448871670467 ) ) ;
#16284=DIRECTION ( 'NONE',  ( 1.000000000000000000, 0.000000000000000000, 0.000000000000000000 ) ) ;
#16286=VERTEX_POINT ( 'NONE', #51240 ) ;
#16288=ADVANCED_FACE ( 'NONE', ( #10985 ), #31268, .T. ) ;
#16289=VERTEX_POINT ( 'NONE', #10631 ) ;
#16290=CARTESIAN_POINT ( 'NONE',  ( 35.00000000000000000, -2.544412758415763864, 11.91791701451268715 ) ) ;
#16291=EDGE_CURVE ( 'NONE', #42846, #46638, #61197, .T. ) ;
#16292=AXIS2_PLACEMENT_3D ( 'NONE', #62898, #37641, #32619 ) ;
#16293=DIRECTION ( 'NONE',  ( -1.000000000000000000, -1.836970198721029688E-16, -0.000000000000000000 ) ) ;
#16294=EDGE_CURVE ( 'NONE', #56356, #44514, #32161, .T. ) ;
#16295=DIRECTION ( 'NONE',  ( -1.000000000000000000, 0.000000000000000000, 0.000000000000000000 ) ) ;
#16297=VECTOR ( 'NONE', #32245, 1000.000000000000000 ) ;
#16298=LINE ( 'NONE', #31572, #12147 ) ;
#16300=AXIS2_PLACEMENT_3D ( 'NONE', #58723, #17148, #63022 ) ;
#16305=ORIENTED_EDGE ( 'NONE', *, *, #41600, .F. ) ;
#16311=DIRECTION ( 'NONE',  ( -1.000000000000000000, 0.000000000000000000, 0.000000000000000000 ) ) ;
#16312=FACE_OUTER_BOUND ( 'NONE', #51193, .T. ) ;
#16314=CYLINDRICAL_SURFACE ( 'NONE', #49438, 5.000000000000000888 ) ;
#16317=DIRECTION ( 'NONE',  ( 1.000000000000000000, 0.000000000000000000, 0.000000000000000000 ) ) ;
#16319=EDGE_CURVE ( 'NONE', #21959, #40917, #18449, .T. ) ;
#16320=CARTESIAN_POINT ( 'NONE',  ( -4.806344283790351390, -7.508992741355383416, 25.00000000000000000 ) ) ;
#16322=DIRECTION ( 'NONE',  ( 1.000000000000000000, -0.000000000000000000, -0.000000000000000000 ) ) ;
#16323=CARTESIAN_POINT ( 'NONE',  ( 35.00000000000000000, 9.060822531526046220, -7.474872387601039669 ) ) ;
#16324=LINE ( 'NONE', #41576, #53520 ) ;
#16327=AXIS2_PLACEMENT_3D ( 'NONE', #49649, #44622, #4426 ) ;
#16328=AXIS2_PLACEMENT_3D ( 'NONE', #2921, #17872, #64703 ) ;
#16329=ORIENTED_EDGE ( 'NONE', *, *, #27889, .F. ) ;
#16330=ORIENTED_EDGE ( 'NONE', *, *, #14786, .T. ) ;
#16331=FACE_OUTER_BOUND ( 'NONE', #38706, .T. ) ;
#16332=AXIS2_PLACEMENT_3D ( 'NONE', #27422, #47720, #38051 ) ;
#16335=AXIS2_PLACEMENT_3D ( 'NONE', #56451, #40835, #10896 ) ;
#16336=DIRECTION ( 'NONE',  ( -1.000000000000000000, 0.000000000000000000, 0.000000000000000000 ) ) ;
#16338=CIRCLE ( 'NONE', #44655, 4.999999999999999112 ) ;
#16342=CARTESIAN_POINT ( 'NONE',  ( 35.00000000000000000, 2.905556151562782574, 11.38112321385047210 ) ) ;
#16343=VECTOR ( 'NONE', #53648, 1000.000000000000000 ) ;
#16344=EDGE_CURVE ( 'NONE', #58914, #12785, #25615, .T. ) ;
#16345=CARTESIAN_POINT ( 'NONE',  ( -47.00000000000000711, 0.000000000000000000, 0.000000000000000000 ) ) ;
#16348=CARTESIAN_POINT ( 'NONE',  ( 35.00000000000000000, 4.705694406421931860E-17, -3.469127814946512892E-15 ) ) ;
#16352=CARTESIAN_POINT ( 'NONE',  ( 24.89778902934379090, -0.9306873417793930514, 11.96553346855706934 ) ) ;
#16354=DIRECTION ( 'NONE',  ( -1.000000000000000000, 0.000000000000000000, -0.000000000000000000 ) ) ;
#16357=B_SPLINE_CURVE_WITH_KNOTS ( 'NONE', 3,
 ( #56366, #10160, #51414, #36744, #46397, #16133, #36417, #11154, #51728, #40753, #6174, #51068, #21457, #62022, #16475, #20473, #35737, #57038, #31736, #25453, #25793, #61042 ),
 .UNSPECIFIED., .F., .F.,
 ( 4, 2, 2, 2, 2, 2, 2, 2, 2, 2, 4 ),
 ( 2.453269466693398698E-18, 0.002704593263307899717, 0.003380741579134873345, 0.004056889894961846973, 0.005409186526615791628, 0.006085334842442765256, 0.006761483158269738017, 0.008113779789923683539, 0.008789928105750657167, 0.009466076421577630795, 0.01081837305323157805 ),
 .UNSPECIFIED. ) ;
#16358=CARTESIAN_POINT ( 'NONE',  ( 35.00000000000000000, -9.512294188640847636, 6.891188680298922620 ) ) ;
#16360=FACE_OUTER_BOUND ( 'NONE', #46651, .T. ) ;
#16361=VECTOR ( 'NONE', #61263, 1000.000000000000000 ) ;
#16362=CARTESIAN_POINT ( 'NONE',  ( 145.1370849898475797, 3.309064568108273190E-14, 0.000000000000000000 ) ) ;
#16363=EDGE_CURVE ( 'NONE', #42534, #55068, #53463, .T. ) ;
#16364=CARTESIAN_POINT ( 'NONE',  ( 10.39253138699964474, 0.7544984855469610840, 11.97748485473318780 ) ) ;
#16366=CARTESIAN_POINT ( 'NONE',  ( 8.682549669955445637, 5.989798744006710862, -10.40639624049628686 ) ) ;
#16367=ORIENTED_EDGE ( 'NONE', *, *, #26594, .T. ) ;
#16368=CARTESIAN_POINT ( 'NONE',  ( 36.00000000000000711, -12.26766708251988902, 3.473736367725380081 ) ) ;
#16369=ORIENTED_EDGE ( 'NONE', *, *, #65790, .T. ) ;
#16370=CARTESIAN_POINT ( 'NONE',  ( -36.00000000000000711, 11.47561260193584864, -5.556331110570289944 ) ) ;
#16371=EDGE_CURVE ( 'NONE', #10789, #56661, #1441, .T. ) ;
#16372=CARTESIAN_POINT ( 'NONE',  ( -47.00000000000000711, 0.000000000000000000, 0.000000000000000000 ) ) ;
#16375=ORIENTED_EDGE ( 'NONE', *, *, #25734, .T. ) ;
#16377=VECTOR ( 'NONE', #22235, 1000.000000000000000 ) ;
#16379=FACE_OUTER_BOUND ( 'NONE', #39974, .T. ) ;
#16380=CARTESIAN_POINT ( 'NONE',  ( 9.575800908719084958, -13.45729701195359240, -1.072919909436246266 ) ) ;
#16383=CARTESIAN_POINT ( 'NONE',  ( -19.16689948115911335, -3.912184365920206464, -11.34481683777750582 ) ) ;
#16384=ORIENTED_EDGE ( 'NONE', *, *, #22016, .T. ) ;
#16385=EDGE_CURVE ( 'NONE', #6586, #32962, #15181, .T. ) ;
#16388=DIRECTION ( 'NONE',  ( 0.000000000000000000, -0.01356324068817998940, 0.9999080150203990547 ) ) ;
#16389=EDGE_CURVE ( 'NONE', #44234, #61480, #361, .T. ) ;
#16390=EDGE_LOOP ( 'NONE', ( #14437, #12551, #56325, #30772 ) ) ;
#16391=AXIS2_PLACEMENT_3D ( 'NONE', #14228, #54814, #18264 ) ;
#16392=DIRECTION ( 'NONE',  ( 0.000000000000000000, 0.2960891610144441022, 0.9551603052523500725 ) ) ;
#16393=EDGE_CURVE ( 'NONE', #49368, #63364, #18491, .T. ) ;
#16394=CIRCLE ( 'NONE', #57794, 11.99999999999999822 ) ;
#16395=EDGE_CURVE ( 'NONE', #7895, #31335, #52419, .T. ) ;
#16396=CARTESIAN_POINT ( 'NONE',  ( 24.97568612634365337, -8.683198485571610448, -8.285225425757140272 ) ) ;
#16398=VECTOR ( 'NONE', #42984, 1000.000000000000000 ) ;
#16404=CARTESIAN_POINT ( 'NONE',  ( 35.00000000000000000, 9.076753354953996933, -8.954052073409636492 ) ) ;
#16405=AXIS2_PLACEMENT_3D ( 'NONE', #48134, #57785, #22859 ) ;
#16406=AXIS2_PLACEMENT_3D ( 'NONE', #24545, #54161, #60780 ) ;
#16407=VERTEX_POINT ( 'NONE', #61843 ) ;
#16408=DIRECTION ( 'NONE',  ( 1.000000000000000000, 0.000000000000000000, 0.000000000000000000 ) ) ;
#16413=CARTESIAN_POINT ( 'NONE',  ( 37.00000000000000711, -12.05416472667166694, -1.791059740004382839 ) ) ;
#16417=CIRCLE ( 'NONE', #23834, 12.75000000000000178 ) ;
#16420=ORIENTED_EDGE ( 'NONE', *, *, #24628, .F. ) ;
#16422=CARTESIAN_POINT ( 'NONE',  ( -2.952869152607111136, -7.581333670610126418, 11.17020052527586138 ) ) ;
#16425=DIRECTION ( 'NONE',  ( 0.000000000000000000, -0.01356324068817998940, 0.9999080150203990547 ) ) ;
#16427=FACE_OUTER_BOUND ( 'NONE', #46693, .T. ) ;
#16428=FACE_OUTER_BOUND ( 'NONE', #20333, .T. ) ;
#16429=VERTEX_POINT ( 'NONE', #42868 ) ;
#16430=AXIS2_PLACEMENT_3D ( 'NONE', #36061, #56722, #22097 ) ;
#16433=LINE ( 'NONE', #36700, #14333 ) ;
#16434=DIRECTION ( 'NONE',  ( 0.000000000000000000, 0.01356324068817998940, -0.9999080150203990547 ) ) ;
#16435=ORIENTED_EDGE ( 'NONE', *, *, #12359, .T. ) ;
#16436=CARTESIAN_POINT ( 'NONE',  ( -27.67932024734484031, 8.922843848540177092, -8.046304320001306465 ) ) ;
#16437=EDGE_LOOP ( 'NONE', ( #9362, #6640, #6469, #63738 ) ) ;
#16439=EDGE_CURVE ( 'NONE', #21988, #45204, #22937, .T. ) ;
#16441=CARTESIAN_POINT ( 'NONE',  ( 22.83619264212346067, -9.759093346436447547, -6.990946369225183865 ) ) ;
#16443=CIRCLE ( 'NONE', #8979, 12.18649999999999700 ) ;
#16445=ORIENTED_EDGE ( 'NONE', *, *, #10221, .F. ) ;
#16446=CARTESIAN_POINT ( 'NONE',  ( 35.00000000000000000, -1.591260454995155671, 12.08216339958901742 ) ) ;
#16447=EDGE_CURVE ( 'NONE', #29014, #10001, #43911, .T. ) ;
#16451=ORIENTED_EDGE ( 'NONE', *, *, #35872, .F. ) ;
#16453=VERTEX_POINT ( 'NONE', #22605 ) ;
#16454=EDGE_CURVE ( 'NONE', #12453, #2190, #23756, .T. ) ;
#16455=VERTEX_POINT ( 'NONE', #27252 ) ;
#16457=DIRECTION ( 'NONE',  ( 1.000000000000000000, 0.000000000000000000, 0.000000000000000000 ) ) ;
#16458=DIRECTION ( 'NONE',  ( 0.000000000000000000, -0.8169148498130212044, 0.5767582926625058892 ) ) ;
#16461=DIRECTION ( 'NONE',  ( 1.000000000000000000, -0.000000000000000000, 0.000000000000000000 ) ) ;
#16462=CARTESIAN_POINT ( 'NONE',  ( -10.00003325919894692, -3.438199368958688940, -11.49838662738022954 ) ) ;
#16463=AXIS2_PLACEMENT_3D ( 'NONE', #35334, #64939, #5773 ) ;
#16464=CARTESIAN_POINT ( 'NONE',  ( 22.78397477906666779, 3.290341966830230724, -11.54089583822152854 ) ) ;
#16465=EDGE_LOOP ( 'NONE', ( #14731, #41086, #12604, #4831 ) ) ;
#16467=AXIS2_PLACEMENT_3D ( 'NONE', #8086, #9053, #3106 ) ;
#16469=EDGE_CURVE ( 'NONE', #23887, #18752, #64074, .T. ) ;
#16472=EDGE_CURVE ( 'NONE', #65189, #14785, #35398, .T. ) ;
#16475=CARTESIAN_POINT ( 'NONE',  ( 2.510731577322978136, 1.829398357709037803, -11.86532612209469484 ) ) ;
#16477=CARTESIAN_POINT ( 'NONE',  ( 47.00000000000000711, 4.705694406421931860E-17, -3.469127814946512892E-15 ) ) ;
#16479=DIRECTION ( 'NONE',  ( 0.000000000000000000, -1.000000000000000000, 0.000000000000000000 ) ) ;
#16480=DIRECTION ( 'NONE',  ( 0.000000000000000000, 0.7617968321374856133, 0.6478160128811973895 ) ) ;
#16481=DIRECTION ( 'NONE',  ( 0.000000000000000000, -0.01356324068818000328, 0.9999080150203990547 ) ) ;
#16483=VECTOR ( 'NONE', #19380, 1000.000000000000000 ) ;
#16484=CARTESIAN_POINT ( 'NONE',  ( 9.274649623867711412, 2.850288540387552416, -13.19772255816346807 ) ) ;
#16485=CARTESIAN_POINT ( 'NONE',  ( -24.85888762414873909, -9.907586878531645880, 9.176240764607326739 ) ) ;
#16486=ORIENTED_EDGE ( 'NONE', *, *, #21713, .T. ) ;
#16488=DIRECTION ( 'NONE',  ( 1.000000000000000000, -0.000000000000000000, 0.000000000000000000 ) ) ;
#16490=EDGE_LOOP ( 'NONE', ( #13599, #62362 ) ) ;
#16493=DIRECTION ( 'NONE',  ( 1.000000000000000000, 0.000000000000000000, 0.000000000000000000 ) ) ;
#16495=EDGE_LOOP ( 'NONE', ( #45308, #7323, #7010, #62154 ) ) ;
#16497=CIRCLE ( 'NONE', #2764, 5.000000000000000888 ) ;
#16500=ORIENTED_EDGE ( 'NONE', *, *, #16527, .T. ) ;
#16503=CARTESIAN_POINT ( 'NONE',  ( 35.00000000000000000, 6.753013023069713405, -10.14433819232436917 ) ) ;
#16504=( BOUNDED_CURVE ( )  B_SPLINE_CURVE ( 3, ( #23397, #45314, #56265, #34982 ),
 .UNSPECIFIED., .F., .F. ) 
 B_SPLINE_CURVE_WITH_KNOTS ( ( 4, 4 ),
 ( 0.7743326424653215190, 0.8261054116032431338 ),
 .UNSPECIFIED. ) 
 CURVE ( )  GEOMETRIC_REPRESENTATION_ITEM ( )  RATIONAL_B_SPLINE_CURVE ( ( 1.000000000000000000, 0.9997766441710536078, 0.9997766441710536078, 1.000000000000000000 ) ) 
 REPRESENTATION_ITEM ( '' )  );
#16507=FACE_OUTER_BOUND ( 'NONE', #498, .T. ) ;
#16508=DIRECTION ( 'NONE',  ( 1.000000000000000000, 0.000000000000000000, 0.000000000000000000 ) ) ;
#16509=DIRECTION ( 'NONE',  ( 0.000000000000000000, -0.01356324068817991828, 0.9999080150203990547 ) ) ;
#16510=EDGE_LOOP ( 'NONE', ( #36195, #61872, #31467, #20115 ) ) ;
#16511=ORIENTED_EDGE ( 'NONE', *, *, #50149, .F. ) ;
#16512=DIRECTION ( 'NONE',  ( 1.000000000000000000, 0.000000000000000000, 0.000000000000000000 ) ) ;
#16513=ORIENTED_EDGE ( 'NONE', *, *, #8361, .T. ) ;
#16514=ADVANCED_FACE ( 'NONE', ( #32543 ), #53533, .T. ) ;
#16521=AXIS2_PLACEMENT_3D ( 'NONE', #13590, #28901, #34203 ) ;
#16522=CARTESIAN_POINT ( 'NONE',  ( 37.00000000000000711, -9.677500615117850202, 6.657191900728419043 ) ) ;
#16523=FACE_BOUND ( 'NONE', #27943, .T. ) ;
#16524=ORIENTED_EDGE ( 'NONE', *, *, #23685, .T. ) ;
#16527=EDGE_CURVE ( 'NONE', #39221, #27370, #49253, .T. ) ;
#16530=DIRECTION ( 'NONE',  ( 1.000000000000000000, 0.000000000000000000, 0.000000000000000000 ) ) ;
#16531=CARTESIAN_POINT ( 'NONE',  ( -35.00000000000000000, 3.287724142101577485, -11.73463472867572932 ) ) ;
#16532=CARTESIAN_POINT ( 'NONE',  ( 9.777492251018479408, 2.011184903788696410, 13.35065112715840563 ) ) ;
#16533=EDGE_CURVE ( 'NONE', #12570, #30330, #33558, .T. ) ;
#16534=AXIS2_PLACEMENT_3D ( 'NONE', #23814, #14765, #19470 ) ;
#16535=DIRECTION ( 'NONE',  ( 0.000000000000000000, 0.01356324068817998940, -0.9999080150203990547 ) ) ;
#16536=DIRECTION ( 'NONE',  ( 0.000000000000000000, -0.2618041379715496664, 0.9651210252299831094 ) ) ;
#16539=EDGE_LOOP ( 'NONE', ( #45558, #22875, #17534, #17698 ) ) ;
#16540=DIRECTION ( 'NONE',  ( 1.000000000000000000, -0.000000000000000000, 0.000000000000000000 ) ) ;
#16542=LINE ( 'NONE', #11858, #33208 ) ;
#16544=CARTESIAN_POINT ( 'NONE',  ( 35.00000000000000000, 5.644643009979216863, 10.30098186818242922 ) ) ;
#16547=LINE ( 'NONE', #27168, #13844 ) ;
#16548=EDGE_CURVE ( 'NONE', #42325, #12979, #58614, .T. ) ;
#16549=ORIENTED_EDGE ( 'NONE', *, *, #46011, .F. ) ;
#16550=EDGE_LOOP ( 'NONE', ( #21526, #17984, #1622, #28318 ) ) ;
#16551=DIRECTION ( 'NONE',  ( -1.000000000000000000, 0.000000000000000000, -0.000000000000000000 ) ) ;
#16557=CARTESIAN_POINT ( 'NONE',  ( 35.00000000000000000, -0.3137578094510123927, -12.74613886779084737 ) ) ;
#16559=ORIENTED_EDGE ( 'NONE', *, *, #1952, .T. ) ;
#16562=DIRECTION ( 'NONE',  ( -1.000000000000000000, 0.000000000000000000, -0.000000000000000000 ) ) ;
#16563=CARTESIAN_POINT ( 'NONE',  ( -21.17861794710831091, 25.00000000000000000, -3.604945070120774808 ) ) ;
#16564=CIRCLE ( 'NONE', #10182, 12.75000000000000178 ) ;
#16565=CARTESIAN_POINT ( 'NONE',  ( -36.00000000000000711, 2.865935305911801123, -12.42372387097879383 ) ) ;
#16566=CARTESIAN_POINT ( 'NONE',  ( 35.00000000000000000, 11.05394794832829497, -5.130401251914769922 ) ) ;
#16567=VECTOR ( 'NONE', #13507, 1000.000000000000000 ) ;
#16568=ORIENTED_EDGE ( 'NONE', *, *, #57234, .F. ) ;
#16569=DIRECTION ( 'NONE',  ( -1.000000000000000000, -0.000000000000000000, 0.000000000000000000 ) ) ;
#16570=ORIENTED_EDGE ( 'NONE', *, *, #35554, .T. ) ;
#16576=CARTESIAN_POINT ( 'NONE',  ( -37.00000000000000711, -5.636262487437237567, -10.80478261802188023 ) ) ;
#16577=AXIS2_PLACEMENT_3D ( 'NONE', #56255, #11046, #51626 ) ;
#16578=ORIENTED_EDGE ( 'NONE', *, *, #2604, .T. ) ;
#16579=VERTEX_POINT ( 'NONE', #19242 ) ;
#16581=VERTEX_POINT ( 'NONE', #55467 ) ;
#16583=CARTESIAN_POINT ( 'NONE',  ( -35.00000000000000000, -2.021542716731318912, -12.01765980939844169 ) ) ;
#16584=DIRECTION ( 'NONE',  ( 1.000000000000000000, 0.000000000000000000, -0.000000000000000000 ) ) ;
#16585=FACE_OUTER_BOUND ( 'NONE', #1116, .T. ) ;
#16586=LINE ( 'NONE', #26229, #53450 ) ;
#16588=CARTESIAN_POINT ( 'NONE',  ( -11.40165637462999904, -7.508992741355383416, 11.21895841913464409 ) ) ;
#16589=CARTESIAN_POINT ( 'NONE',  ( -9.082707185599058874, -2.483053339704398788, 11.74128942805037212 ) ) ;
#16590=VERTEX_POINT ( 'NONE', #18618 ) ;
#16592=VERTEX_POINT ( 'NONE', #38874 ) ;
#16593=DIRECTION ( 'NONE',  ( -1.000000000000000000, 0.000000000000000000, 0.000000000000000000 ) ) ;
#16594=CARTESIAN_POINT ( 'NONE',  ( 16.87411378711497179, 11.83810385330096082, 6.535220105381315037 ) ) ;
#16595=EDGE_CURVE ( 'NONE', #13015, #37639, #47152, .T. ) ;
#16596=DIRECTION ( 'NONE',  ( -1.000000000000000000, 0.000000000000000000, -0.000000000000000000 ) ) ;
#16599=CARTESIAN_POINT ( 'NONE',  ( -35.00000000000000000, 12.05416472667165806, 1.791059740004466994 ) ) ;
#16601=EDGE_LOOP ( 'NONE', ( #38499, #11191, #44066, #34647 ) ) ;
#16602=ORIENTED_EDGE ( 'NONE', *, *, #55402, .F. ) ;
#16603=CARTESIAN_POINT ( 'NONE',  ( 37.00000000000000711, -11.42599468261426132, 4.237620530777920891 ) ) ;
#16605=EDGE_CURVE ( 'NONE', #60108, #60760, #34365, .T. ) ;
#16606=DIRECTION ( 'NONE',  ( -1.000000000000000000, -0.000000000000000000, 0.000000000000000000 ) ) ;
#16607=ORIENTED_EDGE ( 'NONE', *, *, #62738, .F. ) ;
#16609=VERTEX_POINT ( 'NONE', #39512 ) ;
#16613=LINE ( 'NONE', #7269, #43702 ) ;
#16614=DIRECTION ( 'NONE',  ( 0.000000000000000000, -0.9903235168508566222, -0.1387779952735712363 ) ) ;
#16615=DIRECTION ( 'NONE',  ( 0.000000000000000000, -0.01356324068818000328, 0.9999080150203990547 ) ) ;
#16616=VERTEX_POINT ( 'NONE', #59809 ) ;
#16620=VERTEX_POINT ( 'NONE', #13901 ) ;
#16621=FACE_OUTER_BOUND ( 'NONE', #26847, .T. ) ;
#16622=CARTESIAN_POINT ( 'NONE',  ( -3.548017078132182700, 11.40818985387241824, 7.227869169360847224 ) ) ;
#16623=CARTESIAN_POINT ( 'NONE',  ( 35.00000000000000000, 4.705694406421931860E-17, -3.469127814946512892E-15 ) ) ;
#16628=EDGE_LOOP ( 'NONE', ( #34202, #43449, #654, #63841 ) ) ;
#16637=DIRECTION ( 'NONE',  ( -1.000000000000000000, 0.000000000000000000, 0.000000000000000000 ) ) ;
#16638=CYLINDRICAL_SURFACE ( 'NONE', #1527, 5.000000000000000000 ) ;
#16644=DIRECTION ( 'NONE',  ( 1.000000000000000000, -0.000000000000000000, 0.000000000000000000 ) ) ;
#16645=AXIS2_PLACEMENT_3D ( 'NONE', #12485, #38429, #23469 ) ;
#16646=CIRCLE ( 'NONE', #24099, 12.75000000000000178 ) ;
#16648=EDGE_CURVE ( 'NONE', #11726, #59597, #41462, .T. ) ;
#16649=VERTEX_POINT ( 'NONE', #61111 ) ;
#16650=DIRECTION ( 'NONE',  ( 1.000000000000000000, 0.000000000000000000, 0.000000000000000000 ) ) ;
#16652=CARTESIAN_POINT ( 'NONE',  ( -29.66426065917772092, -2.171908341933164621, 13.32952346240084118 ) ) ;
#16653=DIRECTION ( 'NONE',  ( 0.000000000000000000, -0.01356324068817999114, 0.9999080150203989437 ) ) ;
#16654=EDGE_CURVE ( 'NONE', #11684, #60382, #59869, .T. ) ;
#16655=ORIENTED_EDGE ( 'NONE', *, *, #25131, .F. ) ;
#16656=VERTEX_POINT ( 'NONE', #30831 ) ;
#16658=DIRECTION ( 'NONE',  ( -1.000000000000000000, 0.000000000000000000, 0.000000000000000000 ) ) ;
#16659=CARTESIAN_POINT ( 'NONE',  ( 22.21055375121776976, 11.96926186085322286, -0.8606626411553330858 ) ) ;
#16660=EDGE_CURVE ( 'NONE', #59695, #2788, #41808, .T. ) ;
#16661=ORIENTED_EDGE ( 'NONE', *, *, #60909, .F. ) ;
#16662=LINE ( 'NONE', #20979, #29407 ) ;
#16663=CARTESIAN_POINT ( 'NONE',  ( 35.00000000000000000, -4.309077947445731027, -10.92721691015454510 ) ) ;
#16664=VERTEX_POINT ( 'NONE', #56108 ) ;
#16665=CARTESIAN_POINT ( 'NONE',  ( 35.00000000000000000, 12.14284015767851166, 1.030638227056429157 ) ) ;
#16667=DIRECTION ( 'NONE',  ( -1.000000000000000000, 0.000000000000000000, -0.000000000000000000 ) ) ;
#16668=VERTEX_POINT ( 'NONE', #50807 ) ;
#16669=DIRECTION ( 'NONE',  ( 0.000000000000000000, 0.01356324068817998940, -0.9999080150203990547 ) ) ;
#16670=VERTEX_POINT ( 'NONE', #20554 ) ;
#16675=CARTESIAN_POINT ( 'NONE',  ( -36.00000000000000711, -11.32068061209291265, -5.865551165831199398 ) ) ;
#16676=CARTESIAN_POINT ( 'NONE',  ( 35.00000000000000000, -11.59095880812006385, 1.903127969211307224 ) ) ;
#16677=CARTESIAN_POINT ( 'NONE',  ( 8.932556049095349948, 2.405355177192989746, 11.75892528794417835 ) ) ;
#16678=DIRECTION ( 'NONE',  ( -1.000000000000000000, 0.000000000000000000, 0.000000000000000000 ) ) ;
#16680=EDGE_LOOP ( 'NONE', ( #54715, #3550, #53871, #24758 ) ) ;
#16681=EDGE_CURVE ( 'NONE', #50289, #44901, #36820, .T. ) ;
#16682=DIRECTION ( 'NONE',  ( -1.000000000000000000, 0.000000000000000000, 0.000000000000000000 ) ) ;
#16684=LINE ( 'NONE', #36955, #60387 ) ;
#16686=EDGE_LOOP ( 'NONE', ( #59547, #61005, #30977, #35567 ) ) ;
#16687=CARTESIAN_POINT ( 'NONE',  ( -35.00000000000000000, 11.68758509253248334, -1.171570255487489609 ) ) ;
#16688=CARTESIAN_POINT ( 'NONE',  ( -35.00000000000000000, 0.000000000000000000, 0.000000000000000000 ) ) ;
#16689=CARTESIAN_POINT ( 'NONE',  ( -4.806344283790351390, -7.508992741355383416, 25.00000000000000000 ) ) ;
#16690=AXIS2_PLACEMENT_3D ( 'NONE', #7341, #36947, #2389 ) ;
#16693=VERTEX_POINT ( 'NONE', #16213 ) ;
#16695=CARTESIAN_POINT ( 'NONE',  ( -18.33734242530290004, -4.538935765794358979, -11.11102257328130172 ) ) ;
#16697=ORIENTED_EDGE ( 'NONE', *, *, #50173, .F. ) ;
#16698=DIRECTION ( 'NONE',  ( -1.000000000000000000, 0.000000000000000000, -0.000000000000000000 ) ) ;
#16699=CARTESIAN_POINT ( 'NONE',  ( -37.00000000000000711, 0.000000000000000000, 0.000000000000000000 ) ) ;
#16701=ORIENTED_EDGE ( 'NONE', *, *, #24564, .F. ) ;
#16702=DIRECTION ( 'NONE',  ( -1.000000000000000000, 0.000000000000000000, -0.000000000000000000 ) ) ;
#16703=EDGE_CURVE ( 'NONE', #42839, #49489, #31192, .T. ) ;
#16707=CYLINDRICAL_SURFACE ( 'NONE', #7658, 5.000000000000000888 ) ;
#16708=CARTESIAN_POINT ( 'NONE',  ( 37.00000000000000711, 11.38112321385050585, -2.905556151562669331 ) ) ;
#16709=DIRECTION ( 'NONE',  ( 0.000000000000000000, 0.01356324068818000848, -0.9999080150203990547 ) ) ;
#16710=DIRECTION ( 'NONE',  ( 0.000000000000000000, -0.01356324068817999114, 0.9999080150203989437 ) ) ;
#16714=EDGE_LOOP ( 'NONE', ( #40894, #42648, #24454, #50704 ) ) ;
#16716=CARTESIAN_POINT ( 'NONE',  ( 11.74548640120467979, 25.00000000000000000, -8.184666801472349817 ) ) ;
#16717=ORIENTED_EDGE ( 'NONE', *, *, #7381, .F. ) ;
#16718=EDGE_CURVE ( 'NONE', #25248, #51431, #11228, .T. ) ;
#16719=FACE_OUTER_BOUND ( 'NONE', #65628, .T. ) ;
#16720=DIRECTION ( 'NONE',  ( 0.000000000000000000, -0.01356324068817998940, 0.9999080150203990547 ) ) ;
#16723=EDGE_CURVE ( 'NONE', #7740, #924, #56807, .T. ) ;
#16724=ORIENTED_EDGE ( 'NONE', *, *, #48114, .T. ) ;
#16726=ORIENTED_EDGE ( 'NONE', *, *, #33780, .F. ) ;
#16727=AXIS2_PLACEMENT_3D ( 'NONE', #48443, #48759, #59712 ) ;
#16728=ORIENTED_EDGE ( 'NONE', *, *, #32219, .T. ) ;
#16729=DIRECTION ( 'NONE',  ( -0.000000000000000000, -0.000000000000000000, -1.000000000000000000 ) ) ;
#16731=EDGE_CURVE ( 'NONE', #13080, #6530, #28014, .T. ) ;
#16732=VERTEX_POINT ( 'NONE', #51802 ) ;
#16733=CARTESIAN_POINT ( 'NONE',  ( -25.36156277276711535, -9.869979630862522058, 6.826986832051105125 ) ) ;
#16735=CARTESIAN_POINT ( 'NONE',  ( -35.00000000000000000, 0.000000000000000000, 0.000000000000000000 ) ) ;
#16737=ORIENTED_EDGE ( 'NONE', *, *, #3002, .T. ) ;
#16739=EDGE_CURVE ( 'NONE', #48166, #24413, #65165, .T. ) ;
#16741=CARTESIAN_POINT ( 'NONE',  ( -37.00000000000000711, 0.000000000000000000, 0.000000000000000000 ) ) ;
#16742=CARTESIAN_POINT ( 'NONE',  ( -24.88606550871976708, 5.771222983236214965, 10.55595544087139004 ) ) ;
#16743=VERTEX_POINT ( 'NONE', #60784 ) ;
#16744=FACE_OUTER_BOUND ( 'NONE', #60682, .T. ) ;
#16745=ORIENTED_EDGE ( 'NONE', *, *, #14859, .F. ) ;
#16746=DIRECTION ( 'NONE',  ( -1.000000000000000000, 0.000000000000000000, 0.000000000000000000 ) ) ;
#16748=DIRECTION ( 'NONE',  ( 1.000000000000000000, 0.000000000000000000, 0.000000000000000000 ) ) ;
#16749=EDGE_CURVE ( 'NONE', #23475, #2241, #4682, .T. ) ;
#16752=ORIENTED_EDGE ( 'NONE', *, *, #52425, .F. ) ;
#16753=CARTESIAN_POINT ( 'NONE',  ( 37.00000000000000711, 4.705694406421931860E-17, -3.469127814946512892E-15 ) ) ;
#16754=CARTESIAN_POINT ( 'NONE',  ( -35.00000000000000000, 0.000000000000000000, 0.000000000000000000 ) ) ;
#16755=CARTESIAN_POINT ( 'NONE',  ( -35.00000000000000000, -4.041347439435779343, -11.02904044024213270 ) ) ;
#16756=EDGE_CURVE ( 'NONE', #20776, #173, #5717, .T. ) ;
#16758=VERTEX_POINT ( 'NONE', #30509 ) ;
#16759=CARTESIAN_POINT ( 'NONE',  ( -37.00000000000000711, -0.8294751490780184477, 12.15823808070322620 ) ) ;
#16760=ORIENTED_EDGE ( 'NONE', *, *, #83, .F. ) ;
#16761=EDGE_CURVE ( 'NONE', #3506, #62548, #25528, .T. ) ;
#16762=ORIENTED_EDGE ( 'NONE', *, *, #50923, .T. ) ;
#16764=FACE_OUTER_BOUND ( 'NONE', #21595, .T. ) ;
#16765=DIRECTION ( 'NONE',  ( 0.000000000000000000, 0.01356324068817992175, -0.9999080150203990547 ) ) ;
#16768=VECTOR ( 'NONE', #18160, 1000.000000000000000 ) ;
#16769=DIRECTION ( 'NONE',  ( -1.000000000000000000, 0.000000000000000000, -0.000000000000000000 ) ) ;
#16771=CIRCLE ( 'NONE', #10398, 4.999999999999999112 ) ;
#16775=DIRECTION ( 'NONE',  ( 1.000000000000000000, 0.000000000000000000, 0.000000000000000000 ) ) ;
#16776=AXIS2_PLACEMENT_3D ( 'NONE', #44639, #45985, #5095 ) ;
#16780=CYLINDRICAL_SURFACE ( 'NONE', #42755, 12.18649999999999878 ) ;
#16781=CARTESIAN_POINT ( 'NONE',  ( 35.00000000000000000, -7.499679039483992504, 9.040300684349768190 ) ) ;
#16783=ORIENTED_EDGE ( 'NONE', *, *, #30224, .F. ) ;
#16784=DIRECTION ( 'NONE',  ( -0.000000000000000000, -1.000000000000000000, -0.000000000000000000 ) ) ;
#16785=DIRECTION ( 'NONE',  ( -1.000000000000000000, 0.000000000000000000, 0.000000000000000000 ) ) ;
#16786=CARTESIAN_POINT ( 'NONE',  ( -25.86628395826706850, 5.139808748864376220, 10.84354029019568522 ) ) ;
#16790=CARTESIAN_POINT ( 'NONE',  ( 11.56239109567838597, 0.7119215618323401218, -13.48139877484980609 ) ) ;
#16793=CIRCLE ( 'NONE', #25298, 5.000000000000000000 ) ;
#16795=CARTESIAN_POINT ( 'NONE',  ( -35.00000000000000000, -11.38112321385052716, 2.905556151562584954 ) ) ;
#16796=DIRECTION ( 'NONE',  ( -0.000000000000000000, -1.000000000000000000, -0.000000000000000000 ) ) ;
#16797=DIRECTION ( 'NONE',  ( 0.000000000000000000, -0.01356324068817998940, 0.9999080150203990547 ) ) ;
#16800=DIRECTION ( 'NONE',  ( 1.000000000000000000, -0.000000000000000000, 0.000000000000000000 ) ) ;
#16803=VERTEX_POINT ( 'NONE', #42433 ) ;
#16804=FACE_OUTER_BOUND ( 'NONE', #39883, .T. ) ;
#16805=VECTOR ( 'NONE', #25186, 1000.000000000000000 ) ;
#16806=DIRECTION ( 'NONE',  ( -1.000000000000000000, 0.000000000000000000, 0.000000000000000000 ) ) ;
#16807=EDGE_LOOP ( 'NONE', ( #31567, #10839, #18763, #40896 ) ) ;
#16808=DIRECTION ( 'NONE',  ( 1.000000000000000000, 0.000000000000000000, 0.000000000000000000 ) ) ;
#16809=CARTESIAN_POINT ( 'NONE',  ( -37.00000000000000711, -5.672855678558757830, 10.28547182238005853 ) ) ;
#16810=AXIS2_PLACEMENT_3D ( 'NONE', #60458, #50825, #35175 ) ;
#16812=CIRCLE ( 'NONE', #60342, 12.18649999999999878 ) ;
#16813=CARTESIAN_POINT ( 'NONE',  ( -2.952869152607107139, -12.96714474214480717, 3.755417052241487585 ) ) ;
#16814=CARTESIAN_POINT ( 'NONE',  ( -7.489022030332961322, 5.127957880411581293, -10.84914964302385521 ) ) ;
#16815=ADVANCED_FACE ( 'NONE', ( #28162 ), #32789, .T. ) ;
#16816=DIRECTION ( 'NONE',  ( -1.000000000000000000, 0.000000000000000000, 0.000000000000000000 ) ) ;
#16817=DIRECTION ( 'NONE',  ( 0.000000000000000000, -0.3554799084908835116, -0.9346839223284592046 ) ) ;
#16818=ORIENTED_EDGE ( 'NONE', *, *, #51406, .F. ) ;
#16819=EDGE_CURVE ( 'NONE', #40162, #11383, #15282, .T. ) ;
#16821=CARTESIAN_POINT ( 'NONE',  ( 24.79913956981017975, -1.736766911523203172, -11.87527920162771089 ) ) ;
#16823=AXIS2_PLACEMENT_3D ( 'NONE', #23578, #18910, #39833 ) ;
#16826=ADVANCED_FACE ( 'NONE', ( #48456 ), #2240, .T. ) ;
#16827=CARTESIAN_POINT ( 'NONE',  ( -17.59990429990587657, 3.555202520397811039, 11.46264038328473589 ) ) ;
#16832=CARTESIAN_POINT ( 'NONE',  ( 3.742705681669799667, 4.513412766533817511, -12.75114006814483680 ) ) ;
#16833=VERTEX_POINT ( 'NONE', #7204 ) ;
#16834=ORIENTED_EDGE ( 'NONE', *, *, #45473, .T. ) ;
#16835=EDGE_CURVE ( 'NONE', #38215, #27894, #2904, .T. ) ;
#16836=CARTESIAN_POINT ( 'NONE',  ( 26.76944249566220435, -12.82941635345952847, 4.211941481156896039 ) ) ;
#16840=DIRECTION ( 'NONE',  ( 0.000000000000000000, 0.01356324068817991828, -0.9999080150203990547 ) ) ;
#16843=DIRECTION ( 'NONE',  ( -1.000000000000000000, -0.000000000000000000, 0.000000000000000000 ) ) ;
#16845=DIRECTION ( 'NONE',  ( 0.000000000000000000, 0.01356324068817992175, -0.9999080150203990547 ) ) ;
#16847=DIRECTION ( 'NONE',  ( -1.000000000000000000, 0.000000000000000000, 0.000000000000000000 ) ) ;
#16848=AXIS2_PLACEMENT_3D ( 'NONE', #17764, #53000, #31717 ) ;
#16849=EDGE_LOOP ( 'NONE', ( #571, #18897, #21815, #6879 ) ) ;
#16850=LINE ( 'NONE', #27165, #9800 ) ;
#16851=DIRECTION ( 'NONE',  ( 0.000000000000000000, -0.1740410799127685149, -0.9847383929261604996 ) ) ;
#16854=DIRECTION ( 'NONE',  ( 0.000000000000000000, 0.01356324068817992175, -0.9999080150203990547 ) ) ;
#16857=ORIENTED_EDGE ( 'NONE', *, *, #7691, .T. ) ;
#16858=ADVANCED_FACE ( 'NONE', ( #38455 ), #27827, .T. ) ;
#16861=EDGE_CURVE ( 'NONE', #13432, #53221, #13192, .T. ) ;
#16862=VECTOR ( 'NONE', #35988, 1000.000000000000000 ) ;
#16865=DIRECTION ( 'NONE',  ( 1.000000000000000000, 0.000000000000000000, -0.000000000000000000 ) ) ;
#16867=CIRCLE ( 'NONE', #54042, 12.75000000000000178 ) ;
#16870=ORIENTED_EDGE ( 'NONE', *, *, #25086, .T. ) ;
#16872=CYLINDRICAL_SURFACE ( 'NONE', #3537, 5.000000000000000888 ) ;
#16873=EDGE_CURVE ( 'NONE', #24405, #65324, #19495, .T. ) ;
#16874=DIRECTION ( 'NONE',  ( 0.000000000000000000, 0.000000000000000000, -1.000000000000000000 ) ) ;
#16875=AXIS2_PLACEMENT_3D ( 'NONE', #55722, #55379, #40398 ) ;
#16877=DIRECTION ( 'NONE',  ( 0.000000000000000000, -0.01356324068817991828, 0.9999080150203990547 ) ) ;
#16880=ORIENTED_EDGE ( 'NONE', *, *, #61756, .F. ) ;
#16881=DIRECTION ( 'NONE',  ( 1.000000000000000000, -0.000000000000000000, -0.000000000000000000 ) ) ;
#16884=DIRECTION ( 'NONE',  ( 0.000000000000000000, -0.01356324068817999114, 0.9999080150203989437 ) ) ;
#16886=EDGE_CURVE ( 'NONE', #21123, #1597, #32263, .T. ) ;
#16887=DIRECTION ( 'NONE',  ( 0.000000000000000000, -0.8989688749565110104, -0.4380125133594070519 ) ) ;
#16889=CYLINDRICAL_SURFACE ( 'NONE', #64912, 4.999999999999998224 ) ;
#16890=VECTOR ( 'NONE', #38761, 1000.000000000000000 ) ;
#16892=VERTEX_POINT ( 'NONE', #28805 ) ;
#16894=EDGE_LOOP ( 'NONE', ( #35038, #61752, #59556, #4869 ) ) ;
#16895=CARTESIAN_POINT ( 'NONE',  ( 3.291290029914074378, 8.250315036047103590, 8.713914264323182834 ) ) ;
#16896=CARTESIAN_POINT ( 'NONE',  ( 3.291290029914074378, 8.250315036047103590, -10.68561190601526079 ) ) ;
#16897=CYLINDRICAL_SURFACE ( 'NONE', #61729, 5.000000000000000888 ) ;
#16898=( BOUNDED_CURVE ( )  B_SPLINE_CURVE ( 3, ( #58691, #43687, #54007, #45256 ),
 .UNSPECIFIED., .F., .F. ) 
 B_SPLINE_CURVE_WITH_KNOTS ( ( 4, 4 ),
 ( 1.238310171490985434, 1.242866721674340758 ),
 .UNSPECIFIED. ) 
 CURVE ( )  GEOMETRIC_REPRESENTATION_ITEM ( )  RATIONAL_B_SPLINE_CURVE ( ( 1.000000000000000000, 0.9999982698216172139, 0.9999982698216172139, 1.000000000000000000 ) ) 
 REPRESENTATION_ITEM ( '' )  );
#16900=CIRCLE ( 'NONE', #50895, 12.18649999999999878 ) ;
#16903=CARTESIAN_POINT ( 'NONE',  ( -37.00000000000000711, 7.882940143791919319, -10.02106554660700333 ) ) ;
#16904=VERTEX_POINT ( 'NONE', #59088 ) ;
#16905=DIRECTION ( 'NONE',  ( 1.000000000000000000, 0.000000000000000000, 0.000000000000000000 ) ) ;
#16906=ORIENTED_EDGE ( 'NONE', *, *, #50573, .F. ) ;
#16907=SURFACE_SIDE_STYLE ('',( #2637 ) ) ;
#16909=EDGE_CURVE ( 'NONE', #41059, #37494, #18906, .T. ) ;
#16911=AXIS2_PLACEMENT_3D ( 'NONE', #26232, #15901, #20247 ) ;
#16913=EDGE_CURVE ( 'NONE', #50873, #64499, #63078, .T. ) ;
#16915=CIRCLE ( 'NONE', #30706, 5.000000000000000000 ) ;
#16916=ORIENTED_EDGE ( 'NONE', *, *, #27243, .F. ) ;
#16917=LINE ( 'NONE', #1646, #53494 ) ;
#16918=DIRECTION ( 'NONE',  ( -1.000000000000000000, -0.000000000000000000, -0.000000000000000000 ) ) ;
#16919=DIRECTION ( 'NONE',  ( 1.000000000000000000, -0.000000000000000000, 0.000000000000000000 ) ) ;
#16920=VERTEX_POINT ( 'NONE', #24460 ) ;
#16921=ORIENTED_EDGE ( 'NONE', *, *, #30204, .T. ) ;
#16922=EDGE_CURVE ( 'NONE', #46560, #63220, #40772, .T. ) ;
#16923=CARTESIAN_POINT ( 'NONE',  ( 3.427798639585919016, 7.593315936193067550, 11.19287808785590066 ) ) ;
#16924=ORIENTED_EDGE ( 'NONE', *, *, #8900, .F. ) ;
#16925=EDGE_LOOP ( 'NONE', ( #12474, #4338, #11036, #65401 ) ) ;
#16926=ORIENTED_EDGE ( 'NONE', *, *, #15551, .F. ) ;
#16927=AXIS2_PLACEMENT_3D ( 'NONE', #21024, #51647, #27017 ) ;
#16928=ORIENTED_EDGE ( 'NONE', *, *, #23266, .T. ) ;
#16930=FACE_OUTER_BOUND ( 'NONE', #12743, .T. ) ;
#16934=CARTESIAN_POINT ( 'NONE',  ( -35.00000000000000000, 4.732539170486427693, -11.23004253107759176 ) ) ;
#16935=ORIENTED_EDGE ( 'NONE', *, *, #56803, .F. ) ;
#16936=ADVANCED_FACE ( 'NONE', ( #23497 ), #54749, .T. ) ;
#16937=FACE_OUTER_BOUND ( 'NONE', #57531, .T. ) ;
#16938=ORIENTED_EDGE ( 'NONE', *, *, #21895, .F. ) ;
#16939=DIRECTION ( 'NONE',  ( 1.000000000000000000, 0.000000000000000000, 0.000000000000000000 ) ) ;
#16944=FACE_OUTER_BOUND ( 'NONE', #35586, .T. ) ;
#16947=DIRECTION ( 'NONE',  ( 0.000000000000000000, -0.1118654143051477368, -0.9937233664769776764 ) ) ;
#16948=EDGE_CURVE ( 'NONE', #60501, #9614, #12099, .T. ) ;
#16949=AXIS2_PLACEMENT_3D ( 'NONE', #28393, #64296, #44648 ) ;
#16950=ORIENTED_EDGE ( 'NONE', *, *, #45461, .F. ) ;
#16952=DIRECTION ( 'NONE',  ( -1.000000000000000000, 0.000000000000000000, 0.000000000000000000 ) ) ;
#16953=DIRECTION ( 'NONE',  ( -1.000000000000000000, 0.000000000000000000, -0.000000000000000000 ) ) ;
#16954=CARTESIAN_POINT ( 'NONE',  ( 37.00000000000000711, 6.102719229070675766, -10.54834585426222482 ) ) ;
#16959=DIRECTION ( 'NONE',  ( 1.000000000000000000, 0.000000000000000000, 0.000000000000000000 ) ) ;
#16961=AXIS2_PLACEMENT_3D ( 'NONE', #64484, #39551, #18953 ) ;
#16962=CIRCLE ( 'NONE', #24400, 4.999999999999999112 ) ;
#16963=DIRECTION ( 'NONE',  ( -1.000000000000000000, -0.000000000000000000, 0.000000000000000000 ) ) ;
#16964=ORIENTED_EDGE ( 'NONE', *, *, #19704, .T. ) ;
#16967=ADVANCED_FACE ( 'NONE', ( #65021 ), #18537, .T. ) ;
#16968=AXIS2_PLACEMENT_3D ( 'NONE', #60496, #20265, #40545 ) ;
#16971=VERTEX_POINT ( 'NONE', #24144 ) ;
#16973=CYLINDRICAL_SURFACE ( 'NONE', #51326, 12.74999999999999822 ) ;
#16977=ORIENTED_EDGE ( 'NONE', *, *, #51650, .F. ) ;
#16978=ORIENTED_EDGE ( 'NONE', *, *, #58394, .F. ) ;
#16981=AXIS2_PLACEMENT_3D ( 'NONE', #33576, #62838, #42885 ) ;
#16982=CARTESIAN_POINT ( 'NONE',  ( -37.00000000000000711, -10.14433819232429812, -6.753013023069823539 ) ) ;
#16983=AXIS2_PLACEMENT_3D ( 'NONE', #17930, #37879, #53178 ) ;
#16987=ORIENTED_EDGE ( 'NONE', *, *, #29485, .F. ) ;
#16989=FACE_OUTER_BOUND ( 'NONE', #54194, .T. ) ;
#16990=FACE_OUTER_BOUND ( 'NONE', #64558, .T. ) ;
#16991=EDGE_LOOP ( 'NONE', ( #40232, #1964, #37600, #56151 ) ) ;
#16992=DIRECTION ( 'NONE',  ( 0.000000000000000000, -0.01356324068817998940, 0.9999080150203990547 ) ) ;
#16994=DIRECTION ( 'NONE',  ( 1.000000000000000000, 0.000000000000000000, 0.000000000000000000 ) ) ;
#16996=AXIS2_PLACEMENT_3D ( 'NONE', #23451, #17489, #16817 ) ;
#16997=EDGE_CURVE ( 'NONE', #10987, #43919, #46715, .T. ) ;
#17000=DIRECTION ( 'NONE',  ( 1.000000000000000000, -0.000000000000000000, 0.000000000000000000 ) ) ;
#17002=CARTESIAN_POINT ( 'NONE',  ( 35.00000000000000000, 4.705694406421931860E-17, -3.469127814946512892E-15 ) ) ;
#17003=ORIENTED_EDGE ( 'NONE', *, *, #39388, .F. ) ;
#17004=CARTESIAN_POINT ( 'NONE',  ( -35.00000000000000000, -9.512294188640947112, 6.891188680298791169 ) ) ;
#17006=CARTESIAN_POINT ( 'NONE',  ( -35.00000000000000000, 0.000000000000000000, 0.000000000000000000 ) ) ;
#17008=ORIENTED_EDGE ( 'NONE', *, *, #17879, .F. ) ;
#17010=CARTESIAN_POINT ( 'NONE',  ( -37.00000000000000711, -12.46157735505191333, 2.696588552979012121 ) ) ;
#17012=CIRCLE ( 'NONE', #62653, 12.18650000000000055 ) ;
#17013=CARTESIAN_POINT ( 'NONE',  ( -35.00000000000000000, -11.13736569743278082, 4.946702696913133579 ) ) ;
#17016=ORIENTED_EDGE ( 'NONE', *, *, #22167, .T. ) ;
#17019=AXIS2_PLACEMENT_3D ( 'NONE', #47224, #32535, #1670 ) ;
#17020=EDGE_CURVE ( 'NONE', #64858, #2304, #12005, .T. ) ;
#17023=DIRECTION ( 'NONE',  ( 0.000000000000000000, 0.2006870767258820687, -0.9796553971857756560 ) ) ;
#17024=ADVANCED_FACE ( 'NONE', ( #40403 ), #51066, .T. ) ;
#17026=CARTESIAN_POINT ( 'NONE',  ( 36.00000000000000711, -0.1414404973753014549, -12.74921544981111055 ) ) ;
#17028=ORIENTED_EDGE ( 'NONE', *, *, #8175, .F. ) ;
#17030=CIRCLE ( 'NONE', #58490, 5.000000000000000000 ) ;
#17032=EDGE_CURVE ( 'NONE', #2632, #53954, #30437, .T. ) ;
#17033=CIRCLE ( 'NONE', #57384, 5.000000000000000000 ) ;
#17034=CARTESIAN_POINT ( 'NONE',  ( 29.23374216858299945, 9.169383756589978063, 9.943439309940176329 ) ) ;
#17035=DIRECTION ( 'NONE',  ( -0.000000000000000000, -0.000000000000000000, -1.000000000000000000 ) ) ;
#17036=CARTESIAN_POINT ( 'NONE',  ( 24.44415356966865360, 11.03103468991324654, -7.786488058063032014 ) ) ;
#17037=CARTESIAN_POINT ( 'NONE',  ( -35.00000000000000000, 14.99999999999998757, 1.836970198721028406E-15 ) ) ;
#17039=EDGE_CURVE ( 'NONE', #50979, #59495, #841, .T. ) ;
#17045=CARTESIAN_POINT ( 'NONE',  ( 4.492447587936224451, -10.17925049329322107, 8.868279803853196697 ) ) ;
#17046=ORIENTED_EDGE ( 'NONE', *, *, #42742, .F. ) ;
#17048=DIRECTION ( 'NONE',  ( -1.000000000000000000, 0.000000000000000000, 0.000000000000000000 ) ) ;
#17049=ORIENTED_EDGE ( 'NONE', *, *, #2976, .T. ) ;
#17053=CARTESIAN_POINT ( 'NONE',  ( -35.00000000000000000, -8.534258022646161734, 8.699265615722952205 ) ) ;
#17055=ORIENTED_EDGE ( 'NONE', *, *, #43434, .F. ) ;
#17056=DIRECTION ( 'NONE',  ( 1.000000000000000000, -0.000000000000000000, 0.000000000000000000 ) ) ;
#17060=DIRECTION ( 'NONE',  ( 0.000000000000000000, -0.01356324068817999114, 0.9999080150203989437 ) ) ;
#17061=VECTOR ( 'NONE', #9530, 1000.000000000000000 ) ;
#17063=ORIENTED_EDGE ( 'NONE', *, *, #20516, .T. ) ;
#17067=CARTESIAN_POINT ( 'NONE',  ( -24.79033130866653067, 9.927070015466320285, 6.752286632236016217 ) ) ;
#17069=CARTESIAN_POINT ( 'NONE',  ( 37.00000000000000711, -9.621072037176935154, 8.366449238204463512 ) ) ;
#17070=VECTOR ( 'NONE', #49781, 1000.000000000000000 ) ;
#17071=ORIENTED_EDGE ( 'NONE', *, *, #28185, .F. ) ;
#17075=DIRECTION ( 'NONE',  ( -1.000000000000000000, -0.000000000000000000, 0.000000000000000000 ) ) ;
#17078=ADVANCED_FACE ( 'NONE', ( #10473 ), #25791, .T. ) ;
#17079=AXIS2_PLACEMENT_3D ( 'NONE', #63002, #37067, #37401 ) ;
#17080=VERTEX_POINT ( 'NONE', #30749 ) ;
#17082=LINE ( 'NONE', #17426, #61183 ) ;
#17083=VECTOR ( 'NONE', #33509, 1000.000000000000000 ) ;
#17084=DIRECTION ( 'NONE',  ( -1.000000000000000000, 0.000000000000000000, 0.000000000000000000 ) ) ;
#17090=CIRCLE ( 'NONE', #50034, 12.18650000000000055 ) ;
#17091=CARTESIAN_POINT ( 'NONE',  ( -19.47984447937493613, -1.416020129149132334, 25.00000000000000000 ) ) ;
#17092=ORIENTED_EDGE ( 'NONE', *, *, #30774, .F. ) ;
#17094=DIRECTION ( 'NONE',  ( 0.000000000000000000, 0.8009703041134146329, 0.5987040770935705414 ) ) ;
#17095=CYLINDRICAL_SURFACE ( 'NONE', #14743, 5.000000000000000888 ) ;
#17097=DIRECTION ( 'NONE',  ( 0.000000000000000000, -0.9847383929261634972, 0.1740410799127515007 ) ) ;
#17100=AXIS2_PLACEMENT_3D ( 'NONE', #44558, #34900, #39913 ) ;
#17101=DIRECTION ( 'NONE',  ( 1.000000000000000000, 0.000000000000000000, 0.000000000000000000 ) ) ;
#17102=EDGE_CURVE ( 'NONE', #35595, #18920, #48107, .T. ) ;
#17104=AXIS2_PLACEMENT_3D ( 'NONE', #13353, #33638, #48948 ) ;
#17106=ORIENTED_EDGE ( 'NONE', *, *, #6617, .F. ) ;
#17107=VECTOR ( 'NONE', #57111, 1000.000000000000000 ) ;
#17108=LINE ( 'NONE', #22770, #14303 ) ;
#17109=EDGE_CURVE ( 'NONE', #32649, #63467, #13207, .T. ) ;
#17111=AXIS2_PLACEMENT_3D ( 'NONE', #13562, #13261, #2311 ) ;
#17112=CYLINDRICAL_SURFACE ( 'NONE', #14162, 12.74999999999999822 ) ;
#17114=EDGE_CURVE ( 'NONE', #34626, #59781, #59771, .T. ) ;
#17115=AXIS2_PLACEMENT_3D ( 'NONE', #10056, #31320, #61558 ) ;
#17117=EDGE_CURVE ( 'NONE', #50873, #7202, #39593, .T. ) ;
#17118=CARTESIAN_POINT ( 'NONE',  ( 9.213956812938336682, 1.933777648958550310, -11.84564966864138746 ) ) ;
#17119=VERTEX_POINT ( 'NONE', #30116 ) ;
#17120=DIRECTION ( 'NONE',  ( 0.000000000000000000, 0.9651210252299786685, 0.2618041379715667083 ) ) ;
#17122=CARTESIAN_POINT ( 'NONE',  ( -35.00000000000000000, 3.213188559034398040, -11.29812557209473667 ) ) ;
#17128=CARTESIAN_POINT ( 'NONE',  ( -24.90406945800131311, 9.123033189230673301, 7.797728632319192776 ) ) ;
#17130=ORIENTED_EDGE ( 'NONE', *, *, #60548, .T. ) ;
#17133=CARTESIAN_POINT ( 'NONE',  ( -37.00000000000000711, -2.346765782874520312, 11.95840593935200857 ) ) ;
#17135=ORIENTED_EDGE ( 'NONE', *, *, #26536, .F. ) ;
#17136=CARTESIAN_POINT ( 'NONE',  ( 145.1370849898475797, 3.309064568108273190E-14, 0.000000000000000000 ) ) ;
#17137=CARTESIAN_POINT ( 'NONE',  ( -35.00000000000000000, 6.584150480049696164, -10.25474254703945931 ) ) ;
#17141=VECTOR ( 'NONE', #25763, 1000.000000000000000 ) ;
#17147=CARTESIAN_POINT ( 'NONE',  ( -36.00000000000000711, 6.018036132182325915, -11.24036214326513949 ) ) ;
#17148=DIRECTION ( 'NONE',  ( -1.000000000000000000, 0.000000000000000000, -0.000000000000000000 ) ) ;
#17150=CARTESIAN_POINT ( 'NONE',  ( 26.08439714455133185, 12.97057518889166516, 3.743551691817328386 ) ) ;
#17153=CARTESIAN_POINT ( 'NONE',  ( -37.00000000000000711, -10.23119532541078058, 7.608228585767692564 ) ) ;
#17154=ORIENTED_EDGE ( 'NONE', *, *, #53422, .T. ) ;
#17155=CARTESIAN_POINT ( 'NONE',  ( -37.00000000000000711, 0.000000000000000000, 0.000000000000000000 ) ) ;
#17159=CARTESIAN_POINT ( 'NONE',  ( -37.00000000000000711, 0.000000000000000000, 0.000000000000000000 ) ) ;
#17160=CARTESIAN_POINT ( 'NONE',  ( -3.689171339445763032, 10.77932410358149795, 5.277713104131331434 ) ) ;
#17166=CARTESIAN_POINT ( 'NONE',  ( -24.60592215467821831, -6.662391132441423558, 9.982918610336051657 ) ) ;
#17168=EDGE_LOOP ( 'NONE', ( #16513, #34548, #44568, #40380 ) ) ;
#17169=VERTEX_POINT ( 'NONE', #37389 ) ;
#17171=CIRCLE ( 'NONE', #54351, 12.18649999999999878 ) ;
#17172=VECTOR ( 'NONE', #21049, 1000.000000000000000 ) ;
#17173=EDGE_CURVE ( 'NONE', #32750, #50873, #27739, .T. ) ;
#17174=EDGE_LOOP ( 'NONE', ( #3372, #6514, #43912, #41016 ) ) ;
#17175=CARTESIAN_POINT ( 'NONE',  ( 29.03457606387295087, -7.862146963512102182, 10.97436308512422265 ) ) ;
#17176=DIRECTION ( 'NONE',  ( -0.000000000000000000, -0.000000000000000000, -1.000000000000000000 ) ) ;
#17177=CARTESIAN_POINT ( 'NONE',  ( 11.56167612769134045, 0.7121690593505338729, 13.48138618271499745 ) ) ;
#17179=CIRCLE ( 'NONE', #55432, 12.18649999999999878 ) ;
#17180=DIRECTION ( 'NONE',  ( 0.000000000000000000, 0.5472293298355215274, -0.8369827122275381726 ) ) ;
#17181=DIRECTION ( 'NONE',  ( 0.000000000000000000, -0.01356324068817992175, 0.9999080150203990547 ) ) ;
#17182=CIRCLE ( 'NONE', #60707, 5.000000000000000888 ) ;
#17183=ADVANCED_FACE ( 'NONE', ( #27409 ), #47063, .T. ) ;
#17184=DIRECTION ( 'NONE',  ( 0.000000000000000000, -0.7790879021242573810, 0.6269146997507903940 ) ) ;
#17185=ORIENTED_EDGE ( 'NONE', *, *, #38962, .F. ) ;
#17187=EDGE_CURVE ( 'NONE', #34326, #37599, #49157, .T. ) ;
#17188=ORIENTED_EDGE ( 'NONE', *, *, #25008, .T. ) ;
#17189=CARTESIAN_POINT ( 'NONE',  ( 35.00000000000000000, 10.63508530065521640, -4.986700593229742573 ) ) ;
#17191=CARTESIAN_POINT ( 'NONE',  ( -9.316487364114289349, -12.33901589261846254, -5.488921151462630377 ) ) ;
#17195=AXIS2_PLACEMENT_3D ( 'NONE', #61440, #1618, #16884 ) ;
#17196=ORIENTED_EDGE ( 'NONE', *, *, #63421, .F. ) ;
#17198=CIRCLE ( 'NONE', #61805, 12.74999999999999822 ) ;
#17199=EDGE_LOOP ( 'NONE', ( #65126, #44906, #47605, #22192 ) ) ;
#17200=CARTESIAN_POINT ( 'NONE',  ( -29.92777678363736626, -3.750539801530011985, 11.39883551934754635 ) ) ;
#17201=EDGE_CURVE ( 'NONE', #32661, #56228, #62934, .T. ) ;
#17202=CARTESIAN_POINT ( 'NONE',  ( 8.489363379069230220, 5.256536079434125597, 10.79531771019706810 ) ) ;
#17203=AXIS2_PLACEMENT_3D ( 'NONE', #12001, #62218, #16669 ) ;
#17206=ADVANCED_FACE ( 'NONE', ( #36742 ), #16780, .T. ) ;
#17207=ORIENTED_EDGE ( 'NONE', *, *, #27126, .T. ) ;
#17209=DIRECTION ( 'NONE',  ( 1.000000000000000000, -0.000000000000000000, 0.000000000000000000 ) ) ;
#17210=VECTOR ( 'NONE', #44021, 1000.000000000000000 ) ;
#17212=DIRECTION ( 'NONE',  ( 0.000000000000000000, -1.000000000000000000, 0.000000000000000000 ) ) ;
#17213=ADVANCED_FACE ( 'NONE', ( #47705 ), #53016, .T. ) ;
#17214=ADVANCED_FACE ( 'NONE', ( #11781 ), #57036, .T. ) ;
#17216=LINE ( 'NONE', #42131, #35144 ) ;
#17217=VECTOR ( 'NONE', #7515, 1000.000000000000000 ) ;
#17219=ORIENTED_EDGE ( 'NONE', *, *, #48125, .T. ) ;
#17221=ADVANCED_FACE ( 'NONE', ( #62990 ), #52383, .T. ) ;
#17222=ORIENTED_EDGE ( 'NONE', *, *, #38128, .T. ) ;
#17223=CARTESIAN_POINT ( 'NONE',  ( -5.434714954071925064, -0.9285630528112753801, -13.46803340916659231 ) ) ;
#17225=FACE_OUTER_BOUND ( 'NONE', #5088, .T. ) ;
#17226=AXIS2_PLACEMENT_3D ( 'NONE', #49947, #33429, #64890 ) ;
#17227=DIRECTION ( 'NONE',  ( 1.000000000000000000, 0.000000000000000000, 0.000000000000000000 ) ) ;
#17228=DIRECTION ( 'NONE',  ( 1.000000000000000000, -0.000000000000000000, 0.000000000000000000 ) ) ;
#17230=ORIENTED_EDGE ( 'NONE', *, *, #61029, .F. ) ;
#17231=ORIENTED_EDGE ( 'NONE', *, *, #59094, .F. ) ;
#17234=CARTESIAN_POINT ( 'NONE',  ( 1.294038020999240590, 1.103269716799493150, 11.95280541775544592 ) ) ;
#17235=CARTESIAN_POINT ( 'NONE',  ( 1.292668453954261221, 1.054608513093608924, -13.47545724770707487 ) ) ;
#17238=DIRECTION ( 'NONE',  ( 0.000000000000000000, -0.01356324068817991828, 0.9999080150203990547 ) ) ;
#17240=CARTESIAN_POINT ( 'NONE',  ( 35.00000000000000000, 4.705694406421931860E-17, -3.469127814946512892E-15 ) ) ;
#17241=ORIENTED_EDGE ( 'NONE', *, *, #30308, .F. ) ;
#17242=VERTEX_POINT ( 'NONE', #32393 ) ;
#17245=AXIS2_PLACEMENT_3D ( 'NONE', #35773, #20511, #51108 ) ;
#17246=CARTESIAN_POINT ( 'NONE',  ( 24.82652845881425208, -10.42385221765392700, -8.578654028722157321 ) ) ;
#17248=CARTESIAN_POINT ( 'NONE',  ( 35.00000000000000000, 9.321877890560537949, 7.146664589317804683 ) ) ;
#17251=EDGE_LOOP ( 'NONE', ( #57084, #6980, #39743, #57494 ) ) ;
#17252=FACE_OUTER_BOUND ( 'NONE', #44224, .T. ) ;
#17253=VECTOR ( 'NONE', #50542, 1000.000000000000000 ) ;
#17255=CARTESIAN_POINT ( 'NONE',  ( 35.00000000000000000, 9.217970097227839332, 7.971186206369370808 ) ) ;
#17259=DIRECTION ( 'NONE',  ( 0.000000000000000000, -0.01356324068817999114, 0.9999080150203989437 ) ) ;
#17261=ORIENTED_EDGE ( 'NONE', *, *, #39669, .F. ) ;
#17262=DIRECTION ( 'NONE',  ( 0.000000000000000000, 0.1740410799127544150, 0.9847383929261631641 ) ) ;
#17266=DIRECTION ( 'NONE',  ( 0.000000000000000000, 0.9796553971857749898, 0.2006870767258855104 ) ) ;
#17267=CARTESIAN_POINT ( 'NONE',  ( -35.00000000000000000, 10.63508530065528923, -4.986700593229593359 ) ) ;
#17268=FACE_OUTER_BOUND ( 'NONE', #5822, .T. ) ;
#17269=CARTESIAN_POINT ( 'NONE',  ( -35.00000000000000000, -1.030638227056651424, 12.14284015767849567 ) ) ;
#17271=CARTESIAN_POINT ( 'NONE',  ( -37.00000000000000711, -12.05416472667164207, -1.791059740004549372 ) ) ;
#17272=VECTOR ( 'NONE', #17927, 1000.000000000000000 ) ;
#17274=CARTESIAN_POINT ( 'NONE',  ( -35.00000000000000000, 0.000000000000000000, 0.000000000000000000 ) ) ;
#17275=DIRECTION ( 'NONE',  ( 0.000000000000000000, -0.01356324068818000848, 0.9999080150203990547 ) ) ;
#17277=CIRCLE ( 'NONE', #51269, 5.000000000000001776 ) ;
#17278=DIRECTION ( 'NONE',  ( 1.000000000000000000, 0.000000000000000000, 0.000000000000000000 ) ) ;
#17280=FACE_OUTER_BOUND ( 'NONE', #11884, .T. ) ;
#17281=CIRCLE ( 'NONE', #27914, 4.999999999999999112 ) ;
#17284=CARTESIAN_POINT ( 'NONE',  ( -14.11589373245165469, 8.250315036047107142, -8.713914264323175729 ) ) ;
#17285=( BOUNDED_CURVE ( )  B_SPLINE_CURVE ( 3, ( #57237, #46281, #61544, #723 ),
 .UNSPECIFIED., .F., .F. ) 
 B_SPLINE_CURVE_WITH_KNOTS ( ( 4, 4 ),
 ( 5.023979252657118977, 5.040864206341344911 ),
 .UNSPECIFIED. ) 
 CURVE ( )  GEOMETRIC_REPRESENTATION_ITEM ( )  RATIONAL_B_SPLINE_CURVE ( ( 1.000000000000000000, 0.9999762416693727118, 0.9999762416693727118, 1.000000000000000000 ) ) 
 REPRESENTATION_ITEM ( '' )  );
#17286=VERTEX_POINT ( 'NONE', #33957 ) ;
#17287=DIRECTION ( 'NONE',  ( -1.000000000000000000, 0.000000000000000000, -0.000000000000000000 ) ) ;
#17289=CARTESIAN_POINT ( 'NONE',  ( 9.967256768512323006, -13.45016586142041959, -1.162363687967992165 ) ) ;
#17292=EDGE_LOOP ( 'NONE', ( #55282, #47623, #24904, #45673 ) ) ;
#17294=CYLINDRICAL_SURFACE ( 'NONE', #7993, 4.999999999999999112 ) ;
#17295=CARTESIAN_POINT ( 'NONE',  ( 35.00000000000000000, 3.827046518385079032, -11.56998259273179386 ) ) ;
#17296=B_SPLINE_CURVE_WITH_KNOTS ( 'NONE', 3,
 ( #47283, #1723, #21989, #22301, #32929, #17988, #18334, #32595, #38249, #43567, #2728, #38599, #27972, #43241, #18670, #52903, #2383, #59217 ),
 .UNSPECIFIED., .F., .F.,
 ( 4, 2, 2, 2, 2, 2, 2, 2, 4 ),
 ( 0.000000000000000000, 0.0008320272794029127473, 0.001664054558805825495, 0.002496081838208737917, 0.003328109117611650989, 0.004160136397014563628, 0.004992163676417476700, 0.005824190955820389773, 0.006656218235223304580 ),
 .UNSPECIFIED. ) ;
#17297=CARTESIAN_POINT ( 'NONE',  ( 35.00000000000000000, 10.99909370905164430, 5.246972444133898072 ) ) ;
#17298=CARTESIAN_POINT ( 'NONE',  ( -3.472928581034699924, 8.809056386856843446, 10.25973817351390416 ) ) ;
#17300=AXIS2_PLACEMENT_3D ( 'NONE', #48256, #18645, #38905 ) ;
#17302=DIRECTION ( 'NONE',  ( 0.000000000000000000, -0.01356324068817992175, 0.9999080150203990547 ) ) ;
#17303=VERTEX_POINT ( 'NONE', #4378 ) ;
#17305=VECTOR ( 'NONE', #20699, 1000.000000000000000 ) ;
#17306=PRODUCT_DEFINITION_CONTEXT ( 'detailed design', #12786, 'design' ) ;
#17307=CARTESIAN_POINT ( 'NONE',  ( 37.00000000000000711, -3.093009498343839869, 11.78745411414842437 ) ) ;
#17308=EDGE_CURVE ( 'NONE', #59495, #51211, #45963, .T. ) ;
#17310=ORIENTED_EDGE ( 'NONE', *, *, #8748, .T. ) ;
#17315=DIRECTION ( 'NONE',  ( -1.000000000000000000, -1.836970198721029688E-16, -0.000000000000000000 ) ) ;
#17317=ORIENTED_EDGE ( 'NONE', *, *, #12422, .T. ) ;
#17318=CIRCLE ( 'NONE', #62970, 5.000000000000000888 ) ;
#17319=VECTOR ( 'NONE', #53061, 1000.000000000000000 ) ;
#17320=EDGE_LOOP ( 'NONE', ( #59894, #19864, #9874, #55466 ) ) ;
#17324=DIRECTION ( 'NONE',  ( 1.000000000000000000, -0.000000000000000000, 0.000000000000000000 ) ) ;
#17325=EDGE_CURVE ( 'NONE', #64117, #54444, #1402, .T. ) ;
#17326=ORIENTED_EDGE ( 'NONE', *, *, #21466, .T. ) ;
#17328=DIRECTION ( 'NONE',  ( 0.000000000000000000, -0.01356324068818685717, 0.9999080150203989437 ) ) ;
#17329=EDGE_CURVE ( 'NONE', #45530, #34672, #47060, .T. ) ;
#17332=DIRECTION ( 'NONE',  ( 0.000000000000000000, 0.01356324068817992175, -0.9999080150203990547 ) ) ;
#17333=DIRECTION ( 'NONE',  ( 0.000000000000000000, 0.4134677391718512007, 0.9105187689795953832 ) ) ;
#17334=ORIENTED_EDGE ( 'NONE', *, *, #42675, .F. ) ;
#17336=ORIENTED_EDGE ( 'NONE', *, *, #21479, .F. ) ;
#17337=CARTESIAN_POINT ( 'NONE',  ( -16.98800322446194855, 2.922502605998049674, 25.00000000000000000 ) ) ;
#17338=EDGE_LOOP ( 'NONE', ( #53383, #41493, #6316, #4735 ) ) ;
#17339=DIRECTION ( 'NONE',  ( 1.000000000000000000, 0.000000000000000000, 0.000000000000000000 ) ) ;
#17341=LINE ( 'NONE', #51619, #39352 ) ;
#17343=LINE ( 'NONE', #16675, #5032 ) ;
#17346=DIRECTION ( 'NONE',  ( 1.000000000000000000, 0.000000000000000000, -0.000000000000000000 ) ) ;
#17347=CARTESIAN_POINT ( 'NONE',  ( 6.530088489467589241, -4.706431572448715350, -11.04498340397446654 ) ) ;
#17348=ORIENTED_EDGE ( 'NONE', *, *, #27310, .F. ) ;
#17349=CARTESIAN_POINT ( 'NONE',  ( -35.00000000000000000, 0.000000000000000000, 0.000000000000000000 ) ) ;
#17350=EDGE_LOOP ( 'NONE', ( #389, #37607, #20759, #61369 ) ) ;
#17351=DIRECTION ( 'NONE',  ( 0.000000000000000000, 0.01356324068818000848, -0.9999080150203990547 ) ) ;
#17352=CIRCLE ( 'NONE', #53484, 4.999999999999999112 ) ;
#17355=ADVANCED_FACE ( 'NONE', ( #24648 ), #14973, .T. ) ;
#17356=ORIENTED_EDGE ( 'NONE', *, *, #32945, .T. ) ;
#17358=DIRECTION ( 'NONE',  ( -0.000000000000000000, -1.000000000000000000, -0.000000000000000000 ) ) ;
#17361=EDGE_LOOP ( 'NONE', ( #42903, #29088, #45630, #3699 ) ) ;
#17363=ORIENTED_EDGE ( 'NONE', *, *, #7567, .T. ) ;
#17364=DIRECTION ( 'NONE',  ( 0.000000000000000000, 0.7381862504171926576, -0.6745969609292690183 ) ) ;
#17366=CARTESIAN_POINT ( 'NONE',  ( -47.00000000000000711, 0.000000000000000000, 0.000000000000000000 ) ) ;
#17367=CARTESIAN_POINT ( 'NONE',  ( -35.00000000000000000, -1.488153103997047033, 11.65150730582934102 ) ) ;
#17369=CARTESIAN_POINT ( 'NONE',  ( -18.71095331498199243, -4.888783180482830559, 10.95964276331128318 ) ) ;
#17373=DIRECTION ( 'NONE',  ( 0.000000000000000000, -0.2960891610144378849, -0.9551603052523519599 ) ) ;
#17374=EDGE_CURVE ( 'NONE', #48262, #53955, #45572, .T. ) ;
#17375=CIRCLE ( 'NONE', #58840, 12.75000000000000178 ) ;
#17376=AXIS2_PLACEMENT_3D ( 'NONE', #36450, #41761, #42726 ) ;
#17377=EDGE_CURVE ( 'NONE', #55094, #23142, #33233, .T. ) ;
#17378=CARTESIAN_POINT ( 'NONE',  ( -27.45775109278350712, -13.35262336282553441, -1.989333891161978674 ) ) ;
#17379=DIRECTION ( 'NONE',  ( -1.000000000000000000, 0.000000000000000000, 0.000000000000000000 ) ) ;
#17380=VECTOR ( 'NONE', #25874, 1000.000000000000000 ) ;
#17381=CARTESIAN_POINT ( 'NONE',  ( -36.00000000000000711, 10.02106554660708859, 7.882940143791811849 ) ) ;
#17383=DIRECTION ( 'NONE',  ( -1.000000000000000000, -0.000000000000000000, 0.000000000000000000 ) ) ;
#17384=FACE_OUTER_BOUND ( 'NONE', #23870, .T. ) ;
#17386=AXIS2_PLACEMENT_3D ( 'NONE', #19506, #34759, #55061 ) ;
#17387=AXIS2_PLACEMENT_3D ( 'NONE', #26387, #46670, #36694 ) ;
#17388=EDGE_LOOP ( 'NONE', ( #15664, #9294, #15283, #45165 ) ) ;
#17390=CARTESIAN_POINT ( 'NONE',  ( 4.038317478791936033, -10.40617629760990859, 8.603232183407900635 ) ) ;
#17393=DIRECTION ( 'NONE',  ( -1.000000000000000000, -0.000000000000000000, 0.000000000000000000 ) ) ;
#17394=AXIS2_PLACEMENT_3D ( 'NONE', #22163, #57769, #43763 ) ;
#17395=ORIENTED_EDGE ( 'NONE', *, *, #35412, .T. ) ;
#17397=VERTEX_POINT ( 'NONE', #19676 ) ;
#17398=FACE_OUTER_BOUND ( 'NONE', #54858, .T. ) ;
#17399=ORIENTED_EDGE ( 'NONE', *, *, #12828, .F. ) ;
#17400=ORIENTED_EDGE ( 'NONE', *, *, #38317, .F. ) ;
#17401=CARTESIAN_POINT ( 'NONE',  ( -35.00000000000000000, 11.50504120060943158, 4.018060380616439886 ) ) ;
#17402=CIRCLE ( 'NONE', #55623, 12.75000000000000178 ) ;
#17404=CARTESIAN_POINT ( 'NONE',  ( -27.27855387000350262, -10.59660315834921107, 5.631341004100471892 ) ) ;
#17406=DIRECTION ( 'NONE',  ( 0.000000000000000000, 0.01356324068817992175, -0.9999080150203990547 ) ) ;
#17407=FACE_OUTER_BOUND ( 'NONE', #21846, .T. ) ;
#17408=EDGE_CURVE ( 'NONE', #42135, #35454, #9868, .T. ) ;
#17409=ORIENTED_EDGE ( 'NONE', *, *, #42067, .F. ) ;
#17410=CARTESIAN_POINT ( 'NONE',  ( -35.00000000000000000, 5.015831474386455824, -10.62137734850263016 ) ) ;
#17412=CARTESIAN_POINT ( 'NONE',  ( -2.952869152607111136, 4.384817011589738911, 11.17020052527586138 ) ) ;
#17413=LINE ( 'NONE', #37689, #52085 ) ;
#17414=ORIENTED_EDGE ( 'NONE', *, *, #27685, .T. ) ;
#17415=DIRECTION ( 'NONE',  ( 1.000000000000000000, 0.000000000000000000, -0.000000000000000000 ) ) ;
#17416=VERTEX_POINT ( 'NONE', #3748 ) ;
#17418=AXIS2_PLACEMENT_3D ( 'NONE', #64424, #9219, #29502 ) ;
#17421=CARTESIAN_POINT ( 'NONE',  ( -35.00000000000000000, -12.68495603654570836, -1.286231064351444742 ) ) ;
#17423=DIRECTION ( 'NONE',  ( 0.000000000000000000, 0.01356324068817998940, -0.9999080150203990547 ) ) ;
#17424=ORIENTED_EDGE ( 'NONE', *, *, #31435, .F. ) ;
#17426=CARTESIAN_POINT ( 'NONE',  ( -35.00000000000000000, -8.146229107149334681, -9.063649021439044162 ) ) ;
#17429=ORIENTED_EDGE ( 'NONE', *, *, #60292, .F. ) ;
#17430=AXIS2_PLACEMENT_3D ( 'NONE', #12777, #42058, #32409 ) ;
#17432=CARTESIAN_POINT ( 'NONE',  ( -36.00000000000000711, 12.08151691381196002, -4.074242145635880163 ) ) ;
#17433=ORIENTED_EDGE ( 'NONE', *, *, #22048, .T. ) ;
#17434=B_SPLINE_CURVE_WITH_KNOTS ( 'NONE', 3,
 ( #46208, #20909, #56499, #41183, #61465, #31230, #53146, #6292, #47832, #27534, #16594, #41854 ),
 .UNSPECIFIED., .F., .F.,
 ( 4, 2, 2, 2, 2, 4 ),
 ( 2.693015029076738270E-17, 0.002303342557757002800, 0.004606685115513976109, 0.005758356394392463197, 0.006910027673270949418, 0.009213370231027924462 ),
 .UNSPECIFIED. ) ;
#17435=ORIENTED_EDGE ( 'NONE', *, *, #9364, .F. ) ;
#17436=AXIS2_PLACEMENT_3D ( 'NONE', #6480, #51718, #26758 ) ;
#17437=DIRECTION ( 'NONE',  ( 0.000000000000000000, 0.000000000000000000, -1.000000000000000000 ) ) ;
#17438=CARTESIAN_POINT ( 'NONE',  ( 35.00000000000000000, -7.110831038798346881, -9.896810808925367908 ) ) ;
#17439=CARTESIAN_POINT ( 'NONE',  ( 35.00000000000000000, 4.705694406421931860E-17, -3.469127814946512892E-15 ) ) ;
#17442=AXIS2_PLACEMENT_3D ( 'NONE', #6177, #27104, #17120 ) ;
#17443=CARTESIAN_POINT ( 'NONE',  ( -37.00000000000000711, 11.42599468261435192, -4.237620530777677530 ) ) ;
#17444=DIRECTION ( 'NONE',  ( 0.000000000000000000, 0.9970832820307041766, 0.07632122047556146038 ) ) ;
#17445=VERTEX_POINT ( 'NONE', #21956 ) ;
#17446=AXIS2_PLACEMENT_3D ( 'NONE', #4509, #35391, #10784 ) ;
#17448=CARTESIAN_POINT ( 'NONE',  ( 47.00000000000000711, 4.705694406421931860E-17, -3.469127814946512892E-15 ) ) ;
#17449=EDGE_CURVE ( 'NONE', #50524, #14759, #36594, .T. ) ;
#17451=CARTESIAN_POINT ( 'NONE',  ( -35.00000000000000000, 0.000000000000000000, 0.000000000000000000 ) ) ;
#17452=AXIS2_PLACEMENT_3D ( 'NONE', #45556, #44909, #60868 ) ;
#17453=CARTESIAN_POINT ( 'NONE',  ( -35.00000000000000000, 0.000000000000000000, 0.000000000000000000 ) ) ;
#17454=DIRECTION ( 'NONE',  ( -1.000000000000000000, 0.000000000000000000, -0.000000000000000000 ) ) ;
#17455=CARTESIAN_POINT ( 'NONE',  ( 12.52750123246316072, 0.4973700281276248192, -11.98968819674306374 ) ) ;
#17456=ORIENTED_EDGE ( 'NONE', *, *, #16718, .T. ) ;
#17457=CARTESIAN_POINT ( 'NONE',  ( -34.00000000000000000, 1.836970198721035357E-16, 0.000000000000000000 ) ) ;
#17458=AXIS2_PLACEMENT_3D ( 'NONE', #60653, #60320, #15091 ) ;
#17459=DIRECTION ( 'NONE',  ( -1.000000000000000000, 0.000000000000000000, 0.000000000000000000 ) ) ;
#17460=CARTESIAN_POINT ( 'NONE',  ( 35.00000000000000000, 7.745827850123149005, 10.12742074351887744 ) ) ;
#17461=AXIS2_PLACEMENT_3D ( 'NONE', #42453, #11563, #31836 ) ;
#17462=CARTESIAN_POINT ( 'NONE',  ( -17.72811806012732916, -13.27197368940280064, 2.555533621652877230 ) ) ;
#17464=CARTESIAN_POINT ( 'NONE',  ( -25.27881376661855484, 6.347467180810850707, 10.18972282614729608 ) ) ;
#17465=CARTESIAN_POINT ( 'NONE',  ( -25.80019021537189516, -11.91931523669747151, 6.339780118509601436 ) ) ;
#17466=ORIENTED_EDGE ( 'NONE', *, *, #60136, .T. ) ;
#17468=CARTESIAN_POINT ( 'NONE',  ( -37.00000000000000711, -11.23004253107761130, -4.732539170486383284 ) ) ;
#17469=CARTESIAN_POINT ( 'NONE',  ( -37.00000000000000711, -4.545979934229493757, 11.30684963584387859 ) ) ;
#17471=ORIENTED_EDGE ( 'NONE', *, *, #20317, .F. ) ;
#17472=CARTESIAN_POINT ( 'NONE',  ( 23.57978631083511445, 11.05404059788998161, -7.754718420896370645 ) ) ;
#17473=CARTESIAN_POINT ( 'NONE',  ( 37.00000000000000711, 11.72397916322012179, -0.7214809346829029746 ) ) ;
#17474=VERTEX_POINT ( 'NONE', #6030 ) ;
#17476=DIRECTION ( 'NONE',  ( 0.000000000000000000, -0.01356324068817999114, 0.9999080150203989437 ) ) ;
#17477=AXIS2_PLACEMENT_3D ( 'NONE', #34147, #3613, #38827 ) ;
#17478=CIRCLE ( 'NONE', #34459, 12.74999999999999822 ) ;
#17479=DIRECTION ( 'NONE',  ( 0.000000000000000000, 0.01356324068817991481, -0.9999080150203990547 ) ) ;
#17480=ORIENTED_EDGE ( 'NONE', *, *, #140, .F. ) ;
#17483=CARTESIAN_POINT ( 'NONE',  ( -37.00000000000000711, 8.927548052241016663, -8.295159312811756891 ) ) ;
#17487=DIRECTION ( 'NONE',  ( -1.000000000000000000, 0.000000000000000000, 0.000000000000000000 ) ) ;
#17489=DIRECTION ( 'NONE',  ( -1.000000000000000000, -0.000000000000000000, 0.000000000000000000 ) ) ;
#17490=VERTEX_POINT ( 'NONE', #62187 ) ;
#17491=EDGE_CURVE ( 'NONE', #54227, #17416, #15187, .T. ) ;
#17492=DIRECTION ( 'NONE',  ( -1.000000000000000000, 0.000000000000000000, 0.000000000000000000 ) ) ;
#17493=ORIENTED_EDGE ( 'NONE', *, *, #18400, .F. ) ;
#17494=DIRECTION ( 'NONE',  ( -1.000000000000000000, 0.000000000000000000, 0.000000000000000000 ) ) ;
#17495=ORIENTED_EDGE ( 'NONE', *, *, #8361, .F. ) ;
#17500=CARTESIAN_POINT ( 'NONE',  ( -17.16655223576323408, 3.059552638032528638, 11.60427096643701361 ) ) ;
#17501=VECTOR ( 'NONE', #40829, 1000.000000000000000 ) ;
#17502=EDGE_CURVE ( 'NONE', #4318, #4780, #33804, .T. ) ;
#17504=CARTESIAN_POINT ( 'NONE',  ( -28.85619398320021745, 3.750539801530000439, 25.00000000000000000 ) ) ;
#17505=ORIENTED_EDGE ( 'NONE', *, *, #12828, .T. ) ;
#17507=CARTESIAN_POINT ( 'NONE',  ( 3.154808525168153022, 2.889958543828632820, -13.21403070427456505 ) ) ;
#17508=EDGE_CURVE ( 'NONE', #38941, #51664, #36909, .T. ) ;
#17509=EDGE_LOOP ( 'NONE', ( #37193, #1906, #18851, #20630 ) ) ;
#17510=EDGE_LOOP ( 'NONE', ( #48559, #57136, #22654, #34618 ) ) ;
#17512=EDGE_CURVE ( 'NONE', #1280, #27364, #37498, .T. ) ;
#17515=CARTESIAN_POINT ( 'NONE',  ( 37.00000000000000711, -11.78745411414841726, -3.093009498343884722 ) ) ;
#17517=CARTESIAN_POINT ( 'NONE',  ( 35.00000000000000000, 7.215058775251253387, -9.821084925794595577 ) ) ;
#17520=CARTESIAN_POINT ( 'NONE',  ( -28.82752767077929335, 2.766519351427261686, 13.23585947174678701 ) ) ;
#17522=DIRECTION ( 'NONE',  ( 1.000000000000000000, 0.000000000000000000, 0.000000000000000000 ) ) ;
#17525=CARTESIAN_POINT ( 'NONE',  ( -35.00000000000000000, 10.84030624090606487, 6.711949091238180287 ) ) ;
#17530=VECTOR ( 'NONE', #57254, 1000.000000000000000 ) ;
#17531=CARTESIAN_POINT ( 'NONE',  ( -35.00000000000000000, -5.710938531231627202, -11.39945968423477751 ) ) ;
#17533=AXIS2_PLACEMENT_3D ( 'NONE', #48996, #18411, #3453 ) ;
#17534=ORIENTED_EDGE ( 'NONE', *, *, #36728, .T. ) ;
#17535=VERTEX_POINT ( 'NONE', #6673 ) ;
#17537=ORIENTED_EDGE ( 'NONE', *, *, #31386, .F. ) ;
#17539=DIRECTION ( 'NONE',  ( -1.000000000000000000, 0.000000000000000000, 0.000000000000000000 ) ) ;
#17540=CARTESIAN_POINT ( 'NONE',  ( -35.00000000000000000, 0.000000000000000000, 0.000000000000000000 ) ) ;
#17544=CARTESIAN_POINT ( 'NONE',  ( 18.31509512384567273, 9.277234456363913750, 9.833198574146647886 ) ) ;
#17554=CARTESIAN_POINT ( 'NONE',  ( 35.00000000000000000, 4.705694406421931860E-17, -3.469127814946512892E-15 ) ) ;
#17555=ORIENTED_EDGE ( 'NONE', *, *, #4952, .T. ) ;
#17556=CARTESIAN_POINT ( 'NONE',  ( -11.40165637463000436, -7.508992741355388745, -9.360289953322599388 ) ) ;
#17557=LINE ( 'NONE', #52795, #27824 ) ;
#17558=CYLINDRICAL_SURFACE ( 'NONE', #57459, 12.75000000000000178 ) ;
#17565=CARTESIAN_POINT ( 'NONE',  ( -35.00000000000000000, 0.7008968033238767159, 12.16632754454236931 ) ) ;
#17567=DIRECTION ( 'NONE',  ( 0.000000000000000000, 0.01356324068817998940, -0.9999080150203989437 ) ) ;
#17569=AXIS2_PLACEMENT_3D ( 'NONE', #6671, #41563, #10995 ) ;
#17570=CARTESIAN_POINT ( 'NONE',  ( 35.00000000000000000, -6.917234959366766134, 9.493370459201765144 ) ) ;
#17573=EDGE_CURVE ( 'NONE', #32993, #23409, #52428, .T. ) ;
#17575=CARTESIAN_POINT ( 'NONE',  ( 145.1370849898475797, 3.309064568108273190E-14, 0.000000000000000000 ) ) ;
#17576=ORIENTED_EDGE ( 'NONE', *, *, #13485, .T. ) ;
#17578=VERTEX_POINT ( 'NONE', #17948 ) ;
#17580=ORIENTED_EDGE ( 'NONE', *, *, #9714, .F. ) ;
#17581=VECTOR ( 'NONE', #42401, 1000.000000000000000 ) ;
#17582=CARTESIAN_POINT ( 'NONE',  ( 35.00000000000000000, -0.2661492558802491248, 12.18359334611896116 ) ) ;
#17584=EDGE_CURVE ( 'NONE', #57334, #23325, #40730, .T. ) ;
#17585=CARTESIAN_POINT ( 'NONE',  ( 36.00000000000000711, 11.32068061209303345, 5.865551165830958702 ) ) ;
#17586=ORIENTED_EDGE ( 'NONE', *, *, #56934, .T. ) ;
#17590=EDGE_CURVE ( 'NONE', #20923, #51040, #1999, .T. ) ;
#17592=ORIENTED_EDGE ( 'NONE', *, *, #29363, .T. ) ;
#17593=LINE ( 'NONE', #33532, #26835 ) ;
#17595=VERTEX_POINT ( 'NONE', #47554 ) ;
#17597=ORIENTED_EDGE ( 'NONE', *, *, #29566, .T. ) ;
#17598=ORIENTED_EDGE ( 'NONE', *, *, #17374, .F. ) ;
#17599=EDGE_CURVE ( 'NONE', #4304, #52011, #5336, .T. ) ;
#17600=DIRECTION ( 'NONE',  ( 1.836970198721029688E-16, -1.000000000000000000, 0.000000000000000000 ) ) ;
#17601=CARTESIAN_POINT ( 'NONE',  ( -27.01437459610461644, -13.31613970204372421, -2.220455681983950935 ) ) ;
#17602=CIRCLE ( 'NONE', #65362, 12.75000000000000178 ) ;
#17603=DIRECTION ( 'NONE',  ( -1.000000000000000000, 0.000000000000000000, 0.000000000000000000 ) ) ;
#17604=CYLINDRICAL_SURFACE ( 'NONE', #57468, 5.000000000000000888 ) ;
#17608=CARTESIAN_POINT ( 'NONE',  ( -35.00000000000000000, -10.54834585426215732, -6.102719229070786788 ) ) ;
#17610=VERTEX_POINT ( 'NONE', #58188 ) ;
#17613=EDGE_CURVE ( 'NONE', #17080, #55989, #2687, .T. ) ;
#17614=LINE ( 'NONE', #12586, #61831 ) ;
#17615=CARTESIAN_POINT ( 'NONE',  ( 29.61270049156755135, 5.476238065135014210, 10.68911382491602424 ) ) ;
#17616=LINE ( 'NONE', #12935, #10617 ) ;
#17619=CARTESIAN_POINT ( 'NONE',  ( 37.00000000000000711, 5.143145423404281047, -11.66664283989682005 ) ) ;
#17621=ORIENTED_EDGE ( 'NONE', *, *, #48313, .T. ) ;
#17622=CARTESIAN_POINT ( 'NONE',  ( -37.00000000000000711, 0.000000000000000000, 0.000000000000000000 ) ) ;
#17623=AXIS2_PLACEMENT_3D ( 'NONE', #51733, #848, #61678 ) ;
#17624=ORIENTED_EDGE ( 'NONE', *, *, #20881, .F. ) ;
#17625=CARTESIAN_POINT ( 'NONE',  ( -35.00000000000000000, 6.950793414699794504, 10.68873102412845100 ) ) ;
#17627=DIRECTION ( 'NONE',  ( 1.000000000000000000, 0.000000000000000000, 0.000000000000000000 ) ) ;
#17630=ORIENTED_EDGE ( 'NONE', *, *, #16454, .F. ) ;
#17633=CARTESIAN_POINT ( 'NONE',  ( -3.757056674316401779, 9.653459166343935749, 9.445297855425245359 ) ) ;
#17635=EDGE_CURVE ( 'NONE', #38476, #10194, #12051, .T. ) ;
#17636=EDGE_CURVE ( 'NONE', #55391, #26236, #42808, .T. ) ;
#17638=ORIENTED_EDGE ( 'NONE', *, *, #15589, .F. ) ;
#17640=CARTESIAN_POINT ( 'NONE',  ( 3.291290029914074378, 8.250315036047103590, -8.713914264323182834 ) ) ;
#17641=EDGE_CURVE ( 'NONE', #37431, #40269, #43201, .T. ) ;
#17642=EDGE_CURVE ( 'NONE', #16592, #60501, #60905, .T. ) ;
#17643=ORIENTED_EDGE ( 'NONE', *, *, #47390, .F. ) ;
#17644=CARTESIAN_POINT ( 'NONE',  ( 10.22196962362456851, 7.431669770566725397, -9.426540164465942340 ) ) ;
#17645=VERTEX_POINT ( 'NONE', #17297 ) ;
#17646=DIRECTION ( 'NONE',  ( -1.000000000000000000, 0.000000000000000000, 0.000000000000000000 ) ) ;
#17647=FACE_OUTER_BOUND ( 'NONE', #22386, .T. ) ;
#17648=DIRECTION ( 'NONE',  ( 1.000000000000000000, 0.000000000000000000, 0.000000000000000000 ) ) ;
#17649=CARTESIAN_POINT ( 'NONE',  ( -35.00000000000000000, -8.624332853796127907, 9.390600770287958809 ) ) ;
#17654=B_SPLINE_CURVE_WITH_KNOTS ( 'NONE', 3,
 ( #65075, #45447, #50134, #60416, #4588, #56082, #35128, #55439, #30164, #9212, #45787, #25497, #14518, #10204, #29497, #44793, #9876, #20842, #50780, #24516, #19550, #5229, #250, #20523 ),
 .UNSPECIFIED., .F., .F.,
 ( 4, 2, 2, 2, 2, 2, 2, 2, 2, 2, 2, 4 ),
 ( 2.168404344971008868E-19, 0.001212199945010031558, 0.001818299917515049614, 0.002424399890020067887, 0.003030499862525085943, 0.003636599835030103998, 0.004848799780040138376, 0.005454899752545154697, 0.006060999725050171018, 0.007273199670060210599, 0.008485399615070249313, 0.009697599560080288894 ),
 .UNSPECIFIED. ) ;
#17655=ORIENTED_EDGE ( 'NONE', *, *, #35908, .F. ) ;
#17656=CARTESIAN_POINT ( 'NONE',  ( 37.00000000000000711, 4.705694406421931860E-17, -3.469127814946512892E-15 ) ) ;
#17660=DIRECTION ( 'NONE',  ( -1.000000000000000000, 0.000000000000000000, -0.000000000000000000 ) ) ;
#17662=ORIENTED_EDGE ( 'NONE', *, *, #14697, .F. ) ;
#17663=VECTOR ( 'NONE', #62332, 1000.000000000000000 ) ;
#17666=ADVANCED_FACE ( 'NONE', ( #59178 ), #2341, .T. ) ;
#17669=EDGE_LOOP ( 'NONE', ( #29248, #11105, #29572, #43057 ) ) ;
#17672=EDGE_LOOP ( 'NONE', ( #60529, #57729, #29629, #62869 ) ) ;
#17675=EDGE_CURVE ( 'NONE', #47279, #9626, #20564, .T. ) ;
#17676=CYLINDRICAL_SURFACE ( 'NONE', #5457, 12.18649999999999878 ) ;
#17677=DIRECTION ( 'NONE',  ( 1.000000000000000000, 0.000000000000000000, 0.000000000000000000 ) ) ;
#17679=FACE_OUTER_BOUND ( 'NONE', #48438, .T. ) ;
#17680=CYLINDRICAL_SURFACE ( 'NONE', #9025, 4.999999999999999112 ) ;
#17681=CARTESIAN_POINT ( 'NONE',  ( -35.00000000000000000, -10.30098186818253758, 5.644643009979033899 ) ) ;
#17684=CYLINDRICAL_SURFACE ( 'NONE', #21582, 12.18650000000000055 ) ;
#17689=EDGE_CURVE ( 'NONE', #21896, #20774, #58798, .T. ) ;
#17690=VERTEX_POINT ( 'NONE', #32886 ) ;
#17691=DIRECTION ( 'NONE',  ( 0.000000000000000000, 0.01356324068818000848, -0.9999080150203990547 ) ) ;
#17694=B_SPLINE_CURVE_WITH_KNOTS ( 'NONE', 3,
 ( #25286, #17, #55221, #28980, #39602, #60874, #20301, #4369 ),
 .UNSPECIFIED., .F., .F.,
 ( 4, 2, 2, 4 ),
 ( 0.000000000000000000, 0.002295434919525721467, 0.003443152379288585020, 0.004590869839051449006 ),
 .UNSPECIFIED. ) ;
#17695=VERTEX_POINT ( 'NONE', #43524 ) ;
#17696=ORIENTED_EDGE ( 'NONE', *, *, #7585, .F. ) ;
#17697=LINE ( 'NONE', #57611, #47101 ) ;
#17698=ORIENTED_EDGE ( 'NONE', *, *, #58178, .T. ) ;
#17702=DIRECTION ( 'NONE',  ( 1.000000000000000000, 0.000000000000000000, 0.000000000000000000 ) ) ;
#17704=AXIS2_PLACEMENT_3D ( 'NONE', #15368, #15027, #5746 ) ;
#17708=EDGE_CURVE ( 'NONE', #817, #3673, #25953, .T. ) ;
#17710=CARTESIAN_POINT ( 'NONE',  ( -28.41827485489077532, 3.509237424706437292, 11.47541949982830722 ) ) ;
#17715=EDGE_CURVE ( 'NONE', #8013, #54679, #64080, .T. ) ;
#17716=ORIENTED_EDGE ( 'NONE', *, *, #64580, .F. ) ;
#17722=ORIENTED_EDGE ( 'NONE', *, *, #60671, .F. ) ;
#17724=CARTESIAN_POINT ( 'NONE',  ( -37.00000000000000711, 6.657191900728318679, 9.677500615117924809 ) ) ;
#17729=VERTEX_POINT ( 'NONE', #35174 ) ;
#17730=CARTESIAN_POINT ( 'NONE',  ( -35.00000000000000000, -10.25474254703948418, -6.584150480049660636 ) ) ;
#17731=ADVANCED_FACE ( 'NONE', ( #55480 ), #34536, .T. ) ;
#17735=DIRECTION ( 'NONE',  ( -1.000000000000000000, 0.000000000000000000, -0.000000000000000000 ) ) ;
#17736=CARTESIAN_POINT ( 'NONE',  ( -35.00000000000000000, 0.000000000000000000, 0.000000000000000000 ) ) ;
#17739=EDGE_LOOP ( 'NONE', ( #54341, #974, #62245, #31885 ) ) ;
#17740=DIRECTION ( 'NONE',  ( 0.000000000000000000, -0.01356324068817992175, 0.9999080150203990547 ) ) ;
#17741=DIRECTION ( 'NONE',  ( 0.000000000000000000, 0.01356324068817999808, -0.9999080150203990547 ) ) ;
#17744=CYLINDRICAL_SURFACE ( 'NONE', #61761, 5.000000000000000888 ) ;
#17745=ORIENTED_EDGE ( 'NONE', *, *, #58602, .T. ) ;
#17748=AXIS2_PLACEMENT_3D ( 'NONE', #20692, #737, #41278 ) ;
#17749=LINE ( 'NONE', #53327, #51828 ) ;
#17750=FACE_OUTER_BOUND ( 'NONE', #28747, .T. ) ;
#17751=EDGE_CURVE ( 'NONE', #53297, #46246, #6756, .T. ) ;
#17752=CARTESIAN_POINT ( 'NONE',  ( -35.00000000000000000, 5.246972444134173408, -10.99909370905151995 ) ) ;
#17753=CARTESIAN_POINT ( 'NONE',  ( -35.00000000000000000, -9.063649021439015740, 8.146229107149364879 ) ) ;
#17756=CARTESIAN_POINT ( 'NONE',  ( 13.22184092363782604, 12.92131670040196134, -3.916134364945811352 ) ) ;
#17760=CARTESIAN_POINT ( 'NONE',  ( 35.00000000000000000, 4.705694406421931860E-17, -3.469127814946512892E-15 ) ) ;
#17761=ORIENTED_EDGE ( 'NONE', *, *, #1083, .T. ) ;
#17763=EDGE_LOOP ( 'NONE', ( #21811, #26910, #49634, #57538 ) ) ;
#17764=CARTESIAN_POINT ( 'NONE',  ( -37.00000000000000711, 0.000000000000000000, 0.000000000000000000 ) ) ;
#17768=DIRECTION ( 'NONE',  ( -0.000000000000000000, -1.000000000000000000, -0.000000000000000000 ) ) ;
#17770=CARTESIAN_POINT ( 'NONE',  ( 47.00000000000000711, 4.705694406421931860E-17, -3.469127814946512892E-15 ) ) ;
#17771=ORIENTED_EDGE ( 'NONE', *, *, #42094, .T. ) ;
#17773=CARTESIAN_POINT ( 'NONE',  ( -17.14223920962179548, -7.219260785924160650, 11.41241003048411429 ) ) ;
#17774=CARTESIAN_POINT ( 'NONE',  ( 35.00000000000000000, 4.705694406421931860E-17, -3.469127814946512892E-15 ) ) ;
#17775=CARTESIAN_POINT ( 'NONE',  ( -35.00000000000000000, -5.644643009978993931, -10.30098186818255890 ) ) ;
#17776=EDGE_CURVE ( 'NONE', #6781, #11746, #30094, .T. ) ;
#17780=CARTESIAN_POINT ( 'NONE',  ( 37.00000000000000711, 4.705694406421931860E-17, -3.469127814946512892E-15 ) ) ;
#17784=AXIS2_PLACEMENT_3D ( 'NONE', #12573, #48202, #26913 ) ;
#17785=CIRCLE ( 'NONE', #58142, 12.18650000000000233 ) ;
#17788=CARTESIAN_POINT ( 'NONE',  ( 35.00000000000000000, -12.57916205664482590, -2.080187960898520316 ) ) ;
#17789=EDGE_LOOP ( 'NONE', ( #34487, #47670, #35636, #35688 ) ) ;
#17790=CARTESIAN_POINT ( 'NONE',  ( -25.86628395826706850, 25.00000000000000000, 10.84354029019568522 ) ) ;
#17791=CARTESIAN_POINT ( 'NONE',  ( 35.00000000000000000, 12.74921544981110877, -0.1414404973752607098 ) ) ;
#17793=ORIENTED_EDGE ( 'NONE', *, *, #1398, .T. ) ;
#17796=ORIENTED_EDGE ( 'NONE', *, *, #48916, .F. ) ;
#17797=EDGE_CURVE ( 'NONE', #886, #24291, #3969, .T. ) ;
#17799=DIRECTION ( 'NONE',  ( 1.000000000000000000, 0.000000000000000000, 0.000000000000000000 ) ) ;
#17800=ADVANCED_FACE ( 'NONE', ( #9253 ), #29535, .T. ) ;
#17801=DIRECTION ( 'NONE',  ( 1.000000000000000000, 1.836970198721029688E-16, 0.000000000000000000 ) ) ;
#17803=DIRECTION ( 'NONE',  ( 1.000000000000000000, 0.000000000000000000, 0.000000000000000000 ) ) ;
#17804=DIRECTION ( 'NONE',  ( -1.000000000000000000, 0.000000000000000000, 0.000000000000000000 ) ) ;
#17807=CARTESIAN_POINT ( 'NONE',  ( -27.01437459610461644, 8.723448335974111956, -8.240233560378637634 ) ) ;
#17809=CARTESIAN_POINT ( 'NONE',  ( -2.672254813960866393, 12.91372982010633841, 3.936302266217769130 ) ) ;
#17810=VERTEX_POINT ( 'NONE', #41148 ) ;
#17812=ORIENTED_EDGE ( 'NONE', *, *, #22635, .F. ) ;
#17814=ORIENTED_EDGE ( 'NONE', *, *, #25069, .T. ) ;
#17816=CARTESIAN_POINT ( 'NONE',  ( -16.44683101004208581, 8.250250954730093511, 10.68587204513299582 ) ) ;
#17820=CARTESIAN_POINT ( 'NONE',  ( -24.45674484725088149, 9.483701336929913239, 9.615580680626223398 ) ) ;
#17822=CARTESIAN_POINT ( 'NONE',  ( 22.88594695219327235, 3.421158645304719137, 13.05931366970166962 ) ) ;
#17824=CARTESIAN_POINT ( 'NONE',  ( -25.60701309404801052, -10.48086169146383106, 5.846161800792287977 ) ) ;
#17825=CARTESIAN_POINT ( 'NONE',  ( 1.019420486327238695, 0.09895457231945321841, -13.50926513763734960 ) ) ;
#17831=FACE_OUTER_BOUND ( 'NONE', #57690, .T. ) ;
#17832=CIRCLE ( 'NONE', #16727, 4.999999999999999112 ) ;
#17834=DIRECTION ( 'NONE',  ( 0.000000000000000000, 0.01356324068817998593, -0.9999080150203990547 ) ) ;
#17835=LINE ( 'NONE', #7871, #2947 ) ;
#17836=ADVANCED_FACE ( 'NONE', ( #61769 ), #56817, .T. ) ;
#17838=DIRECTION ( 'NONE',  ( 1.000000000000000000, 0.000000000000000000, -0.000000000000000000 ) ) ;
#17839=AXIS2_PLACEMENT_3D ( 'NONE', #54186, #53204, #63486 ) ;
#17840=CARTESIAN_POINT ( 'NONE',  ( -7.389643752995853632, -8.206056478905798812, -10.72177447465197275 ) ) ;
#17841=ORIENTED_EDGE ( 'NONE', *, *, #22989, .T. ) ;
#17843=EDGE_LOOP ( 'NONE', ( #3741, #40603, #26148, #53632 ) ) ;
#17844=CARTESIAN_POINT ( 'NONE',  ( -9.248427021356883770, -11.50593189300519725, -7.070361659645593377 ) ) ;
#17845=DIRECTION ( 'NONE',  ( -0.000000000000000000, -1.000000000000000000, -0.000000000000000000 ) ) ;
#17847=CARTESIAN_POINT ( 'NONE',  ( -10.48620311856347875, -9.720786832536937538, 7.036071585506805448 ) ) ;
#17848=ORIENTED_EDGE ( 'NONE', *, *, #62711, .T. ) ;
#17849=ORIENTED_EDGE ( 'NONE', *, *, #28974, .F. ) ;
#17850=DIRECTION ( 'NONE',  ( 0.000000000000000000, -0.01356324068817998940, 0.9999080150203990547 ) ) ;
#17851=EDGE_CURVE ( 'NONE', #40103, #6736, #54514, .T. ) ;
#17856=EDGE_CURVE ( 'NONE', #17595, #31528, #11238, .T. ) ;
#17861=CARTESIAN_POINT ( 'NONE',  ( -29.11945779004042478, 1.962419008656826502, -13.36268013567996604 ) ) ;
#17863=AXIS2_PLACEMENT_3D ( 'NONE', #43842, #64432, #8920 ) ;
#17867=CIRCLE ( 'NONE', #15761, 5.000000000000001776 ) ;
#17868=( BOUNDED_CURVE ( )  B_SPLINE_CURVE ( 3, ( #45811, #40827, #10225, #40481 ),
 .UNSPECIFIED., .F., .F. ) 
 B_SPLINE_CURVE_WITH_KNOTS ( ( 4, 4 ),
 ( 4.993910677237380469, 5.028906353039236166 ),
 .UNSPECIFIED. ) 
 CURVE ( )  GEOMETRIC_REPRESENTATION_ITEM ( )  RATIONAL_B_SPLINE_CURVE ( ( 1.000000000000000000, 0.9998979444935354177, 0.9998979444935354177, 1.000000000000000000 ) ) 
 REPRESENTATION_ITEM ( '' )  );
#17869=EDGE_LOOP ( 'NONE', ( #14869, #62201, #57968, #13094 ) ) ;
#17872=DIRECTION ( 'NONE',  ( 1.000000000000000000, 0.000000000000000000, 0.000000000000000000 ) ) ;
#17873=CARTESIAN_POINT ( 'NONE',  ( -36.00000000000000711, -4.074242145635922796, -12.08151691381194581 ) ) ;
#17874=ORIENTED_EDGE ( 'NONE', *, *, #50463, .F. ) ;
#17875=AXIS2_PLACEMENT_3D ( 'NONE', #19063, #38016, #23394 ) ;
#17876=CARTESIAN_POINT ( 'NONE',  ( -11.31210385045561573, -8.611009510439803449, -8.362799969824267876 ) ) ;
#17877=DIRECTION ( 'NONE',  ( 0.000000000000000000, -0.01356324068817991828, 0.9999080150203990547 ) ) ;
#17878=DIRECTION ( 'NONE',  ( -1.000000000000000000, 0.000000000000000000, 0.000000000000000000 ) ) ;
#17879=EDGE_CURVE ( 'NONE', #58222, #40199, #22661, .T. ) ;
#17881=CARTESIAN_POINT ( 'NONE',  ( -30.04210686634944949, 0.3871513321129805840, -13.50186640917502245 ) ) ;
#17883=ORIENTED_EDGE ( 'NONE', *, *, #9179, .F. ) ;
#17884=FACE_BOUND ( 'NONE', #25397, .T. ) ;
#17885=ORIENTED_EDGE ( 'NONE', *, *, #60127, .F. ) ;
#17886=CARTESIAN_POINT ( 'NONE',  ( -36.00000000000000711, 5.143145423404448913, -11.66664283989674367 ) ) ;
#17889=PLANE ( 'NONE',  #30122 ) ;
#17890=DIRECTION ( 'NONE',  ( 0.000000000000000000, -0.6478160128811839558, 0.7617968321374970486 ) ) ;
#17892=DIRECTION ( 'NONE',  ( -1.000000000000000000, 0.000000000000000000, 0.000000000000000000 ) ) ;
#17893=VERTEX_POINT ( 'NONE', #15236 ) ;
#17894=ORIENTED_EDGE ( 'NONE', *, *, #5555, .T. ) ;
#17896=EDGE_LOOP ( 'NONE', ( #60333, #11605, #55667, #22310 ) ) ;
#17897=SHAPE_REPRESENTATION_RELATIONSHIP ( 'NONE' , 'NONE' ,  #45039, #65033 ) ;
#17900=AXIS2_PLACEMENT_3D ( 'NONE', #28894, #64768, #28245 ) ;
#17901=DIRECTION ( 'NONE',  ( 1.000000000000000000, 0.000000000000000000, 0.000000000000000000 ) ) ;
#17905=CIRCLE ( 'NONE', #55053, 5.000000000000000888 ) ;
#17908=ORIENTED_EDGE ( 'NONE', *, *, #54073, .F. ) ;
#17910=ORIENTED_EDGE ( 'NONE', *, *, #38374, .F. ) ;
#17911=CARTESIAN_POINT ( 'NONE',  ( -35.00000000000000000, -11.37311665002361494, -2.936739658819992549 ) ) ;
#17913=VERTEX_POINT ( 'NONE', #36830 ) ;
#17922=VECTOR ( 'NONE', #13781, 1000.000000000000000 ) ;
#17923=ORIENTED_EDGE ( 'NONE', *, *, #40778, .F. ) ;
#17925=CARTESIAN_POINT ( 'NONE',  ( -35.00000000000000000, -11.23004253107761130, -4.732539170486383284 ) ) ;
#17927=DIRECTION ( 'NONE',  ( -1.000000000000000000, -0.000000000000000000, 0.000000000000000000 ) ) ;
#17929=DIRECTION ( 'NONE',  ( 0.000000000000000000, 0.8515178078024850938, -0.5243256840888592674 ) ) ;
#17930=CARTESIAN_POINT ( 'NONE',  ( 35.00000000000000000, 3.213188559034240832, -11.29812557209478285 ) ) ;
#17932=LINE ( 'NONE', #8278, #23868 ) ;
#17935=ORIENTED_EDGE ( 'NONE', *, *, #1671, .T. ) ;
#17939=LINE ( 'NONE', #33227, #28518 ) ;
#17940=CARTESIAN_POINT ( 'NONE',  ( -35.00000000000000000, -4.603882218679629545, 10.80631716521665453 ) ) ;
#17941=CARTESIAN_POINT ( 'NONE',  ( 35.00000000000000000, 4.705694406421931860E-17, -3.469127814946512892E-15 ) ) ;
#17942=CARTESIAN_POINT ( 'NONE',  ( -25.86628395826706850, -8.041618865309574815, 10.84354029019568522 ) ) ;
#17947=DIRECTION ( 'NONE',  ( -1.000000000000000000, 0.000000000000000000, -0.000000000000000000 ) ) ;
#17948=CARTESIAN_POINT ( 'NONE',  ( 35.00000000000000000, 4.426194442447407340, 11.35427606708800852 ) ) ;
#17950=EDGE_CURVE ( 'NONE', #37639, #26820, #15233, .T. ) ;
#17951=CARTESIAN_POINT ( 'NONE',  ( -37.00000000000000711, 11.59095880812008161, -1.903127969211228621 ) ) ;
#17952=ORIENTED_EDGE ( 'NONE', *, *, #40335, .T. ) ;
#17953=VECTOR ( 'NONE', #46066, 1000.000000000000000 ) ;
#17958=AXIS2_PLACEMENT_3D ( 'NONE', #52368, #47376, #30735 ) ;
#17959=AXIS2_PLACEMENT_3D ( 'NONE', #51175, #5628, #56474 ) ;
#17960=VERTEX_POINT ( 'NONE', #37485 ) ;
#17964=VERTEX_POINT ( 'NONE', #43439 ) ;
#17966=DIRECTION ( 'NONE',  ( 1.000000000000000000, 0.000000000000000000, 0.000000000000000000 ) ) ;
#17967=DIRECTION ( 'NONE',  ( 1.000000000000000000, -0.000000000000000000, 0.000000000000000000 ) ) ;
#17968=CARTESIAN_POINT ( 'NONE',  ( 35.00000000000000000, 4.705694406421931860E-17, -3.469127814946512892E-15 ) ) ;
#17969=ADVANCED_FACE ( 'NONE', ( #42791 ), #57792, .T. ) ;
#17971=ORIENTED_EDGE ( 'NONE', *, *, #36251, .F. ) ;
#17972=ORIENTED_EDGE ( 'NONE', *, *, #28806, .T. ) ;
#17973=AXIS2_PLACEMENT_3D ( 'NONE', #42040, #47387, #62637 ) ;
#17974=EDGE_LOOP ( 'NONE', ( #27967, #48584, #40698, #61844 ) ) ;
#17976=CARTESIAN_POINT ( 'NONE',  ( 47.00000000000000711, 4.705694406421931860E-17, -3.469127814946512892E-15 ) ) ;
#17978=CARTESIAN_POINT ( 'NONE',  ( 37.00000000000000711, -12.01765980939840439, 2.021542716731525413 ) ) ;
#17980=ORIENTED_EDGE ( 'NONE', *, *, #22061, .T. ) ;
#17981=FACE_OUTER_BOUND ( 'NONE', #4800, .T. ) ;
#17983=DIRECTION ( 'NONE',  ( 0.000000000000000000, 0.01356324068817998940, -0.9999080150203990547 ) ) ;
#17984=ORIENTED_EDGE ( 'NONE', *, *, #33750, .F. ) ;
#17985=ORIENTED_EDGE ( 'NONE', *, *, #28357, .F. ) ;
#17986=CARTESIAN_POINT ( 'NONE',  ( 0.1901047366177790743, -0.2738782441758320640, 11.99765584512894989 ) ) ;
#17987=ORIENTED_EDGE ( 'NONE', *, *, #58192, .T. ) ;
#17988=CARTESIAN_POINT ( 'NONE',  ( 10.63279796331799787, 0.6010364628809637955, -13.48722014042763462 ) ) ;
#17989=ORIENTED_EDGE ( 'NONE', *, *, #61758, .T. ) ;
#17992=CARTESIAN_POINT ( 'NONE',  ( 35.00000000000000000, -8.766823244861932096, 7.817610399097601359 ) ) ;
#17993=EDGE_CURVE ( 'NONE', #4915, #18413, #62424, .T. ) ;
#17994=AXIS2_PLACEMENT_3D ( 'NONE', #50503, #56813, #45828 ) ;
#17998=CARTESIAN_POINT ( 'NONE',  ( 5.973846796310454010, -8.876357692484395656, -8.083262641105859458 ) ) ;
#17999=VERTEX_POINT ( 'NONE', #47795 ) ;
#18000=DIRECTION ( 'NONE',  ( 0.000000000000000000, 0.01356324068817991828, -0.9999080150203990547 ) ) ;
#18007=ADVANCED_FACE ( 'NONE', ( #23173 ), #38125, .F. ) ;
#18012=ORIENTED_EDGE ( 'NONE', *, *, #60127, .T. ) ;
#18015=DIRECTION ( 'NONE',  ( 1.000000000000000000, 0.000000000000000000, -0.000000000000000000 ) ) ;
#18016=AXIS2_PLACEMENT_3D ( 'NONE', #52876, #56660, #2701 ) ;
#18017=ORIENTED_EDGE ( 'NONE', *, *, #2025, .F. ) ;
#18020=CARTESIAN_POINT ( 'NONE',  ( -3.552825562195119247, 9.416395929211306637, 7.449814802983512507 ) ) ;
#18023=VERTEX_POINT ( 'NONE', #8524 ) ;
#18024=CIRCLE ( 'NONE', #19069, 5.000000000000001776 ) ;
#18025=LINE ( 'NONE', #38286, #34779 ) ;
#18030=EDGE_CURVE ( 'NONE', #18023, #14592, #50091, .T. ) ;
#18034=EDGE_CURVE ( 'NONE', #61175, #22451, #62002, .T. ) ;
#18035=AXIS2_PLACEMENT_3D ( 'NONE', #24149, #13504, #65027 ) ;
#18036=VECTOR ( 'NONE', #63067, 1000.000000000000000 ) ;
#18038=ADVANCED_FACE ( 'NONE', ( #13823 ), #59737, .T. ) ;
#18039=CARTESIAN_POINT ( 'NONE',  ( 11.97712667809381770, -9.005688583286994842, -7.937970216750675156 ) ) ;
#18040=ADVANCED_FACE ( 'NONE', ( #14800 ), #33790, .T. ) ;
#18045=ORIENTED_EDGE ( 'NONE', *, *, #21290, .T. ) ;
#18048=EDGE_LOOP ( 'NONE', ( #18177, #29647, #7820, #2740 ) ) ;
#18049=DIRECTION ( 'NONE',  ( -1.000000000000000000, 0.000000000000000000, 0.000000000000000000 ) ) ;
#18050=ORIENTED_EDGE ( 'NONE', *, *, #59477, .T. ) ;
#18051=VERTEX_POINT ( 'NONE', #24154 ) ;
#18052=CARTESIAN_POINT ( 'NONE',  ( -10.84987915304990658, -8.326549988222685883, -8.645316455905160069 ) ) ;
#18056=CARTESIAN_POINT ( 'NONE',  ( -37.00000000000000711, 3.916263239775508165, -11.07407352312208459 ) ) ;
#18057=CARTESIAN_POINT ( 'NONE',  ( 3.831474068947881229, 5.123838571001932962, 12.49171852625460488 ) ) ;
#18058=AXIS2_PLACEMENT_3D ( 'NONE', #54694, #53378, #58710 ) ;
#18059=DIRECTION ( 'NONE',  ( -1.000000000000000000, 0.000000000000000000, 0.000000000000000000 ) ) ;
#18063=CYLINDRICAL_SURFACE ( 'NONE', #62824, 5.000000000000000888 ) ;
#18066=CARTESIAN_POINT ( 'NONE',  ( 36.00000000000000711, -2.527899948230726057, -12.49688848680883346 ) ) ;
#18067=ORIENTED_EDGE ( 'NONE', *, *, #28615, .F. ) ;
#18070=CARTESIAN_POINT ( 'NONE',  ( -20.35303972915886561, 13.07716483859543999, -3.365615382918716758 ) ) ;
#18071=AXIS2_PLACEMENT_3D ( 'NONE', #39231, #65792, #59527 ) ;
#18072=ORIENTED_EDGE ( 'NONE', *, *, #16922, .T. ) ;
#18073=CARTESIAN_POINT ( 'NONE',  ( 21.44111281379507261, -11.69236863416677075, -2.731880686291859206 ) ) ;
#18075=DIRECTION ( 'NONE',  ( 0.000000000000000000, -0.01356324068817991828, 0.9999080150203990547 ) ) ;
#18077=EDGE_CURVE ( 'NONE', #21253, #60341, #46065, .T. ) ;
#18081=VERTEX_POINT ( 'NONE', #14481 ) ;
#18082=FACE_OUTER_BOUND ( 'NONE', #54123, .T. ) ;
#18083=ORIENTED_EDGE ( 'NONE', *, *, #8692, .F. ) ;
#18084=VERTEX_POINT ( 'NONE', #4550 ) ;
#18087=CYLINDRICAL_SURFACE ( 'NONE', #55977, 12.18649999999999878 ) ;
#18088=DIRECTION ( 'NONE',  ( 1.000000000000000000, 0.000000000000000000, 0.000000000000000000 ) ) ;
#18090=DIRECTION ( 'NONE',  ( 1.000000000000000000, 0.000000000000000000, 0.000000000000000000 ) ) ;
#18091=CARTESIAN_POINT ( 'NONE',  ( -35.00000000000000000, 0.000000000000000000, 0.000000000000000000 ) ) ;
#18092=VECTOR ( 'NONE', #6748, 1000.000000000000000 ) ;
#18094=AXIS2_PLACEMENT_3D ( 'NONE', #39370, #65611, #14101 ) ;
#18095=CARTESIAN_POINT ( 'NONE',  ( 37.00000000000000711, 5.672855678558685888, -10.28547182238010116 ) ) ;
#18096=ORIENTED_EDGE ( 'NONE', *, *, #18298, .T. ) ;
#18099=DIRECTION ( 'NONE',  ( 0.000000000000000000, -0.01356324068817999114, 0.9999080150203989437 ) ) ;
#18100=EDGE_CURVE ( 'NONE', #46798, #63438, #4700, .T. ) ;
#18101=EDGE_CURVE ( 'NONE', #57337, #20539, #34369, .T. ) ;
#18102=CARTESIAN_POINT ( 'NONE',  ( -35.00000000000000000, 12.73293890771483206, 0.6593684648220944355 ) ) ;
#18104=AXIS2_PLACEMENT_3D ( 'NONE', #62351, #16806, #37416 ) ;
#18105=CARTESIAN_POINT ( 'NONE',  ( -6.521449894988646356, -1.136726751579723249, 13.45215267574590889 ) ) ;
#18106=CARTESIAN_POINT ( 'NONE',  ( -10.84199523828880984, -6.639569374722061212, 11.75613028300089091 ) ) ;
#18107=EDGE_LOOP ( 'NONE', ( #50495, #3800, #26526, #45886 ) ) ;
#18108=CARTESIAN_POINT ( 'NONE',  ( 47.00000000000000711, 4.705694406421931860E-17, -3.469127814946512892E-15 ) ) ;
#18110=DIRECTION ( 'NONE',  ( -1.000000000000000000, 0.000000000000000000, 0.000000000000000000 ) ) ;
#18112=EDGE_CURVE ( 'NONE', #4846, #1056, #65172, .T. ) ;
#18114=DIRECTION ( 'NONE',  ( 0.000000000000000000, -0.5472293298355330737, 0.8369827122275305120 ) ) ;
#18115=CARTESIAN_POINT ( 'NONE',  ( 35.00000000000000000, -10.14408668126217350, -5.921969905510321652 ) ) ;
#18117=VERTEX_POINT ( 'NONE', #20805 ) ;
#18118=CARTESIAN_POINT ( 'NONE',  ( 18.99404383257591178, -0.5703370437478472166, 12.04059188870767372 ) ) ;
#18120=LINE ( 'NONE', #28413, #49912 ) ;
#18122=EDGE_CURVE ( 'NONE', #52452, #63611, #5721, .T. ) ;
#18123=LINE ( 'NONE', #38393, #35048 ) ;
#18124=AXIS2_PLACEMENT_3D ( 'NONE', #48079, #64006, #8815 ) ;
#18127=ORIENTED_EDGE ( 'NONE', *, *, #37443, .T. ) ;
#18129=AXIS2_PLACEMENT_3D ( 'NONE', #13281, #33563, #62487 ) ;
#18130=AXIS2_PLACEMENT_3D ( 'NONE', #10845, #6521, #47737 ) ;
#18131=ADVANCED_FACE ( 'NONE', ( #203 ), #45408, .T. ) ;
#18135=DIRECTION ( 'NONE',  ( 1.000000000000000000, 0.000000000000000000, 0.000000000000000000 ) ) ;
#18137=DIRECTION ( 'NONE',  ( 1.000000000000000000, 0.000000000000000000, 0.000000000000000000 ) ) ;
#18141=FACE_OUTER_BOUND ( 'NONE', #9210, .T. ) ;
#18143=CARTESIAN_POINT ( 'NONE',  ( 35.00000000000000000, -0.3025107581130382917, 11.74226168163341022 ) ) ;
#18145=ORIENTED_EDGE ( 'NONE', *, *, #53832, .F. ) ;
#18147=CARTESIAN_POINT ( 'NONE',  ( -24.81811232574347059, 10.66920234648263488, 8.273232917182683721 ) ) ;
#18148=CIRCLE ( 'NONE', #55301, 12.18650000000000055 ) ;
#18150=CARTESIAN_POINT ( 'NONE',  ( -24.95274435386256329, 11.81191533060742493, 6.539041355910289788 ) ) ;
#18151=AXIS2_PLACEMENT_3D ( 'NONE', #33057, #39357, #53363 ) ;
#18152=LINE ( 'NONE', #28133, #9413 ) ;
#18154=CARTESIAN_POINT ( 'NONE',  ( -35.00000000000000000, 9.493370459201697642, 6.917234959366862057 ) ) ;
#18155=CIRCLE ( 'NONE', #35065, 5.000000000000001776 ) ;
#18156=EDGE_LOOP ( 'NONE', ( #12353, #37693, #27516, #58958 ) ) ;
#18157=EDGE_CURVE ( 'NONE', #40994, #8415, #62030, .T. ) ;
#18158=CARTESIAN_POINT ( 'NONE',  ( -26.34357995062409330, -10.72024744338163593, 5.392951959879463075 ) ) ;
#18159=DIRECTION ( 'NONE',  ( 0.000000000000000000, 0.01356324068818000848, -0.9999080150203990547 ) ) ;
#18160=DIRECTION ( 'NONE',  ( -1.000000000000000000, -1.836970198721029688E-16, -0.000000000000000000 ) ) ;
#18161=EDGE_LOOP ( 'NONE', ( #9382, #2305, #34863, #52352 ) ) ;
#18162=AXIS2_PLACEMENT_3D ( 'NONE', #61106, #15538, #24544 ) ;
#18164=ORIENTED_EDGE ( 'NONE', *, *, #25315, .F. ) ;
#18165=AXIS2_PLACEMENT_3D ( 'NONE', #5006, #25266, #45544 ) ;
#18166=EDGE_CURVE ( 'NONE', #25415, #60864, #28021, .T. ) ;
#18168=CARTESIAN_POINT ( 'NONE',  ( -10.60783295782091074, -9.408442966608031810, 7.467594787374099319 ) ) ;
#18169=DIRECTION ( 'NONE',  ( -1.000000000000000000, 0.000000000000000000, 0.000000000000000000 ) ) ;
#18171=CARTESIAN_POINT ( 'NONE',  ( -37.00000000000000711, 10.14408668126213442, 5.921969905510389154 ) ) ;
#18172=DIRECTION ( 'NONE',  ( -0.000000000000000000, -0.000000000000000000, -1.000000000000000000 ) ) ;
#18174=AXIS2_PLACEMENT_3D ( 'NONE', #25672, #40965, #61244 ) ;
#18175=VERTEX_POINT ( 'NONE', #15149 ) ;
#18176=CARTESIAN_POINT ( 'NONE',  ( -35.00000000000000000, 9.700295462048664774, 7.376655759824919834 ) ) ;
#18177=ORIENTED_EDGE ( 'NONE', *, *, #15168, .T. ) ;
#18178=CIRCLE ( 'NONE', #5465, 5.000000000000000888 ) ;
#18179=ADVANCED_FACE ( 'NONE', ( #16140 ), #46725, .T. ) ;
#18182=CARTESIAN_POINT ( 'NONE',  ( -35.00000000000000000, 11.73463472867576129, 3.287724142101457137 ) ) ;
#18183=DIRECTION ( 'NONE',  ( -1.000000000000000000, 0.000000000000000000, 0.000000000000000000 ) ) ;
#18186=CIRCLE ( 'NONE', #94, 5.000000000000000888 ) ;
#18189=CIRCLE ( 'NONE', #47900, 11.99999999999998579 ) ;
#18191=CARTESIAN_POINT ( 'NONE',  ( 8.829757094950462459, 6.323861778933462574, 10.20043549987153497 ) ) ;
#18192=DIRECTION ( 'NONE',  ( -1.000000000000000000, 0.000000000000000000, 0.000000000000000000 ) ) ;
#18193=FACE_OUTER_BOUND ( 'NONE', #11409, .T. ) ;
#18196=DIRECTION ( 'NONE',  ( -1.000000000000000000, -0.000000000000000000, -0.000000000000000000 ) ) ;
#18198=DIRECTION ( 'NONE',  ( 1.000000000000000000, -0.000000000000000000, -0.000000000000000000 ) ) ;
#18199=EDGE_CURVE ( 'NONE', #4143, #23433, #46402, .T. ) ;
#18200=AXIS2_PLACEMENT_3D ( 'NONE', #61945, #41978, #16709 ) ;
#18203=CARTESIAN_POINT ( 'NONE',  ( -36.00000000000000711, -12.21925492305359562, -3.640372113593682624 ) ) ;
#18204=VERTEX_POINT ( 'NONE', #5532 ) ;
#18209=CARTESIAN_POINT ( 'NONE',  ( -11.40165637463000614, -7.508992741355387857, -11.21895841913464587 ) ) ;
#18211=CARTESIAN_POINT ( 'NONE',  ( 17.48309864844228301, -10.09872697878719627, 8.990776945112616048 ) ) ;
#18213=CYLINDRICAL_SURFACE ( 'NONE', #10531, 12.18650000000000055 ) ;
#18215=ORIENTED_EDGE ( 'NONE', *, *, #10741, .T. ) ;
#18216=CYLINDRICAL_SURFACE ( 'NONE', #41430, 12.74999999999999822 ) ;
#18217=ORIENTED_EDGE ( 'NONE', *, *, #63178, .F. ) ;
#18219=DIRECTION ( 'NONE',  ( 1.000000000000000000, 0.000000000000000000, 0.000000000000000000 ) ) ;
#18220=CYLINDRICAL_SURFACE ( 'NONE', #38557, 5.000000000000000888 ) ;
#18222=LINE ( 'NONE', #38493, #26953 ) ;
#18223=DIRECTION ( 'NONE',  ( 1.000000000000000000, 0.000000000000000000, -0.000000000000000000 ) ) ;
#18231=SURFACE_STYLE_USAGE ( .BOTH. , #16907 ) ;
#18236=CIRCLE ( 'NONE', #26674, 5.000000000000000000 ) ;
#18238=ORIENTED_EDGE ( 'NONE', *, *, #65269, .F. ) ;
#18240=EDGE_CURVE ( 'NONE', #26911, #48492, #540, .T. ) ;
#18246=ORIENTED_EDGE ( 'NONE', *, *, #3925, .T. ) ;
#18247=DIRECTION ( 'NONE',  ( -1.000000000000000000, 0.000000000000000000, 0.000000000000000000 ) ) ;
#18250=ORIENTED_EDGE ( 'NONE', *, *, #17512, .T. ) ;
#18251=CIRCLE ( 'NONE', #41578, 5.000000000000001776 ) ;
#18252=CYLINDRICAL_SURFACE ( 'NONE', #6542, 12.18650000000000055 ) ;
#18253=CARTESIAN_POINT ( 'NONE',  ( 37.00000000000000711, -10.14408668126217350, -5.921969905510321652 ) ) ;
#18254=AXIS2_PLACEMENT_3D ( 'NONE', #59497, #9261, #49849 ) ;
#18255=DIRECTION ( 'NONE',  ( 0.000000000000000000, 0.01356324068817991828, -0.9999080150203990547 ) ) ;
#18256=CARTESIAN_POINT ( 'NONE',  ( -35.00000000000000000, -8.854740511458796703, -7.717887834988336415 ) ) ;
#18257=ADVANCED_FACE ( 'NONE', ( #15791 ), #45742, .T. ) ;
#18260=CARTESIAN_POINT ( 'NONE',  ( 145.1370849898475797, 3.309064568108273190E-14, 0.000000000000000000 ) ) ;
#18264=DIRECTION ( 'NONE',  ( 0.000000000000000000, 0.01356324068817992175, -0.9999080150203990547 ) ) ;
#18268=CARTESIAN_POINT ( 'NONE',  ( 35.00000000000000000, -1.463443770872862482, -12.09831040184923978 ) ) ;
#18270=CARTESIAN_POINT ( 'NONE',  ( 28.91461756896324786, 10.37982945138888446, 6.039709648425571231 ) ) ;
#18274=CARTESIAN_POINT ( 'NONE',  ( 35.00000000000000000, 4.705694406421931860E-17, -3.469127814946512892E-15 ) ) ;
#18275=CARTESIAN_POINT ( 'NONE',  ( -4.989057617119011745, -0.9162120371760335003, 11.96497202265570259 ) ) ;
#18276=ORIENTED_EDGE ( 'NONE', *, *, #38061, .T. ) ;
#18278=( BOUNDED_CURVE ( )  B_SPLINE_CURVE ( 3, ( #32472, #7540, #47471, #2907 ),
 .UNSPECIFIED., .F., .F. ) 
 B_SPLINE_CURVE_WITH_KNOTS ( ( 4, 4 ),
 ( 5.009162659680186813, 5.030260039792340265 ),
 .UNSPECIFIED. ) 
 CURVE ( )  GEOMETRIC_REPRESENTATION_ITEM ( )  RATIONAL_B_SPLINE_CURVE ( ( 1.000000000000000000, 0.9999629087233127267, 0.9999629087233127267, 1.000000000000000000 ) ) 
 REPRESENTATION_ITEM ( '' )  );
#18280=CARTESIAN_POINT ( 'NONE',  ( 35.00000000000000000, -10.99909370905160699, -5.246972444133983338 ) ) ;
#18281=DIRECTION ( 'NONE',  ( 0.000000000000000000, -0.9551603052523448545, 0.2960891610144612551 ) ) ;
#18282=CARTESIAN_POINT ( 'NONE',  ( 12.90917927732748360, -12.48803436428174507, -5.132121098330106435 ) ) ;
#18285=ORIENTED_EDGE ( 'NONE', *, *, #22901, .T. ) ;
#18287=CARTESIAN_POINT ( 'NONE',  ( 22.88594695219327235, -4.822122601967141264, 12.60940655271284427 ) ) ;
#18289=DIRECTION ( 'NONE',  ( 0.000000000000000000, 0.01356324068817998940, -0.9999080150203990547 ) ) ;
#18291=AXIS2_PLACEMENT_3D ( 'NONE', #17681, #60107, #34502 ) ;
#18292=VECTOR ( 'NONE', #31671, 1000.000000000000000 ) ;
#18294=ORIENTED_EDGE ( 'NONE', *, *, #64112, .T. ) ;
#18295=DIRECTION ( 'NONE',  ( -1.000000000000000000, -0.000000000000000000, 0.000000000000000000 ) ) ;
#18298=EDGE_CURVE ( 'NONE', #9098, #60526, #23805, .T. ) ;
#18299=VECTOR ( 'NONE', #4434, 1000.000000000000000 ) ;
#18300=EDGE_CURVE ( 'NONE', #49629, #57610, #55963, .T. ) ;
#18301=AXIS2_PLACEMENT_3D ( 'NONE', #54771, #55407, #23863 ) ;
#18302=ORIENTED_EDGE ( 'NONE', *, *, #2506, .T. ) ;
#18304=CARTESIAN_POINT ( 'NONE',  ( 36.00000000000000711, -10.93004082984023029, -6.564808257521734802 ) ) ;
#18305=ORIENTED_EDGE ( 'NONE', *, *, #14517, .T. ) ;
#18310=CIRCLE ( 'NONE', #52249, 5.000000000000000888 ) ;
#18317=CARTESIAN_POINT ( 'NONE',  ( -37.00000000000000711, 12.57916205664481346, 2.080187960898606470 ) ) ;
#18320=DIRECTION ( 'NONE',  ( -1.000000000000000000, 0.000000000000000000, 0.000000000000000000 ) ) ;
#18334=CARTESIAN_POINT ( 'NONE',  ( 10.39889529048551964, 0.7502239413564057990, -13.48021515222736966 ) ) ;
#18335=ORIENTED_EDGE ( 'NONE', *, *, #27853, .F. ) ;
#18336=VECTOR ( 'NONE', #42227, 1000.000000000000000 ) ;
#18340=CIRCLE ( 'NONE', #3441, 12.75000000000000178 ) ;
#18342=AXIS2_PLACEMENT_3D ( 'NONE', #8721, #3760, #49614 ) ;
#18344=EDGE_CURVE ( 'NONE', #53824, #41945, #36096, .T. ) ;
#18348=ORIENTED_EDGE ( 'NONE', *, *, #60046, .F. ) ;
#18349=CARTESIAN_POINT ( 'NONE',  ( -37.00000000000000711, -0.6593684648221369571, 12.73293890771483383 ) ) ;
#18350=ADVANCED_FACE ( 'NONE', ( #57366 ), #10379, .T. ) ;
#18353=DIRECTION ( 'NONE',  ( 0.000000000000000000, -0.3807014730195085739, 0.9246979985058777496 ) ) ;
#18356=ORIENTED_EDGE ( 'NONE', *, *, #8257, .T. ) ;
#18357=VECTOR ( 'NONE', #24585, 1000.000000000000000 ) ;
#18358=EDGE_LOOP ( 'NONE', ( #22000, #26305, #32908, #56490 ) ) ;
#18359=DIRECTION ( 'NONE',  ( -1.000000000000000000, 0.000000000000000000, 0.000000000000000000 ) ) ;
#18361=CIRCLE ( 'NONE', #5592, 5.000000000000001776 ) ;
#18362=VERTEX_POINT ( 'NONE', #62237 ) ;
#18364=DIRECTION ( 'NONE',  ( 0.000000000000000000, 0.01356324068817991828, -0.9999080150203990547 ) ) ;
#18365=VECTOR ( 'NONE', #47520, 1000.000000000000000 ) ;
#18367=CARTESIAN_POINT ( 'NONE',  ( -2.747358470950249654, 5.743717875782093252, 10.56616121202656977 ) ) ;
#18368=DIRECTION ( 'NONE',  ( 1.000000000000000000, 0.000000000000000000, 0.000000000000000000 ) ) ;
#18370=CARTESIAN_POINT ( 'NONE',  ( 35.00000000000000000, 6.303578524887091916, 10.42955799785312720 ) ) ;
#18372=DIRECTION ( 'NONE',  ( 0.000000000000000000, -0.3807014730195285579, 0.9246979985058696450 ) ) ;
#18373=LINE ( 'NONE', #2074, #23496 ) ;
#18374=CARTESIAN_POINT ( 'NONE',  ( -35.00000000000000000, -7.817492529713920391, 9.348667969174380588 ) ) ;
#18375=DIRECTION ( 'NONE',  ( 0.000000000000000000, -0.1118654143051476951, -0.9937233664769775654 ) ) ;
#18379=VECTOR ( 'NONE', #2290, 1000.000000000000000 ) ;
#18380=CIRCLE ( 'NONE', #11989, 5.000000000000000000 ) ;
#18382=VECTOR ( 'NONE', #45590, 1000.000000000000000 ) ;
#18383=ORIENTED_EDGE ( 'NONE', *, *, #55409, .F. ) ;
#18385=VERTEX_POINT ( 'NONE', #51633 ) ;
#18386=DIRECTION ( 'NONE',  ( 0.000000000000000000, -0.01356324068818000328, 0.9999080150203990547 ) ) ;
#18389=AXIS2_PLACEMENT_3D ( 'NONE', #25363, #20379, #60953 ) ;
#18393=ORIENTED_EDGE ( 'NONE', *, *, #65660, .T. ) ;
#18394=AXIS2_PLACEMENT_3D ( 'NONE', #60217, #10323, #30600 ) ;
#18395=ORIENTED_EDGE ( 'NONE', *, *, #8284, .F. ) ;
#18396=ORIENTED_EDGE ( 'NONE', *, *, #11777, .F. ) ;
#18397=CARTESIAN_POINT ( 'NONE',  ( 29.58334585860551513, -8.059223888209368525, 10.83973719671545233 ) ) ;
#18398=CIRCLE ( 'NONE', #49216, 5.000000000000000000 ) ;
#18400=EDGE_CURVE ( 'NONE', #2234, #61618, #60963, .T. ) ;
#18401=ORIENTED_EDGE ( 'NONE', *, *, #61027, .F. ) ;
#18405=DIRECTION ( 'NONE',  ( 1.000000000000000000, 0.000000000000000000, 0.000000000000000000 ) ) ;
#18406=ORIENTED_EDGE ( 'NONE', *, *, #11568, .F. ) ;
#18407=DIRECTION ( 'NONE',  ( 0.000000000000000000, 0.01356324068817998940, -0.9999080150203990547 ) ) ;
#18408=ADVANCED_FACE ( 'NONE', ( #57261 ), #20369, .T. ) ;
#18411=DIRECTION ( 'NONE',  ( -0.000000000000000000, -1.000000000000000000, -0.000000000000000000 ) ) ;
#18413=VERTEX_POINT ( 'NONE', #6728 ) ;
#18415=EDGE_CURVE ( 'NONE', #61311, #8578, #35449, .T. ) ;
#18416=ORIENTED_EDGE ( 'NONE', *, *, #38692, .T. ) ;
#18417=CARTESIAN_POINT ( 'NONE',  ( -37.00000000000000711, 0.000000000000000000, 0.000000000000000000 ) ) ;
#18418=VERTEX_POINT ( 'NONE', #35652 ) ;
#18419=CARTESIAN_POINT ( 'NONE',  ( 21.90174657591892071, -11.97747433400148864, -0.7349207973210698519 ) ) ;
#18421=LINE ( 'NONE', #17752, #34045 ) ;
#18422=CARTESIAN_POINT ( 'NONE',  ( -35.00000000000000000, 11.72195762423408816, 0.7536123767500589876 ) ) ;
#18423=AXIS2_PLACEMENT_3D ( 'NONE', #62735, #37476, #7207 ) ;
#18425=CARTESIAN_POINT ( 'NONE',  ( -7.165178994131125023, -1.884899025446307830, -13.36804325434021479 ) ) ;
#18426=CARTESIAN_POINT ( 'NONE',  ( 12.59797654570207293, 10.92525928803750190, -7.940295129871110191 ) ) ;
#18427=VERTEX_POINT ( 'NONE', #41290 ) ;
#18428=CYLINDRICAL_SURFACE ( 'NONE', #5112, 12.18649999999999878 ) ;
#18429=ORIENTED_EDGE ( 'NONE', *, *, #47239, .T. ) ;
#18430=EDGE_CURVE ( 'NONE', #35879, #56806, #49309, .T. ) ;
#18431=EDGE_CURVE ( 'NONE', #45226, #22711, #21346, .T. ) ;
#18435=CIRCLE ( 'NONE', #33314, 12.18650000000000055 ) ;
#18439=EDGE_CURVE ( 'NONE', #56824, #32709, #11017, .T. ) ;
#18441=CIRCLE ( 'NONE', #43898, 12.18650000000000233 ) ;
#18445=ADVANCED_FACE ( 'NONE', ( #30997 ), #26024, .T. ) ;
#18448=CARTESIAN_POINT ( 'NONE',  ( 35.00000000000000000, -8.927548052240835474, 8.295159312811946961 ) ) ;
#18449=CIRCLE ( 'NONE', #61941, 12.18650000000000411 ) ;
#18450=EDGE_CURVE ( 'NONE', #22470, #28861, #16338, .T. ) ;
#18451=CYLINDRICAL_SURFACE ( 'NONE', #2712, 12.18649999999999878 ) ;
#18453=AXIS2_PLACEMENT_3D ( 'NONE', #45833, #21200, #41471 ) ;
#18456=FACE_OUTER_BOUND ( 'NONE', #34334, .T. ) ;
#18457=DIRECTION ( 'NONE',  ( 0.000000000000000000, 0.01356324068817998940, -0.9999080150203990547 ) ) ;
#18458=AXIS2_PLACEMENT_3D ( 'NONE', #38984, #24035, #63930 ) ;
#18459=CARTESIAN_POINT ( 'NONE',  ( -9.958172265059427986, -3.385416999472194544, 13.06986580931351938 ) ) ;
#18460=AXIS2_PLACEMENT_3D ( 'NONE', #12341, #32606, #7349 ) ;
#18461=CARTESIAN_POINT ( 'NONE',  ( -9.811405951060844899, -4.024453971883430903, 12.88726659228943028 ) ) ;
#18462=ORIENTED_EDGE ( 'NONE', *, *, #19108, .T. ) ;
#18463=FACE_OUTER_BOUND ( 'NONE', #49802, .T. ) ;
#18464=DIRECTION ( 'NONE',  ( 0.000000000000000000, -0.01356324068817998940, 0.9999080150203990547 ) ) ;
#18465=CARTESIAN_POINT ( 'NONE',  ( -35.00000000000000000, 12.09831040184926287, -1.463443770872647542 ) ) ;
#18466=ADVANCED_FACE ( 'NONE', ( #11054 ), #41626, .T. ) ;
#18469=( BOUNDED_CURVE ( )  B_SPLINE_CURVE ( 3, ( #18275, #54162, #32871, #7973 ),
 .UNSPECIFIED., .F., .F. ) 
 B_SPLINE_CURVE_WITH_KNOTS ( ( 4, 4 ),
 ( 1.647221706219855974, 1.689073584867815336 ),
 .UNSPECIFIED. ) 
 CURVE ( )  GEOMETRIC_REPRESENTATION_ITEM ( )  RATIONAL_B_SPLINE_CURVE ( ( 1.000000000000000000, 0.9998540403475023597, 0.9998540403475023597, 1.000000000000000000 ) ) 
 REPRESENTATION_ITEM ( '' )  );
#18470=ORIENTED_EDGE ( 'NONE', *, *, #49161, .F. ) ;
#18471=DIRECTION ( 'NONE',  ( -1.000000000000000000, 0.000000000000000000, 0.000000000000000000 ) ) ;
#18472=CARTESIAN_POINT ( 'NONE',  ( 10.48620311856346454, 8.250315036047107142, -8.713914264323181058 ) ) ;
#18473=CARTESIAN_POINT ( 'NONE',  ( -18.58686583997218378, 5.151216734910788908, -10.83812558286602012 ) ) ;
#18474=EDGE_LOOP ( 'NONE', ( #28215, #61924, #33250, #19666 ) ) ;
#18475=DIRECTION ( 'NONE',  ( 0.000000000000000000, -0.9937233664769749009, 0.1118654143051720229 ) ) ;
#18478=VECTOR ( 'NONE', #58341, 1000.000000000000000 ) ;
#18479=EDGE_CURVE ( 'NONE', #19210, #26974, #5440, .T. ) ;
#18480=AXIS2_PLACEMENT_3D ( 'NONE', #47845, #7951, #2303 ) ;
#18481=EDGE_LOOP ( 'NONE', ( #45950, #12376, #10344, #47444, #52441, #4013 ) ) ;
#18482=FACE_OUTER_BOUND ( 'NONE', #62592, .T. ) ;
#18483=CIRCLE ( 'NONE', #38634, 5.000000000000000888 ) ;
#18484=EDGE_CURVE ( 'NONE', #57324, #47803, #13899, .T. ) ;
#18486=CARTESIAN_POINT ( 'NONE',  ( 35.00000000000000000, 0.06441628369836321921, -12.18632975068353019 ) ) ;
#18487=CARTESIAN_POINT ( 'NONE',  ( -20.92021774235402276, -12.94977746786776684, -3.816457577290517822 ) ) ;
#18488=CARTESIAN_POINT ( 'NONE',  ( 35.00000000000000000, 8.766823244861988940, -7.817610399097547180 ) ) ;
#18490=AXIS2_PLACEMENT_3D ( 'NONE', #381, #4730, #20660 ) ;
#18491=CIRCLE ( 'NONE', #53522, 5.000000000000000888 ) ;
#18493=B_SPLINE_CURVE_WITH_KNOTS ( 'NONE', 3,
 ( #42407, #17825, #32445, #42749, #17507, #16832, #28138, #7179, #37778, #12486 ),
 .UNSPECIFIED., .F., .F.,
 ( 4, 2, 2, 2, 4 ),
 ( 0.000000000000000000, 0.002646595623854251962, 0.005293191247708503924, 0.007939786871562756754, 0.01058638249541700785 ),
 .UNSPECIFIED. ) ;
#18495=ORIENTED_EDGE ( 'NONE', *, *, #10098, .F. ) ;
#18497=FACE_OUTER_BOUND ( 'NONE', #64849, .T. ) ;
#18499=ORIENTED_EDGE ( 'NONE', *, *, #10886, .F. ) ;
#18502=ORIENTED_EDGE ( 'NONE', *, *, #20340, .T. ) ;
#18503=ORIENTED_EDGE ( 'NONE', *, *, #42335, .F. ) ;
#18504=CARTESIAN_POINT ( 'NONE',  ( -16.82301864121118484, 8.090309307062092614, 10.80809437597500100 ) ) ;
#18506=CARTESIAN_POINT ( 'NONE',  ( -35.00000000000000000, -8.295159312811792418, -8.927548052240984688 ) ) ;
#18508=CARTESIAN_POINT ( 'NONE',  ( 37.00000000000000711, 12.12087942037209842, -1.262958560998807656 ) ) ;
#18509=CARTESIAN_POINT ( 'NONE',  ( -35.00000000000000000, 0.000000000000000000, 0.000000000000000000 ) ) ;
#18510=EDGE_LOOP ( 'NONE', ( #24558, #11593, #27506, #46936 ) ) ;
#18512=DIRECTION ( 'NONE',  ( 0.000000000000000000, 0.01356324068817998940, -0.9999080150203990547 ) ) ;
#18513=DIRECTION ( 'NONE',  ( -1.000000000000000000, -0.000000000000000000, 0.000000000000000000 ) ) ;
#18514=VECTOR ( 'NONE', #19809, 1000.000000000000000 ) ;
#18516=CARTESIAN_POINT ( 'NONE',  ( -35.00000000000000000, 0.000000000000000000, 0.000000000000000000 ) ) ;
#18520=CARTESIAN_POINT ( 'NONE',  ( 35.00000000000000000, -0.9416912585475287756, -12.71517666308947625 ) ) ;
#18521=EDGE_CURVE ( 'NONE', #5898, #35815, #37257, .T. ) ;
#18523=DIRECTION ( 'NONE',  ( 0.000000000000000000, 0.01356324068817992175, -0.9999080150203990547 ) ) ;
#18525=CIRCLE ( 'NONE', #31266, 12.75000000000000178 ) ;
#18526=EDGE_CURVE ( 'NONE', #40488, #14909, #44704, .T. ) ;
#18527=CARTESIAN_POINT ( 'NONE',  ( -8.891032880924177206, 12.93614229090409395, -3.860857758255646921 ) ) ;
#18528=ORIENTED_EDGE ( 'NONE', *, *, #63618, .T. ) ;
#18529=ORIENTED_EDGE ( 'NONE', *, *, #28088, .T. ) ;
#18533=CARTESIAN_POINT ( 'NONE',  ( 37.00000000000000711, 4.705694406421931860E-17, -3.469127814946512892E-15 ) ) ;
#18534=AXIS2_PLACEMENT_3D ( 'NONE', #2261, #16235, #41158 ) ;
#18535=CARTESIAN_POINT ( 'NONE',  ( -10.64440273086533040, -9.782391350870078384, 6.950960968970282927 ) ) ;
#18536=ORIENTED_EDGE ( 'NONE', *, *, #1398, .F. ) ;
#18537=CYLINDRICAL_SURFACE ( 'NONE', #2442, 12.18650000000000055 ) ;
#18538=CARTESIAN_POINT ( 'NONE',  ( -10.41759788416483623, -5.099336898890864056, -10.86981208156591094 ) ) ;
#18539=CARTESIAN_POINT ( 'NONE',  ( 9.883938789068938746, 7.802108911151313997, 9.123879608504731564 ) ) ;
#18541=DIRECTION ( 'NONE',  ( -0.2034311943119418153, 0.9790892447477997917, 0.000000000000000000 ) ) ;
#18542=ORIENTED_EDGE ( 'NONE', *, *, #2660, .T. ) ;
#18543=AXIS2_PLACEMENT_3D ( 'NONE', #23084, #32694, #43344 ) ;
#18544=DIRECTION ( 'NONE',  ( 1.000000000000000000, -0.000000000000000000, -0.000000000000000000 ) ) ;
#18548=CIRCLE ( 'NONE', #23853, 12.18649999999999878 ) ;
#18549=EDGE_CURVE ( 'NONE', #43866, #18956, #47939, .T. ) ;
#18551=EDGE_CURVE ( 'NONE', #36349, #19607, #15985, .T. ) ;
#18553=VERTEX_POINT ( 'NONE', #43256 ) ;
#18555=CARTESIAN_POINT ( 'NONE',  ( 29.52239426923290466, 11.14864943672236564, 7.625421059268382429 ) ) ;
#18556=AXIS2_PLACEMENT_3D ( 'NONE', #62204, #16658, #26095 ) ;
#18558=ORIENTED_EDGE ( 'NONE', *, *, #46981, .T. ) ;
#18559=CARTESIAN_POINT ( 'NONE',  ( -11.34436572679164712, -8.403365156751931409, -8.571542621278755547 ) ) ;
#18560=CARTESIAN_POINT ( 'NONE',  ( -47.00000000000000711, 0.000000000000000000, 0.000000000000000000 ) ) ;
#18562=ADVANCED_FACE ( 'NONE', ( #37947 ), #2398, .T. ) ;
#18563=LINE ( 'NONE', #23527, #34921 ) ;
#18566=DIRECTION ( 'NONE',  ( -1.000000000000000000, 0.000000000000000000, 0.000000000000000000 ) ) ;
#18568=FACE_OUTER_BOUND ( 'NONE', #48951, .T. ) ;
#18575=CARTESIAN_POINT ( 'NONE',  ( -17.29244623348158783, 2.525873743887551814, -13.26159725786978072 ) ) ;
#18578=VECTOR ( 'NONE', #60011, 1000.000000000000000 ) ;
#18580=DIRECTION ( 'NONE',  ( 0.000000000000000000, -0.9847383929261634972, 0.1740410799127515284 ) ) ;
#18582=EDGE_CURVE ( 'NONE', #57580, #7123, #40433, .T. ) ;
#18583=FACE_OUTER_BOUND ( 'NONE', #41924, .T. ) ;
#18584=DIRECTION ( 'NONE',  ( -0.000000000000000000, -0.000000000000000000, -1.000000000000000000 ) ) ;
#18586=EDGE_LOOP ( 'NONE', ( #964, #31883, #16169, #41199 ) ) ;
#18587=CARTESIAN_POINT ( 'NONE',  ( -37.00000000000000711, 0.000000000000000000, 0.000000000000000000 ) ) ;
#18588=CIRCLE ( 'NONE', #50419, 12.18649999999999878 ) ;
#18589=DIRECTION ( 'NONE',  ( 0.000000000000000000, 0.5243256840888502746, 0.8515178078024904229 ) ) ;
#18592=EDGE_LOOP ( 'NONE', ( #32605, #31249, #37165, #211 ) ) ;
#18593=DIRECTION ( 'NONE',  ( 0.000000000000000000, 0.07632122047556495759, -0.9970832820307038435 ) ) ;
#18595=DIRECTION ( 'NONE',  ( 0.000000000000000000, 0.01356324068817998940, -0.9999080150203990547 ) ) ;
#18596=EDGE_LOOP ( 'NONE', ( #46623, #53788, #39403, #23222 ) ) ;
#18598=CARTESIAN_POINT ( 'NONE',  ( 35.00000000000000000, 11.73555825188276280, -4.983891302653623789 ) ) ;
#18600=AXIS2_PLACEMENT_3D ( 'NONE', #53803, #13536, #54117 ) ;
#18601=DIRECTION ( 'NONE',  ( 0.000000000000000000, -0.01356324068817991828, 0.9999080150203990547 ) ) ;
#18603=DIRECTION ( 'NONE',  ( -1.000000000000000000, 0.000000000000000000, 0.000000000000000000 ) ) ;
#18605=ADVANCED_FACE ( 'NONE', ( #24964 ), #34271, .T. ) ;
#18607=EDGE_LOOP ( 'NONE', ( #27241, #3714, #57566, #2394 ) ) ;
#18611=DIRECTION ( 'NONE',  ( -1.000000000000000000, 0.000000000000000000, 0.000000000000000000 ) ) ;
#18612=DIRECTION ( 'NONE',  ( 0.000000000000000000, -0.01356324068817998940, 0.9999080150203990547 ) ) ;
#18613=CARTESIAN_POINT ( 'NONE',  ( 23.12239576763279914, 2.549905108198637915, 13.26000697717500643 ) ) ;
#18614=DIRECTION ( 'NONE',  ( 0.000000000000000000, 0.01356324068817991481, -0.9999080150203990547 ) ) ;
#18616=CARTESIAN_POINT ( 'NONE',  ( -35.00000000000000000, 0.000000000000000000, 0.000000000000000000 ) ) ;
#18617=ORIENTED_EDGE ( 'NONE', *, *, #28579, .T. ) ;
#18618=CARTESIAN_POINT ( 'NONE',  ( -35.00000000000000000, -7.608228585767649044, -10.23119532541080901 ) ) ;
#18619=EDGE_CURVE ( 'NONE', #20061, #58290, #7549, .T. ) ;
#18620=ORIENTED_EDGE ( 'NONE', *, *, #22215, .F. ) ;
#18621=CARTESIAN_POINT ( 'NONE',  ( 37.00000000000000711, 8.551552972817191289, 8.052525312709789773 ) ) ;
#18622=FACE_OUTER_BOUND ( 'NONE', #55861, .T. ) ;
#18623=CARTESIAN_POINT ( 'NONE',  ( 11.74548640120467979, -10.73597826697111124, -8.184666801472349817 ) ) ;
#18624=CARTESIAN_POINT ( 'NONE',  ( 3.459614771489464946, -11.09853614738469396, -4.563167253695070258 ) ) ;
#18625=DIRECTION ( 'NONE',  ( 0.000000000000000000, -0.01356324068817992175, 0.9999080150203990547 ) ) ;
#18626=ORIENTED_EDGE ( 'NONE', *, *, #14413, .T. ) ;
#18631=ADVANCED_FACE ( 'NONE', ( #54582 ), #34590, .T. ) ;
#18632=CARTESIAN_POINT ( 'NONE',  ( -35.00000000000000000, -0.1652884326465054732, 12.18537902504609249 ) ) ;
#18633=VERTEX_POINT ( 'NONE', #65187 ) ;
#18635=ORIENTED_EDGE ( 'NONE', *, *, #9673, .F. ) ;
#18637=CARTESIAN_POINT ( 'NONE',  ( 3.618571554686976999, 8.318316264554045603, -8.649151353875886628 ) ) ;
#18638=CARTESIAN_POINT ( 'NONE',  ( 6.463891187881699807, -7.979741258536692250, 10.89069007513759324 ) ) ;
#18639=CIRCLE ( 'NONE', #40880, 12.18650000000000411 ) ;
#18641=EDGE_LOOP ( 'NONE', ( #57147, #47993, #11922, #18393 ) ) ;
#18642=ORIENTED_EDGE ( 'NONE', *, *, #45563, .T. ) ;
#18643=CYLINDRICAL_SURFACE ( 'NONE', #46716, 12.74999999999999822 ) ;
#18644=CARTESIAN_POINT ( 'NONE',  ( -27.27855387000350262, 25.00000000000000000, 5.631341004100471892 ) ) ;
#18645=DIRECTION ( 'NONE',  ( 1.000000000000000000, 0.000000000000000000, 0.000000000000000000 ) ) ;
#18652=ORIENTED_EDGE ( 'NONE', *, *, #3925, .F. ) ;
#18653=CYLINDRICAL_SURFACE ( 'NONE', #26644, 12.18650000000000055 ) ;
#18654=EDGE_CURVE ( 'NONE', #45219, #7826, #10730, .T. ) ;
#18655=CIRCLE ( 'NONE', #45208, 12.18649999999999878 ) ;
#18656=CARTESIAN_POINT ( 'NONE',  ( 37.00000000000000711, -8.839356091080105671, -8.389074212634254124 ) ) ;
#18657=ORIENTED_EDGE ( 'NONE', *, *, #46988, .T. ) ;
#18660=VERTEX_POINT ( 'NONE', #13982 ) ;
#18664=LINE ( 'NONE', #7681, #14377 ) ;
#18666=ORIENTED_EDGE ( 'NONE', *, *, #17993, .F. ) ;
#18667=CARTESIAN_POINT ( 'NONE',  ( 35.00000000000000000, -10.25474254703957477, -6.584150480049516752 ) ) ;
#18670=CARTESIAN_POINT ( 'NONE',  ( 8.555539599251753557, 3.416301611567257979, -13.06349654673114991 ) ) ;
#18674=DIRECTION ( 'NONE',  ( -1.000000000000000000, -0.000000000000000000, 0.000000000000000000 ) ) ;
#18675=EDGE_CURVE ( 'NONE', #18204, #28784, #59581, .T. ) ;
#18676=DIRECTION ( 'NONE',  ( -1.000000000000000000, 0.000000000000000000, 0.000000000000000000 ) ) ;
#18678=CARTESIAN_POINT ( 'NONE',  ( 35.00000000000000000, 10.91536515067648239, 4.339012074899986970 ) ) ;
#18680=ORIENTED_EDGE ( 'NONE', *, *, #36780, .F. ) ;
#18681=DIRECTION ( 'NONE',  ( 0.000000000000000000, 0.01356324068817998940, -0.9999080150203989437 ) ) ;
#18682=AXIS2_PLACEMENT_3D ( 'NONE', #4948, #51159, #20565 ) ;
#18683=ORIENTED_EDGE ( 'NONE', *, *, #29388, .T. ) ;
#18684=FACE_OUTER_BOUND ( 'NONE', #53303, .T. ) ;
#18686=ORIENTED_EDGE ( 'NONE', *, *, #57346, .F. ) ;
#18688=DIRECTION ( 'NONE',  ( 0.000000000000000000, -0.01356324068817999114, 0.9999080150203989437 ) ) ;
#18691=ORIENTED_EDGE ( 'NONE', *, *, #48633, .F. ) ;
#18693=ORIENTED_EDGE ( 'NONE', *, *, #43768, .T. ) ;
#18694=DIRECTION ( 'NONE',  ( 1.000000000000000000, 0.000000000000000000, -0.000000000000000000 ) ) ;
#18697=DIRECTION ( 'NONE',  ( -1.000000000000000000, -0.000000000000000000, -0.000000000000000000 ) ) ;
#18698=DIRECTION ( 'NONE',  ( 0.9947400562552481951, -0.1024315404614497965, 0.000000000000000000 ) ) ;
#18700=ORIENTED_EDGE ( 'NONE', *, *, #50509, .T. ) ;
#18701=DIRECTION ( 'NONE',  ( 1.000000000000000000, 0.000000000000000000, -0.000000000000000000 ) ) ;
#18706=DIRECTION ( 'NONE',  ( -1.000000000000000000, 0.000000000000000000, 0.000000000000000000 ) ) ;
#18707=EDGE_CURVE ( 'NONE', #62820, #27619, #20272, .T. ) ;
#18709=CARTESIAN_POINT ( 'NONE',  ( 5.126543808314632855, -10.38684015690950169, -6.021752670102713978 ) ) ;
#18710=LINE ( 'NONE', #54276, #5710 ) ;
#18711=ADVANCED_FACE ( 'NONE', ( #59889 ), #14311, .T. ) ;
#18712=CIRCLE ( 'NONE', #28243, 4.999999999999999112 ) ;
#18713=VERTEX_POINT ( 'NONE', #44905 ) ;
#18716=ORIENTED_EDGE ( 'NONE', *, *, #26056, .T. ) ;
#18719=DIRECTION ( 'NONE',  ( 1.000000000000000000, 0.000000000000000000, 0.000000000000000000 ) ) ;
#18724=DIRECTION ( 'NONE',  ( 0.000000000000000000, -0.4134677391718386552, -0.9105187689796012673 ) ) ;
#18725=AXIS2_PLACEMENT_3D ( 'NONE', #45305, #45970, #39983 ) ;
#18726=EDGE_LOOP ( 'NONE', ( #13618, #30551, #463, #44069 ) ) ;
#18727=ADVANCED_FACE ( 'NONE', ( #12769 ), #64616, .T. ) ;
#18729=CARTESIAN_POINT ( 'NONE',  ( 0.2851083653049504285, -0.4107471485392698018, 13.49374991542258151 ) ) ;
#18731=CARTESIAN_POINT ( 'NONE',  ( -35.00000000000000000, 4.824807283154122217, 11.80185301892982430 ) ) ;
#18732=VERTEX_POINT ( 'NONE', #19089 ) ;
#18735=CARTESIAN_POINT ( 'NONE',  ( -37.00000000000000711, -11.29812557209474733, -3.213188559034363401 ) ) ;
#18737=VERTEX_POINT ( 'NONE', #54012 ) ;
#18740=CARTESIAN_POINT ( 'NONE',  ( 35.00000000000000000, -11.61175578952786758, -1.771820996347120092 ) ) ;
#18741=ORIENTED_EDGE ( 'NONE', *, *, #42771, .T. ) ;
#18744=LINE ( 'NONE', #54317, #9592 ) ;
#18745=CARTESIAN_POINT ( 'NONE',  ( -35.00000000000000000, -5.556331110570326359, -11.47561260193582733 ) ) ;
#18747=LINE ( 'NONE', #39004, #4907 ) ;
#18748=CARTESIAN_POINT ( 'NONE',  ( -32.00000000000000000, 5.510910596163098430E-16, 0.000000000000000000 ) ) ;
#18749=ORIENTED_EDGE ( 'NONE', *, *, #8083, .F. ) ;
#18750=CARTESIAN_POINT ( 'NONE',  ( -4.979815405451806676, -1.249695498034863350, 13.44307378499100913 ) ) ;
#18752=VERTEX_POINT ( 'NONE', #9106 ) ;
#18754=CARTESIAN_POINT ( 'NONE',  ( -17.61421642177270996, -11.57952024119405721, 3.221331910940534726 ) ) ;
#18755=DIRECTION ( 'NONE',  ( 0.000000000000000000, 0.01356324068817991828, -0.9999080150203990547 ) ) ;
#18761=CARTESIAN_POINT ( 'NONE',  ( -11.40165637463000436, -7.508992741355388745, -9.360289953322599388 ) ) ;
#18762=AXIS2_PLACEMENT_3D ( 'NONE', #55579, #34928, #45583 ) ;
#18763=ORIENTED_EDGE ( 'NONE', *, *, #27584, .T. ) ;
#18766=CARTESIAN_POINT ( 'NONE',  ( 19.28625800530496903, 25.00000000000000000, 11.87904264843580471 ) ) ;
#18767=EDGE_CURVE ( 'NONE', #11975, #6620, #4346, .T. ) ;
#18768=CARTESIAN_POINT ( 'NONE',  ( -11.39386375410057539, -7.136722497414110578, 11.46148400915446075 ) ) ;
#18770=CARTESIAN_POINT ( 'NONE',  ( 11.32119323119160548, 0.8088561146804297275, -11.97325730400089050 ) ) ;
#18771=ADVANCED_FACE ( 'NONE', ( #18463 ), #3826, .T. ) ;
#18773=CYLINDRICAL_SURFACE ( 'NONE', #14942, 12.75000000000000178 ) ;
#18775=CARTESIAN_POINT ( 'NONE',  ( 3.409665710615477963, 3.588105730534572047, 11.45304521538101739 ) ) ;
#18776=EDGE_CURVE ( 'NONE', #21758, #19892, #1163, .T. ) ;
#18777=FACE_OUTER_BOUND ( 'NONE', #35506, .T. ) ;
#18781=ADVANCED_FACE ( 'NONE', ( #58347 ), #63635, .T. ) ;
#18783=DIRECTION ( 'NONE',  ( 1.000000000000000000, 0.000000000000000000, 0.000000000000000000 ) ) ;
#18784=VERTEX_POINT ( 'NONE', #49046 ) ;
#18787=ORIENTED_EDGE ( 'NONE', *, *, #14483, .F. ) ;
#18791=VECTOR ( 'NONE', #54299, 1000.000000000000000 ) ;
#18792=ORIENTED_EDGE ( 'NONE', *, *, #63079, .T. ) ;
#18793=EDGE_CURVE ( 'NONE', #26770, #40228, #46810, .T. ) ;
#18794=DIRECTION ( 'NONE',  ( -1.000000000000000000, 0.000000000000000000, -0.000000000000000000 ) ) ;
#18796=FACE_OUTER_BOUND ( 'NONE', #18888, .T. ) ;
#18797=CARTESIAN_POINT ( 'NONE',  ( 35.00000000000000000, -6.415447294506781084, -11.01837265713071190 ) ) ;
#18798=ADVANCED_FACE ( 'NONE', ( #13116 ), #18773, .T. ) ;
#18799=CARTESIAN_POINT ( 'NONE',  ( -35.00000000000000000, 11.72397916322013600, -0.7214809346827312231 ) ) ;
#18801=EDGE_LOOP ( 'NONE', ( #64337, #31490, #2613, #31206 ) ) ;
#18804=CYLINDRICAL_SURFACE ( 'NONE', #65641, 12.75000000000000178 ) ;
#18806=ORIENTED_EDGE ( 'NONE', *, *, #31827, .F. ) ;
#18808=CARTESIAN_POINT ( 'NONE',  ( -37.00000000000000711, -8.496612874013226957, 9.506317355798344693 ) ) ;
#18810=CARTESIAN_POINT ( 'NONE',  ( -24.31508151051078315, 10.66642090741561510, 8.277493316746310725 ) ) ;
#18811=CARTESIAN_POINT ( 'NONE',  ( -37.00000000000000711, -8.854740511458796703, -7.717887834988336415 ) ) ;
#18812=CARTESIAN_POINT ( 'NONE',  ( 3.426183256940671829, -10.95277051985667427, -4.917698437020843194 ) ) ;
#18813=FACE_OUTER_BOUND ( 'NONE', #46928, .T. ) ;
#18814=ORIENTED_EDGE ( 'NONE', *, *, #7105, .F. ) ;
#18815=CARTESIAN_POINT ( 'NONE',  ( 35.00000000000000000, 1.030638227056565048, -12.14284015767850278 ) ) ;
#18818=DIRECTION ( 'NONE',  ( 0.000000000000000000, -0.4935949184179134752, 0.8696919319575254770 ) ) ;
#18819=ORIENTED_EDGE ( 'NONE', *, *, #6263, .F. ) ;
#18820=DIRECTION ( 'NONE',  ( 1.000000000000000000, 0.000000000000000000, 0.000000000000000000 ) ) ;
#18821=CARTESIAN_POINT ( 'NONE',  ( -37.00000000000000711, -9.076753354954062658, 8.954052073409570767 ) ) ;
#18826=DIRECTION ( 'NONE',  ( -0.7886918350401329603, -0.6147887355352468219, 0.000000000000000000 ) ) ;
#18827=CARTESIAN_POINT ( 'NONE',  ( -37.00000000000000711, -7.817492529713920391, 9.348667969174380588 ) ) ;
#18829=ORIENTED_EDGE ( 'NONE', *, *, #59501, .F. ) ;
#18830=CARTESIAN_POINT ( 'NONE',  ( -35.00000000000000000, 0.000000000000000000, 0.000000000000000000 ) ) ;
#18831=DIRECTION ( 'NONE',  ( 1.000000000000000000, 0.000000000000000000, 0.000000000000000000 ) ) ;
#18833=AXIS2_PLACEMENT_3D ( 'NONE', #34580, #53903, #54571 ) ;
#18836=EDGE_CURVE ( 'NONE', #9845, #37953, #40331, .T. ) ;
#18837=CARTESIAN_POINT ( 'NONE',  ( -27.45775109278350712, 13.35262336282554152, -1.989333891161978674 ) ) ;
#18838=VECTOR ( 'NONE', #1224, 1000.000000000000000 ) ;
#18840=CARTESIAN_POINT ( 'NONE',  ( -9.082173403709882464, -3.146272781168804045, -11.58446707970393774 ) ) ;
#18841=CARTESIAN_POINT ( 'NONE',  ( 35.00000000000000000, -5.428340790341627198, 10.91072401419415883 ) ) ;
#18843=DIRECTION ( 'NONE',  ( 0.000000000000000000, -0.6745969609292717939, -0.7381862504171901040 ) ) ;
#18845=ORIENTED_EDGE ( 'NONE', *, *, #13824, .F. ) ;
#18846=CARTESIAN_POINT ( 'NONE',  ( -37.00000000000000711, -12.12087942037210553, 1.262958560998716617 ) ) ;
#18851=ORIENTED_EDGE ( 'NONE', *, *, #396, .F. ) ;
#18854=EDGE_CURVE ( 'NONE', #19934, #65334, #56393, .T. ) ;
#18856=ORIENTED_EDGE ( 'NONE', *, *, #43704, .F. ) ;
#18857=CARTESIAN_POINT ( 'NONE',  ( -9.961160847258154760, -3.372123831127339155, -13.07617202219271135 ) ) ;
#18858=CARTESIAN_POINT ( 'NONE',  ( 35.00000000000000000, 4.705694406421931860E-17, -3.469127814946512892E-15 ) ) ;
#18860=ADVANCED_FACE ( 'NONE', ( #65595 ), #35002, .T. ) ;
#18866=EDGE_CURVE ( 'NONE', #49313, #55012, #24738, .T. ) ;
#18871=AXIS2_PLACEMENT_3D ( 'NONE', #28546, #63779, #33547 ) ;
#18875=DIRECTION ( 'NONE',  ( -1.000000000000000000, -1.836970198721029688E-16, -0.000000000000000000 ) ) ;
#18878=CYLINDRICAL_SURFACE ( 'NONE', #48872, 12.74999999999999822 ) ;
#18883=CIRCLE ( 'NONE', #44344, 5.000000000000000888 ) ;
#18885=CARTESIAN_POINT ( 'NONE',  ( 37.00000000000000711, 0.06441628369836321921, -12.18632975068353019 ) ) ;
#18886=CIRCLE ( 'NONE', #58191, 12.74999999999999822 ) ;
#18887=CARTESIAN_POINT ( 'NONE',  ( 47.00000000000000711, 4.705694406421931860E-17, -3.469127814946512892E-15 ) ) ;
#18888=EDGE_LOOP ( 'NONE', ( #34349, #18741, #16001, #39312 ) ) ;
#18890=DIRECTION ( 'NONE',  ( 1.000000000000000000, -0.000000000000000000, 0.000000000000000000 ) ) ;
#18892=ORIENTED_EDGE ( 'NONE', *, *, #63921, .F. ) ;
#18893=ORIENTED_EDGE ( 'NONE', *, *, #24661, .F. ) ;
#18896=ORIENTED_EDGE ( 'NONE', *, *, #60275, .T. ) ;
#18897=ORIENTED_EDGE ( 'NONE', *, *, #38279, .F. ) ;
#18898=CARTESIAN_POINT ( 'NONE',  ( 12.51043607184429796, 0.3316456940255351760, 13.49694458083817672 ) ) ;
#18900=EDGE_CURVE ( 'NONE', #55595, #39189, #1204, .T. ) ;
#18902=DIRECTION ( 'NONE',  ( 1.000000000000000000, 0.000000000000000000, 0.000000000000000000 ) ) ;
#18903=CYLINDRICAL_SURFACE ( 'NONE', #53538, 13.50000000000000178 ) ;
#18904=EDGE_CURVE ( 'NONE', #22729, #47974, #60675, .T. ) ;
#18905=ORIENTED_EDGE ( 'NONE', *, *, #50082, .T. ) ;
#18906=B_SPLINE_CURVE_WITH_KNOTS ( 'NONE', 3,
 ( #39427, #3571, #34104, #4539, #13814, #3884, #33779, #39098, #29447, #53765, #3225, #8201, #34748, #18837 ),
 .UNSPECIFIED., .F., .F.,
 ( 4, 2, 2, 2, 2, 2, 4 ),
 ( 0.000000000000000000, 0.001838460847883235504, 0.002757691271824853040, 0.003676921695766471009, 0.004596152119708088978, 0.005515382543649706079, 0.007353843391532942017 ),
 .UNSPECIFIED. ) ;
#18910=DIRECTION ( 'NONE',  ( 1.000000000000000000, 0.000000000000000000, -0.000000000000000000 ) ) ;
#18913=CARTESIAN_POINT ( 'NONE',  ( -35.00000000000000000, -8.366449238204298311, -9.621072037177086145 ) ) ;
#18914=CARTESIAN_POINT ( 'NONE',  ( 37.00000000000000711, 7.238157050195626496, -10.49626516989273384 ) ) ;
#18915=EDGE_CURVE ( 'NONE', #22151, #43665, #15713, .T. ) ;
#18916=VECTOR ( 'NONE', #10608, 1000.000000000000000 ) ;
#18917=ORIENTED_EDGE ( 'NONE', *, *, #46912, .F. ) ;
#18919=AXIS2_PLACEMENT_3D ( 'NONE', #28326, #22696, #52937 ) ;
#18920=VERTEX_POINT ( 'NONE', #25716 ) ;
#18923=CARTESIAN_POINT ( 'NONE',  ( -16.15963131418214971, 7.828775782396976801, -10.99875241953665927 ) ) ;
#18924=AXIS2_PLACEMENT_3D ( 'NONE', #11441, #52995, #22400 ) ;
#18925=DIRECTION ( 'NONE',  ( 0.000000000000000000, -0.01356324068817992175, 0.9999080150203990547 ) ) ;
#18926=EDGE_CURVE ( 'NONE', #10959, #35622, #24596, .T. ) ;
#18928=DIRECTION ( 'NONE',  ( 1.000000000000000000, 0.000000000000000000, -0.000000000000000000 ) ) ;
#18929=CARTESIAN_POINT ( 'NONE',  ( 35.00000000000000000, 12.01765980939841683, -2.021542716731445921 ) ) ;
#18933=EDGE_CURVE ( 'NONE', #12489, #10479, #7611, .T. ) ;
#18934=DIRECTION ( 'NONE',  ( 0.000000000000000000, 0.9246979985058709772, 0.3807014730195252272 ) ) ;
#18935=EDGE_LOOP ( 'NONE', ( #50703, #8134, #48127, #35894 ) ) ;
#18937=VERTEX_POINT ( 'NONE', #32634 ) ;
#18939=DIRECTION ( 'NONE',  ( 1.000000000000000000, 0.000000000000000000, 0.000000000000000000 ) ) ;
#18940=DIRECTION ( 'NONE',  ( 1.000000000000000000, 0.000000000000000000, 0.000000000000000000 ) ) ;
#18942=EDGE_CURVE ( 'NONE', #60252, #65370, #47323, .T. ) ;
#18943=ORIENTED_EDGE ( 'NONE', *, *, #58044, .F. ) ;
#18944=ORIENTED_EDGE ( 'NONE', *, *, #50552, .F. ) ;
#18945=DIRECTION ( 'NONE',  ( 0.000000000000000000, -0.8009703041134234036, -0.5987040770935587730 ) ) ;
#18946=ADVANCED_FACE ( 'NONE', ( #2076 ), #7377, .T. ) ;
#18947=DIRECTION ( 'NONE',  ( 1.000000000000000000, 0.000000000000000000, 0.000000000000000000 ) ) ;
#18948=DIRECTION ( 'NONE',  ( 1.000000000000000000, -0.000000000000000000, 0.000000000000000000 ) ) ;
#18950=AXIS2_PLACEMENT_3D ( 'NONE', #2888, #52100, #37451 ) ;
#18953=DIRECTION ( 'NONE',  ( 0.000000000000000000, 0.9796553971857735466, 0.2006870767258926436 ) ) ;
#18956=VERTEX_POINT ( 'NONE', #46646 ) ;
#18958=AXIS2_PLACEMENT_3D ( 'NONE', #36216, #41875, #993 ) ;
#18961=ADVANCED_FACE ( 'NONE', ( #22026 ), #31665, .T. ) ;
#18963=CARTESIAN_POINT ( 'NONE',  ( 35.00000000000000000, 12.38385022362085941, 3.033604067594442011 ) ) ;
#18966=AXIS2_PLACEMENT_3D ( 'NONE', #11429, #37019, #27373 ) ;
#18967=DIRECTION ( 'NONE',  ( 0.000000000000000000, -0.01356324068817998940, 0.9999080150203990547 ) ) ;
#18968=CARTESIAN_POINT ( 'NONE',  ( -30.18541646480309026, -1.416020129149132334, -13.42553116244734746 ) ) ;
#18970=EDGE_LOOP ( 'NONE', ( #25876, #43112, #44831, #19446 ) ) ;
#18972=AXIS2_PLACEMENT_3D ( 'NONE', #44557, #64839, #31568 ) ;
#18975=CARTESIAN_POINT ( 'NONE',  ( 10.75853767213705048, 7.830989516993144051, 10.99661780661416088 ) ) ;
#18977=VERTEX_POINT ( 'NONE', #51660 ) ;
#18978=AXIS2_PLACEMENT_3D ( 'NONE', #27820, #48123, #2580 ) ;
#18982=DIRECTION ( 'NONE',  ( -1.000000000000000000, 0.000000000000000000, 0.000000000000000000 ) ) ;
#18984=FACE_OUTER_BOUND ( 'NONE', #49254, .T. ) ;
#18987=EDGE_CURVE ( 'NONE', #63181, #58825, #24547, .T. ) ;
#18988=EDGE_LOOP ( 'NONE', ( #36204, #16924, #11205, #23249 ) ) ;
#18989=CYLINDRICAL_SURFACE ( 'NONE', #6252, 13.50000000000000178 ) ;
#18994=VERTEX_POINT ( 'NONE', #6420 ) ;
#18995=CIRCLE ( 'NONE', #10472, 5.000000000000000000 ) ;
#18996=ORIENTED_EDGE ( 'NONE', *, *, #47374, .T. ) ;
#18998=AXIS2_PLACEMENT_3D ( 'NONE', #56017, #31412, #6152 ) ;
#18999=ORIENTED_EDGE ( 'NONE', *, *, #29515, .T. ) ;
#19000=CARTESIAN_POINT ( 'NONE',  ( -35.00000000000000000, -0.06441628369844946966, 12.18632975068352842 ) ) ;
#19001=PLANE ( 'NONE',  #15969 ) ;
#19003=LINE ( 'NONE', #8701, #44709 ) ;
#19004=CARTESIAN_POINT ( 'NONE',  ( 10.13479916714561568, 11.98071251699297690, -0.6877595805417434649 ) ) ;
#19006=VERTEX_POINT ( 'NONE', #16048 ) ;
#19008=CARTESIAN_POINT ( 'NONE',  ( -30.07634502127111631, -2.989967992425739851, 13.17072238577171106 ) ) ;
#19009=ADVANCED_FACE ( 'NONE', ( #42614 ), #56646, .T. ) ;
#19011=AXIS2_PLACEMENT_3D ( 'NONE', #13204, #3237, #30038 ) ;
#19014=CIRCLE ( 'NONE', #27492, 5.000000000000000888 ) ;
#19018=CARTESIAN_POINT ( 'NONE',  ( -37.00000000000000711, 6.303578524886947143, 10.42955799785322490 ) ) ;
#19020=EDGE_CURVE ( 'NONE', #54027, #65390, #1763, .T. ) ;
#19021=VERTEX_POINT ( 'NONE', #11082 ) ;
#19023=( BOUNDED_CURVE ( )  B_SPLINE_CURVE ( 3, ( #62415, #37150, #57460, #11883 ),
 .UNSPECIFIED., .F., .F. ) 
 B_SPLINE_CURVE_WITH_KNOTS ( ( 4, 4 ),
 ( 1.481266777651250033, 1.521986778384522232 ),
 .UNSPECIFIED. ) 
 CURVE ( )  GEOMETRIC_REPRESENTATION_ITEM ( )  RATIONAL_B_SPLINE_CURVE ( ( 1.000000000000000000, 0.9998618282348130659, 0.9998618282348130659, 1.000000000000000000 ) ) 
 REPRESENTATION_ITEM ( '' )  );
#19024=EDGE_LOOP ( 'NONE', ( #57865, #15311, #64105, #10898 ) ) ;
#19026=CARTESIAN_POINT ( 'NONE',  ( 36.00000000000000711, -12.49688848680882103, 2.527899948230769578 ) ) ;
#19032=CARTESIAN_POINT ( 'NONE',  ( 29.63669315105201463, -8.416703354620286959, 10.56457041555997378 ) ) ;
#19033=ADVANCED_FACE ( 'NONE', ( #21377 ), #62259, .T. ) ;
#19034=CIRCLE ( 'NONE', #39195, 4.999999999999999112 ) ;
#19037=FACE_OUTER_BOUND ( 'NONE', #40274, .T. ) ;
#19040=ORIENTED_EDGE ( 'NONE', *, *, #58267, .F. ) ;
#19041=CARTESIAN_POINT ( 'NONE',  ( -37.00000000000000711, 5.556331110570408960, 11.47561260193578825 ) ) ;
#19046=ORIENTED_EDGE ( 'NONE', *, *, #62585, .T. ) ;
#19048=ORIENTED_EDGE ( 'NONE', *, *, #48222, .T. ) ;
#19051=CARTESIAN_POINT ( 'NONE',  ( -35.00000000000000000, -10.80631716521663854, -4.603882218679666849 ) ) ;
#19052=AXIS2_PLACEMENT_3D ( 'NONE', #39451, #50108, #59415 ) ;
#19053=DIRECTION ( 'NONE',  ( 0.000000000000000000, -0.01356324068817998940, 0.9999080150203990547 ) ) ;
#19054=CARTESIAN_POINT ( 'NONE',  ( -2.812214508280806324, 11.36735472963162508, 3.846083643116565920 ) ) ;
#19056=DIRECTION ( 'NONE',  ( -1.000000000000000000, 0.000000000000000000, 0.000000000000000000 ) ) ;
#19060=AXIS2_PLACEMENT_3D ( 'NONE', #44045, #34389, #59671 ) ;
#19061=ADVANCED_FACE ( 'NONE', ( #57629 ), #12367, .T. ) ;
#19062=VERTEX_POINT ( 'NONE', #12048 ) ;
#19063=CARTESIAN_POINT ( 'NONE',  ( 19.67311005600952711, -0.7004819783312107306, 25.00000000000000000 ) ) ;
#19064=EDGE_LOOP ( 'NONE', ( #18067, #50932, #60254, #62100 ) ) ;
#19065=EDGE_CURVE ( 'NONE', #37445, #10053, #30949, .T. ) ;
#19066=VERTEX_POINT ( 'NONE', #7065 ) ;
#19067=FACE_OUTER_BOUND ( 'NONE', #1664, .T. ) ;
#19068=CARTESIAN_POINT ( 'NONE',  ( 37.00000000000000711, 10.62137734850267989, 5.015831474386340361 ) ) ;
#19069=AXIS2_PLACEMENT_3D ( 'NONE', #52304, #16033, #36327 ) ;
#19070=CARTESIAN_POINT ( 'NONE',  ( 37.00000000000000711, 4.705694406421931860E-17, -3.469127814946512892E-15 ) ) ;
#19074=EDGE_CURVE ( 'NONE', #54100, #20923, #61700, .T. ) ;
#19075=LINE ( 'NONE', #5098, #33275 ) ;
#19076=AXIS2_PLACEMENT_3D ( 'NONE', #9313, #4360, #14624 ) ;
#19078=CARTESIAN_POINT ( 'NONE',  ( -35.00000000000000000, -3.704519465651227694, -11.60979404548638705 ) ) ;
#19083=VERTEX_POINT ( 'NONE', #8379 ) ;
#19085=AXIS2_PLACEMENT_3D ( 'NONE', #29518, #4269, #56799 ) ;
#19088=ORIENTED_EDGE ( 'NONE', *, *, #33756, .F. ) ;
#19089=CARTESIAN_POINT ( 'NONE',  ( 35.00000000000000000, -12.05416472667166516, -1.791059740004382617 ) ) ;
#19092=AXIS2_PLACEMENT_3D ( 'NONE', #57379, #23357, #57722 ) ;
#19093=CARTESIAN_POINT ( 'NONE',  ( 35.00000000000000000, -5.391785509271032062, -10.43555801961473861 ) ) ;
#19096=ORIENTED_EDGE ( 'NONE', *, *, #45550, .T. ) ;
#19097=DIRECTION ( 'NONE',  ( 0.000000000000000000, 0.01356324068817998940, -0.9999080150203990547 ) ) ;
#19098=LINE ( 'NONE', #39046, #4527 ) ;
#19101=PLANE ( 'NONE',  #18094 ) ;
#19103=VERTEX_POINT ( 'NONE', #38641 ) ;
#19104=EDGE_CURVE ( 'NONE', #11231, #6620, #53225, .T. ) ;
#19105=VECTOR ( 'NONE', #41860, 1000.000000000000000 ) ;
#19106=VERTEX_POINT ( 'NONE', #2424 ) ;
#19107=CARTESIAN_POINT ( 'NONE',  ( -35.00000000000000000, -2.185196060783795691, -11.54110654723651486 ) ) ;
#19108=EDGE_CURVE ( 'NONE', #2190, #9138, #27768, .T. ) ;
#19110=DIRECTION ( 'NONE',  ( 1.000000000000000000, 0.000000000000000000, 0.000000000000000000 ) ) ;
#19111=DIRECTION ( 'NONE',  ( 0.000000000000000000, 0.000000000000000000, -1.000000000000000000 ) ) ;
#19112=PLANE ( 'NONE',  #35406 ) ;
#19113=CYLINDRICAL_SURFACE ( 'NONE', #61634, 12.75000000000000178 ) ;
#19115=FACE_OUTER_BOUND ( 'NONE', #16190, .T. ) ;
#19116=ORIENTED_EDGE ( 'NONE', *, *, #65276, .T. ) ;
#19117=DIRECTION ( 'NONE',  ( 0.000000000000000000, 0.01356324068817998940, -0.9999080150203990547 ) ) ;
#19118=ORIENTED_EDGE ( 'NONE', *, *, #13906, .T. ) ;
#19120=ORIENTED_EDGE ( 'NONE', *, *, #3034, .T. ) ;
#19121=ORIENTED_EDGE ( 'NONE', *, *, #44997, .F. ) ;
#19122=CARTESIAN_POINT ( 'NONE',  ( -26.94359064758800670, 12.23578565015750286, 5.704334401058154036 ) ) ;
#19125=ADVANCED_FACE ( 'NONE', ( #47969 ), #58618, .T. ) ;
#19126=CIRCLE ( 'NONE', #60512, 4.999999999999999112 ) ;
#19127=CARTESIAN_POINT ( 'NONE',  ( -35.00000000000000000, 0.000000000000000000, 0.000000000000000000 ) ) ;
#19128=DIRECTION ( 'NONE',  ( 1.000000000000000000, 0.000000000000000000, 0.000000000000000000 ) ) ;
#19134=EDGE_CURVE ( 'NONE', #56264, #13249, #33649, .T. ) ;
#19135=ORIENTED_EDGE ( 'NONE', *, *, #32590, .T. ) ;
#19136=CARTESIAN_POINT ( 'NONE',  ( 37.00000000000000711, 4.705694406421931860E-17, -3.469127814946512892E-15 ) ) ;
#19138=DIRECTION ( 'NONE',  ( -1.000000000000000000, 0.000000000000000000, 0.000000000000000000 ) ) ;
#19139=CARTESIAN_POINT ( 'NONE',  ( -27.27855387000350262, 10.59660315834921640, 5.631341004100471892 ) ) ;
#19140=AXIS2_PLACEMENT_3D ( 'NONE', #26548, #42152, #15580 ) ;
#19142=ADVANCED_FACE ( 'NONE', ( #58272 ), #14010, .T. ) ;
#19144=AXIS2_PLACEMENT_3D ( 'NONE', #42464, #11899, #58454 ) ;
#19149=CARTESIAN_POINT ( 'NONE',  ( 35.00000000000000000, 4.705694406421931860E-17, -3.469127814946512892E-15 ) ) ;
#19150=AXIS2_PLACEMENT_3D ( 'NONE', #58397, #11837, #12822 ) ;
#19151=CARTESIAN_POINT ( 'NONE',  ( 6.511276587883020106, -4.283181266385641450, -12.80273922584868629 ) ) ;
#19152=CARTESIAN_POINT ( 'NONE',  ( -18.25006854224444908, -9.443202773001939221, -7.404452808139720510 ) ) ;
#19156=CARTESIAN_POINT ( 'NONE',  ( 7.238144804251998465, -5.479122853610516763, -12.33991764455425866 ) ) ;
#19158=CARTESIAN_POINT ( 'NONE',  ( 35.00000000000000000, 4.705694406421931860E-17, -3.469127814946512892E-15 ) ) ;
#19159=CARTESIAN_POINT ( 'NONE',  ( -37.00000000000000711, -6.711949091238219367, 10.84030624090604356 ) ) ;
#19160=AXIS2_PLACEMENT_3D ( 'NONE', #35765, #60400, #55423 ) ;
#19161=EDGE_LOOP ( 'NONE', ( #7350, #16655, #23521, #65801 ) ) ;
#19166=CIRCLE ( 'NONE', #35046, 12.18650000000000055 ) ;
#19170=EDGE_LOOP ( 'NONE', ( #7243, #55004, #13299, #31394 ) ) ;
#19174=VERTEX_POINT ( 'NONE', #13362 ) ;
#19175=DIRECTION ( 'NONE',  ( 0.000000000000000000, 0.01356324068818000848, -0.9999080150203990547 ) ) ;
#19176=CARTESIAN_POINT ( 'NONE',  ( -27.74257803791718402, -13.27121782910951353, -2.535736602234749171 ) ) ;
#19177=CARTESIAN_POINT ( 'NONE',  ( -35.00000000000000000, 12.17626345777664376, -0.4993900848166082374 ) ) ;
#19178=DIRECTION ( 'NONE',  ( 0.000000000000000000, -0.01356324068817998940, 0.9999080150203990547 ) ) ;
#19179=CARTESIAN_POINT ( 'NONE',  ( -9.843523776114507129, -12.00711794201791172, -6.183557206441264498 ) ) ;
#19180=AXIS2_PLACEMENT_3D ( 'NONE', #30068, #54384, #13457 ) ;
#19183=ORIENTED_EDGE ( 'NONE', *, *, #8866, .T. ) ;
#19184=CIRCLE ( 'NONE', #35106, 12.18650000000000055 ) ;
#19188=CARTESIAN_POINT ( 'NONE',  ( -14.79101291032822019, 8.427946710105242545, -10.54609284329090535 ) ) ;
#19192=AXIS2_PLACEMENT_3D ( 'NONE', #63962, #13416, #14070 ) ;
#19193=CARTESIAN_POINT ( 'NONE',  ( 37.00000000000000711, 12.49688848680884234, -2.527899948230686977 ) ) ;
#19195=ORIENTED_EDGE ( 'NONE', *, *, #5471, .F. ) ;
#19196=EDGE_LOOP ( 'NONE', ( #39225, #47840, #47941, #25065 ) ) ;
#19197=DIRECTION ( 'NONE',  ( 1.000000000000000000, 0.000000000000000000, 0.000000000000000000 ) ) ;
#19198=AXIS2_PLACEMENT_3D ( 'NONE', #60856, #15296, #35572 ) ;
#19203=ORIENTED_EDGE ( 'NONE', *, *, #51971, .F. ) ;
#19207=EDGE_CURVE ( 'NONE', #20112, #395, #34115, .T. ) ;
#19208=CARTESIAN_POINT ( 'NONE',  ( 24.52718794524056278, -2.675527299323683383, 13.23708621095143201 ) ) ;
#19210=VERTEX_POINT ( 'NONE', #9669 ) ;
#19212=VECTOR ( 'NONE', #29091, 1000.000000000000000 ) ;
#19215=ORIENTED_EDGE ( 'NONE', *, *, #28704, .T. ) ;
#19216=DIRECTION ( 'NONE',  ( 1.000000000000000000, -0.000000000000000000, 0.000000000000000000 ) ) ;
#19217=ORIENTED_EDGE ( 'NONE', *, *, #51064, .T. ) ;
#19218=CARTESIAN_POINT ( 'NONE',  ( -35.00000000000000000, 11.10408318471068512, -6.265926637539371846 ) ) ;
#19221=DIRECTION ( 'NONE',  ( 0.000000000000000000, 0.01356324068817992001, -0.9999080150203990547 ) ) ;
#19224=VERTEX_POINT ( 'NONE', #380 ) ;
#19225=( BOUNDED_CURVE ( )  B_SPLINE_CURVE ( 3, ( #48658, #13391, #33675, #59947 ),
 .UNSPECIFIED., .F., .F. ) 
 B_SPLINE_CURVE_WITH_KNOTS ( ( 4, 4 ),
 ( 5.020709631077181712, 5.030260039792340265 ),
 .UNSPECIFIED. ) 
 CURVE ( )  GEOMETRIC_REPRESENTATION_ITEM ( )  RATIONAL_B_SPLINE_CURVE ( ( 1.000000000000000000, 0.9999923991555577096, 0.9999923991555577096, 1.000000000000000000 ) ) 
 REPRESENTATION_ITEM ( '' )  );
#19231=EDGE_CURVE ( 'NONE', #24479, #13166, #49024, .T. ) ;
#19237=CARTESIAN_POINT ( 'NONE',  ( -35.00000000000000000, 5.391785509270962784, 10.43555801961477236 ) ) ;
#19239=CIRCLE ( 'NONE', #46865, 12.18650000000000055 ) ;
#19241=EDGE_LOOP ( 'NONE', ( #30416, #52508, #2523, #38093 ) ) ;
#19242=CARTESIAN_POINT ( 'NONE',  ( -37.00000000000000711, 5.143145423404449801, -11.66664283989674367 ) ) ;
#19243=AXIS2_PLACEMENT_3D ( 'NONE', #34444, #8851, #4190 ) ;
#19244=EDGE_CURVE ( 'NONE', #49413, #55105, #30299, .T. ) ;
#19246=ORIENTED_EDGE ( 'NONE', *, *, #35481, .T. ) ;
#19247=DIRECTION ( 'NONE',  ( 1.000000000000000000, 0.000000000000000000, 0.000000000000000000 ) ) ;
#19248=LINE ( 'NONE', #9914, #58492 ) ;
#19250=CIRCLE ( 'NONE', #14953, 5.000000000000002665 ) ;
#19251=EDGE_CURVE ( 'NONE', #21398, #58025, #2309, .T. ) ;
#19253=DIRECTION ( 'NONE',  ( -1.000000000000000000, 0.000000000000000000, 0.000000000000000000 ) ) ;
#19255=CARTESIAN_POINT ( 'NONE',  ( -11.40165637463000614, -7.508992741355387857, -11.21895841913464587 ) ) ;
#19256=CARTESIAN_POINT ( 'NONE',  ( -35.00000000000000000, -11.35427606708809556, 4.426194442447198618 ) ) ;
#19257=CIRCLE ( 'NONE', #38370, 5.000000000000001776 ) ;
#19259=DIRECTION ( 'NONE',  ( -1.000000000000000000, 0.000000000000000000, 0.000000000000000000 ) ) ;
#19260=CIRCLE ( 'NONE', #64895, 5.000000000000000000 ) ;
#19261=CARTESIAN_POINT ( 'NONE',  ( -47.00000000000000711, 0.000000000000000000, 0.000000000000000000 ) ) ;
#19262=ORIENTED_EDGE ( 'NONE', *, *, #20837, .T. ) ;
#19263=DIRECTION ( 'NONE',  ( 0.000000000000000000, 0.000000000000000000, -1.000000000000000000 ) ) ;
#19264=ORIENTED_EDGE ( 'NONE', *, *, #53695, .F. ) ;
#19265=CIRCLE ( 'NONE', #50073, 5.000000000000000000 ) ;
#19267=DIRECTION ( 'NONE',  ( -1.000000000000000000, -0.000000000000000000, -0.000000000000000000 ) ) ;
#19268=CYLINDRICAL_SURFACE ( 'NONE', #27822, 12.18649999999999878 ) ;
#19270=CIRCLE ( 'NONE', #44736, 12.74999999999999822 ) ;
#19272=VECTOR ( 'NONE', #47075, 1000.000000000000000 ) ;
#19274=ORIENTED_EDGE ( 'NONE', *, *, #7991, .F. ) ;
#19275=DIRECTION ( 'NONE',  ( 0.000000000000000000, 0.01356324068817998940, -0.9999080150203990547 ) ) ;
#19276=LINE ( 'NONE', #39544, #47856 ) ;
#19277=LINE ( 'NONE', #20243, #51296 ) ;
#19283=EDGE_CURVE ( 'NONE', #14292, #61981, #46868, .T. ) ;
#19287=CIRCLE ( 'NONE', #62796, 5.000000000000000888 ) ;
#19288=AXIS2_PLACEMENT_3D ( 'NONE', #28653, #48963, #18375 ) ;
#19291=DIRECTION ( 'NONE',  ( -1.000000000000000000, 0.000000000000000000, 0.000000000000000000 ) ) ;
#19292=FACE_BOUND ( 'NONE', #64168, .T. ) ;
#19293=ORIENTED_EDGE ( 'NONE', *, *, #47441, .F. ) ;
#19296=CARTESIAN_POINT ( 'NONE',  ( 5.887998910375843664, -9.753598045600698541, 7.002626515174585897 ) ) ;
#19297=ORIENTED_EDGE ( 'NONE', *, *, #29269, .T. ) ;
#19298=AXIS2_PLACEMENT_3D ( 'NONE', #34714, #63665, #13150 ) ;
#19300=LINE ( 'NONE', #50225, #19347 ) ;
#19301=ADVANCED_FACE ( 'NONE', ( #11646 ), #21646, .T. ) ;
#19302=VERTEX_POINT ( 'NONE', #1028 ) ;
#19303=DIRECTION ( 'NONE',  ( 1.000000000000000000, 0.000000000000000000, 0.000000000000000000 ) ) ;
#19304=ORIENTED_EDGE ( 'NONE', *, *, #8004, .T. ) ;
#19305=AXIS2_PLACEMENT_3D ( 'NONE', #18171, #12184, #38441 ) ;
#19306=ORIENTED_EDGE ( 'NONE', *, *, #6020, .F. ) ;
#19307=ORIENTED_EDGE ( 'NONE', *, *, #60490, .F. ) ;
#19310=CARTESIAN_POINT ( 'NONE',  ( -35.00000000000000000, 2.696588552979059639, 12.46157735505190089 ) ) ;
#19311=LINE ( 'NONE', #44899, #47880 ) ;
#19312=FACE_OUTER_BOUND ( 'NONE', #21841, .T. ) ;
#19313=VERTEX_POINT ( 'NONE', #52572 ) ;
#19315=AXIS2_PLACEMENT_3D ( 'NONE', #42341, #22082, #26421 ) ;
#19317=DIRECTION ( 'NONE',  ( 0.000000000000000000, 0.01356324068817998940, -0.9999080150203989437 ) ) ;
#19319=AXIS2_PLACEMENT_3D ( 'NONE', #29024, #44961, #18407 ) ;
#19321=VERTEX_POINT ( 'NONE', #5706 ) ;
#19322=DIRECTION ( 'NONE',  ( 0.000000000000000000, 0.01356324068817992175, -0.9999080150203990547 ) ) ;
#19323=CARTESIAN_POINT ( 'NONE',  ( -35.00000000000000000, 0.000000000000000000, 0.000000000000000000 ) ) ;
#19328=AXIS2_PLACEMENT_3D ( 'NONE', #30265, #56178, #10616 ) ;
#19332=ADVANCED_FACE ( 'NONE', ( #42537 ), #15965, .T. ) ;
#19334=CARTESIAN_POINT ( 'NONE',  ( -36.00000000000000711, 9.913596905230114942, 8.017674001891819557 ) ) ;
#19335=CARTESIAN_POINT ( 'NONE',  ( 37.00000000000000711, -11.66953048682396954, 3.511814412392239682 ) ) ;
#19337=EDGE_CURVE ( 'NONE', #30904, #7231, #52238, .T. ) ;
#19344=CIRCLE ( 'NONE', #56498, 12.75000000000000178 ) ;
#19345=CIRCLE ( 'NONE', #64974, 12.18649999999999878 ) ;
#19347=VECTOR ( 'NONE', #4684, 1000.000000000000000 ) ;
#19350=DIRECTION ( 'NONE',  ( 1.000000000000000000, -0.000000000000000000, 0.000000000000000000 ) ) ;
#19351=CARTESIAN_POINT ( 'NONE',  ( -35.00000000000000000, 9.348667969174405457, 7.817492529713891081 ) ) ;
#19356=AXIS2_PLACEMENT_3D ( 'NONE', #22250, #42511, #17275 ) ;
#19358=ORIENTED_EDGE ( 'NONE', *, *, #25830, .F. ) ;
#19360=DIRECTION ( 'NONE',  ( -1.000000000000000000, -0.000000000000000000, 0.000000000000000000 ) ) ;
#19361=DIRECTION ( 'NONE',  ( 0.000000000000000000, -0.01356324068817998940, 0.9999080150203990547 ) ) ;
#19363=VERTEX_POINT ( 'NONE', #51587 ) ;
#19364=EDGE_CURVE ( 'NONE', #52959, #44677, #46572, .T. ) ;
#19366=ORIENTED_EDGE ( 'NONE', *, *, #44004, .F. ) ;
#19367=CARTESIAN_POINT ( 'NONE',  ( 29.61403717302718519, -5.490544854489863624, 10.71644165484303457 ) ) ;
#19368=CIRCLE ( 'NONE', #34208, 5.000000000000000888 ) ;
#19369=CARTESIAN_POINT ( 'NONE',  ( -27.73962451255497541, 10.56031772329400731, -5.706676279454582890 ) ) ;
#19375=DIRECTION ( 'NONE',  ( -1.000000000000000000, 0.000000000000000000, 0.000000000000000000 ) ) ;
#19377=ORIENTED_EDGE ( 'NONE', *, *, #50298, .T. ) ;
#19378=CARTESIAN_POINT ( 'NONE',  ( 37.00000000000000711, 4.705694406421931860E-17, -3.469127814946512892E-15 ) ) ;
#19380=DIRECTION ( 'NONE',  ( 1.000000000000000000, 0.000000000000000000, 0.000000000000000000 ) ) ;
#19382=VERTEX_POINT ( 'NONE', #3007 ) ;
#19383=EDGE_CURVE ( 'NONE', #52549, #23040, #43210, .T. ) ;
#19386=CYLINDRICAL_SURFACE ( 'NONE', #64509, 12.75000000000000178 ) ;
#19388=CARTESIAN_POINT ( 'NONE',  ( -29.68541646480307605, -0.9852353464181112797, -11.96735172698778626 ) ) ;
#19390=CARTESIAN_POINT ( 'NONE',  ( 13.03306451323199155, -11.51507849167763631, -3.383716369314965888 ) ) ;
#19391=EDGE_CURVE ( 'NONE', #44608, #60941, #38563, .T. ) ;
#19394=CIRCLE ( 'NONE', #58662, 12.18650000000000233 ) ;
#19395=CARTESIAN_POINT ( 'NONE',  ( 36.00000000000000711, -0.3137578094510115045, -12.74613886779085092 ) ) ;
#19396=CARTESIAN_POINT ( 'NONE',  ( -8.071794517351818854, -2.346129881092677838, -13.29681922941937344 ) ) ;
#19398=DIRECTION ( 'NONE',  ( 0.000000000000000000, -0.9718671068226484300, 0.2355298848897411923 ) ) ;
#19399=ORIENTED_EDGE ( 'NONE', *, *, #42682, .F. ) ;
#19401=LINE ( 'NONE', #20043, #876 ) ;
#19402=ORIENTED_EDGE ( 'NONE', *, *, #47300, .F. ) ;
#19403=CIRCLE ( 'NONE', #35322, 12.74999999999999822 ) ;
#19409=CARTESIAN_POINT ( 'NONE',  ( 21.90174657591892071, 13.47998113580524659, -0.7349207973210680755 ) ) ;
#19410=EDGE_CURVE ( 'NONE', #64921, #33298, #58266, .T. ) ;
#19411=LINE ( 'NONE', #4788, #14013 ) ;
#19412=DIRECTION ( 'NONE',  ( -1.000000000000000000, -0.000000000000000000, 0.000000000000000000 ) ) ;
#19413=EDGE_CURVE ( 'NONE', #10611, #42570, #57512, .T. ) ;
#19414=AXIS2_PLACEMENT_3D ( 'NONE', #51565, #26269, #46544 ) ;
#19416=DIRECTION ( 'NONE',  ( 0.000000000000000000, -0.01356324068817998940, 0.9999080150203990547 ) ) ;
#19417=DIRECTION ( 'NONE',  ( 1.000000000000000000, 0.000000000000000000, -0.000000000000000000 ) ) ;
#19419=ORIENTED_EDGE ( 'NONE', *, *, #2204, .F. ) ;
#19420=CIRCLE ( 'NONE', #59912, 5.000000000000001776 ) ;
#19421=AXIS2_PLACEMENT_3D ( 'NONE', #20255, #51538, #41509 ) ;
#19422=AXIS2_PLACEMENT_3D ( 'NONE', #40084, #4871, #20144 ) ;
#19423=VECTOR ( 'NONE', #41, 1000.000000000000000 ) ;
#19424=( BOUNDED_CURVE ( )  B_SPLINE_CURVE ( 3, ( #21643, #26610, #377, #20656 ),
 .UNSPECIFIED., .F., .F. ) 
 B_SPLINE_CURVE_WITH_KNOTS ( ( 4, 4 ),
 ( 4.417647514148206334, 4.442076100497985180 ),
 .UNSPECIFIED. ) 
 CURVE ( )  GEOMETRIC_REPRESENTATION_ITEM ( )  RATIONAL_B_SPLINE_CURVE ( ( 1.000000000000000000, 0.9999502709656691302, 0.9999502709656691302, 1.000000000000000000 ) ) 
 REPRESENTATION_ITEM ( '' )  );
#19425=CARTESIAN_POINT ( 'NONE',  ( -11.22840640265205892, -5.993912459648431224, 12.09830627065808173 ) ) ;
#19426=CARTESIAN_POINT ( 'NONE',  ( 35.00000000000000000, -10.63508530065518443, 4.986700593229810963 ) ) ;
#19427=ORIENTED_EDGE ( 'NONE', *, *, #13297, .F. ) ;
#19428=DIRECTION ( 'NONE',  ( 0.000000000000000000, 0.01356324068817992175, -0.9999080150203990547 ) ) ;
#19430=DIRECTION ( 'NONE',  ( 1.000000000000000000, -0.000000000000000000, 0.000000000000000000 ) ) ;
#19432=AXIS2_PLACEMENT_3D ( 'NONE', #3987, #24251, #35198 ) ;
#19435=ADVANCED_FACE ( 'NONE', ( #13604 ), #22625, .T. ) ;
#19436=ORIENTED_EDGE ( 'NONE', *, *, #34802, .T. ) ;
#19437=DIRECTION ( 'NONE',  ( 1.000000000000000000, -0.000000000000000000, -0.000000000000000000 ) ) ;
#19438=DIRECTION ( 'NONE',  ( 0.000000000000000000, 0.01356324068817991828, -0.9999080150203990547 ) ) ;
#19439=CIRCLE ( 'NONE', #14098, 12.75000000000000178 ) ;
#19441=ORIENTED_EDGE ( 'NONE', *, *, #59646, .F. ) ;
#19442=DIRECTION ( 'NONE',  ( 0.000000000000000000, -0.01356324068817991828, 0.9999080150203990547 ) ) ;
#19443=CARTESIAN_POINT ( 'NONE',  ( -35.00000000000000000, 0.000000000000000000, 0.000000000000000000 ) ) ;
#19445=ORIENTED_EDGE ( 'NONE', *, *, #63752, .T. ) ;
#19446=ORIENTED_EDGE ( 'NONE', *, *, #5028, .T. ) ;
#19447=DIRECTION ( 'NONE',  ( 0.000000000000000000, -0.01356324068817992175, 0.9999080150203990547 ) ) ;
#19448=EDGE_CURVE ( 'NONE', #56955, #25443, #6576, .T. ) ;
#19449=VERTEX_POINT ( 'NONE', #3339 ) ;
#19452=DIRECTION ( 'NONE',  ( 0.9946347501772865307, 0.000000000000000000, -0.1034490876700550205 ) ) ;
#19456=DIRECTION ( 'NONE',  ( 0.9759340573753173542, 0.2180658516479614117, 0.000000000000000000 ) ) ;
#19457=ORIENTED_EDGE ( 'NONE', *, *, #57360, .F. ) ;
#19459=ORIENTED_EDGE ( 'NONE', *, *, #22840, .F. ) ;
#19460=VECTOR ( 'NONE', #65144, 1000.000000000000000 ) ;
#19461=DIRECTION ( 'NONE',  ( -1.000000000000000000, 0.000000000000000000, -0.000000000000000000 ) ) ;
#19462=EDGE_LOOP ( 'NONE', ( #18127, #31897, #49857, #16330 ) ) ;
#19466=VECTOR ( 'NONE', #27747, 1000.000000000000000 ) ;
#19467=FACE_OUTER_BOUND ( 'NONE', #30017, .T. ) ;
#19468=AXIS2_PLACEMENT_3D ( 'NONE', #63185, #7664, #62513 ) ;
#19469=CARTESIAN_POINT ( 'NONE',  ( 23.11735034598994076, 2.555142731765482456, 11.72821463604131687 ) ) ;
#19470=DIRECTION ( 'NONE',  ( 0.000000000000000000, 0.01356324068817998940, -0.9999080150203989437 ) ) ;
#19471=DIRECTION ( 'NONE',  ( 1.000000000000000000, 0.000000000000000000, 0.000000000000000000 ) ) ;
#19472=ORIENTED_EDGE ( 'NONE', *, *, #16654, .F. ) ;
#19473=VERTEX_POINT ( 'NONE', #12617 ) ;
#19474=CARTESIAN_POINT ( 'NONE',  ( -35.00000000000000000, 0.000000000000000000, 0.000000000000000000 ) ) ;
#19475=ORIENTED_EDGE ( 'NONE', *, *, #15919, .T. ) ;
#19476=CIRCLE ( 'NONE', #59815, 12.75000000000000178 ) ;
#19477=VERTEX_POINT ( 'NONE', #38896 ) ;
#19483=EDGE_CURVE ( 'NONE', #30093, #5329, #9733, .T. ) ;
#19485=DIRECTION ( 'NONE',  ( 0.9261641133930337277, 0.000000000000000000, -0.3771207168306929813 ) ) ;
#19487=AXIS2_PLACEMENT_3D ( 'NONE', #12072, #51363, #6127 ) ;
#19488=ORIENTED_EDGE ( 'NONE', *, *, #42171, .T. ) ;
#19489=CIRCLE ( 'NONE', #59831, 12.75000000000000178 ) ;
#19491=DIRECTION ( 'NONE',  ( -1.000000000000000000, 0.000000000000000000, 0.000000000000000000 ) ) ;
#19495=LINE ( 'NONE', #65353, #3646 ) ;
#19496=CARTESIAN_POINT ( 'NONE',  ( 4.895484889895522329, -10.53691681195900465, -8.443780401669316760 ) ) ;
#19497=LINE ( 'NONE', #4867, #24757 ) ;
#19498=DIRECTION ( 'NONE',  ( 1.000000000000000000, 0.000000000000000000, 0.000000000000000000 ) ) ;
#19499=CARTESIAN_POINT ( 'NONE',  ( -35.00000000000000000, 12.15823808070322798, 0.8294751490779768144 ) ) ;
#19501=CIRCLE ( 'NONE', #44989, 12.75000000000000178 ) ;
#19502=CARTESIAN_POINT ( 'NONE',  ( 37.00000000000000711, 0.7008968033240532414, 12.16632754454235332 ) ) ;
#19506=CARTESIAN_POINT ( 'NONE',  ( 35.00000000000000000, -9.240395740215580744, 7.251710744571670197 ) ) ;
#19507=AXIS2_PLACEMENT_3D ( 'NONE', #9335, #4051, #59259 ) ;
#19510=CARTESIAN_POINT ( 'NONE',  ( -28.25737660011475327, -10.82118954187360949, -5.196380785642891631 ) ) ;
#19512=AXIS2_PLACEMENT_3D ( 'NONE', #63321, #6842, #47408 ) ;
#19514=EDGE_CURVE ( 'NONE', #57971, #6586, #50517, .T. ) ;
#19515=CARTESIAN_POINT ( 'NONE',  ( -17.54726996257253191, 25.00000000000000000, 3.865003848717349033 ) ) ;
#19516=DIRECTION ( 'NONE',  ( 0.000000000000000000, 0.01356324068817991828, -0.9999080150203990547 ) ) ;
#19517=VECTOR ( 'NONE', #50496, 1000.000000000000000 ) ;
#19519=VERTEX_POINT ( 'NONE', #65131 ) ;
#19520=ADVANCED_FACE ( 'NONE', ( #29545 ), #4645, .T. ) ;
#19524=CARTESIAN_POINT ( 'NONE',  ( -36.00000000000000711, 4.983891302653583821, 11.73555825188278590 ) ) ;
#19526=AXIS2_PLACEMENT_3D ( 'NONE', #65619, #65314, #19779 ) ;
#19527=EDGE_CURVE ( 'NONE', #25443, #37186, #25696, .T. ) ;
#19529=ORIENTED_EDGE ( 'NONE', *, *, #56058, .F. ) ;
#19530=CARTESIAN_POINT ( 'NONE',  ( 9.687175622948609899, 13.48729812737144940, -0.5854820436212360146 ) ) ;
#19533=CARTESIAN_POINT ( 'NONE',  ( 8.937200413559443390, 4.476360154859203355, 11.13383131558893346 ) ) ;
#19537=DIRECTION ( 'NONE',  ( 0.000000000000000000, -0.01356324068817999114, 0.9999080150203989437 ) ) ;
#19540=ORIENTED_EDGE ( 'NONE', *, *, #29761, .F. ) ;
#19541=CARTESIAN_POINT ( 'NONE',  ( -37.00000000000000711, -6.657191900728257394, -9.677500615117970995 ) ) ;
#19542=ORIENTED_EDGE ( 'NONE', *, *, #13089, .F. ) ;
#19544=CARTESIAN_POINT ( 'NONE',  ( 3.386626873725977038, -10.78029969106401253, -8.130803614474327645 ) ) ;
#19545=CIRCLE ( 'NONE', #10000, 5.000000000000000000 ) ;
#19549=FACE_OUTER_BOUND ( 'NONE', #27304, .T. ) ;
#19550=CARTESIAN_POINT ( 'NONE',  ( 12.51045778728196289, 9.694119109124677891, -7.082454569427619973 ) ) ;
#19551=CARTESIAN_POINT ( 'NONE',  ( 24.54836029594799385, 1.223829190784184728, 13.44931652200175343 ) ) ;
#19552=ORIENTED_EDGE ( 'NONE', *, *, #22756, .T. ) ;
#19553=ORIENTED_EDGE ( 'NONE', *, *, #33129, .T. ) ;
#19555=AXIS2_PLACEMENT_3D ( 'NONE', #14501, #39131, #55083 ) ;
#19556=VECTOR ( 'NONE', #43834, 1000.000000000000000 ) ;
#19557=ORIENTED_EDGE ( 'NONE', *, *, #23954, .T. ) ;
#19558=CARTESIAN_POINT ( 'NONE',  ( 4.622486058658314079, -10.10462791929411530, -6.474617390905248904 ) ) ;
#19559=ORIENTED_EDGE ( 'NONE', *, *, #22938, .T. ) ;
#19560=CARTESIAN_POINT ( 'NONE',  ( -35.00000000000000000, 0.000000000000000000, 0.000000000000000000 ) ) ;
#19564=LINE ( 'NONE', #14854, #31656 ) ;
#19565=DIRECTION ( 'NONE',  ( 0.000000000000000000, 0.3807014730195152907, -0.9246979985058750851 ) ) ;
#19566=VERTEX_POINT ( 'NONE', #59836 ) ;
#19568=CARTESIAN_POINT ( 'NONE',  ( -16.89440222264807190, 7.451370833537603211, 9.406604778602895678 ) ) ;
#19569=CARTESIAN_POINT ( 'NONE',  ( 37.00000000000000711, 4.705694406421931860E-17, -3.469127814946512892E-15 ) ) ;
#19570=CARTESIAN_POINT ( 'NONE',  ( 12.16520966156148909, 13.20908209050864457, -2.809526505251493500 ) ) ;
#19571=AXIS2_PLACEMENT_3D ( 'NONE', #41057, #52376, #62012 ) ;
#19573=LINE ( 'NONE', #49823, #51058 ) ;
#19574=CARTESIAN_POINT ( 'NONE',  ( -36.00000000000000711, 1.286231064351496922, -12.68495603654570481 ) ) ;
#19575=DIRECTION ( 'NONE',  ( -1.000000000000000000, 0.000000000000000000, 0.000000000000000000 ) ) ;
#19576=VECTOR ( 'NONE', #26438, 1000.000000000000000 ) ;
#19577=EDGE_CURVE ( 'NONE', #2026, #6959, #45845, .T. ) ;
#19580=ORIENTED_EDGE ( 'NONE', *, *, #50486, .F. ) ;
#19583=VECTOR ( 'NONE', #1383, 1000.000000000000000 ) ;
#19585=DIRECTION ( 'NONE',  ( -1.000000000000000000, 0.000000000000000000, 0.000000000000000000 ) ) ;
#19588=ORIENTED_EDGE ( 'NONE', *, *, #50914, .T. ) ;
#19589=CARTESIAN_POINT ( 'NONE',  ( -11.39029853170218587, -7.950373430328300906, -10.91384404852269796 ) ) ;
#19591=CIRCLE ( 'NONE', #59039, 5.000000000000000888 ) ;
#19592=CARTESIAN_POINT ( 'NONE',  ( 11.55880380088042969, 0.7131711660007539200, 11.97899817320787363 ) ) ;
#19595=ADVANCED_FACE ( 'NONE', ( #54842 ), #55491, .T. ) ;
#19596=DIRECTION ( 'NONE',  ( -1.000000000000000000, 0.000000000000000000, -0.000000000000000000 ) ) ;
#19597=VERTEX_POINT ( 'NONE', #9939 ) ;
#19598=EDGE_CURVE ( 'NONE', #8078, #7570, #5534, .T. ) ;
#19599=CARTESIAN_POINT ( 'NONE',  ( 37.00000000000000711, 9.060822531526046220, -7.474872387601039669 ) ) ;
#19600=EDGE_LOOP ( 'NONE', ( #13090, #26198, #25494, #35224 ) ) ;
#19601=EDGE_CURVE ( 'NONE', #52455, #15087, #4299, .T. ) ;
#19602=CARTESIAN_POINT ( 'NONE',  ( -37.00000000000000711, 10.25474254703953036, 6.584150480049589582 ) ) ;
#19603=CARTESIAN_POINT ( 'NONE',  ( 37.00000000000000711, -1.456211999474423369, -11.65554240571057143 ) ) ;
#19604=AXIS2_PLACEMENT_3D ( 'NONE', #12795, #16808, #32735 ) ;
#19607=VERTEX_POINT ( 'NONE', #44853 ) ;
#19608=EDGE_CURVE ( 'NONE', #429, #65629, #20376, .T. ) ;
#19609=ORIENTED_EDGE ( 'NONE', *, *, #52981, .F. ) ;
#19611=ORIENTED_EDGE ( 'NONE', *, *, #47390, .T. ) ;
#19613=DIRECTION ( 'NONE',  ( 0.000000000000000000, 0.000000000000000000, -1.000000000000000000 ) ) ;
#19614=DIRECTION ( 'NONE',  ( 0.000000000000000000, 0.2006870767258889243, -0.9796553971857742127 ) ) ;
#19615=DIRECTION ( 'NONE',  ( 1.000000000000000000, 0.000000000000000000, 0.000000000000000000 ) ) ;
#19618=CARTESIAN_POINT ( 'NONE',  ( -35.00000000000000000, -11.81949347079749124, 2.968224442958359965 ) ) ;
#19620=ORIENTED_EDGE ( 'NONE', *, *, #29275, .T. ) ;
#19622=ORIENTED_EDGE ( 'NONE', *, *, #40871, .T. ) ;
#19623=ORIENTED_EDGE ( 'NONE', *, *, #5347, .T. ) ;
#19624=CARTESIAN_POINT ( 'NONE',  ( 0.2851083653049504285, -0.4107471485392698018, 13.49374991542258151 ) ) ;
#19625=ADVANCED_FACE ( 'NONE', ( #11564 ), #6272, .T. ) ;
#19626=AXIS2_PLACEMENT_3D ( 'NONE', #58726, #49409, #13147 ) ;
#19627=DIRECTION ( 'NONE',  ( 0.000000000000000000, -1.000000000000000000, 0.000000000000000000 ) ) ;
#19628=ORIENTED_EDGE ( 'NONE', *, *, #8242, .T. ) ;
#19630=DIRECTION ( 'NONE',  ( -1.000000000000000000, -1.836970198721029688E-16, -0.000000000000000000 ) ) ;
#19634=FACE_OUTER_BOUND ( 'NONE', #36856, .T. ) ;
#19638=EDGE_CURVE ( 'NONE', #39558, #52452, #11865, .T. ) ;
#19639=CARTESIAN_POINT ( 'NONE',  ( -37.00000000000000711, 0.3137578094509230753, 12.74613886779085270 ) ) ;
#19641=ORIENTED_EDGE ( 'NONE', *, *, #24463, .F. ) ;
#19643=VERTEX_POINT ( 'NONE', #26531 ) ;
#19644=VERTEX_POINT ( 'NONE', #1286 ) ;
#19645=CYLINDRICAL_SURFACE ( 'NONE', #44668, 12.74999999999999822 ) ;
#19646=LINE ( 'NONE', #60186, #13493 ) ;
#19647=AXIS2_PLACEMENT_3D ( 'NONE', #25956, #26590, #5686 ) ;
#19648=DIRECTION ( 'NONE',  ( 1.000000000000000000, -0.000000000000000000, 0.000000000000000000 ) ) ;
#19650=ORIENTED_EDGE ( 'NONE', *, *, #43987, .T. ) ;
#19651=CARTESIAN_POINT ( 'NONE',  ( -35.00000000000000000, -11.72195762423409349, -0.7536123767499773862 ) ) ;
#19652=ORIENTED_EDGE ( 'NONE', *, *, #8284, .T. ) ;
#19653=DIRECTION ( 'NONE',  ( 0.000000000000000000, -0.9246979985058680906, -0.3807014730195321661 ) ) ;
#19655=AXIS2_PLACEMENT_3D ( 'NONE', #44956, #50295, #62139 ) ;
#19656=ORIENTED_EDGE ( 'NONE', *, *, #44428, .T. ) ;
#19663=ORIENTED_EDGE ( 'NONE', *, *, #63538, .F. ) ;
#19665=AXIS2_PLACEMENT_3D ( 'NONE', #50588, #28722, #4377 ) ;
#19666=ORIENTED_EDGE ( 'NONE', *, *, #9196, .T. ) ;
#19667=DIRECTION ( 'NONE',  ( 0.5417962735734935809, -0.000000000000000000, 0.8405098440481683086 ) ) ;
#19672=ORIENTED_EDGE ( 'NONE', *, *, #31727, .T. ) ;
#19674=DIRECTION ( 'NONE',  ( 0.000000000000000000, -0.2960891610144577024, -0.9551603052523457427 ) ) ;
#19676=CARTESIAN_POINT ( 'NONE',  ( 35.00000000000000000, 10.01317267707886671, -6.946017217729977489 ) ) ;
#19677=FACE_OUTER_BOUND ( 'NONE', #17672, .T. ) ;
#19680=ADVANCED_FACE ( 'NONE', ( #40857 ), #31837, .T. ) ;
#19682=DIRECTION ( 'NONE',  ( 0.000000000000000000, -0.01356324068817991828, 0.9999080150203990547 ) ) ;
#19684=CARTESIAN_POINT ( 'NONE',  ( -37.00000000000000711, -11.47758908105692655, -2.497432891016966749 ) ) ;
#19687=AXIS2_PLACEMENT_3D ( 'NONE', #56959, #62559, #32312 ) ;
#19688=ORIENTED_EDGE ( 'NONE', *, *, #17708, .T. ) ;
#19689=CARTESIAN_POINT ( 'NONE',  ( -29.92777678363736626, -3.750539801530011985, 11.39883551934754635 ) ) ;
#19690=ORIENTED_EDGE ( 'NONE', *, *, #63979, .F. ) ;
#19691=CARTESIAN_POINT ( 'NONE',  ( -14.17299601508879192, 8.097942500480229455, -8.858180248946757374 ) ) ;
#19692=DIRECTION ( 'NONE',  ( -0.9915282196991074271, 0.000000000000000000, 0.1298914529148032515 ) ) ;
#19693=CYLINDRICAL_SURFACE ( 'NONE', #57634, 12.18649999999999878 ) ;
#19694=EDGE_CURVE ( 'NONE', #55015, #24413, #51197, .T. ) ;
#19695=DIRECTION ( 'NONE',  ( -1.000000000000000000, 0.000000000000000000, 0.000000000000000000 ) ) ;
#19697=EDGE_CURVE ( 'NONE', #38454, #37450, #51174, .T. ) ;
#19699=VERTEX_POINT ( 'NONE', #51821 ) ;
#19702=CYLINDRICAL_SURFACE ( 'NONE', #17226, 5.000000000000000888 ) ;
#19704=EDGE_CURVE ( 'NONE', #11383, #41793, #3412, .T. ) ;
#19705=DIRECTION ( 'NONE',  ( 1.000000000000000000, -0.000000000000000000, 0.000000000000000000 ) ) ;
#19709=ORIENTED_EDGE ( 'NONE', *, *, #1855, .F. ) ;
#19710=VECTOR ( 'NONE', #40926, 1000.000000000000000 ) ;
#19711=DIRECTION ( 'NONE',  ( -0.9915282196991074271, 0.000000000000000000, 0.1298914529148032515 ) ) ;
#19713=DIRECTION ( 'NONE',  ( 0.000000000000000000, -0.5472293298355331848, 0.8369827122275305120 ) ) ;
#19714=CARTESIAN_POINT ( 'NONE',  ( 36.00000000000000711, -10.39746860227895731, -7.379373053628834889 ) ) ;
#19715=ORIENTED_EDGE ( 'NONE', *, *, #61217, .T. ) ;
#19716=EDGE_CURVE ( 'NONE', #16620, #30257, #63894, .T. ) ;
#19721=LINE ( 'NONE', #64908, #31632 ) ;
#19724=CARTESIAN_POINT ( 'NONE',  ( 37.00000000000000711, -11.61976888909157246, -3.827969819614423841 ) ) ;
#19725=DIRECTION ( 'NONE',  ( 0.000000000000000000, 0.01356324068817992175, -0.9999080150203990547 ) ) ;
#19726=DIRECTION ( 'NONE',  ( 1.000000000000000000, 0.000000000000000000, 0.000000000000000000 ) ) ;
#19727=CARTESIAN_POINT ( 'NONE',  ( 37.00000000000000711, -2.497432891016756251, 11.47758908105696740 ) ) ;
#19728=LINE ( 'NONE', #49653, #59839 ) ;
#19730=ORIENTED_EDGE ( 'NONE', *, *, #49533, .T. ) ;
#19733=ORIENTED_EDGE ( 'NONE', *, *, #41457, .F. ) ;
#19736=DIRECTION ( 'NONE',  ( 1.000000000000000000, 0.000000000000000000, 0.000000000000000000 ) ) ;
#19737=CARTESIAN_POINT ( 'NONE',  ( -35.00000000000000000, 3.033604067594749765, -12.38385022362078658 ) ) ;
#19739=DIRECTION ( 'NONE',  ( -1.000000000000000000, 0.000000000000000000, 0.000000000000000000 ) ) ;
#19740=VECTOR ( 'NONE', #56114, 1000.000000000000000 ) ;
#19741=ADVANCED_FACE ( 'NONE', ( #943 ), #21211, .T. ) ;
#19742=CARTESIAN_POINT ( 'NONE',  ( -37.00000000000000711, 7.110831038798280268, 9.896810808925419423 ) ) ;
#19743=ADVANCED_FACE ( 'NONE', ( #1927 ), #23523, .F. ) ;
#19748=EDGE_LOOP ( 'NONE', ( #23957, #60619, #48598, #56741 ) ) ;
#19749=EDGE_CURVE ( 'NONE', #21040, #49572, #54102, .T. ) ;
#19750=VECTOR ( 'NONE', #18982, 1000.000000000000000 ) ;
#19751=AXIS2_PLACEMENT_3D ( 'NONE', #38797, #54434, #8522 ) ;
#19752=FACE_OUTER_BOUND ( 'NONE', #50896, .T. ) ;
#19753=CARTESIAN_POINT ( 'NONE',  ( -35.00000000000000000, 11.65150730582932503, 1.488153103997165605 ) ) ;
#19755=EDGE_CURVE ( 'NONE', #48169, #23887, #19344, .T. ) ;
#19756=ORIENTED_EDGE ( 'NONE', *, *, #30522, .T. ) ;
#19758=CARTESIAN_POINT ( 'NONE',  ( -47.00000000000000711, 0.000000000000000000, 0.000000000000000000 ) ) ;
#19759=DIRECTION ( 'NONE',  ( 1.000000000000000000, 0.000000000000000000, -0.000000000000000000 ) ) ;
#19761=VECTOR ( 'NONE', #51301, 1000.000000000000000 ) ;
#19765=CARTESIAN_POINT ( 'NONE',  ( -35.00000000000000000, -12.18359334611896472, -0.2661492558804631203 ) ) ;
#19767=FACE_OUTER_BOUND ( 'NONE', #2009, .T. ) ;
#19768=ORIENTED_EDGE ( 'NONE', *, *, #31297, .T. ) ;
#19769=CARTESIAN_POINT ( 'NONE',  ( 10.63145532060650744, 0.6018409079247246662, 13.48718478653089647 ) ) ;
#19771=VERTEX_POINT ( 'NONE', #47806 ) ;
#19772=ORIENTED_EDGE ( 'NONE', *, *, #47287, .T. ) ;
#19773=ORIENTED_EDGE ( 'NONE', *, *, #39993, .F. ) ;
#19779=DIRECTION ( 'NONE',  ( 0.000000000000000000, -0.5472293298355331848, 0.8369827122275305120 ) ) ;
#19780=CARTESIAN_POINT ( 'NONE',  ( -35.00000000000000000, 3.473736367725253515, 12.26766708251992810 ) ) ;
#19781=B_SPLINE_CURVE_WITH_KNOTS ( 'NONE', 3,
 ( #9355, #54925, #43063, #2538, #33088, #27776, #4068, #19369, #58725, #63341, #29642, #48080, #13144, #17807 ),
 .UNSPECIFIED., .F., .F.,
 ( 4, 2, 2, 2, 2, 2, 4 ),
 ( 1.301042606982605321E-18, 0.001757691579725207103, 0.002636537369587810004, 0.003515383159450412905, 0.004394228949313015373, 0.005273074739175619141, 0.007030766318900821474 ),
 .UNSPECIFIED. ) ;
#19783=CARTESIAN_POINT ( 'NONE',  ( 23.20048651429565112, 3.175973680696976498, -13.12354496719417085 ) ) ;
#19785=ORIENTED_EDGE ( 'NONE', *, *, #43211, .T. ) ;
#19786=EDGE_CURVE ( 'NONE', #7570, #2448, #17557, .T. ) ;
#19787=CARTESIAN_POINT ( 'NONE',  ( 145.1370849898475797, 3.309064568108273190E-14, 0.000000000000000000 ) ) ;
#19790=EDGE_LOOP ( 'NONE', ( #34276, #63291, #41337, #55312 ) ) ;
#19796=CIRCLE ( 'NONE', #20869, 5.000000000000000888 ) ;
#19797=CARTESIAN_POINT ( 'NONE',  ( 37.00000000000000711, 11.81949347079746637, -2.968224442958448783 ) ) ;
#19798=CYLINDRICAL_SURFACE ( 'NONE', #21420, 4.999999999999999112 ) ;
#19802=VERTEX_POINT ( 'NONE', #12223 ) ;
#19803=ORIENTED_EDGE ( 'NONE', *, *, #50264, .F. ) ;
#19804=CARTESIAN_POINT ( 'NONE',  ( 3.347841273039249721, -10.61118957148187825, 8.345816669330455184 ) ) ;
#19806=CARTESIAN_POINT ( 'NONE',  ( 17.93387043762216493, -6.318682511722990114, 10.20511618420410116 ) ) ;
#19808=CARTESIAN_POINT ( 'NONE',  ( -11.24065750081571835, -6.047149079109201075, -10.36726786815886214 ) ) ;
#19809=DIRECTION ( 'NONE',  ( -1.000000000000000000, 0.000000000000000000, 0.000000000000000000 ) ) ;
#19811=VERTEX_POINT ( 'NONE', #2925 ) ;
#19812=( BOUNDED_CURVE ( )  B_SPLINE_CURVE ( 3, ( #25171, #29822, #65395, #55101 ),
 .UNSPECIFIED., .F., .F. ) 
 B_SPLINE_CURVE_WITH_KNOTS ( ( 4, 4 ),
 ( 1.140504141920692494, 1.180309962260583934 ),
 .UNSPECIFIED. ) 
 CURVE ( )  GEOMETRIC_REPRESENTATION_ITEM ( )  RATIONAL_B_SPLINE_CURVE ( ( 1.000000000000000000, 0.9998679624143003153, 0.9998679624143003153, 1.000000000000000000 ) ) 
 REPRESENTATION_ITEM ( '' )  );
#19813=VERTEX_POINT ( 'NONE', #58447 ) ;
#19814=DIRECTION ( 'NONE',  ( -1.000000000000000000, -0.000000000000000000, 0.000000000000000000 ) ) ;
#19815=DIRECTION ( 'NONE',  ( 1.000000000000000000, 0.000000000000000000, 0.000000000000000000 ) ) ;
#19816=DIRECTION ( 'NONE',  ( 0.000000000000000000, 0.3807014730195151797, -0.9246979985058750851 ) ) ;
#19817=CARTESIAN_POINT ( 'NONE',  ( 3.347841273039249721, -10.61118957148187825, 5.603807266321171987 ) ) ;
#19818=CARTESIAN_POINT ( 'NONE',  ( 6.681371532684399206, -8.678434492379226484, -10.34286318303527352 ) ) ;
#19819=CYLINDRICAL_SURFACE ( 'NONE', #60885, 4.999999999999999112 ) ;
#19821=ADVANCED_FACE ( 'NONE', ( #53467 ), #7912, .T. ) ;
#19826=AXIS2_PLACEMENT_3D ( 'NONE', #35641, #31630, #40967 ) ;
#19827=EDGE_CURVE ( 'NONE', #51664, #40551, #21424, .T. ) ;
#19828=CIRCLE ( 'NONE', #52820, 12.18650000000000233 ) ;
#19831=ORIENTED_EDGE ( 'NONE', *, *, #64422, .F. ) ;
#19833=CARTESIAN_POINT ( 'NONE',  ( -37.00000000000000711, 9.040300684349693583, 7.499679039484089316 ) ) ;
#19836=DIRECTION ( 'NONE',  ( 0.000000000000000000, 0.01356324068817998940, -0.9999080150203990547 ) ) ;
#19837=FACE_OUTER_BOUND ( 'NONE', #17168, .T. ) ;
#19839=CARTESIAN_POINT ( 'NONE',  ( -35.00000000000000000, 0.000000000000000000, 0.000000000000000000 ) ) ;
#19840=CARTESIAN_POINT ( 'NONE',  ( -16.98800322446194855, 2.922502605998049674, 11.63868456991315625 ) ) ;
#19841=ADVANCED_FACE ( 'NONE', ( #43798 ), #64078, .T. ) ;
#19842=DIRECTION ( 'NONE',  ( 1.000000000000000000, -0.000000000000000000, 0.000000000000000000 ) ) ;
#19844=LINE ( 'NONE', #15814, #64113 ) ;
#19846=CARTESIAN_POINT ( 'NONE',  ( -17.05724255175752901, 7.953322362475236496, -10.91012176226558417 ) ) ;
#19847=CYLINDRICAL_SURFACE ( 'NONE', #22383, 4.999999999999999112 ) ;
#19848=CARTESIAN_POINT ( 'NONE',  ( -37.00000000000000711, -11.35427606708809556, 4.426194442447198618 ) ) ;
#19849=CARTESIAN_POINT ( 'NONE',  ( 35.00000000000000000, -6.102719229070595830, 10.54834585426226390 ) ) ;
#19850=DIRECTION ( 'NONE',  ( -1.000000000000000000, -0.000000000000000000, 0.000000000000000000 ) ) ;
#19851=VERTEX_POINT ( 'NONE', #55075 ) ;
#19852=ORIENTED_EDGE ( 'NONE', *, *, #30815, .T. ) ;
#19854=EDGE_LOOP ( 'NONE', ( #54121, #32338, #7879, #11289 ) ) ;
#19856=EDGE_CURVE ( 'NONE', #11898, #10126, #11913, .T. ) ;
#19857=CYLINDRICAL_SURFACE ( 'NONE', #11985, 12.18650000000000055 ) ;
#19858=DIRECTION ( 'NONE',  ( 1.000000000000000000, 0.000000000000000000, 0.000000000000000000 ) ) ;
#19859=ORIENTED_EDGE ( 'NONE', *, *, #56044, .T. ) ;
#19860=DIRECTION ( 'NONE',  ( 0.000000000000000000, 0.000000000000000000, -1.000000000000000000 ) ) ;
#19863=CARTESIAN_POINT ( 'NONE',  ( 35.00000000000000000, -5.391785509271032062, -10.43555801961473861 ) ) ;
#19864=ORIENTED_EDGE ( 'NONE', *, *, #58022, .F. ) ;
#19867=ORIENTED_EDGE ( 'NONE', *, *, #53993, .T. ) ;
#19869=CIRCLE ( 'NONE', #18833, 5.000000000000000000 ) ;
#19876=VECTOR ( 'NONE', #25489, 1000.000000000000000 ) ;
#19877=CARTESIAN_POINT ( 'NONE',  ( -14.29135464769095520, 7.782112657557433089, -11.03126115115966854 ) ) ;
#19878=EDGE_CURVE ( 'NONE', #41187, #20717, #56557, .T. ) ;
#19879=ORIENTED_EDGE ( 'NONE', *, *, #50684, .T. ) ;
#19881=EDGE_CURVE ( 'NONE', #41694, #31670, #29170, .T. ) ;
#19882=CARTESIAN_POINT ( 'NONE',  ( 22.22678687964571864, 10.97453491530256464, -4.866768194205650211 ) ) ;
#19883=CARTESIAN_POINT ( 'NONE',  ( -27.19357181888462094, 12.48377454417557253, 5.138615876886901468 ) ) ;
#19884=CARTESIAN_POINT ( 'NONE',  ( 35.00000000000000000, 11.56998259273182583, 3.827046518384956020 ) ) ;
#19886=DIRECTION ( 'NONE',  ( 0.000000000000000000, -0.9903235168508564001, -0.1387779952735713473 ) ) ;
#19887=FACE_OUTER_BOUND ( 'NONE', #26706, .T. ) ;
#19889=EDGE_LOOP ( 'NONE', ( #30404, #45676, #58155, #24036 ) ) ;
#19892=VERTEX_POINT ( 'NONE', #29467 ) ;
#19893=DIRECTION ( 'NONE',  ( 1.000000000000000000, -0.000000000000000000, 0.000000000000000000 ) ) ;
#19895=CARTESIAN_POINT ( 'NONE',  ( 37.00000000000000711, -2.080187960898473687, 12.57916205664483122 ) ) ;
#19897=DIRECTION ( 'NONE',  ( 0.000000000000000000, 0.01356324068817998940, -0.9999080150203989437 ) ) ;
#19898=ADVANCED_FACE ( 'NONE', ( #19837 ), #35447, .T. ) ;
#19900=DIRECTION ( 'NONE',  ( -1.000000000000000000, -0.000000000000000000, 0.000000000000000000 ) ) ;
#19902=CARTESIAN_POINT ( 'NONE',  ( 8.957194808219908211, 4.011391350595442162, 11.31236870852682941 ) ) ;
#19903=FACE_OUTER_BOUND ( 'NONE', #62739, .T. ) ;
#19904=CIRCLE ( 'NONE', #39027, 12.74999999999999822 ) ;
#19905=CARTESIAN_POINT ( 'NONE',  ( 9.584295231686237315, 6.682444889156122336, -11.73468901934476705 ) ) ;
#19906=CYLINDRICAL_SURFACE ( 'NONE', #53165, 12.75000000000000178 ) ;
#19907=ORIENTED_EDGE ( 'NONE', *, *, #42072, .T. ) ;
#19909=VERTEX_POINT ( 'NONE', #60727 ) ;
#19910=CYLINDRICAL_SURFACE ( 'NONE', #60946, 12.18650000000000055 ) ;
#19912=CIRCLE ( 'NONE', #48607, 5.000000000000001776 ) ;
#19915=ORIENTED_EDGE ( 'NONE', *, *, #12462, .F. ) ;
#19916=AXIS2_PLACEMENT_3D ( 'NONE', #46125, #575, #41101 ) ;
#19917=ORIENTED_EDGE ( 'NONE', *, *, #64696, .T. ) ;
#19920=LINE ( 'NONE', #39874, #48904 ) ;
#19921=DIRECTION ( 'NONE',  ( 0.000000000000000000, 0.6943713148249640588, -0.7196168960969792083 ) ) ;
#19922=DIRECTION ( 'NONE',  ( 0.000000000000000000, 0.2006870767258819854, -0.9796553971857756560 ) ) ;
#19923=CARTESIAN_POINT ( 'NONE',  ( -36.00000000000000711, 6.711949091238296639, -10.84030624090599559 ) ) ;
#19924=FACE_OUTER_BOUND ( 'NONE', #18641, .T. ) ;
#19929=ORIENTED_EDGE ( 'NONE', *, *, #46056, .T. ) ;
#19932=ADVANCED_FACE ( 'NONE', ( #3597 ), #49466, .T. ) ;
#19934=VERTEX_POINT ( 'NONE', #4215 ) ;
#19935=DIRECTION ( 'NONE',  ( 0.000000000000000000, 0.01356324068817998940, -0.9999080150203990547 ) ) ;
#19936=ORIENTED_EDGE ( 'NONE', *, *, #28185, .T. ) ;
#19937=CARTESIAN_POINT ( 'NONE',  ( 35.00000000000000000, -11.73808581813437613, 0.4353888892049613824 ) ) ;
#19938=CARTESIAN_POINT ( 'NONE',  ( 5.635198476044180893, -9.293512099126084891, -9.797319838910391709 ) ) ;
#19939=CYLINDRICAL_SURFACE ( 'NONE', #16968, 4.999999999999999112 ) ;
#19940=CARTESIAN_POINT ( 'NONE',  ( 4.681985117566611621, -10.64506698050158207, 5.541855235442475269 ) ) ;
#19941=ORIENTED_EDGE ( 'NONE', *, *, #4956, .T. ) ;
#19943=CARTESIAN_POINT ( 'NONE',  ( -35.00000000000000000, -3.213188559034318992, 11.29812557209475798 ) ) ;
#19944=VERTEX_POINT ( 'NONE', #45111 ) ;
#19945=DIRECTION ( 'NONE',  ( -1.000000000000000000, 0.000000000000000000, -0.000000000000000000 ) ) ;
#19946=EDGE_LOOP ( 'NONE', ( #41348, #44396, #37010, #44446 ) ) ;
#19947=ORIENTED_EDGE ( 'NONE', *, *, #31725, .F. ) ;
#19948=ORIENTED_EDGE ( 'NONE', *, *, #18987, .F. ) ;
#19952=ADVANCED_FACE ( 'NONE', ( #29789 ), #39124, .T. ) ;
#19955=DIRECTION ( 'NONE',  ( 0.000000000000000000, -0.01356324068818000328, 0.9999080150203990547 ) ) ;
#19956=ORIENTED_EDGE ( 'NONE', *, *, #1728, .T. ) ;
#19958=AXIS2_PLACEMENT_3D ( 'NONE', #32627, #58261, #17373 ) ;
#19960=LINE ( 'NONE', #60194, #48695 ) ;
#19962=CARTESIAN_POINT ( 'NONE',  ( -18.54676851533650961, -5.050683831495517140, -12.52189472075509613 ) ) ;
#19963=ADVANCED_FACE ( 'NONE', ( #44426 ), #60389, .T. ) ;
#19964=ORIENTED_EDGE ( 'NONE', *, *, #27319, .T. ) ;
#19968=AXIS2_PLACEMENT_3D ( 'NONE', #14703, #9731, #30021 ) ;
#19969=ORIENTED_EDGE ( 'NONE', *, *, #37619, .T. ) ;
#19970=EDGE_CURVE ( 'NONE', #12635, #42754, #40601, .T. ) ;
#19972=ORIENTED_EDGE ( 'NONE', *, *, #25103, .F. ) ;
#19974=CARTESIAN_POINT ( 'NONE',  ( -24.53364844038847892, -11.34588198318266095, 7.318208206151304296 ) ) ;
#19978=CARTESIAN_POINT ( 'NONE',  ( 11.15383795322125771, 11.94197166349967532, -1.183955411781195011 ) ) ;
#19983=DIRECTION ( 'NONE',  ( 0.000000000000000000, 0.4134677391718449835, 0.9105187689795983808 ) ) ;
#19984=EDGE_CURVE ( 'NONE', #20076, #16407, #28710, .T. ) ;
#19988=DIRECTION ( 'NONE',  ( -1.000000000000000000, 0.000000000000000000, 0.000000000000000000 ) ) ;
#19990=DIRECTION ( 'NONE',  ( 1.000000000000000000, 0.000000000000000000, 0.000000000000000000 ) ) ;
#19991=CARTESIAN_POINT ( 'NONE',  ( 35.00000000000000000, 0.7214809346830272085, 11.72397916322010936 ) ) ;
#19993=VERTEX_POINT ( 'NONE', #58281 ) ;
#19995=CIRCLE ( 'NONE', #23180, 12.18650000000000233 ) ;
#19996=ORIENTED_EDGE ( 'NONE', *, *, #46988, .F. ) ;
#19997=CARTESIAN_POINT ( 'NONE',  ( 35.00000000000000000, -3.645068577059948911, 11.16627499335658413 ) ) ;
#19999=DIRECTION ( 'NONE',  ( 0.000000000000000000, 0.1118654143051615590, 0.9937233664769760111 ) ) ;
#20001=AXIS2_PLACEMENT_3D ( 'NONE', #39912, #40229, #10304 ) ;
#20003=VERTEX_POINT ( 'NONE', #51432 ) ;
#20004=ORIENTED_EDGE ( 'NONE', *, *, #13906, .F. ) ;
#20005=AXIS2_PLACEMENT_3D ( 'NONE', #5596, #14861, #35149 ) ;
#20007=CARTESIAN_POINT ( 'NONE',  ( 29.60305162835625126, -8.975199590264201888, 7.980219161752089008 ) ) ;
#20010=ORIENTED_EDGE ( 'NONE', *, *, #3512, .F. ) ;
#20011=CARTESIAN_POINT ( 'NONE',  ( 37.00000000000000711, -11.01837265713068703, 6.415447294506815723 ) ) ;
#20012=DIRECTION ( 'NONE',  ( -1.000000000000000000, 0.000000000000000000, 0.000000000000000000 ) ) ;
#20014=ORIENTED_EDGE ( 'NONE', *, *, #58452, .F. ) ;
#20016=ADVANCED_FACE ( 'NONE', ( #46736 ), #5545, .T. ) ;
#20018=CARTESIAN_POINT ( 'NONE',  ( -4.806344283790351390, -7.508992741355383416, 25.00000000000000000 ) ) ;
#20020=ORIENTED_EDGE ( 'NONE', *, *, #7883, .T. ) ;
#20021=LINE ( 'NONE', #9369, #43726 ) ;
#20022=ORIENTED_EDGE ( 'NONE', *, *, #26584, .T. ) ;
#20024=EDGE_CURVE ( 'NONE', #63348, #50423, #62895, .T. ) ;
#20026=B_SPLINE_CURVE_WITH_KNOTS ( 'NONE', 3,
 ( #60367, #4196, #50083, #19156, #39428, #4542, #9169, #49448, #13500, #49749, #24808, #33782, #24462, #19818, #53767, #44742, #65024, #64053, #40079, #28472, #19496, #54084, #39766, #8517 ),
 .UNSPECIFIED., .F., .F.,
 ( 4, 2, 2, 2, 2, 2, 2, 2, 2, 2, 2, 4 ),
 ( 0.000000000000000000, 0.001281805353653630913, 0.001922708030480444093, 0.002563610707307257489, 0.003204513384134070452, 0.003845416060960883849, 0.005127221414614510642, 0.005768124091441322737, 0.006409026768268135700, 0.007690832121921758156, 0.008972637475575379745, 0.01025444282922900220 ),
 .UNSPECIFIED. ) ;
#20028=CARTESIAN_POINT ( 'NONE',  ( 12.36261888780203222, -8.715147324829775499, -8.257870389522178556 ) ) ;
#20029=CARTESIAN_POINT ( 'NONE',  ( -37.00000000000000711, -11.53507381115581687, -2.216820770815207897 ) ) ;
#20032=CIRCLE ( 'NONE', #41279, 5.000000000000000000 ) ;
#20033=DIRECTION ( 'NONE',  ( 0.000000000000000000, -0.9246979985058764173, -0.3807014730195119045 ) ) ;
#20034=EDGE_CURVE ( 'NONE', #53922, #31267, #59725, .T. ) ;
#20035=DIRECTION ( 'NONE',  ( 1.000000000000000000, 0.000000000000000000, 0.000000000000000000 ) ) ;
#20037=CARTESIAN_POINT ( 'NONE',  ( -35.00000000000000000, 0.8294751490781091530, -12.15823808070321732 ) ) ;
#20038=CARTESIAN_POINT ( 'NONE',  ( -18.36801285212142432, 3.941043466613568746, -12.91410746298855372 ) ) ;
#20040=CYLINDRICAL_SURFACE ( 'NONE', #26886, 5.000000000000000888 ) ;
#20041=ORIENTED_EDGE ( 'NONE', *, *, #20881, .T. ) ;
#20042=AXIS2_PLACEMENT_3D ( 'NONE', #4848, #25117, #31082 ) ;
#20043=CARTESIAN_POINT ( 'NONE',  ( -2.952869152607106251, 25.00000000000000000, 3.755417052241485365 ) ) ;
#20044=ORIENTED_EDGE ( 'NONE', *, *, #20628, .T. ) ;
#20047=LINE ( 'NONE', #45636, #31783 ) ;
#20048=CARTESIAN_POINT ( 'NONE',  ( 36.00000000000000711, -12.71517666308947092, 0.9416912585475705200 ) ) ;
#20050=DIRECTION ( 'NONE',  ( -1.000000000000000000, 0.000000000000000000, 0.000000000000000000 ) ) ;
#20052=DIRECTION ( 'NONE',  ( -0.000000000000000000, -1.000000000000000000, -0.000000000000000000 ) ) ;
#20053=CIRCLE ( 'NONE', #30667, 12.18650000000000055 ) ;
#20055=ORIENTED_EDGE ( 'NONE', *, *, #29547, .F. ) ;
#20058=DIRECTION ( 'NONE',  ( 0.000000000000000000, 0.01356324068817992175, -0.9999080150203990547 ) ) ;
#20059=FACE_OUTER_BOUND ( 'NONE', #33796, .T. ) ;
#20061=VERTEX_POINT ( 'NONE', #21477 ) ;
#20063=EDGE_CURVE ( 'NONE', #8847, #31243, #20816, .T. ) ;
#20064=ADVANCED_FACE ( 'NONE', ( #41083 ), #41748, .T. ) ;
#20065=ADVANCED_FACE ( 'NONE', ( #26787 ), #23352, .T. ) ;
#20067=ADVANCED_FACE ( 'NONE', ( #29322 ), #58627, .T. ) ;
#20070=VERTEX_POINT ( 'NONE', #28341 ) ;
#20071=CARTESIAN_POINT ( 'NONE',  ( 37.00000000000000711, 4.705694406421931860E-17, -3.469127814946512892E-15 ) ) ;
#20072=CYLINDRICAL_SURFACE ( 'NONE', #12321, 12.18650000000000055 ) ;
#20073=CARTESIAN_POINT ( 'NONE',  ( 3.329269835863156501, 3.383330847102705263, 11.51505321664975412 ) ) ;
#20074=DIRECTION ( 'NONE',  ( 0.000000000000000000, -0.01356324068817999114, 0.9999080150203989437 ) ) ;
#20076=VERTEX_POINT ( 'NONE', #13689 ) ;
#20079=CARTESIAN_POINT ( 'NONE',  ( 3.419514237176616067, 7.633187743098319267, -9.298209040439605388 ) ) ;
#20082=DIRECTION ( 'NONE',  ( -1.000000000000000000, 0.000000000000000000, 0.000000000000000000 ) ) ;
#20086=ORIENTED_EDGE ( 'NONE', *, *, #62484, .T. ) ;
#20087=AXIS2_PLACEMENT_3D ( 'NONE', #6153, #26419, #41369 ) ;
#20089=ORIENTED_EDGE ( 'NONE', *, *, #19694, .T. ) ;
#20091=CARTESIAN_POINT ( 'NONE',  ( 37.00000000000000711, 4.705694406421931860E-17, -3.469127814946512892E-15 ) ) ;
#20093=FACE_OUTER_BOUND ( 'NONE', #13291, .T. ) ;
#20094=FACE_OUTER_BOUND ( 'NONE', #25895, .T. ) ;
#20096=DIRECTION ( 'NONE',  ( 0.000000000000000000, -0.01356324068818000848, 0.9999080150203990547 ) ) ;
#20098=VERTEX_POINT ( 'NONE', #38305 ) ;
#20099=CYLINDRICAL_SURFACE ( 'NONE', #21435, 13.50000000000000178 ) ;
#20100=ORIENTED_EDGE ( 'NONE', *, *, #28579, .F. ) ;
#20109=CARTESIAN_POINT ( 'NONE',  ( -36.00000000000000711, -4.237174932027141239, -12.02534193257725725 ) ) ;
#20110=DIRECTION ( 'NONE',  ( -1.000000000000000000, 0.000000000000000000, 0.000000000000000000 ) ) ;
#20111=LINE ( 'NONE', #25108, #50093 ) ;
#20112=VERTEX_POINT ( 'NONE', #38972 ) ;
#20113=VERTEX_POINT ( 'NONE', #48974 ) ;
#20115=ORIENTED_EDGE ( 'NONE', *, *, #65433, .F. ) ;
#20117=ADVANCED_FACE ( 'NONE', ( #4058 ), #34306, .T. ) ;
#20119=DIRECTION ( 'NONE',  ( -1.000000000000000000, 0.000000000000000000, 0.000000000000000000 ) ) ;
#20122=CARTESIAN_POINT ( 'NONE',  ( 18.21295819262132554, -5.177675556671182733, 10.87722373139338572 ) ) ;
#20123=DIRECTION ( 'NONE',  ( -1.000000000000000000, 0.000000000000000000, 0.000000000000000000 ) ) ;
#20124=CARTESIAN_POINT ( 'NONE',  ( 37.00000000000000711, 10.70999494708492250, -5.814360711498331113 ) ) ;
#20125=AXIS2_PLACEMENT_3D ( 'NONE', #28564, #65434, #64772 ) ;
#20126=DIRECTION ( 'NONE',  ( 1.000000000000000000, 0.000000000000000000, -0.000000000000000000 ) ) ;
#20127=ORIENTED_EDGE ( 'NONE', *, *, #8853, .T. ) ;
#20128=AXIS2_PLACEMENT_3D ( 'NONE', #62812, #17278, #36226 ) ;
#20131=CARTESIAN_POINT ( 'NONE',  ( 37.00000000000000711, 4.986700593229853595, 10.63508530065516311 ) ) ;
#20134=ADVANCED_FACE ( 'NONE', ( #29007 ), #7741, .T. ) ;
#20135=CARTESIAN_POINT ( 'NONE',  ( 6.645030759940484977, -5.062125397348413713, 10.88741911013856267 ) ) ;
#20138=CARTESIAN_POINT ( 'NONE',  ( 24.36109623891380949, -0.0007059690029652561632, -13.50466814640359914 ) ) ;
#20140=EDGE_CURVE ( 'NONE', #10101, #41887, #2776, .T. ) ;
#20142=ORIENTED_EDGE ( 'NONE', *, *, #19638, .T. ) ;
#20144=DIRECTION ( 'NONE',  ( 0.000000000000000000, 0.5987040770935622147, -0.8009703041134208501 ) ) ;
#20145=DIRECTION ( 'NONE',  ( 1.000000000000000000, 0.000000000000000000, 0.000000000000000000 ) ) ;
#20151=CARTESIAN_POINT ( 'NONE',  ( 35.00000000000000000, -7.146664589317845540, 9.321877890560507751 ) ) ;
#20153=ORIENTED_EDGE ( 'NONE', *, *, #18900, .F. ) ;
#20155=DIRECTION ( 'NONE',  ( 1.000000000000000000, -0.000000000000000000, 0.000000000000000000 ) ) ;
#20159=DIRECTION ( 'NONE',  ( 0.000000000000000000, 0.8696919319575200369, 0.4935949184179230786 ) ) ;
#20160=AXIS2_PLACEMENT_3D ( 'NONE', #11322, #46260, #55895 ) ;
#20161=EDGE_CURVE ( 'NONE', #17080, #13015, #19394, .T. ) ;
#20162=VECTOR ( 'NONE', #25868, 1000.000000000000000 ) ;
#20163=CARTESIAN_POINT ( 'NONE',  ( 35.00000000000000000, 11.71932350927024657, -3.511386971104992760 ) ) ;
#20167=CARTESIAN_POINT ( 'NONE',  ( -2.682146249266192939, -4.811221336669188275, 10.99569137319423007 ) ) ;
#20168=DIRECTION ( 'NONE',  ( 0.000000000000000000, 0.01356324068817998940, -0.9999080150203990547 ) ) ;
#20171=CARTESIAN_POINT ( 'NONE',  ( -17.68605346665446731, 2.867042001558842035, 13.19364479757039454 ) ) ;
#20172=FACE_OUTER_BOUND ( 'NONE', #4133, .T. ) ;
#20173=ORIENTED_EDGE ( 'NONE', *, *, #33703, .F. ) ;
#20174=DIRECTION ( 'NONE',  ( 0.000000000000000000, -0.01356324068817991828, 0.9999080150203990547 ) ) ;
#20175=ORIENTED_EDGE ( 'NONE', *, *, #10532, .F. ) ;
#20176=ADVANCED_FACE ( 'NONE', ( #14654 ), #45935, .T. ) ;
#20178=CARTESIAN_POINT ( 'NONE',  ( 35.00000000000000000, 8.954052073409734192, 9.076753354953893904 ) ) ;
#20180=VECTOR ( 'NONE', #55415, 1000.000000000000000 ) ;
#20184=CYLINDRICAL_SURFACE ( 'NONE', #35070, 11.99999999999998579 ) ;
#20185=ORIENTED_EDGE ( 'NONE', *, *, #60748, .T. ) ;
#20187=CARTESIAN_POINT ( 'NONE',  ( -36.00000000000000711, -5.300372733891724586, 11.59605747147784882 ) ) ;
#20188=ADVANCED_FACE ( 'NONE', ( #25985 ), #4739, .T. ) ;
#20189=ADVANCED_FACE ( 'NONE', ( #10664 ), #39951, .T. ) ;
#20190=VERTEX_POINT ( 'NONE', #9682 ) ;
#20191=DIRECTION ( 'NONE',  ( 1.000000000000000000, 0.000000000000000000, -0.000000000000000000 ) ) ;
#20192=CARTESIAN_POINT ( 'NONE',  ( -37.00000000000000711, 0.000000000000000000, 0.000000000000000000 ) ) ;
#20196=CARTESIAN_POINT ( 'NONE',  ( -35.00000000000000000, 5.428340790341860789, -10.91072401419405402 ) ) ;
#20198=DIRECTION ( 'NONE',  ( 1.000000000000000000, -0.000000000000000000, 0.000000000000000000 ) ) ;
#20202=DIRECTION ( 'NONE',  ( 1.000000000000000000, 0.000000000000000000, 0.000000000000000000 ) ) ;
#20203=CARTESIAN_POINT ( 'NONE',  ( 10.52156035929954392, 13.42709648837756475, -1.404459109811407203 ) ) ;
#20205=DIRECTION ( 'NONE',  ( 0.000000000000000000, -0.01356324068817991828, 0.9999080150203990547 ) ) ;
#20206=DIRECTION ( 'NONE',  ( -1.000000000000000000, 0.000000000000000000, 0.000000000000000000 ) ) ;
#20207=CARTESIAN_POINT ( 'NONE',  ( 35.00000000000000000, 4.705694406421931860E-17, -3.469127814946512892E-15 ) ) ;
#20208=ADVANCED_FACE ( 'NONE', ( #46270 ), #4397, .T. ) ;
#20209=AXIS2_PLACEMENT_3D ( 'NONE', #36160, #11243, #41477 ) ;
#20210=VECTOR ( 'NONE', #45394, 1000.000000000000000 ) ;
#20212=CIRCLE ( 'NONE', #13827, 5.000000000000001776 ) ;
#20213=DIRECTION ( 'NONE',  ( 1.000000000000000000, 0.000000000000000000, 0.000000000000000000 ) ) ;
#20214=EDGE_CURVE ( 'NONE', #20076, #42325, #5655, .T. ) ;
#20215=ORIENTED_EDGE ( 'NONE', *, *, #48446, .F. ) ;
#20216=CARTESIAN_POINT ( 'NONE',  ( 47.00000000000000711, 4.705694406421931860E-17, -3.469127814946512892E-15 ) ) ;
#20217=CARTESIAN_POINT ( 'NONE',  ( -29.68541646480307250, -1.416020129149132334, 11.91616074890920451 ) ) ;
#20218=DIRECTION ( 'NONE',  ( -1.000000000000000000, 0.000000000000000000, -0.000000000000000000 ) ) ;
#20221=ORIENTED_EDGE ( 'NONE', *, *, #37159, .T. ) ;
#20222=DIRECTION ( 'NONE',  ( 0.2235469969004301449, -0.9746931518056330956, 0.000000000000000000 ) ) ;
#20226=VECTOR ( 'NONE', #57432, 1000.000000000000000 ) ;
#20227=CYLINDRICAL_SURFACE ( 'NONE', #63819, 5.000000000000000888 ) ;
#20228=LINE ( 'NONE', #10246, #11704 ) ;
#20229=ORIENTED_EDGE ( 'NONE', *, *, #10667, .T. ) ;
#20230=CARTESIAN_POINT ( 'NONE',  ( -37.00000000000000711, 0.000000000000000000, 0.000000000000000000 ) ) ;
#20231=ORIENTED_EDGE ( 'NONE', *, *, #10514, .F. ) ;
#20234=AXIS2_PLACEMENT_3D ( 'NONE', #1571, #21845, #48101 ) ;
#20236=DIRECTION ( 'NONE',  ( 1.000000000000000000, -0.000000000000000000, 0.000000000000000000 ) ) ;
#20237=ORIENTED_EDGE ( 'NONE', *, *, #29753, .T. ) ;
#20239=CYLINDRICAL_SURFACE ( 'NONE', #54180, 5.000000000000000888 ) ;
#20241=ADVANCED_FACE ( 'NONE', ( #24665 ), #51263, .T. ) ;
#20243=CARTESIAN_POINT ( 'NONE',  ( -35.00000000000000000, -11.99999999999998579, 0.000000000000000000 ) ) ;
#20247=DIRECTION ( 'NONE',  ( 0.000000000000000000, -0.01356324068817992522, 0.9999080150203990547 ) ) ;
#20248=CARTESIAN_POINT ( 'NONE',  ( -18.22624239770570753, -11.73180942638131086, 2.608750867700459608 ) ) ;
#20249=ORIENTED_EDGE ( 'NONE', *, *, #5941, .T. ) ;
#20250=AXIS2_PLACEMENT_3D ( 'NONE', #64640, #3522, #53721 ) ;
#20254=AXIS2_PLACEMENT_3D ( 'NONE', #59996, #24085, #38387 ) ;
#20255=CARTESIAN_POINT ( 'NONE',  ( -37.00000000000000711, 0.000000000000000000, 0.000000000000000000 ) ) ;
#20256=AXIS2_PLACEMENT_3D ( 'NONE', #59170, #13584, #39846 ) ;
#20257=EDGE_CURVE ( 'NONE', #22753, #28214, #32075, .T. ) ;
#20258=VECTOR ( 'NONE', #52734, 1000.000000000000000 ) ;
#20260=DIRECTION ( 'NONE',  ( -1.000000000000000000, 0.000000000000000000, 0.000000000000000000 ) ) ;
#20262=CARTESIAN_POINT ( 'NONE',  ( 36.00000000000000711, 6.711949091238144760, -10.84030624090609152 ) ) ;
#20263=CARTESIAN_POINT ( 'NONE',  ( 6.806460418408726731, -6.060177178964488043, -12.06934091410146870 ) ) ;
#20265=DIRECTION ( 'NONE',  ( 1.000000000000000000, 0.000000000000000000, -0.000000000000000000 ) ) ;
#20266=CARTESIAN_POINT ( 'NONE',  ( 7.137024968749563492, -4.954338426407852047, 10.93925397463267757 ) ) ;
#20272=B_SPLINE_CURVE_WITH_KNOTS ( 'NONE', 3,
 ( #33937, #60196, #49274, #23987, #19962, #40230, #59549, #8351, #44247, #24293, #64518, #9008, #29291, #49586, #4025, #14620, #64840, #39589 ),
 .UNSPECIFIED., .F., .F.,
 ( 4, 2, 2, 2, 2, 2, 2, 2, 4 ),
 ( 0.000000000000000000, 0.0008755766307286345571, 0.001751153261457269114, 0.002626729892185903671, 0.003502306522914538228, 0.004377883153643172785, 0.005253459784371807342, 0.006129036415100441899, 0.007004613045829076456 ),
 .UNSPECIFIED. ) ;
#20273=CARTESIAN_POINT ( 'NONE',  ( -37.00000000000000711, 0.000000000000000000, 0.000000000000000000 ) ) ;
#20274=ORIENTED_EDGE ( 'NONE', *, *, #17636, .F. ) ;
#20277=CIRCLE ( 'NONE', #59580, 12.18649999999999878 ) ;
#20278=CARTESIAN_POINT ( 'NONE',  ( -37.00000000000000711, -11.73463472867573643, -3.287724142101541958 ) ) ;
#20280=VECTOR ( 'NONE', #60301, 1000.000000000000000 ) ;
#20283=DIRECTION ( 'NONE',  ( -1.000000000000000000, 0.000000000000000000, 0.000000000000000000 ) ) ;
#20284=VERTEX_POINT ( 'NONE', #55590 ) ;
#20285=AXIS2_PLACEMENT_3D ( 'NONE', #10637, #45914, #20646 ) ;
#20287=AXIS2_PLACEMENT_3D ( 'NONE', #7226, #21212, #57140 ) ;
#20288=VERTEX_POINT ( 'NONE', #5044 ) ;
#20289=DIRECTION ( 'NONE',  ( 1.000000000000000000, 0.000000000000000000, 0.000000000000000000 ) ) ;
#20291=CIRCLE ( 'NONE', #51104, 4.999999999999999112 ) ;
#20292=EDGE_LOOP ( 'NONE', ( #54, #3816, #20055, #44465 ) ) ;
#20293=CARTESIAN_POINT ( 'NONE',  ( -27.74367520006269672, 12.26553276005925142, -5.646909315955152664 ) ) ;
#20296=ORIENTED_EDGE ( 'NONE', *, *, #5905, .T. ) ;
#20297=DIRECTION ( 'NONE',  ( -1.000000000000000000, 0.000000000000000000, 0.000000000000000000 ) ) ;
#20298=CIRCLE ( 'NONE', #48991, 5.000000000000000000 ) ;
#20301=CARTESIAN_POINT ( 'NONE',  ( -18.63139410836038934, -13.49999999999999645, -0.3569054240395071464 ) ) ;
#20306=CARTESIAN_POINT ( 'NONE',  ( 35.00000000000000000, 10.23119532541072552, -7.608228585767763619 ) ) ;
#20307=DIRECTION ( 'NONE',  ( -0.000000000000000000, -0.000000000000000000, -1.000000000000000000 ) ) ;
#20308=CARTESIAN_POINT ( 'NONE',  ( 37.00000000000000711, 11.72195762423409704, 0.7536123767498881243 ) ) ;
#20309=FACE_OUTER_BOUND ( 'NONE', #45222, .T. ) ;
#20312=DIRECTION ( 'NONE',  ( -1.000000000000000000, -0.000000000000000000, 0.000000000000000000 ) ) ;
#20314=CARTESIAN_POINT ( 'NONE',  ( -35.00000000000000000, 0.000000000000000000, 0.000000000000000000 ) ) ;
#20315=CYLINDRICAL_SURFACE ( 'NONE', #61988, 12.18649999999999878 ) ;
#20316=VECTOR ( 'NONE', #20771, 1000.000000000000000 ) ;
#20317=EDGE_CURVE ( 'NONE', #50474, #35130, #10337, .T. ) ;
#20318=ORIENTED_EDGE ( 'NONE', *, *, #39277, .F. ) ;
#20321=EDGE_LOOP ( 'NONE', ( #14844, #63255, #56084, #30681 ) ) ;
#20323=CARTESIAN_POINT ( 'NONE',  ( 37.00000000000000711, 4.237174932027401475, 12.02534193257715600 ) ) ;
#20324=DIRECTION ( 'NONE',  ( 0.000000000000000000, -0.8696919319575238116, -0.4935949184179166949 ) ) ;
#20327=ORIENTED_EDGE ( 'NONE', *, *, #33201, .F. ) ;
#20328=ORIENTED_EDGE ( 'NONE', *, *, #53812, .T. ) ;
#20331=DIRECTION ( 'NONE',  ( 1.000000000000000000, 0.000000000000000000, 0.000000000000000000 ) ) ;
#20332=EDGE_CURVE ( 'NONE', #44597, #28690, #49162, .T. ) ;
#20333=EDGE_LOOP ( 'NONE', ( #55533, #1882, #50564, #43070 ) ) ;
#20334=DIRECTION ( 'NONE',  ( -1.000000000000000000, -1.836970198721029688E-16, 0.000000000000000000 ) ) ;
#20335=CIRCLE ( 'NONE', #36233, 4.999999999999998224 ) ;
#20340=EDGE_CURVE ( 'NONE', #48418, #16579, #24743, .T. ) ;
#20342=CARTESIAN_POINT ( 'NONE',  ( 35.00000000000000000, -12.08151691381186943, 4.074242145636128853 ) ) ;
#20343=VERTEX_POINT ( 'NONE', #62197 ) ;
#20344=AXIS2_PLACEMENT_3D ( 'NONE', #26585, #40908, #46236 ) ;
#20345=DIRECTION ( 'NONE',  ( 0.000000000000000000, -0.01356324068817998767, 0.9999080150203990547 ) ) ;
#20346=ORIENTED_EDGE ( 'NONE', *, *, #269, .T. ) ;
#20348=B_SPLINE_CURVE_WITH_KNOTS ( 'NONE', 3,
 ( #12203, #2243, #17202, #7891, #12856, #18191, #58774, #37806, #33139, #18539, #3229, #43109 ),
 .UNSPECIFIED., .F., .F.,
 ( 4, 2, 2, 2, 2, 4 ),
 ( 0.006679463946646270120, 0.007945415845128882618, 0.008578391794370190601, 0.009211367743611496850, 0.01047731964209411108, 0.01174327154057672531 ),
 .UNSPECIFIED. ) ;
#20350=DIRECTION ( 'NONE',  ( 0.000000000000000000, -0.01356324068817992175, 0.9999080150203990547 ) ) ;
#20351=CARTESIAN_POINT ( 'NONE',  ( 13.38593951179966623, -10.48414865564773635, -5.855826257454635808 ) ) ;
#20352=CARTESIAN_POINT ( 'NONE',  ( -35.00000000000000000, -10.32377448871672598, 6.475373545682264975 ) ) ;
#20354=LINE ( 'NONE', #20996, #53825 ) ;
#20357=CARTESIAN_POINT ( 'NONE',  ( -30.18541646480307250, -1.416020129149132112, 11.91616074890920096 ) ) ;
#20358=AXIS2_PLACEMENT_3D ( 'NONE', #29390, #9760, #50359 ) ;
#20359=CARTESIAN_POINT ( 'NONE',  ( -37.00000000000000711, 10.30098186818257666, -5.644643009978957515 ) ) ;
#20360=CARTESIAN_POINT ( 'NONE',  ( 35.00000000000000000, -11.13736569743270621, 4.946702696913284569 ) ) ;
#20362=CARTESIAN_POINT ( 'NONE',  ( 7.119412768985514894, -4.899345716645643556, 12.58666189623589382 ) ) ;
#20363=ORIENTED_EDGE ( 'NONE', *, *, #60284, .F. ) ;
#20364=ADVANCED_FACE ( 'NONE', ( #16331 ), #31601, .T. ) ;
#20367=DIRECTION ( 'NONE',  ( -1.000000000000000000, 0.000000000000000000, 0.000000000000000000 ) ) ;
#20368=ORIENTED_EDGE ( 'NONE', *, *, #4307, .F. ) ;
#20369=CYLINDRICAL_SURFACE ( 'NONE', #32267, 4.999999999999999112 ) ;
#20370=ORIENTED_EDGE ( 'NONE', *, *, #38834, .F. ) ;
#20372=CARTESIAN_POINT ( 'NONE',  ( 35.00000000000000000, 6.547236723514018308, -9.752226076388918585 ) ) ;
#20373=DIRECTION ( 'NONE',  ( 1.000000000000000000, 0.000000000000000000, 0.000000000000000000 ) ) ;
#20374=LINE ( 'NONE', #40655, #13593 ) ;
#20375=CIRCLE ( 'NONE', #28866, 12.18649999999999878 ) ;
#20376=CIRCLE ( 'NONE', #57554, 5.000000000000000888 ) ;
#20377=CARTESIAN_POINT ( 'NONE',  ( 3.618261583105321755, 8.318251859915347879, -10.63289868894575285 ) ) ;
#20379=DIRECTION ( 'NONE',  ( -0.4327406564646559262, 0.9015184547431841500, 0.000000000000000000 ) ) ;
#20380=CIRCLE ( 'NONE', #54377, 5.000000000000000000 ) ;
#20381=ORIENTED_EDGE ( 'NONE', *, *, #2130, .T. ) ;
#20384=FACE_OUTER_BOUND ( 'NONE', #48509, .T. ) ;
#20385=CARTESIAN_POINT ( 'NONE',  ( -2.682146249266190718, 4.811221336669198045, 10.99569137319423007 ) ) ;
#20386=ORIENTED_EDGE ( 'NONE', *, *, #25476, .T. ) ;
#20387=AXIS2_PLACEMENT_3D ( 'NONE', #2892, #23151, #63693 ) ;
#20391=( BOUNDED_CURVE ( )  B_SPLINE_CURVE ( 3, ( #39491, #59788, #54806, #7954 ),
 .UNSPECIFIED., .F., .F. ) 
 B_SPLINE_CURVE_WITH_KNOTS ( ( 4, 4 ),
 ( 5.030260039792340265, 5.070137490277369707 ),
 .UNSPECIFIED. ) 
 CURVE ( )  GEOMETRIC_REPRESENTATION_ITEM ( )  RATIONAL_B_SPLINE_CURVE ( ( 1.000000000000000000, 0.9998674868020707152, 0.9998674868020707152, 1.000000000000000000 ) ) 
 REPRESENTATION_ITEM ( '' )  );
#20393=CARTESIAN_POINT ( 'NONE',  ( -6.985495616976492350, -1.802010734008522741, 13.38029624267572082 ) ) ;
#20395=ORIENTED_EDGE ( 'NONE', *, *, #47287, .F. ) ;
#20397=CARTESIAN_POINT ( 'NONE',  ( -35.00000000000000000, 6.265926637539494415, 11.10408318471061584 ) ) ;
#20399=AXIS2_PLACEMENT_3D ( 'NONE', #52076, #6525, #47100 ) ;
#20401=AXIS2_PLACEMENT_3D ( 'NONE', #45814, #44486, #45160 ) ;
#20407=DIRECTION ( 'NONE',  ( 0.000000000000000000, -0.01356324068817998940, 0.9999080150203990547 ) ) ;
#20408=CARTESIAN_POINT ( 'NONE',  ( -1.734723475976807094E-15, -3.469446951953614189E-15, -11.99999999999998934 ) ) ;
#20411=FACE_OUTER_BOUND ( 'NONE', #63646, .T. ) ;
#20414=ORIENTED_EDGE ( 'NONE', *, *, #60444, .F. ) ;
#20415=ORIENTED_EDGE ( 'NONE', *, *, #48537, .F. ) ;
#20416=ORIENTED_EDGE ( 'NONE', *, *, #39526, .F. ) ;
#20417=AXIS2_PLACEMENT_3D ( 'NONE', #50459, #25487, #15505 ) ;
#20418=EDGE_CURVE ( 'NONE', #51873, #65690, #47566, .T. ) ;
#20420=CYLINDRICAL_SURFACE ( 'NONE', #25968, 12.74999999999999822 ) ;
#20423=CARTESIAN_POINT ( 'NONE',  ( 8.937200413559443390, 4.476360154859203355, 11.13383131558893346 ) ) ;
#20424=CIRCLE ( 'NONE', #63988, 12.18649999999999878 ) ;
#20425=DIRECTION ( 'NONE',  ( 0.000000000000000000, 0.9718671068226450993, -0.2355298848897551256 ) ) ;
#20427=CIRCLE ( 'NONE', #28928, 5.000000000000000000 ) ;
#20429=CARTESIAN_POINT ( 'NONE',  ( -17.54726996257253191, 11.36053454945672847, 3.865003848717349033 ) ) ;
#20430=CARTESIAN_POINT ( 'NONE',  ( -35.00000000000000000, -11.66953048682402283, 3.511814412392074480 ) ) ;
#20431=ORIENTED_EDGE ( 'NONE', *, *, #63899, .F. ) ;
#20432=CARTESIAN_POINT ( 'NONE',  ( -35.00000000000000000, -5.130401251914653571, -11.05394794832835359 ) ) ;
#20433=ADVANCED_FACE ( 'NONE', ( #17647 ), #8970, .T. ) ;
#20434=EDGE_LOOP ( 'NONE', ( #50785, #5128, #64150, #44966 ) ) ;
#20435=DIRECTION ( 'NONE',  ( 0.000000000000000000, 0.01356324068817992175, -0.9999080150203990547 ) ) ;
#20436=ORIENTED_EDGE ( 'NONE', *, *, #26646, .F. ) ;
#20438=DIRECTION ( 'NONE',  ( -1.000000000000000000, 0.000000000000000000, 0.000000000000000000 ) ) ;
#20439=EDGE_CURVE ( 'NONE', #47144, #55517, #37909, .T. ) ;
#20441=DIRECTION ( 'NONE',  ( 0.000000000000000000, 0.01356324068817998940, -0.9999080150203990547 ) ) ;
#20447=VECTOR ( 'NONE', #24879, 1000.000000000000000 ) ;
#20448=ORIENTED_EDGE ( 'NONE', *, *, #57584, .T. ) ;
#20449=DIRECTION ( 'NONE',  ( 1.000000000000000000, -0.000000000000000000, 0.000000000000000000 ) ) ;
#20450=ORIENTED_EDGE ( 'NONE', *, *, #39872, .F. ) ;
#20452=EDGE_LOOP ( 'NONE', ( #9080, #44546, #41098, #25730 ) ) ;
#20453=CARTESIAN_POINT ( 'NONE',  ( -36.00000000000000711, 0.3137578094509230753, 12.74613886779085270 ) ) ;
#20454=AXIS2_PLACEMENT_3D ( 'NONE', #23959, #38583, #44874 ) ;
#20456=CARTESIAN_POINT ( 'NONE',  ( 34.00000000000000000, 1.267509437117510519E-14, 0.000000000000000000 ) ) ;
#20460=CARTESIAN_POINT ( 'NONE',  ( -37.00000000000000711, 0.000000000000000000, 0.000000000000000000 ) ) ;
#20461=AXIS2_PLACEMENT_3D ( 'NONE', #37980, #17048, #58283 ) ;
#20462=ORIENTED_EDGE ( 'NONE', *, *, #61756, .T. ) ;
#20464=CARTESIAN_POINT ( 'NONE',  ( -37.00000000000000711, 0.000000000000000000, 0.000000000000000000 ) ) ;
#20466=AXIS2_PLACEMENT_3D ( 'NONE', #56033, #26430, #65665 ) ;
#20468=CIRCLE ( 'NONE', #62939, 5.000000000000000000 ) ;
#20470=CARTESIAN_POINT ( 'NONE',  ( 4.631701379227551207, -10.10996076783195008, 6.470577568759368070 ) ) ;
#20471=DIRECTION ( 'NONE',  ( -1.000000000000000000, 0.000000000000000000, 0.000000000000000000 ) ) ;
#20472=DIRECTION ( 'NONE',  ( -1.000000000000000000, 0.000000000000000000, -0.000000000000000000 ) ) ;
#20473=CARTESIAN_POINT ( 'NONE',  ( 2.102182802109547666, 1.287158751533839629, -11.93215772323105561 ) ) ;
#20474=VECTOR ( 'NONE', #25684, 1000.000000000000000 ) ;
#20475=LINE ( 'NONE', #55389, #12927 ) ;
#20478=CYLINDRICAL_SURFACE ( 'NONE', #59015, 4.999999999999999112 ) ;
#20481=CARTESIAN_POINT ( 'NONE',  ( 47.00000000000000711, 4.705694406421931860E-17, -3.469127814946512892E-15 ) ) ;
#20482=EDGE_CURVE ( 'NONE', #27103, #5815, #23950, .T. ) ;
#20484=DIRECTION ( 'NONE',  ( 1.000000000000000000, 0.000000000000000000, -0.000000000000000000 ) ) ;
#20485=ORIENTED_EDGE ( 'NONE', *, *, #56058, .T. ) ;
#20487=DIRECTION ( 'NONE',  ( 1.000000000000000000, 0.000000000000000000, 0.000000000000000000 ) ) ;
#20489=VERTEX_POINT ( 'NONE', #33900 ) ;
#20490=CARTESIAN_POINT ( 'NONE',  ( -36.00000000000000711, -12.49688848680886011, 2.527899948230591942 ) ) ;
#20491=CARTESIAN_POINT ( 'NONE',  ( -14.51259464223477735, 7.865023325494275852, -9.063844199178094030 ) ) ;
#20493=EDGE_CURVE ( 'NONE', #22257, #43258, #35310, .T. ) ;
#20498=VECTOR ( 'NONE', #34298, 1000.000000000000000 ) ;
#20499=VECTOR ( 'NONE', #42150, 1000.000000000000000 ) ;
#20501=ORIENTED_EDGE ( 'NONE', *, *, #53688, .T. ) ;
#20502=CARTESIAN_POINT ( 'NONE',  ( 0.2851083653049504285, -0.4107471485392698018, -11.99296822225284131 ) ) ;
#20503=DIRECTION ( 'NONE',  ( -1.000000000000000000, -0.000000000000000000, 0.000000000000000000 ) ) ;
#20504=CARTESIAN_POINT ( 'NONE',  ( -17.65816380191525425, 7.464113067668815660, -11.25126181107559553 ) ) ;
#20505=DIRECTION ( 'NONE',  ( 0.000000000000000000, -0.01356324068817998940, 0.9999080150203990547 ) ) ;
#20507=CIRCLE ( 'NONE', #22655, 5.000000000000000000 ) ;
#20508=DIRECTION ( 'NONE',  ( 0.000000000000000000, 0.9796553971857735466, 0.2006870767258926436 ) ) ;
#20509=CARTESIAN_POINT ( 'NONE',  ( 37.00000000000000711, -12.14284015767850455, -1.030638227056526413 ) ) ;
#20511=DIRECTION ( 'NONE',  ( 1.000000000000000000, 0.000000000000000000, 0.000000000000000000 ) ) ;
#20512=AXIS2_PLACEMENT_3D ( 'NONE', #64776, #14255, #8952 ) ;
#20513=ORIENTED_EDGE ( 'NONE', *, *, #30165, .T. ) ;
#20515=DIRECTION ( 'NONE',  ( 1.000000000000000000, 0.000000000000000000, 0.000000000000000000 ) ) ;
#20516=EDGE_CURVE ( 'NONE', #31372, #13725, #58701, .T. ) ;
#20517=AXIS2_PLACEMENT_3D ( 'NONE', #25159, #60738, #59761 ) ;
#20519=EDGE_CURVE ( 'NONE', #36611, #62352, #25789, .T. ) ;
#20521=ORIENTED_EDGE ( 'NONE', *, *, #8060, .T. ) ;
#20522=DIRECTION ( 'NONE',  ( -1.000000000000000000, 0.000000000000000000, 0.000000000000000000 ) ) ;
#20523=CARTESIAN_POINT ( 'NONE',  ( 11.74548640120467979, 8.775604215601129354, -8.184666801472349817 ) ) ;
#20524=CYLINDRICAL_SURFACE ( 'NONE', #54189, 11.99999999999999289 ) ;
#20525=ORIENTED_EDGE ( 'NONE', *, *, #20847, .F. ) ;
#20526=AXIS2_PLACEMENT_3D ( 'NONE', #56526, #10302, #15933 ) ;
#20527=ORIENTED_EDGE ( 'NONE', *, *, #55500, .F. ) ;
#20528=EDGE_CURVE ( 'NONE', #37925, #65184, #44912, .T. ) ;
#20529=CARTESIAN_POINT ( 'NONE',  ( 35.00000000000000000, -6.018036132182079889, 11.24036214326526562 ) ) ;
#20531=CARTESIAN_POINT ( 'NONE',  ( 22.22762455518017433, -10.97323854681321897, -4.869946340165640208 ) ) ;
#20535=LINE ( 'NONE', #61095, #34085 ) ;
#20536=DIRECTION ( 'NONE',  ( -0.000000000000000000, -1.000000000000000000, -0.000000000000000000 ) ) ;
#20538=CARTESIAN_POINT ( 'NONE',  ( -35.00000000000000000, -7.745827850122939395, -10.12742074351904975 ) ) ;
#20539=VERTEX_POINT ( 'NONE', #34228 ) ;
#20541=FACE_OUTER_BOUND ( 'NONE', #48572, .T. ) ;
#20542=DIRECTION ( 'NONE',  ( 1.000000000000000000, 0.000000000000000000, 0.000000000000000000 ) ) ;
#20543=AXIS2_PLACEMENT_3D ( 'NONE', #52163, #6615, #13227 ) ;
#20544=DIRECTION ( 'NONE',  ( 1.000000000000000000, 0.000000000000000000, 0.000000000000000000 ) ) ;
#20545=CARTESIAN_POINT ( 'NONE',  ( 35.00000000000000000, 6.584150480049550502, -10.25474254703955701 ) ) ;
#20546=DIRECTION ( 'NONE',  ( -0.000000000000000000, -0.000000000000000000, -1.000000000000000000 ) ) ;
#20547=CARTESIAN_POINT ( 'NONE',  ( -35.00000000000000000, 0.000000000000000000, 0.000000000000000000 ) ) ;
#20548=AXIS2_PLACEMENT_3D ( 'NONE', #2807, #23388, #43656 ) ;
#20550=CIRCLE ( 'NONE', #57725, 5.000000000000000888 ) ;
#20551=AXIS2_PLACEMENT_3D ( 'NONE', #39135, #58462, #48488 ) ;
#20552=EDGE_CURVE ( 'NONE', #23557, #42938, #60813, .T. ) ;
#20553=EDGE_LOOP ( 'NONE', ( #45351, #57503, #61757, #41261 ) ) ;
#20554=CARTESIAN_POINT ( 'NONE',  ( 37.00000000000000711, 11.90598845858539967, 4.561791185930283099 ) ) ;
#20555=EDGE_CURVE ( 'NONE', #53879, #29231, #30002, .T. ) ;
#20556=ORIENTED_EDGE ( 'NONE', *, *, #32039, .T. ) ;
#20557=CARTESIAN_POINT ( 'NONE',  ( -35.00000000000000000, -7.474872387600942858, -9.060822531526127932 ) ) ;
#20558=LINE ( 'NONE', #21543, #24529 ) ;
#20559=FACE_OUTER_BOUND ( 'NONE', #20967, .T. ) ;
#20560=AXIS2_PLACEMENT_3D ( 'NONE', #13579, #29525, #33868 ) ;
#20563=ORIENTED_EDGE ( 'NONE', *, *, #12500, .F. ) ;
#20564=CIRCLE ( 'NONE', #14135, 5.000000000000000888 ) ;
#20565=DIRECTION ( 'NONE',  ( 0.000000000000000000, 0.2960891610144510966, 0.9551603052523478521 ) ) ;
#20566=LINE ( 'NONE', #30209, #37384 ) ;
#20567=EDGE_CURVE ( 'NONE', #48396, #10868, #55496, .T. ) ;
#20570=VECTOR ( 'NONE', #11108, 1000.000000000000000 ) ;
#20571=CARTESIAN_POINT ( 'NONE',  ( -17.72572367302459639, -5.320256682235254608, 10.76019785545453722 ) ) ;
#20573=AXIS2_PLACEMENT_3D ( 'NONE', #56675, #52339, #6780 ) ;
#20574=ORIENTED_EDGE ( 'NONE', *, *, #56212, .F. ) ;
#20576=CARTESIAN_POINT ( 'NONE',  ( -37.00000000000000711, 10.32377448871677039, -6.475373545682194809 ) ) ;
#20580=EDGE_CURVE ( 'NONE', #15890, #52774, #19277, .T. ) ;
#20583=CARTESIAN_POINT ( 'NONE',  ( -9.606767908028034597, -3.747519102173751282, 11.40110431394993640 ) ) ;
#20584=CIRCLE ( 'NONE', #30115, 12.75000000000000178 ) ;
#20585=ORIENTED_EDGE ( 'NONE', *, *, #59834, .F. ) ;
#20587=DIRECTION ( 'NONE',  ( -0.000000000000000000, -0.000000000000000000, -1.000000000000000000 ) ) ;
#20588=ORIENTED_EDGE ( 'NONE', *, *, #31364, .T. ) ;
#20589=DIRECTION ( 'NONE',  ( -1.000000000000000000, 0.000000000000000000, -0.000000000000000000 ) ) ;
#20591=DIRECTION ( 'NONE',  ( -1.000000000000000000, -1.836970198721029688E-16, -0.000000000000000000 ) ) ;
#20599=ORIENTED_EDGE ( 'NONE', *, *, #63233, .F. ) ;
#20600=DIRECTION ( 'NONE',  ( -1.000000000000000000, 0.000000000000000000, 0.000000000000000000 ) ) ;
#20601=EDGE_CURVE ( 'NONE', #30121, #22151, #56600, .T. ) ;
#20602=CYLINDRICAL_SURFACE ( 'NONE', #43854, 5.000000000000000888 ) ;
#20603=ORIENTED_EDGE ( 'NONE', *, *, #37954, .F. ) ;
#20606=ORIENTED_EDGE ( 'NONE', *, *, #5156, .F. ) ;
#20607=CARTESIAN_POINT ( 'NONE',  ( -28.85619398320021745, 3.750539801530000439, -11.39883551934754280 ) ) ;
#20608=CARTESIAN_POINT ( 'NONE',  ( 6.742208325808031866, -7.058475617584183404, -11.51382290311167722 ) ) ;
#20609=CYLINDRICAL_SURFACE ( 'NONE', #47782, 12.74999999999999822 ) ;
#20611=ORIENTED_EDGE ( 'NONE', *, *, #55988, .T. ) ;
#20612=ORIENTED_EDGE ( 'NONE', *, *, #4458, .T. ) ;
#20614=VERTEX_POINT ( 'NONE', #29892 ) ;
#20616=ORIENTED_EDGE ( 'NONE', *, *, #65306, .F. ) ;
#20617=VECTOR ( 'NONE', #60374, 1000.000000000000000 ) ;
#20618=ORIENTED_EDGE ( 'NONE', *, *, #8120, .T. ) ;
#20620=ORIENTED_EDGE ( 'NONE', *, *, #60552, .T. ) ;
#20621=CARTESIAN_POINT ( 'NONE',  ( 35.00000000000000000, -5.246972444133939817, 10.99909370905162298 ) ) ;
#20623=CARTESIAN_POINT ( 'NONE',  ( -35.00000000000000000, 4.986700593229701717, 10.63508530065523772 ) ) ;
#20625=CYLINDRICAL_SURFACE ( 'NONE', #28735, 7.115568257478080305 ) ;
#20627=VERTEX_POINT ( 'NONE', #30864 ) ;
#20628=EDGE_CURVE ( 'NONE', #23325, #31648, #25235, .T. ) ;
#20629=CARTESIAN_POINT ( 'NONE',  ( -29.68541646480313645, -1.416020129149148543, -11.91616074890925780 ) ) ;
#20630=ORIENTED_EDGE ( 'NONE', *, *, #39710, .F. ) ;
#20631=CARTESIAN_POINT ( 'NONE',  ( -16.98800322446194855, 2.922502605998049674, 13.17987020110344787 ) ) ;
#20633=CARTESIAN_POINT ( 'NONE',  ( -2.532614230583026593, 7.965877694534055031, 10.89930238848911337 ) ) ;
#20634=DIRECTION ( 'NONE',  ( 1.000000000000000000, 0.000000000000000000, 0.000000000000000000 ) ) ;
#20635=CARTESIAN_POINT ( 'NONE',  ( -27.74685410543621344, 12.59748157192950480, -4.861485140711778286 ) ) ;
#20638=CIRCLE ( 'NONE', #57807, 12.18649999999999878 ) ;
#20640=DIRECTION ( 'NONE',  ( 0.000000000000000000, -0.9999080150203989437, -0.01356324068819032662 ) ) ;
#20641=EDGE_CURVE ( 'NONE', #19302, #52228, #39597, .T. ) ;
#20643=PLANE ( 'NONE',  #3063 ) ;
#20646=DIRECTION ( 'NONE',  ( 0.000000000000000000, -0.01356324068817999114, 0.9999080150203989437 ) ) ;
#20648=ORIENTED_EDGE ( 'NONE', *, *, #26977, .F. ) ;
#20649=CIRCLE ( 'NONE', #24909, 12.74999999999999822 ) ;
#20650=CIRCLE ( 'NONE', #12128, 12.74999999999999822 ) ;
#20651=LINE ( 'NONE', #10321, #19710 ) ;
#20652=CARTESIAN_POINT ( 'NONE',  ( 35.00000000000000000, -12.02534193257717554, 4.237174932027349961 ) ) ;
#20653=DIRECTION ( 'NONE',  ( 1.000000000000000000, 0.000000000000000000, 0.000000000000000000 ) ) ;
#20656=CARTESIAN_POINT ( 'NONE',  ( -21.17861794710831091, 13.00977982294135593, -3.604945070120774808 ) ) ;
#20659=EDGE_CURVE ( 'NONE', #17610, #43228, #20468, .T. ) ;
#20660=DIRECTION ( 'NONE',  ( 0.000000000000000000, 0.01356324068817991828, -0.9999080150203990547 ) ) ;
#20662=VECTOR ( 'NONE', #53007, 1000.000000000000000 ) ;
#20665=ORIENTED_EDGE ( 'NONE', *, *, #40231, .F. ) ;
#20668=LINE ( 'NONE', #40943, #15170 ) ;
#20670=EDGE_LOOP ( 'NONE', ( #14134, #28930, #35228, #18856 ) ) ;
#20671=ORIENTED_EDGE ( 'NONE', *, *, #36251, .T. ) ;
#20672=ORIENTED_EDGE ( 'NONE', *, *, #36398, .F. ) ;
#20674=EDGE_CURVE ( 'NONE', #43816, #65741, #14092, .T. ) ;
#20675=CARTESIAN_POINT ( 'NONE',  ( 35.00000000000000000, -8.258652103341374229, 8.352657516904754331 ) ) ;
#20676=EDGE_LOOP ( 'NONE', ( #29474, #34501, #52262, #50675 ) ) ;
#20677=CARTESIAN_POINT ( 'NONE',  ( -18.08686583997218733, 5.151216734910788908, -10.83812558286602012 ) ) ;
#20678=CARTESIAN_POINT ( 'NONE',  ( -35.00000000000000000, -5.644643009978993931, -10.30098186818255890 ) ) ;
#20683=VERTEX_POINT ( 'NONE', #50845 ) ;
#20684=DIRECTION ( 'NONE',  ( 1.000000000000000000, 0.000000000000000000, 0.000000000000000000 ) ) ;
#20685=ORIENTED_EDGE ( 'NONE', *, *, #31704, .T. ) ;
#20688=CARTESIAN_POINT ( 'NONE',  ( -35.00000000000000000, -5.865551165831157654, 11.32068061209293219 ) ) ;
#20691=ADVANCED_FACE ( 'NONE', ( #9272 ), #15258, .F. ) ;
#20692=CARTESIAN_POINT ( 'NONE',  ( 35.00000000000000000, 5.273331777780336793, -10.49591321039682690 ) ) ;
#20694=CYLINDRICAL_SURFACE ( 'NONE', #44617, 4.999999999999997335 ) ;
#20698=EDGE_LOOP ( 'NONE', ( #25683, #21972, #38766, #33128 ) ) ;
#20699=DIRECTION ( 'NONE',  ( -1.000000000000000000, -0.000000000000000000, 0.000000000000000000 ) ) ;
#20700=AXIS2_PLACEMENT_3D ( 'NONE', #57697, #7447, #32703 ) ;
#20701=ORIENTED_EDGE ( 'NONE', *, *, #35983, .T. ) ;
#20704=DIRECTION ( 'NONE',  ( 0.000000000000000000, -0.01356324068817992175, 0.9999080150203990547 ) ) ;
#20705=CIRCLE ( 'NONE', #57886, 4.999999999999999112 ) ;
#20706=EDGE_LOOP ( 'NONE', ( #29045, #17317, #31232, #45650 ) ) ;
#20707=DIRECTION ( 'NONE',  ( -1.000000000000000000, -0.000000000000000000, 0.000000000000000000 ) ) ;
#20709=DIRECTION ( 'NONE',  ( 0.000000000000000000, 0.9937233664769756780, -0.1118654143051653060 ) ) ;
#20710=B_SPLINE_CURVE_WITH_KNOTS ( 'NONE', 3,
 ( #50764, #231, #29179, #34478, #54779, #9514, #40440, #20504, #50115, #19846, #5214, #44439, #65697, #55422, #64717, #19188, #40107, #60399, #4572, #15177 ),
 .UNSPECIFIED., .F., .F.,
 ( 4, 2, 2, 2, 2, 2, 2, 2, 2, 4 ),
 ( 0.003127060359999195467, 0.003972907705248850986, 0.004818755050498505638, 0.005664602395748161157, 0.006510449740997816676, 0.007356297086247472194, 0.008202144431497127713, 0.009047991776746791906, 0.009470915449371621400, 0.009893839121996452629 ),
 .UNSPECIFIED. ) ;
#20712=CIRCLE ( 'NONE', #57888, 12.74999999999999822 ) ;
#20713=CARTESIAN_POINT ( 'NONE',  ( 35.00000000000000000, 4.705694406421931860E-17, -3.469127814946512892E-15 ) ) ;
#20714=ORIENTED_EDGE ( 'NONE', *, *, #48045, .F. ) ;
#20715=DIRECTION ( 'NONE',  ( 1.000000000000000000, 0.000000000000000000, 0.000000000000000000 ) ) ;
#20716=EDGE_CURVE ( 'NONE', #22402, #56626, #49862, .T. ) ;
#20717=VERTEX_POINT ( 'NONE', #44863 ) ;
#20718=DIRECTION ( 'NONE',  ( 1.000000000000000000, 0.000000000000000000, 0.000000000000000000 ) ) ;
#20719=ADVANCED_FACE ( 'NONE', ( #65142 ), #60477, .T. ) ;
#20721=ORIENTED_EDGE ( 'NONE', *, *, #39904, .F. ) ;
#20724=ADVANCED_FACE ( 'NONE', ( #11902 ), #639, .T. ) ;
#20725=LINE ( 'NONE', #40997, #18092 ) ;
#20727=DIRECTION ( 'NONE',  ( 0.000000000000000000, -0.01356324068817991828, 0.9999080150203990547 ) ) ;
#20730=DIRECTION ( 'NONE',  ( 0.000000000000000000, 0.01356324068817991828, -0.9999080150203990547 ) ) ;
#20734=B_SPLINE_CURVE_WITH_KNOTS ( 'NONE', 3,
 ( #35402, #55711, #15457, #35723, #10459, #52283, #51302, #36951, #16366, #41620, #36639, #5407, #26017, #31326 ),
 .UNSPECIFIED., .F., .F.,
 ( 4, 2, 2, 2, 2, 2, 4 ),
 ( 0.000000000000000000, 0.001263061922348848558, 0.001894592883523271102, 0.002526123844697694080, 0.003789185767046541337, 0.004420716728220965182, 0.005052247689395389027 ),
 .UNSPECIFIED. ) ;
#20735=EDGE_CURVE ( 'NONE', #19909, #45349, #16241, .T. ) ;
#20737=CARTESIAN_POINT ( 'NONE',  ( 17.27839441901508621, -12.20388373500082224, 5.771933972472480967 ) ) ;
#20738=CIRCLE ( 'NONE', #47295, 12.75000000000000178 ) ;
#20739=ORIENTED_EDGE ( 'NONE', *, *, #35510, .T. ) ;
#20741=CARTESIAN_POINT ( 'NONE',  ( 47.00000000000000711, 4.705694406421931860E-17, -3.469127814946512892E-15 ) ) ;
#20742=DIRECTION ( 'NONE',  ( 1.000000000000000000, 0.000000000000000000, 0.000000000000000000 ) ) ;
#20747=ORIENTED_EDGE ( 'NONE', *, *, #1871, .F. ) ;
#20749=AXIS2_PLACEMENT_3D ( 'NONE', #13470, #24782, #45060 ) ;
#20754=CARTESIAN_POINT ( 'NONE',  ( 9.272965915927473546, 6.113671464449896398, 10.33142599188169974 ) ) ;
#20757=DIRECTION ( 'NONE',  ( 0.000000000000000000, 0.4698238015817364777, 0.8827602140260315533 ) ) ;
#20759=ORIENTED_EDGE ( 'NONE', *, *, #41113, .F. ) ;
#20760=CARTESIAN_POINT ( 'NONE',  ( 22.88594695219327235, -4.822122601967141264, 25.00000000000000000 ) ) ;
#20761=EDGE_LOOP ( 'NONE', ( #32232, #38925, #30207, #62705 ) ) ;
#20764=EDGE_LOOP ( 'NONE', ( #32696, #23783, #64589, #27701 ) ) ;
#20767=CYLINDRICAL_SURFACE ( 'NONE', #34353, 5.000000000000000888 ) ;
#20768=EDGE_CURVE ( 'NONE', #65529, #18937, #10924, .T. ) ;
#20769=CARTESIAN_POINT ( 'NONE',  ( 37.00000000000000711, -12.49688848680882103, 2.527899948230768690 ) ) ;
#20771=DIRECTION ( 'NONE',  ( -1.000000000000000000, 0.000000000000000000, 0.000000000000000000 ) ) ;
#20772=ORIENTED_EDGE ( 'NONE', *, *, #61080, .T. ) ;
#20774=VERTEX_POINT ( 'NONE', #15896 ) ;
#20776=VERTEX_POINT ( 'NONE', #6934 ) ;
#20778=CARTESIAN_POINT ( 'NONE',  ( -37.00000000000000711, 0.000000000000000000, 0.000000000000000000 ) ) ;
#20779=CARTESIAN_POINT ( 'NONE',  ( -37.00000000000000711, 11.68758509253248334, -1.171570255487489609 ) ) ;
#20783=CARTESIAN_POINT ( 'NONE',  ( -7.994277101543554309, -1.718098006006025580, -11.87788732319827822 ) ) ;
#20785=CARTESIAN_POINT ( 'NONE',  ( 36.00000000000000711, -8.366449238204431538, -9.621072037176967129 ) ) ;
#20786=AXIS2_PLACEMENT_3D ( 'NONE', #63715, #22528, #11878 ) ;
#20789=ORIENTED_EDGE ( 'NONE', *, *, #36424, .F. ) ;
#20791=DIRECTION ( 'NONE',  ( 1.000000000000000000, 0.000000000000000000, 0.000000000000000000 ) ) ;
#20792=DIRECTION ( 'NONE',  ( 1.000000000000000000, 0.000000000000000000, 0.000000000000000000 ) ) ;
#20793=CARTESIAN_POINT ( 'NONE',  ( -3.116620688030298680, -9.325418049453649161, 9.768128050516612149 ) ) ;
#20795=CARTESIAN_POINT ( 'NONE',  ( 6.361445718264521432, -4.355102044641763648, 11.18181944858514498 ) ) ;
#20797=EDGE_CURVE ( 'NONE', #62352, #10311, #47496, .T. ) ;
#20798=CARTESIAN_POINT ( 'NONE',  ( 36.00000000000000711, 4.561791185930414549, -11.90598845858535704 ) ) ;
#20799=EDGE_CURVE ( 'NONE', #61423, #42768, #24795, .T. ) ;
#20800=FACE_OUTER_BOUND ( 'NONE', #39907, .T. ) ;
#20801=CYLINDRICAL_SURFACE ( 'NONE', #25700, 12.74999999999999822 ) ;
#20802=ORIENTED_EDGE ( 'NONE', *, *, #51650, .T. ) ;
#20805=CARTESIAN_POINT ( 'NONE',  ( 35.00000000000000000, -9.217970097227778936, -7.971186206369441862 ) ) ;
#20809=ORIENTED_EDGE ( 'NONE', *, *, #44402, .F. ) ;
#20810=CARTESIAN_POINT ( 'NONE',  ( -18.39961019094981509, -4.493736647258883110, -12.73074473482842883 ) ) ;
#20811=CARTESIAN_POINT ( 'NONE',  ( -37.00000000000000711, 10.01317267707896441, -6.946017217729827387 ) ) ;
#20813=EDGE_CURVE ( 'NONE', #9428, #14609, #62767, .T. ) ;
#20814=ORIENTED_EDGE ( 'NONE', *, *, #29753, .F. ) ;
#20816=LINE ( 'NONE', #5203, #12964 ) ;
#20817=CARTESIAN_POINT ( 'NONE',  ( -36.00000000000000711, 12.74068829017554094, 0.4871980014161925165 ) ) ;
#20818=CARTESIAN_POINT ( 'NONE',  ( -35.00000000000000000, -11.01837265713077585, 6.415447294506668285 ) ) ;
#20819=ORIENTED_EDGE ( 'NONE', *, *, #11648, .F. ) ;
#20824=VERTEX_POINT ( 'NONE', #42147 ) ;
#20826=CARTESIAN_POINT ( 'NONE',  ( -9.342997049464392134, 12.02615817703077283, -6.144013915069329812 ) ) ;
#20827=CARTESIAN_POINT ( 'NONE',  ( 24.40168093369100433, -0.3774522545360152748, -11.99947585575983844 ) ) ;
#20828=CARTESIAN_POINT ( 'NONE',  ( 10.16647825512967351, 8.042666982224721650, -10.84593607609787647 ) ) ;
#20829=DIRECTION ( 'NONE',  ( 0.000000000000000000, -0.01356324068817998940, 0.9999080150203990547 ) ) ;
#20830=LINE ( 'NONE', #56402, #39776 ) ;
#20833=CARTESIAN_POINT ( 'NONE',  ( -37.00000000000000711, 0.000000000000000000, 0.000000000000000000 ) ) ;
#20837=EDGE_CURVE ( 'NONE', #42300, #44156, #11973, .T. ) ;
#20839=CARTESIAN_POINT ( 'NONE',  ( -35.00000000000000000, 11.37311665002359540, 2.936739658820077370 ) ) ;
#20842=CARTESIAN_POINT ( 'NONE',  ( 12.89305137491219710, 10.53990944163839671, -5.751062137880654568 ) ) ;
#20843=DIRECTION ( 'NONE',  ( 1.000000000000000000, 0.000000000000000000, 0.000000000000000000 ) ) ;
#20844=ORIENTED_EDGE ( 'NONE', *, *, #28296, .T. ) ;
#20845=ORIENTED_EDGE ( 'NONE', *, *, #7668, .F. ) ;
#20846=FACE_OUTER_BOUND ( 'NONE', #44359, .T. ) ;
#20847=EDGE_CURVE ( 'NONE', #29772, #37649, #61950, .T. ) ;
#20852=DIRECTION ( 'NONE',  ( 0.000000000000000000, 0.3554799084908970563, 0.9346839223284539866 ) ) ;
#20854=CARTESIAN_POINT ( 'NONE',  ( 26.34661844826604593, -11.53221627053866527, 3.317828791472333005 ) ) ;
#20857=ORIENTED_EDGE ( 'NONE', *, *, #48446, .T. ) ;
#20858=DIRECTION ( 'NONE',  ( 0.000000000000000000, -0.01356324068817999114, 0.9999080150203989437 ) ) ;
#20859=CARTESIAN_POINT ( 'NONE',  ( 35.00000000000000000, -1.286231064351218478, 12.68495603654572612 ) ) ;
#20861=CARTESIAN_POINT ( 'NONE',  ( -37.00000000000000711, 8.017674001891920810, -9.913596905230035006 ) ) ;
#20862=CARTESIAN_POINT ( 'NONE',  ( -9.251009239874910861, 10.88051098239768955, -5.064585925472082195 ) ) ;
#20863=CARTESIAN_POINT ( 'NONE',  ( -35.00000000000000000, -8.295159312811792418, -8.927548052240984688 ) ) ;
#20865=DIRECTION ( 'NONE',  ( 1.000000000000000000, 0.000000000000000000, 0.000000000000000000 ) ) ;
#20867=EDGE_LOOP ( 'NONE', ( #32787, #54290, #30702, #9804 ) ) ;
#20868=CARTESIAN_POINT ( 'NONE',  ( -35.00000000000000000, 0.000000000000000000, 0.000000000000000000 ) ) ;
#20869=AXIS2_PLACEMENT_3D ( 'NONE', #38669, #52968, #13384 ) ;
#20872=EDGE_CURVE ( 'NONE', #11917, #27835, #18398, .T. ) ;
#20873=CARTESIAN_POINT ( 'NONE',  ( -47.00000000000000711, 0.000000000000000000, 0.000000000000000000 ) ) ;
#20875=DIRECTION ( 'NONE',  ( -0.000000000000000000, -0.000000000000000000, -1.000000000000000000 ) ) ;
#20876=ADVANCED_FACE ( 'NONE', ( #47816 ), #18220, .T. ) ;
#20877=ORIENTED_EDGE ( 'NONE', *, *, #64825, .T. ) ;
#20878=CARTESIAN_POINT ( 'NONE',  ( -35.00000000000000000, 9.557269938331666381, -7.561043153947866635 ) ) ;
#20880=LINE ( 'NONE', #50508, #53997 ) ;
#20881=EDGE_CURVE ( 'NONE', #41793, #50474, #14141, .T. ) ;
#20883=CARTESIAN_POINT ( 'NONE',  ( 37.00000000000000711, 11.02904044024202967, -4.041347439436060007 ) ) ;
#20886=DIRECTION ( 'NONE',  ( 0.000000000000000000, 0.6943713148249640588, -0.7196168960969792083 ) ) ;
#20893=ORIENTED_EDGE ( 'NONE', *, *, #23934, .F. ) ;
#20894=DIRECTION ( 'NONE',  ( 0.000000000000000000, -0.01356324068817991828, 0.9999080150203990547 ) ) ;
#20895=ORIENTED_EDGE ( 'NONE', *, *, #15510, .F. ) ;
#20897=DIRECTION ( 'NONE',  ( 0.000000000000000000, 0.2618041379715563277, -0.9651210252299813330 ) ) ;
#20901=DIRECTION ( 'NONE',  ( 0.000000000000000000, 0.9796553971857748788, 0.2006870767258854826 ) ) ;
#20902=DIRECTION ( 'NONE',  ( 1.000000000000000000, -0.000000000000000000, 0.000000000000000000 ) ) ;
#20903=ORIENTED_EDGE ( 'NONE', *, *, #37819, .F. ) ;
#20906=CIRCLE ( 'NONE', #13448, 5.000000000000000000 ) ;
#20907=CARTESIAN_POINT ( 'NONE',  ( 10.75853767213705048, 7.830989516993144051, 10.99661780661416088 ) ) ;
#20909=CARTESIAN_POINT ( 'NONE',  ( 18.66452593080030198, 6.623341608272929726, 11.78786073385051303 ) ) ;
#20910=EDGE_CURVE ( 'NONE', #31853, #32709, #22664, .T. ) ;
#20911=ORIENTED_EDGE ( 'NONE', *, *, #54866, .T. ) ;
#20914=CARTESIAN_POINT ( 'NONE',  ( 9.687175622948609899, 25.00000000000000000, -0.5854820436212360146 ) ) ;
#20919=ORIENTED_EDGE ( 'NONE', *, *, #17109, .T. ) ;
#20920=FACE_OUTER_BOUND ( 'NONE', #51884, .T. ) ;
#20921=ORIENTED_EDGE ( 'NONE', *, *, #49450, .T. ) ;
#20922=DIRECTION ( 'NONE',  ( -1.000000000000000000, 0.000000000000000000, 0.000000000000000000 ) ) ;
#20923=VERTEX_POINT ( 'NONE', #38822 ) ;
#20924=ADVANCED_FACE ( 'NONE', ( #39132 ), #33169, .T. ) ;
#20925=VERTEX_POINT ( 'NONE', #53799 ) ;
#20931=CARTESIAN_POINT ( 'NONE',  ( -35.00000000000000000, 1.903127969211188653, 11.59095880812009227 ) ) ;
#20933=CARTESIAN_POINT ( 'NONE',  ( -36.00000000000000711, -8.017674001891851532, 9.913596905230088296 ) ) ;
#20937=DIRECTION ( 'NONE',  ( 1.000000000000000000, 0.000000000000000000, 0.000000000000000000 ) ) ;
#20939=CARTESIAN_POINT ( 'NONE',  ( 37.00000000000000711, -1.113475361586579337, -12.70128625845192616 ) ) ;
#20940=LINE ( 'NONE', #62173, #64697 ) ;
#20942=EDGE_CURVE ( 'NONE', #24055, #54635, #21623, .T. ) ;
#20943=ORIENTED_EDGE ( 'NONE', *, *, #11869, .T. ) ;
#20944=DIRECTION ( 'NONE',  ( 1.000000000000000000, 0.000000000000000000, 0.000000000000000000 ) ) ;
#20945=ORIENTED_EDGE ( 'NONE', *, *, #54934, .F. ) ;
#20946=DIRECTION ( 'NONE',  ( 0.8405098440481681976, 0.000000000000000000, -0.5417962735734934698 ) ) ;
#20949=DIRECTION ( 'NONE',  ( -1.000000000000000000, 0.000000000000000000, -0.000000000000000000 ) ) ;
#20952=DIRECTION ( 'NONE',  ( 0.000000000000000000, 0.9718671068226452103, -0.2355298848897551256 ) ) ;
#20954=CARTESIAN_POINT ( 'NONE',  ( 24.48817448996944535, 8.566713351873016080, -8.406659586863929334 ) ) ;
#20955=CARTESIAN_POINT ( 'NONE',  ( 22.46687615433434004, -12.34696333092269604, -5.470250127934074946 ) ) ;
#20957=EDGE_CURVE ( 'NONE', #18937, #49613, #52382, .T. ) ;
#20963=DIRECTION ( 'NONE',  ( -1.000000000000000000, 0.000000000000000000, 0.000000000000000000 ) ) ;
#20964=LINE ( 'NONE', #32, #47145 ) ;
#20966=ORIENTED_EDGE ( 'NONE', *, *, #14335, .T. ) ;
#20967=EDGE_LOOP ( 'NONE', ( #32524, #61742, #49763, #49789 ) ) ;
#20968=CARTESIAN_POINT ( 'NONE',  ( 9.687175622948609899, 25.00000000000000000, -0.5854820436212360146 ) ) ;
#20969=CARTESIAN_POINT ( 'NONE',  ( 35.00000000000000000, -0.4353888892049205261, -11.73808581813437968 ) ) ;
#20970=DIRECTION ( 'NONE',  ( 0.000000000000000000, 0.01356324068817992175, -0.9999080150203990547 ) ) ;
#20971=DIRECTION ( 'NONE',  ( 1.000000000000000000, -0.000000000000000000, 0.000000000000000000 ) ) ;
#20972=VERTEX_POINT ( 'NONE', #34142 ) ;
#20973=ORIENTED_EDGE ( 'NONE', *, *, #51406, .T. ) ;
#20976=VECTOR ( 'NONE', #54564, 1000.000000000000000 ) ;
#20977=CARTESIAN_POINT ( 'NONE',  ( -35.00000000000000000, -10.64792938439751246, -5.927257550915431494 ) ) ;
#20978=ORIENTED_EDGE ( 'NONE', *, *, #53978, .T. ) ;
#20979=CARTESIAN_POINT ( 'NONE',  ( 12.10998784662220729, 25.00000000000000000, -8.526922110106905706 ) ) ;
#20981=EDGE_CURVE ( 'NONE', #15531, #60445, #20710, .T. ) ;
#20983=ORIENTED_EDGE ( 'NONE', *, *, #58785, .T. ) ;
#20986=CARTESIAN_POINT ( 'NONE',  ( -19.47984447937493613, -1.416020129149132334, 25.00000000000000000 ) ) ;
#20987=ORIENTED_EDGE ( 'NONE', *, *, #10181, .T. ) ;
#20988=DIRECTION ( 'NONE',  ( -1.000000000000000000, 0.000000000000000000, 0.000000000000000000 ) ) ;
#20989=VERTEX_POINT ( 'NONE', #49475 ) ;
#20991=ORIENTED_EDGE ( 'NONE', *, *, #21503, .T. ) ;
#20992=AXIS2_PLACEMENT_3D ( 'NONE', #7120, #1821, #36729 ) ;
#20996=CARTESIAN_POINT ( 'NONE',  ( 36.00000000000000711, 5.143145423404280159, -11.66664283989682005 ) ) ;
#20997=FACE_OUTER_BOUND ( 'NONE', #6805, .T. ) ;
#20998=CIRCLE ( 'NONE', #24187, 12.74999999999999822 ) ;
#20999=DIRECTION ( 'NONE',  ( 0.000000000000000000, 0.01356324068817998940, -0.9999080150203990547 ) ) ;
#21002=DIRECTION ( 'NONE',  ( 0.000000000000000000, 0.01356324068817998073, -0.9999080150203990547 ) ) ;
#21005=VERTEX_POINT ( 'NONE', #13848 ) ;
#21007=DIRECTION ( 'NONE',  ( -1.000000000000000000, -0.000000000000000000, 0.000000000000000000 ) ) ;
#21008=ADVANCED_FACE ( 'NONE', ( #9860 ), #49780, .T. ) ;
#21009=EDGE_CURVE ( 'NONE', #27444, #44984, #50450, .T. ) ;
#21010=ORIENTED_EDGE ( 'NONE', *, *, #3322, .F. ) ;
#21011=CARTESIAN_POINT ( 'NONE',  ( -35.00000000000000000, -8.534258022646161734, 8.699265615722952205 ) ) ;
#21012=CYLINDRICAL_SURFACE ( 'NONE', #30827, 12.18650000000000055 ) ;
#21014=DIRECTION ( 'NONE',  ( 1.000000000000000000, -0.000000000000000000, -0.000000000000000000 ) ) ;
#21015=EDGE_CURVE ( 'NONE', #18051, #1816, #31148, .T. ) ;
#21016=B_SPLINE_CURVE_WITH_KNOTS ( 'NONE', 3,
 ( #65293, #39359, #29387, #49682, #55315, #59328, #54984, #45339, #4127, #20073, #18775, #24081, #29702, #9108, #35351, #30042, #30376, #45664, #34688, #50010, #60303, #50356 ),
 .UNSPECIFIED., .F., .F.,
 ( 4, 2, 2, 2, 2, 2, 2, 2, 2, 2, 4 ),
 ( 3.297472175031376986E-18, 0.001351328940859378202, 0.002702657881718753367, 0.004053986822578128750, 0.004729651293007815574, 0.005405315763437503265, 0.006756644704296877781, 0.007432309174726568074, 0.008107973645156257500, 0.009459302586015634617, 0.01081063152687501000 ),
 .UNSPECIFIED. ) ;
#21018=ORIENTED_EDGE ( 'NONE', *, *, #3563, .F. ) ;
#21019=CARTESIAN_POINT ( 'NONE',  ( -17.25753826526994317, -6.483132040982834354, -10.09944016160721603 ) ) ;
#21020=B_SPLINE_CURVE_WITH_KNOTS ( 'NONE', 3,
 ( #11039, #1403, #36945, #52273, #5743, #6713, #22302, #26990, #47284, #1724, #21990, #12006, #62534, #37275, #27297, #47595 ),
 .UNSPECIFIED., .F., .F.,
 ( 4, 2, 2, 2, 2, 2, 2, 4 ),
 ( 1.636534854170084423E-17, 0.001750329107626847226, 0.002625493661440261080, 0.003500658215253675369, 0.004375822769067088357, 0.005250987322880503079, 0.006126151876693916067, 0.007001316430507330789 ),
 .UNSPECIFIED. ) ;
#21021=EDGE_LOOP ( 'NONE', ( #22491, #8387, #3736, #21018 ) ) ;
#21023=DIRECTION ( 'NONE',  ( 0.000000000000000000, 0.5987040770935622147, -0.8009703041134208501 ) ) ;
#21024=CARTESIAN_POINT ( 'NONE',  ( -35.00000000000000000, -1.771820996347237331, 11.61175578952785692 ) ) ;
#21025=VERTEX_POINT ( 'NONE', #24498 ) ;
#21027=EDGE_CURVE ( 'NONE', #2404, #38332, #48164, .T. ) ;
#21029=AXIS2_PLACEMENT_3D ( 'NONE', #40591, #60883, #61856 ) ;
#21032=DIRECTION ( 'NONE',  ( 1.000000000000000000, 0.000000000000000000, 0.000000000000000000 ) ) ;
#21035=CARTESIAN_POINT ( 'NONE',  ( -37.00000000000000711, 11.54110654723652196, -2.185196060783755279 ) ) ;
#21036=DIRECTION ( 'NONE',  ( -1.000000000000000000, 0.000000000000000000, -0.000000000000000000 ) ) ;
#21037=CARTESIAN_POINT ( 'NONE',  ( -37.00000000000000711, -3.307597835713158130, -12.31350058095526734 ) ) ;
#21039=EDGE_CURVE ( 'NONE', #14797, #58117, #32565, .T. ) ;
#21040=VERTEX_POINT ( 'NONE', #56760 ) ;
#21045=CARTESIAN_POINT ( 'NONE',  ( -35.00000000000000000, 0.000000000000000000, 0.000000000000000000 ) ) ;
#21049=DIRECTION ( 'NONE',  ( -1.000000000000000000, 0.000000000000000000, 0.000000000000000000 ) ) ;
#21050=ORIENTED_EDGE ( 'NONE', *, *, #16447, .T. ) ;
#21051=LINE ( 'NONE', #27681, #28537 ) ;
#21053=ORIENTED_EDGE ( 'NONE', *, *, #34613, .T. ) ;
#21055=CIRCLE ( 'NONE', #41378, 12.75000000000000178 ) ;
#21056=VERTEX_POINT ( 'NONE', #51758 ) ;
#21059=LINE ( 'NONE', #61624, #51399 ) ;
#21062=ORIENTED_EDGE ( 'NONE', *, *, #28999, .T. ) ;
#21065=CARTESIAN_POINT ( 'NONE',  ( 23.47699541227554931, -4.305096618431536015, -12.79908688602327516 ) ) ;
#21067=ORIENTED_EDGE ( 'NONE', *, *, #38814, .T. ) ;
#21068=ADVANCED_FACE ( 'NONE', ( #1211 ), #41093, .T. ) ;
#21070=ORIENTED_EDGE ( 'NONE', *, *, #23872, .T. ) ;
#21074=DIRECTION ( 'NONE',  ( 0.000000000000000000, 0.01356324068817992175, -0.9999080150203990547 ) ) ;
#21076=AXIS2_PLACEMENT_3D ( 'NONE', #36479, #56792, #11213 ) ;
#21078=ORIENTED_EDGE ( 'NONE', *, *, #53041, .T. ) ;
#21080=DIRECTION ( 'NONE',  ( 1.000000000000000000, 0.000000000000000000, 0.000000000000000000 ) ) ;
#21083=CARTESIAN_POINT ( 'NONE',  ( -17.83419946441818027, -9.720786832536937538, -9.367833439828872955 ) ) ;
#21084=ORIENTED_EDGE ( 'NONE', *, *, #19337, .T. ) ;
#21086=AXIS2_PLACEMENT_3D ( 'NONE', #9135, #39063, #48737 ) ;
#21091=EDGE_CURVE ( 'NONE', #48838, #14758, #15498, .T. ) ;
#21092=EDGE_CURVE ( 'NONE', #45790, #63543, #41770, .T. ) ;
#21095=FACE_OUTER_BOUND ( 'NONE', #38435, .T. ) ;
#21096=CIRCLE ( 'NONE', #60349, 12.18649999999999878 ) ;
#21098=DIRECTION ( 'NONE',  ( 0.000000000000000000, 0.9903235168508555120, 0.1387779952735781475 ) ) ;
#21100=DIRECTION ( 'NONE',  ( 1.000000000000000000, 0.000000000000000000, 0.000000000000000000 ) ) ;
#21101=CARTESIAN_POINT ( 'NONE',  ( -18.58686583997247155, 5.151216734910867068, -12.47858029384659417 ) ) ;
#21102=ORIENTED_EDGE ( 'NONE', *, *, #35185, .F. ) ;
#21103=CYLINDRICAL_SURFACE ( 'NONE', #62519, 1.750000000000000000 ) ;
#21105=CARTESIAN_POINT ( 'NONE',  ( -14.29135464769095520, 7.782112657557433089, -11.03126115115966854 ) ) ;
#21106=CIRCLE ( 'NONE', #902, 12.75000000000000178 ) ;
#21107=DIRECTION ( 'NONE',  ( 1.000000000000000000, 0.000000000000000000, 0.000000000000000000 ) ) ;
#21108=AXIS2_PLACEMENT_3D ( 'NONE', #20778, #15119, #46379 ) ;
#21110=CARTESIAN_POINT ( 'NONE',  ( -36.00000000000000711, 8.496612874013289129, -9.506317355798284296 ) ) ;
#21111=FACE_OUTER_BOUND ( 'NONE', #64013, .T. ) ;
#21112=ORIENTED_EDGE ( 'NONE', *, *, #64985, .F. ) ;
#21115=DIRECTION ( 'NONE',  ( 1.000000000000000000, 0.000000000000000000, 0.000000000000000000 ) ) ;
#21118=VECTOR ( 'NONE', #46781, 1000.000000000000000 ) ;
#21119=ADVANCED_FACE ( 'NONE', ( #61372 ), #37089, .T. ) ;
#21120=CARTESIAN_POINT ( 'NONE',  ( 9.634263811864652638, 2.206861042771444126, -13.32010880124498975 ) ) ;
#21121=CARTESIAN_POINT ( 'NONE',  ( 35.00000000000000000, 2.627174906297071733, 11.44858830469737221 ) ) ;
#21122=VECTOR ( 'NONE', #62572, 1000.000000000000000 ) ;
#21123=VERTEX_POINT ( 'NONE', #32096 ) ;
#21129=CARTESIAN_POINT ( 'NONE',  ( -18.08686583997219799, 5.369856758749883774, -10.73420889163467606 ) ) ;
#21130=DIRECTION ( 'NONE',  ( 1.000000000000000000, -0.000000000000000000, -0.000000000000000000 ) ) ;
#21132=DIRECTION ( 'NONE',  ( 0.000000000000000000, -0.01356324068817991828, 0.9999080150203990547 ) ) ;
#21135=ADVANCED_FACE ( 'NONE', ( #5892 ), #36448, .T. ) ;
#21136=CARTESIAN_POINT ( 'NONE',  ( -35.00000000000000000, -10.80631716521663854, -4.603882218679666849 ) ) ;
#21138=CARTESIAN_POINT ( 'NONE',  ( 0.1901047366177758269, -0.2738782441758274011, -11.99765584512894989 ) ) ;
#21139=CARTESIAN_POINT ( 'NONE',  ( 37.00000000000000711, -10.59380114696464581, 7.094637218249467026 ) ) ;
#21140=( BOUNDED_CURVE ( )  B_SPLINE_CURVE ( 3, ( #11764, #2480, #7785, #21438 ),
 .UNSPECIFIED., .F., .F. ) 
 B_SPLINE_CURVE_WITH_KNOTS ( ( 4, 4 ),
 ( 5.788101898619632202, 5.827247932393759378 ),
 .UNSPECIFIED. ) 
 CURVE ( )  GEOMETRIC_REPRESENTATION_ITEM ( )  RATIONAL_B_SPLINE_CURVE ( ( 1.000000000000000000, 0.9998723030801468514, 0.9998723030801468514, 1.000000000000000000 ) ) 
 REPRESENTATION_ITEM ( '' )  );
#21141=CARTESIAN_POINT ( 'NONE',  ( 23.12237510341146773, 2.549967125219239961, -11.72937603911085347 ) ) ;
#21144=CARTESIAN_POINT ( 'NONE',  ( -7.904596692198818886, 5.813930850916539050, -10.52491773401777486 ) ) ;
#21146=CARTESIAN_POINT ( 'NONE',  ( -17.29244623348158783, 2.525873743887551814, 13.26159725786978960 ) ) ;
#21148=EDGE_LOOP ( 'NONE', ( #41448, #48353, #61890, #27112 ) ) ;
#21149=ADVANCED_FACE ( 'NONE', ( #59045 ), #49072, .T. ) ;
#21152=ORIENTED_EDGE ( 'NONE', *, *, #6255, .T. ) ;
#21154=CARTESIAN_POINT ( 'NONE',  ( -2.672254813960873054, -12.91372982010632420, 3.936302266217765577 ) ) ;
#21155=DIRECTION ( 'NONE',  ( 0.000000000000000000, -0.01356324068817998940, 0.9999080150203990547 ) ) ;
#21157=ADVANCED_FACE ( 'NONE', ( #64005 ), #32426, .T. ) ;
#21158=CARTESIAN_POINT ( 'NONE',  ( -35.00000000000000000, 4.041347439435861943, 11.02904044024210428 ) ) ;
#21159=VERTEX_POINT ( 'NONE', #17483 ) ;
#21160=DIRECTION ( 'NONE',  ( -1.000000000000000000, 0.000000000000000000, 0.000000000000000000 ) ) ;
#21161=CARTESIAN_POINT ( 'NONE',  ( -24.46258210065891703, -7.197801736871879186, 9.604157314396443823 ) ) ;
#21164=FACE_BOUND ( 'NONE', #11571, .T. ) ;
#21166=VERTEX_POINT ( 'NONE', #58374 ) ;
#21167=EDGE_LOOP ( 'NONE', ( #40979, #59266, #53240, #12056 ) ) ;
#21170=CARTESIAN_POINT ( 'NONE',  ( 24.44987046108744266, -9.131562448621981076, -7.790012948628247003 ) ) ;
#21173=LINE ( 'NONE', #36477, #22045 ) ;
#21176=EDGE_CURVE ( 'NONE', #24505, #9287, #59880, .T. ) ;
#21178=AXIS2_PLACEMENT_3D ( 'NONE', #19599, #49537, #39862 ) ;
#21181=B_SPLINE_CURVE_WITH_KNOTS ( 'NONE', 3,
 ( #20737, #51341, #5792, #26059, #41007, #55974, #46338, #15719, #35995, #56295 ),
 .UNSPECIFIED., .F., .F.,
 ( 4, 2, 2, 2, 4 ),
 ( 8.673617379884035472E-18, 0.002186269455787307001, 0.004372538911574607064, 0.006558808367361907560, 0.008745077823149205454 ),
 .UNSPECIFIED. ) ;
#21182=CARTESIAN_POINT ( 'NONE',  ( -35.00000000000000000, 2.346765782874606465, -11.95840593935198903 ) ) ;
#21184=CARTESIAN_POINT ( 'NONE',  ( -9.318060253344532029, 10.62519452515019402, -5.580531082972568946 ) ) ;
#21185=DIRECTION ( 'NONE',  ( -1.000000000000000000, 0.000000000000000000, 0.000000000000000000 ) ) ;
#21186=LINE ( 'NONE', #62095, #17107 ) ;
#21187=CIRCLE ( 'NONE', #47729, 12.18650000000000055 ) ;
#21188=DIRECTION ( 'NONE',  ( -1.000000000000000000, -0.000000000000000000, -0.000000000000000000 ) ) ;
#21190=VERTEX_POINT ( 'NONE', #63339 ) ;
#21193=DIRECTION ( 'NONE',  ( 0.000000000000000000, 0.01356324068817998940, -0.9999080150203990547 ) ) ;
#21194=CARTESIAN_POINT ( 'NONE',  ( 37.00000000000000711, 12.21925492305367200, 3.640372113593418835 ) ) ;
#21198=DIRECTION ( 'NONE',  ( -1.000000000000000000, -0.000000000000000000, 0.000000000000000000 ) ) ;
#21200=DIRECTION ( 'NONE',  ( -1.000000000000000000, 0.000000000000000000, 0.000000000000000000 ) ) ;
#21202=EDGE_CURVE ( 'NONE', #6107, #46339, #1509, .T. ) ;
#21203=CIRCLE ( 'NONE', #58390, 12.75000000000000178 ) ;
#21205=DIRECTION ( 'NONE',  ( 0.000000000000000000, 0.01356324068817998940, -0.9999080150203989437 ) ) ;
#21206=ORIENTED_EDGE ( 'NONE', *, *, #39019, .T. ) ;
#21207=CIRCLE ( 'NONE', #25442, 4.999999999999999112 ) ;
#21208=LINE ( 'NONE', #16233, #12674 ) ;
#21209=VERTEX_POINT ( 'NONE', #48078 ) ;
#21210=CARTESIAN_POINT ( 'NONE',  ( 22.36482863261543486, -13.46837713145126791, -0.9234811557364140944 ) ) ;
#21211=CYLINDRICAL_SURFACE ( 'NONE', #31005, 5.000000000000000888 ) ;
#21212=DIRECTION ( 'NONE',  ( -1.000000000000000000, 0.000000000000000000, 0.000000000000000000 ) ) ;
#21213=CARTESIAN_POINT ( 'NONE',  ( 27.48158180005687612, -10.97080778372832199, 4.873343154589966808 ) ) ;
#21214=CARTESIAN_POINT ( 'NONE',  ( -7.194344000760931834, -1.897124946417909408, 11.84942057751005251 ) ) ;
#21216=EDGE_CURVE ( 'NONE', #53854, #26580, #43060, .T. ) ;
#21218=ORIENTED_EDGE ( 'NONE', *, *, #42958, .T. ) ;
#21220=ORIENTED_EDGE ( 'NONE', *, *, #64279, .T. ) ;
#21221=VECTOR ( 'NONE', #11404, 1000.000000000000000 ) ;
#21222=CARTESIAN_POINT ( 'NONE',  ( 37.00000000000000711, 1.030638227056565270, -12.14284015767850633 ) ) ;
#21223=CARTESIAN_POINT ( 'NONE',  ( 35.00000000000000000, 4.705694406421931860E-17, -3.469127814946512892E-15 ) ) ;
#21226=CARTESIAN_POINT ( 'NONE',  ( -47.00000000000000711, 0.000000000000000000, 0.000000000000000000 ) ) ;
#21228=DIRECTION ( 'NONE',  ( 0.000000000000000000, -1.000000000000000000, 0.000000000000000000 ) ) ;
#21229=CARTESIAN_POINT ( 'NONE',  ( 37.00000000000000711, -0.4871980014160605665, 12.74068829017554094 ) ) ;
#21230=VERTEX_POINT ( 'NONE', #8154 ) ;
#21231=EDGE_CURVE ( 'NONE', #63997, #40547, #47112, .T. ) ;
#21235=CARTESIAN_POINT ( 'NONE',  ( 35.00000000000000000, -2.968224442958486975, -11.81949347079746282 ) ) ;
#21236=DIRECTION ( 'NONE',  ( -1.000000000000000000, 0.000000000000000000, 0.000000000000000000 ) ) ;
#21241=FACE_OUTER_BOUND ( 'NONE', #64028, .T. ) ;
#21242=CARTESIAN_POINT ( 'NONE',  ( 36.00000000000000711, 3.805206332242470957, -12.16893194857551563 ) ) ;
#21245=ORIENTED_EDGE ( 'NONE', *, *, #7567, .F. ) ;
#21246=ORIENTED_EDGE ( 'NONE', *, *, #485, .F. ) ;
#21247=CARTESIAN_POINT ( 'NONE',  ( -35.00000000000000000, 1.039216533673073206, -11.70009620280410445 ) ) ;
#21248=EDGE_CURVE ( 'NONE', #52121, #39182, #53047, .T. ) ;
#21250=CARTESIAN_POINT ( 'NONE',  ( 37.00000000000000711, 11.17622378668006355, -3.614449339633533764 ) ) ;
#21252=ORIENTED_EDGE ( 'NONE', *, *, #32937, .T. ) ;
#21253=VERTEX_POINT ( 'NONE', #28424 ) ;
#21254=EDGE_CURVE ( 'NONE', #58567, #52575, #15238, .T. ) ;
#21256=CARTESIAN_POINT ( 'NONE',  ( 35.00000000000000000, -10.32377448871663006, 6.475373545682407972 ) ) ;
#21257=CIRCLE ( 'NONE', #56282, 12.75000000000000178 ) ;
#21259=AXIS2_PLACEMENT_3D ( 'NONE', #6166, #26428, #23332 ) ;
#21260=LINE ( 'NONE', #62161, #4361 ) ;
#21261=CARTESIAN_POINT ( 'NONE',  ( -35.00000000000000000, 6.753013023069858178, -10.14433819232427147 ) ) ;
#21263=ADVANCED_FACE ( 'NONE', ( #38744 ), #8475, .T. ) ;
#21264=LINE ( 'NONE', #41538, #39645 ) ;
#21265=ORIENTED_EDGE ( 'NONE', *, *, #9356, .T. ) ;
#21268=ADVANCED_FACE ( 'NONE', ( #4494 ), #45358, .T. ) ;
#21270=DIRECTION ( 'NONE',  ( -1.000000000000000000, -0.000000000000000000, -0.000000000000000000 ) ) ;
#21273=CIRCLE ( 'NONE', #37160, 12.18649999999999878 ) ;
#21274=ORIENTED_EDGE ( 'NONE', *, *, #14531, .T. ) ;
#21276=CIRCLE ( 'NONE', #42466, 5.000000000000001776 ) ;
#21280=DIRECTION ( 'NONE',  ( 1.000000000000000000, -0.000000000000000000, 0.000000000000000000 ) ) ;
#21283=VERTEX_POINT ( 'NONE', #64639 ) ;
#21284=DIRECTION ( 'NONE',  ( 0.000000000000000000, 0.01356324068817992175, -0.9999080150203990547 ) ) ;
#21285=DIRECTION ( 'NONE',  ( -1.000000000000000000, 0.000000000000000000, 0.000000000000000000 ) ) ;
#21286=AXIS2_PLACEMENT_3D ( 'NONE', #32291, #57921, #20999 ) ;
#21290=EDGE_CURVE ( 'NONE', #27894, #23892, #55601, .T. ) ;
#21291=AXIS2_PLACEMENT_3D ( 'NONE', #5910, #11512, #62070 ) ;
#21294=CIRCLE ( 'NONE', #6452, 4.999999999999999112 ) ;
#21296=DIRECTION ( 'NONE',  ( 0.000000000000000000, 0.01356324068817992175, -0.9999080150203990547 ) ) ;
#21298=ADVANCED_FACE ( 'NONE', ( #18796 ), #19112, .T. ) ;
#21299=AXIS2_PLACEMENT_3D ( 'NONE', #44503, #38891, #9931 ) ;
#21300=AXIS2_PLACEMENT_3D ( 'NONE', #41893, #56548, #10989 ) ;
#21301=CIRCLE ( 'NONE', #44644, 12.75000000000000178 ) ;
#21308=CARTESIAN_POINT ( 'NONE',  ( -35.00000000000000000, -5.300372733891723698, 11.59605747147784882 ) ) ;
#21309=ORIENTED_EDGE ( 'NONE', *, *, #1365, .T. ) ;
#21310=ADVANCED_FACE ( 'NONE', ( #20093 ), #54381, .T. ) ;
#21314=VECTOR ( 'NONE', #6785, 1000.000000000000000 ) ;
#21315=VECTOR ( 'NONE', #52919, 1000.000000000000000 ) ;
#21316=ORIENTED_EDGE ( 'NONE', *, *, #17573, .F. ) ;
#21317=CARTESIAN_POINT ( 'NONE',  ( -17.16690145660755817, 3.059820691759368660, -11.60420365748035643 ) ) ;
#21318=AXIS2_PLACEMENT_3D ( 'NONE', #60052, #19491, #9819 ) ;
#21319=CIRCLE ( 'NONE', #35108, 5.000000000000000000 ) ;
#21320=LINE ( 'NONE', #61889, #4541 ) ;
#21321=ORIENTED_EDGE ( 'NONE', *, *, #4211, .F. ) ;
#21322=CYLINDRICAL_SURFACE ( 'NONE', #43882, 4.999999999999999112 ) ;
#21325=ORIENTED_EDGE ( 'NONE', *, *, #57047, .T. ) ;
#21326=AXIS2_PLACEMENT_3D ( 'NONE', #59310, #19739, #9734 ) ;
#21327=DIRECTION ( 'NONE',  ( -1.000000000000000000, 0.000000000000000000, 0.000000000000000000 ) ) ;
#21328=ORIENTED_EDGE ( 'NONE', *, *, #47322, .F. ) ;
#21331=CARTESIAN_POINT ( 'NONE',  ( -35.00000000000000000, -6.584150480049623333, 10.25474254703950905 ) ) ;
#21332=EDGE_CURVE ( 'NONE', #8491, #45959, #50348, .T. ) ;
#21334=CYLINDRICAL_SURFACE ( 'NONE', #17748, 4.999999999999999112 ) ;
#21335=DIRECTION ( 'NONE',  ( -1.000000000000000000, 0.000000000000000000, 0.000000000000000000 ) ) ;
#21336=DIRECTION ( 'NONE',  ( 0.000000000000000000, -0.01356324068817991828, 0.9999080150203990547 ) ) ;
#21339=CARTESIAN_POINT ( 'NONE',  ( -18.00928138223606467, 3.265590404870133412, -13.10068440056983796 ) ) ;
#21340=ORIENTED_EDGE ( 'NONE', *, *, #5818, .T. ) ;
#21343=CIRCLE ( 'NONE', #54301, 12.75000000000000178 ) ;
#21346=LINE ( 'NONE', #748, #37557 ) ;
#21348=AXIS2_PLACEMENT_3D ( 'NONE', #47084, #21818, #46737 ) ;
#21350=CARTESIAN_POINT ( 'NONE',  ( 37.00000000000000711, 10.80631716521673447, 4.603882218679430594 ) ) ;
#21354=FACE_OUTER_BOUND ( 'NONE', #43551, .T. ) ;
#21355=AXIS2_PLACEMENT_3D ( 'NONE', #13756, #54990, #54361 ) ;
#21356=CIRCLE ( 'NONE', #8586, 14.99999999999998757 ) ;
#21357=ORIENTED_EDGE ( 'NONE', *, *, #28011, .F. ) ;
#21358=CARTESIAN_POINT ( 'NONE',  ( -17.57571841026333459, -9.333537370853115078, -7.571081700497278355 ) ) ;
#21360=AXIS2_PLACEMENT_3D ( 'NONE', #42671, #18088, #18755 ) ;
#21361=VERTEX_POINT ( 'NONE', #4823 ) ;
#21362=FACE_OUTER_BOUND ( 'NONE', #62275, .T. ) ;
#21364=PLANE ( 'NONE',  #10545 ) ;
#21365=ORIENTED_EDGE ( 'NONE', *, *, #8664, .T. ) ;
#21366=CARTESIAN_POINT ( 'NONE',  ( -35.00000000000000000, -6.102719229070750373, 10.54834585426218041 ) ) ;
#21367=AXIS2_PLACEMENT_3D ( 'NONE', #61388, #10518, #11831 ) ;
#21369=EDGE_CURVE ( 'NONE', #27612, #48877, #52432, .T. ) ;
#21370=CIRCLE ( 'NONE', #17104, 12.18650000000000411 ) ;
#21372=CARTESIAN_POINT ( 'NONE',  ( -35.00000000000000000, 8.699265615722982403, 8.534258022646129760 ) ) ;
#21373=DIRECTION ( 'NONE',  ( 0.000000000000000000, -0.01356324068817992175, 0.9999080150203990547 ) ) ;
#21374=AXIS2_PLACEMENT_3D ( 'NONE', #17155, #17492, #30875 ) ;
#21375=CARTESIAN_POINT ( 'NONE',  ( -35.00000000000000000, 11.96656215839369075, 4.400442035670987018 ) ) ;
#21376=DIRECTION ( 'NONE',  ( -0.000000000000000000, -0.000000000000000000, -1.000000000000000000 ) ) ;
#21377=FACE_OUTER_BOUND ( 'NONE', #4965, .T. ) ;
#21378=CYLINDRICAL_SURFACE ( 'NONE', #36774, 12.74999999999999822 ) ;
#21379=CARTESIAN_POINT ( 'NONE',  ( -17.83419946441818027, -9.720786832536937538, -7.036071585506806336 ) ) ;
#21380=AXIS2_PLACEMENT_3D ( 'NONE', #12836, #42761, #47770 ) ;
#21382=ORIENTED_EDGE ( 'NONE', *, *, #64985, .T. ) ;
#21386=EDGE_LOOP ( 'NONE', ( #35555, #3657, #7073, #14119 ) ) ;
#21389=CARTESIAN_POINT ( 'NONE',  ( 9.586060201835508110, 6.684527016188011039, -9.971514917006311762 ) ) ;
#21390=ORIENTED_EDGE ( 'NONE', *, *, #55111, .T. ) ;
#21391=AXIS2_PLACEMENT_3D ( 'NONE', #3779, #39306, #24343 ) ;
#21392=CARTESIAN_POINT ( 'NONE',  ( 26.17141335727527007, -13.01134923558396572, 3.602278675730974378 ) ) ;
#21394=ORIENTED_EDGE ( 'NONE', *, *, #46981, .F. ) ;
#21395=ADVANCED_FACE ( 'NONE', ( #4152 ), #24416, .T. ) ;
#21397=DIRECTION ( 'NONE',  ( 0.000000000000000000, -0.01356324068817991828, 0.9999080150203990547 ) ) ;
#21398=VERTEX_POINT ( 'NONE', #51684 ) ;
#21400=EDGE_CURVE ( 'NONE', #17474, #52157, #43922, .T. ) ;
#21404=ORIENTED_EDGE ( 'NONE', *, *, #4374, .T. ) ;
#21405=DIRECTION ( 'NONE',  ( 0.000000000000000000, -0.01356324068817991828, 0.9999080150203990547 ) ) ;
#21407=CARTESIAN_POINT ( 'NONE',  ( -35.00000000000000000, 0.000000000000000000, 0.000000000000000000 ) ) ;
#21410=CARTESIAN_POINT ( 'NONE',  ( 34.38695973621796043, 25.00000000000000000, 3.530690241644829364 ) ) ;
#21415=DIRECTION ( 'NONE',  ( 1.000000000000000000, 0.000000000000000000, -0.000000000000000000 ) ) ;
#21416=VERTEX_POINT ( 'NONE', #56674 ) ;
#21417=DIRECTION ( 'NONE',  ( 1.000000000000000000, 0.000000000000000000, 0.000000000000000000 ) ) ;
#21419=CARTESIAN_POINT ( 'NONE',  ( 35.00000000000000000, 11.86701198550355940, -2.772148766916162188 ) ) ;
#21420=AXIS2_PLACEMENT_3D ( 'NONE', #49424, #19471, #24783 ) ;
#21421=FACE_OUTER_BOUND ( 'NONE', #55018, .T. ) ;
#21423=CARTESIAN_POINT ( 'NONE',  ( -35.00000000000000000, 0.7214809346828596759, 11.72397916322012712 ) ) ;
#21424=CIRCLE ( 'NONE', #58611, 12.18649999999999878 ) ;
#21428=DIRECTION ( 'NONE',  ( 1.000000000000000000, 0.000000000000000000, 0.000000000000000000 ) ) ;
#21429=AXIS2_PLACEMENT_3D ( 'NONE', #33481, #37807, #58102 ) ;
#21431=EDGE_CURVE ( 'NONE', #37186, #3067, #8883, .T. ) ;
#21435=AXIS2_PLACEMENT_3D ( 'NONE', #19787, #40709, #9786 ) ;
#21437=CIRCLE ( 'NONE', #50107, 12.75000000000000178 ) ;
#21438=CARTESIAN_POINT ( 'NONE',  ( 18.84867683979356201, -5.944105725974474730, 12.12095735156416509 ) ) ;
#21440=DIRECTION ( 'NONE',  ( 0.000000000000000000, 0.9970832820307037325, 0.07632122047556839928 ) ) ;
#21443=CARTESIAN_POINT ( 'NONE',  ( 37.00000000000000711, 9.076753354953998709, -8.954052073409638268 ) ) ;
#21444=CARTESIAN_POINT ( 'NONE',  ( -6.754644257020094855, -1.192176639353738521, -11.94107717247141132 ) ) ;
#21445=CARTESIAN_POINT ( 'NONE',  ( 47.00000000000000711, 4.705694406421931860E-17, -3.469127814946512892E-15 ) ) ;
#21446=VECTOR ( 'NONE', #24444, 1000.000000000000000 ) ;
#21448=CYLINDRICAL_SURFACE ( 'NONE', #33864, 4.999999999999999112 ) ;
#21451=CIRCLE ( 'NONE', #39474, 5.000000000000000888 ) ;
#21452=CARTESIAN_POINT ( 'NONE',  ( 12.49336350054390365, 0.1658493928153577657, -11.99999999999999645 ) ) ;
#21455=EDGE_CURVE ( 'NONE', #15413, #2234, #41340, .T. ) ;
#21457=CARTESIAN_POINT ( 'NONE',  ( 3.062197852306406620, 2.793213809110397516, -11.67210648529468564 ) ) ;
#21461=CARTESIAN_POINT ( 'NONE',  ( -35.00000000000000000, 0.000000000000000000, 0.000000000000000000 ) ) ;
#21462=DIRECTION ( 'NONE',  ( -1.000000000000000000, 0.000000000000000000, 0.000000000000000000 ) ) ;
#21464=CIRCLE ( 'NONE', #29957, 5.000000000000000888 ) ;
#21466=EDGE_CURVE ( 'NONE', #55606, #26984, #41022, .T. ) ;
#21469=DIRECTION ( 'NONE',  ( 0.000000000000000000, 0.9651210252299785575, 0.2618041379715665973 ) ) ;
#21470=VERTEX_POINT ( 'NONE', #26722 ) ;
#21472=DIRECTION ( 'NONE',  ( -1.000000000000000000, 0.000000000000000000, 0.000000000000000000 ) ) ;
#21474=CARTESIAN_POINT ( 'NONE',  ( -37.00000000000000711, -3.473736367725171359, -12.26766708251995475 ) ) ;
#21475=ORIENTED_EDGE ( 'NONE', *, *, #20768, .F. ) ;
#21477=CARTESIAN_POINT ( 'NONE',  ( -37.00000000000000711, -10.68873102412847764, 6.950793414699757200 ) ) ;
#21479=EDGE_CURVE ( 'NONE', #34180, #25983, #31050, .T. ) ;
#21480=DIRECTION ( 'NONE',  ( 0.000000000000000000, 0.01356324068817992175, -0.9999080150203990547 ) ) ;
#21482=CYLINDRICAL_SURFACE ( 'NONE', #54357, 12.18650000000000055 ) ;
#21483=EDGE_CURVE ( 'NONE', #9921, #14030, #21059, .T. ) ;
#21486=DIRECTION ( 'NONE',  ( -1.000000000000000000, -0.000000000000000000, 0.000000000000000000 ) ) ;
#21487=ORIENTED_EDGE ( 'NONE', *, *, #62040, .F. ) ;
#21489=AXIS2_PLACEMENT_3D ( 'NONE', #5595, #36128, #599 ) ;
#21490=CARTESIAN_POINT ( 'NONE',  ( 35.00000000000000000, 4.705694406421931860E-17, -3.469127814946512892E-15 ) ) ;
#21491=CARTESIAN_POINT ( 'NONE',  ( 47.00000000000000711, 4.705694406421931860E-17, -3.469127814946512892E-15 ) ) ;
#21493=CARTESIAN_POINT ( 'NONE',  ( -18.25006854224444908, -9.443202773001939221, 9.647586298549914119 ) ) ;
#21495=DIRECTION ( 'NONE',  ( -1.000000000000000000, -0.000000000000000000, 0.000000000000000000 ) ) ;
#21496=ORIENTED_EDGE ( 'NONE', *, *, #40975, .T. ) ;
#21497=EDGE_LOOP ( 'NONE', ( #64630, #27000, #10419, #55942 ) ) ;
#21498=CARTESIAN_POINT ( 'NONE',  ( 23.98530306424479619, 2.278180183290474226, -11.78598886095566911 ) ) ;
#21503=EDGE_CURVE ( 'NONE', #11696, #1074, #16079, .T. ) ;
#21504=AXIS2_PLACEMENT_3D ( 'NONE', #64970, #34397, #64323 ) ;
#21507=DIRECTION ( 'NONE',  ( -1.000000000000000000, 0.000000000000000000, 0.000000000000000000 ) ) ;
#21508=ORIENTED_EDGE ( 'NONE', *, *, #30185, .T. ) ;
#21509=CARTESIAN_POINT ( 'NONE',  ( -47.00000000000000711, 0.000000000000000000, 0.000000000000000000 ) ) ;
#21510=DIRECTION ( 'NONE',  ( -1.000000000000000000, -0.000000000000000000, 0.000000000000000000 ) ) ;
#21512=VERTEX_POINT ( 'NONE', #42001 ) ;
#21513=ORIENTED_EDGE ( 'NONE', *, *, #47986, .T. ) ;
#21514=DIRECTION ( 'NONE',  ( 0.3902440745007897949, -0.000000000000000000, 0.9207114435679737419 ) ) ;
#21515=ORIENTED_EDGE ( 'NONE', *, *, #23033, .T. ) ;
#21516=CARTESIAN_POINT ( 'NONE',  ( 22.22080425544861981, -11.93711206880059450, -1.277188082013731574 ) ) ;
#21518=AXIS2_PLACEMENT_3D ( 'NONE', #19541, #14511, #18580 ) ;
#21519=DIRECTION ( 'NONE',  ( -1.000000000000000000, -0.000000000000000000, -0.000000000000000000 ) ) ;
#21521=EDGE_CURVE ( 'NONE', #10081, #49489, #15736, .T. ) ;
#21525=CYLINDRICAL_SURFACE ( 'NONE', #28029, 4.999999999999999112 ) ;
#21526=ORIENTED_EDGE ( 'NONE', *, *, #48071, .F. ) ;
#21527=AXIS2_PLACEMENT_3D ( 'NONE', #16663, #36280, #36934 ) ;
#21531=FACE_OUTER_BOUND ( 'NONE', #2589, .T. ) ;
#21533=FACE_OUTER_BOUND ( 'NONE', #60669, .T. ) ;
#21534=CARTESIAN_POINT ( 'NONE',  ( -35.00000000000000000, -10.01317267707891467, 6.946017217729903770 ) ) ;
#21538=VERTEX_POINT ( 'NONE', #51362 ) ;
#21539=CARTESIAN_POINT ( 'NONE',  ( -36.00000000000000711, -12.71517666308948691, 0.9416912585473986574 ) ) ;
#21542=EDGE_LOOP ( 'NONE', ( #56274, #61551, #50523, #6710 ) ) ;
#21543=CARTESIAN_POINT ( 'NONE',  ( 36.00000000000000711, 11.39945968423471534, -5.710938531231754212 ) ) ;
#21544=FACE_OUTER_BOUND ( 'NONE', #24194, .T. ) ;
#21546=ADVANCED_FACE ( 'NONE', ( #16427 ), #46032, .T. ) ;
#21548=ORIENTED_EDGE ( 'NONE', *, *, #64347, .T. ) ;
#21551=AXIS2_PLACEMENT_3D ( 'NONE', #35854, #10597, #5649 ) ;
#21553=DIRECTION ( 'NONE',  ( 0.000000000000000000, -0.01356324068817991828, 0.9999080150203990547 ) ) ;
#21554=AXIS2_PLACEMENT_3D ( 'NONE', #34111, #23507, #43784 ) ;
#21555=EDGE_CURVE ( 'NONE', #2528, #47268, #41822, .T. ) ;
#21557=LINE ( 'NONE', #16565, #1245 ) ;
#21559=( BOUNDED_CURVE ( )  B_SPLINE_CURVE ( 3, ( #24534, #10535, #65409, #19877 ),
 .UNSPECIFIED., .F., .F. ) 
 B_SPLINE_CURVE_WITH_KNOTS ( ( 4, 4 ),
 ( 4.054895942073102333, 4.098008028811909398 ),
 .UNSPECIFIED. ) 
 CURVE ( )  GEOMETRIC_REPRESENTATION_ITEM ( )  RATIONAL_B_SPLINE_CURVE ( ( 1.000000000000000000, 0.9998451183288734612, 0.9998451183288734612, 1.000000000000000000 ) ) 
 REPRESENTATION_ITEM ( '' )  );
#21560=ORIENTED_EDGE ( 'NONE', *, *, #6676, .F. ) ;
#21563=CARTESIAN_POINT ( 'NONE',  ( 37.00000000000000711, 4.705694406421931860E-17, -3.469127814946512892E-15 ) ) ;
#21564=CARTESIAN_POINT ( 'NONE',  ( -35.00000000000000000, 4.986700593229701717, 10.63508530065523772 ) ) ;
#21565=DIRECTION ( 'NONE',  ( 1.000000000000000000, 0.000000000000000000, 0.000000000000000000 ) ) ;
#21566=EDGE_CURVE ( 'NONE', #44, #61612, #42866, .T. ) ;
#21568=CYLINDRICAL_SURFACE ( 'NONE', #64680, 12.18650000000000055 ) ;
#21571=AXIS2_PLACEMENT_3D ( 'NONE', #14189, #60083, #20168 ) ;
#21573=VERTEX_POINT ( 'NONE', #6442 ) ;
#21574=CARTESIAN_POINT ( 'NONE',  ( -35.00000000000000000, -5.391785509270885512, -10.43555801961481677 ) ) ;
#21575=ADVANCED_FACE ( 'NONE', ( #47015 ), #1472, .T. ) ;
#21577=DIRECTION ( 'NONE',  ( -0.000000000000000000, -1.000000000000000000, -0.000000000000000000 ) ) ;
#21578=DIRECTION ( 'NONE',  ( 1.000000000000000000, 0.000000000000000000, 0.000000000000000000 ) ) ;
#21579=CARTESIAN_POINT ( 'NONE',  ( -35.00000000000000000, -1.456211999474261054, -11.65554240571058742 ) ) ;
#21580=CARTESIAN_POINT ( 'NONE',  ( -37.00000000000000711, -4.561791185930498926, 11.90598845858532329 ) ) ;
#21582=AXIS2_PLACEMENT_3D ( 'NONE', #17349, #51947, #57257 ) ;
#21583=CARTESIAN_POINT ( 'NONE',  ( -9.857392862911050102, -3.262500639785465673, 11.54921333413416207 ) ) ;
#21584=ORIENTED_EDGE ( 'NONE', *, *, #5938, .F. ) ;
#21586=ORIENTED_EDGE ( 'NONE', *, *, #35984, .T. ) ;
#21587=( NAMED_UNIT ( * ) SI_UNIT ( $, .STERADIAN. ) SOLID_ANGLE_UNIT ( ) );
#21588=CYLINDRICAL_SURFACE ( 'NONE', #24886, 12.75000000000000178 ) ;
#21589=LINE ( 'NONE', #6947, #52367 ) ;
#21590=CARTESIAN_POINT ( 'NONE',  ( -47.00000000000000711, 0.000000000000000000, 0.000000000000000000 ) ) ;
#21591=ORIENTED_EDGE ( 'NONE', *, *, #54505, .T. ) ;
#21594=CARTESIAN_POINT ( 'NONE',  ( 17.27839441901508621, 25.00000000000000000, 5.771933972472480967 ) ) ;
#21595=EDGE_LOOP ( 'NONE', ( #58634, #65078, #52655, #28975 ) ) ;
#21596=VERTEX_POINT ( 'NONE', #13385 ) ;
#21597=CARTESIAN_POINT ( 'NONE',  ( -17.29244623348158783, 2.525873743887551814, -11.73115347397429176 ) ) ;
#21598=ORIENTED_EDGE ( 'NONE', *, *, #31909, .F. ) ;
#21600=VERTEX_POINT ( 'NONE', #57979 ) ;
#21601=AXIS2_PLACEMENT_3D ( 'NONE', #12972, #27597, #13304 ) ;
#21603=ORIENTED_EDGE ( 'NONE', *, *, #23268, .T. ) ;
#21606=AXIS2_PLACEMENT_3D ( 'NONE', #2512, #32711, #42698 ) ;
#21607=EDGE_CURVE ( 'NONE', #40174, #43224, #28022, .T. ) ;
#21608=CIRCLE ( 'NONE', #33161, 12.18649999999999700 ) ;
#21609=DIRECTION ( 'NONE',  ( 1.000000000000000000, 0.000000000000000000, 0.000000000000000000 ) ) ;
#21611=DIRECTION ( 'NONE',  ( 0.000000000000000000, 0.9651210252299803338, 0.2618041379715599914 ) ) ;
#21612=ORIENTED_EDGE ( 'NONE', *, *, #45998, .F. ) ;
#21613=CARTESIAN_POINT ( 'NONE',  ( -37.00000000000000711, 3.307597835713245171, 12.31350058095524425 ) ) ;
#21614=ORIENTED_EDGE ( 'NONE', *, *, #1469, .T. ) ;
#21615=DIRECTION ( 'NONE',  ( -1.000000000000000000, -1.836970198721029688E-16, -0.000000000000000000 ) ) ;
#21617=CARTESIAN_POINT ( 'NONE',  ( -2.897877849616106172, 12.67799309120630724, 4.651592531936545427 ) ) ;
#21620=AXIS2_PLACEMENT_3D ( 'NONE', #58872, #13288, #3328 ) ;
#21623=CIRCLE ( 'NONE', #46010, 15.00000000000000000 ) ;
#21624=EDGE_CURVE ( 'NONE', #8899, #35815, #13067, .T. ) ;
#21629=EDGE_CURVE ( 'NONE', #49500, #19944, #53531, .T. ) ;
#21630=CARTESIAN_POINT ( 'NONE',  ( -35.00000000000000000, 8.052525312710004712, -8.551552972816995890 ) ) ;
#21634=EDGE_CURVE ( 'NONE', #56480, #36936, #3523, .T. ) ;
#21636=ORIENTED_EDGE ( 'NONE', *, *, #48794, .F. ) ;
#21638=DIRECTION ( 'NONE',  ( 0.000000000000000000, -0.01356324068817992001, 0.9999080150203990547 ) ) ;
#21641=VECTOR ( 'NONE', #26561, 1000.000000000000000 ) ;
#21642=EDGE_CURVE ( 'NONE', #14797, #36936, #12718, .T. ) ;
#21643=CARTESIAN_POINT ( 'NONE',  ( -20.79170840334646542, 12.91784323155722980, -3.921648409140116698 ) ) ;
#21644=ADVANCED_FACE ( 'NONE', ( #32659 ), #7758, .T. ) ;
#21645=CARTESIAN_POINT ( 'NONE',  ( 36.00000000000000711, 12.46157735505189201, -2.696588552979105380 ) ) ;
#21646=CYLINDRICAL_SURFACE ( 'NONE', #10781, 4.999999999999998224 ) ;
#21647=CARTESIAN_POINT ( 'NONE',  ( -35.00000000000000000, -6.018036132182240650, 11.24036214326518213 ) ) ;
#21648=DIRECTION ( 'NONE',  ( 0.000000000000000000, -0.01356324068817998940, 0.9999080150203990547 ) ) ;
#21650=EDGE_CURVE ( 'NONE', #25546, #14551, #62009, .T. ) ;
#21651=AXIS2_PLACEMENT_3D ( 'NONE', #20151, #20487, #61054 ) ;
#21653=ORIENTED_EDGE ( 'NONE', *, *, #13976, .F. ) ;
#21657=AXIS2_PLACEMENT_3D ( 'NONE', #39117, #50100, #13515 ) ;
#21659=FACE_OUTER_BOUND ( 'NONE', #47040, .T. ) ;
#21660=VECTOR ( 'NONE', #47543, 1000.000000000000000 ) ;
#21664=AXIS2_PLACEMENT_3D ( 'NONE', #11469, #56041, #1184 ) ;
#21665=ORIENTED_EDGE ( 'NONE', *, *, #38401, .F. ) ;
#21666=VERTEX_POINT ( 'NONE', #53314 ) ;
#21667=CARTESIAN_POINT ( 'NONE',  ( 37.00000000000000711, -10.28547182238011715, -5.672855678558653914 ) ) ;
#21669=FACE_OUTER_BOUND ( 'NONE', #29937, .T. ) ;
#21670=EDGE_LOOP ( 'NONE', ( #34068, #36558, #1018, #24199 ) ) ;
#21672=CARTESIAN_POINT ( 'NONE',  ( -37.00000000000000711, 0.000000000000000000, 0.000000000000000000 ) ) ;
#21673=ORIENTED_EDGE ( 'NONE', *, *, #44023, .F. ) ;
#21674=CARTESIAN_POINT ( 'NONE',  ( 37.00000000000000711, -2.346765782874354667, 11.95840593935203522 ) ) ;
#21675=AXIS2_PLACEMENT_3D ( 'NONE', #45389, #20126, #9812 ) ;
#21678=EDGE_LOOP ( 'NONE', ( #41438, #37417, #50484, #46817 ) ) ;
#21680=ORIENTED_EDGE ( 'NONE', *, *, #9327, .F. ) ;
#21682=DIRECTION ( 'NONE',  ( 0.000000000000000000, 0.01356324068817992175, -0.9999080150203990547 ) ) ;
#21684=DIRECTION ( 'NONE',  ( -1.000000000000000000, -0.000000000000000000, 0.000000000000000000 ) ) ;
#21685=EDGE_CURVE ( 'NONE', #20070, #57232, #28041, .T. ) ;
#21686=FACE_OUTER_BOUND ( 'NONE', #13009, .T. ) ;
#21688=CARTESIAN_POINT ( 'NONE',  ( 37.00000000000000711, 0.4353888892050056802, 11.73808581813437080 ) ) ;
#21691=DIRECTION ( 'NONE',  ( -0.000000000000000000, -1.000000000000000000, -0.000000000000000000 ) ) ;
#21694=CARTESIAN_POINT ( 'NONE',  ( -25.54417658651491863, -4.240019242199836391, 11.22596262356930197 ) ) ;
#21696=ORIENTED_EDGE ( 'NONE', *, *, #29620, .F. ) ;
#21697=ADVANCED_FACE ( 'NONE', ( #42639 ), #42307, .T. ) ;
#21698=CYLINDRICAL_SURFACE ( 'NONE', #59383, 4.999999999999999112 ) ;
#21699=VECTOR ( 'NONE', #15673, 1000.000000000000000 ) ;
#21700=DIRECTION ( 'NONE',  ( -0.000000000000000000, -1.000000000000000000, -0.000000000000000000 ) ) ;
#21701=FACE_OUTER_BOUND ( 'NONE', #62817, .T. ) ;
#21703=VERTEX_POINT ( 'NONE', #12071 ) ;
#21706=ORIENTED_EDGE ( 'NONE', *, *, #59582, .T. ) ;
#21707=DIRECTION ( 'NONE',  ( -1.000000000000000000, 0.000000000000000000, -0.000000000000000000 ) ) ;
#21708=VECTOR ( 'NONE', #3224, 1000.000000000000000 ) ;
#21709=ORIENTED_EDGE ( 'NONE', *, *, #58200, .T. ) ;
#21710=FACE_OUTER_BOUND ( 'NONE', #22073, .T. ) ;
#21711=CARTESIAN_POINT ( 'NONE',  ( 35.00000000000000000, -4.237174932027311769, -12.02534193257719508 ) ) ;
#21712=LINE ( 'NONE', #31346, #39220 ) ;
#21713=EDGE_CURVE ( 'NONE', #49092, #19473, #38670, .T. ) ;
#21715=AXIS2_PLACEMENT_3D ( 'NONE', #57688, #57029, #46707 ) ;
#21718=CARTESIAN_POINT ( 'NONE',  ( 28.81837816810347519, 11.51969343814563551, 7.050593228646411248 ) ) ;
#21719=DIRECTION ( 'NONE',  ( 0.000000000000000000, -0.01356324068817998940, 0.9999080150203990547 ) ) ;
#21721=ADVANCED_FACE ( 'NONE', ( #48653 ), #38322, .T. ) ;
#21722=DIRECTION ( 'NONE',  ( 0.000000000000000000, -0.01356324068817998940, 0.9999080150203990547 ) ) ;
#21723=LINE ( 'NONE', #38294, #54034 ) ;
#21728=EDGE_CURVE ( 'NONE', #14627, #41918, #26972, .T. ) ;
#21729=CIRCLE ( 'NONE', #1566, 12.18650000000000411 ) ;
#21730=VERTEX_POINT ( 'NONE', #64257 ) ;
#21731=EDGE_CURVE ( 'NONE', #4063, #33705, #60965, .T. ) ;
#21734=VERTEX_POINT ( 'NONE', #650 ) ;
#21736=CARTESIAN_POINT ( 'NONE',  ( 35.00000000000000000, 4.705694406421931860E-17, -3.469127814946512892E-15 ) ) ;
#21737=ORIENTED_EDGE ( 'NONE', *, *, #38279, .T. ) ;
#21739=CARTESIAN_POINT ( 'NONE',  ( -37.00000000000000711, -0.4993900848166508144, -12.17626345777664554 ) ) ;
#21740=VERTEX_POINT ( 'NONE', #53961 ) ;
#21741=VECTOR ( 'NONE', #54032, 1000.000000000000000 ) ;
#21743=ORIENTED_EDGE ( 'NONE', *, *, #26179, .F. ) ;
#21745=B_SPLINE_CURVE_WITH_KNOTS ( 'NONE', 3,
 ( #7559, #7906, #12873, #43447, #49134, #3592, #48151, #23858, #18555, #2609, #44119, #63726, #64386, #51085, #60071, #60384, #55742, #50749 ),
 .UNSPECIFIED., .F., .F.,
 ( 4, 2, 2, 2, 2, 2, 2, 2, 4 ),
 ( 4.906538933386797396E-18, 0.002682641281242477155, 0.003353301601553095469, 0.004023961921863713348, 0.005365282562484952576, 0.006706603203106191805, 0.008047923843727428431, 0.009389244484348668526, 0.01073056512496990689 ),
 .UNSPECIFIED. ) ;
#21746=CARTESIAN_POINT ( 'NONE',  ( 35.00000000000000000, -10.70999494708488520, 5.814360711498399503 ) ) ;
#21748=ORIENTED_EDGE ( 'NONE', *, *, #28671, .T. ) ;
#21749=CARTESIAN_POINT ( 'NONE',  ( -24.79499881855582188, -8.357637111868410074, 8.619227215508589168 ) ) ;
#21754=DIRECTION ( 'NONE',  ( 0.000000000000000000, 0.000000000000000000, -1.000000000000000000 ) ) ;
#21757=CARTESIAN_POINT ( 'NONE',  ( -37.00000000000000711, -10.28547182238004076, -5.672855678558794246 ) ) ;
#21758=VERTEX_POINT ( 'NONE', #4072 ) ;
#21759=CARTESIAN_POINT ( 'NONE',  ( -27.95874796761056658, 11.60023435971385553, -3.134445752752807568 ) ) ;
#21760=VERTEX_POINT ( 'NONE', #39963 ) ;
#21763=EDGE_LOOP ( 'NONE', ( #16724, #65241, #43333, #1413 ) ) ;
#21764=CARTESIAN_POINT ( 'NONE',  ( 22.22094857615726227, -10.34774274339837419, -6.087373716788684774 ) ) ;
#21766=AXIS2_PLACEMENT_3D ( 'NONE', #29810, #23539, #64722 ) ;
#21770=CARTESIAN_POINT ( 'NONE',  ( -37.00000000000000711, -11.17622378668009020, 3.614449339633449387 ) ) ;
#21771=FACE_OUTER_BOUND ( 'NONE', #41207, .T. ) ;
#21774=EDGE_CURVE ( 'NONE', #41285, #26398, #9055, .T. ) ;
#21775=( BOUNDED_CURVE ( )  B_SPLINE_CURVE ( 3, ( #61648, #36388, #5157, #25424 ),
 .UNSPECIFIED., .F., .T. ) 
 B_SPLINE_CURVE_WITH_KNOTS ( ( 4, 4 ),
 ( 0.8127194087688081048, 0.8598086627273093807 ),
 .UNSPECIFIED. ) 
 CURVE ( )  GEOMETRIC_REPRESENTATION_ITEM ( )  RATIONAL_B_SPLINE_CURVE ( ( 1.000000000000000000, 0.9998152253828482827, 0.9998152253828482827, 1.000000000000000000 ) ) 
 REPRESENTATION_ITEM ( '' )  );
#21779=ORIENTED_EDGE ( 'NONE', *, *, #20813, .F. ) ;
#21781=CARTESIAN_POINT ( 'NONE',  ( -35.00000000000000000, 0.000000000000000000, 0.000000000000000000 ) ) ;
#21783=DIRECTION ( 'NONE',  ( 1.000000000000000000, 0.000000000000000000, 0.000000000000000000 ) ) ;
#21784=FACE_OUTER_BOUND ( 'NONE', #34080, .T. ) ;
#21785=CARTESIAN_POINT ( 'NONE',  ( 35.00000000000000000, 7.718225330433935660, 9.430788938293964918 ) ) ;
#21787=AXIS2_PLACEMENT_3D ( 'NONE', #62251, #61586, #1430 ) ;
#21792=ADVANCED_FACE ( 'NONE', ( #57487 ), #1641, .T. ) ;
#21793=CARTESIAN_POINT ( 'NONE',  ( -4.033241259908380449, -9.046539124021903078, 7.887417314856400630 ) ) ;
#21794=EDGE_CURVE ( 'NONE', #38173, #52755, #44269, .T. ) ;
#21797=DIRECTION ( 'NONE',  ( 0.000000000000000000, -0.01356324068817998940, 0.9999080150203990547 ) ) ;
#21798=VECTOR ( 'NONE', #29953, 1000.000000000000000 ) ;
#21799=CARTESIAN_POINT ( 'NONE',  ( 22.85970942819514917, -4.208613694812052053, -12.82931771421080214 ) ) ;
#21800=DIRECTION ( 'NONE',  ( 1.000000000000000000, -0.000000000000000000, 0.000000000000000000 ) ) ;
#21806=EDGE_CURVE ( 'NONE', #9912, #10001, #31228, .T. ) ;
#21807=AXIS2_PLACEMENT_3D ( 'NONE', #15432, #35699, #55996 ) ;
#21808=EDGE_CURVE ( 'NONE', #54132, #31390, #10941, .T. ) ;
#21809=CARTESIAN_POINT ( 'NONE',  ( -37.00000000000000711, 10.70999494708501132, -5.814360711498173018 ) ) ;
#21810=CARTESIAN_POINT ( 'NONE',  ( -25.86628395826706850, -8.041618865309574815, 10.84354029019568522 ) ) ;
#21811=ORIENTED_EDGE ( 'NONE', *, *, #42607, .F. ) ;
#21813=LINE ( 'NONE', #11167, #64121 ) ;
#21815=ORIENTED_EDGE ( 'NONE', *, *, #61651, .F. ) ;
#21816=EDGE_CURVE ( 'NONE', #2142, #52203, #2603, .T. ) ;
#21818=DIRECTION ( 'NONE',  ( -1.000000000000000000, 0.000000000000000000, 0.000000000000000000 ) ) ;
#21819=CARTESIAN_POINT ( 'NONE',  ( 35.00000000000000000, 4.705694406421931860E-17, -3.469127814946512892E-15 ) ) ;
#21820=ORIENTED_EDGE ( 'NONE', *, *, #4484, .T. ) ;
#21821=DIRECTION ( 'NONE',  ( 0.000000000000000000, -0.01356324068817998940, 0.9999080150203990547 ) ) ;
#21822=AXIS2_PLACEMENT_3D ( 'NONE', #1014, #21280, #36903 ) ;
#21823=EDGE_CURVE ( 'NONE', #25967, #3960, #64953, .T. ) ;
#21824=CARTESIAN_POINT ( 'NONE',  ( -37.00000000000000711, -10.62137734850264614, -5.015831474386418520 ) ) ;
#21826=LINE ( 'NONE', #57387, #35429 ) ;
#21827=LINE ( 'NONE', #42073, #27708 ) ;
#21835=CARTESIAN_POINT ( 'NONE',  ( 24.19827605764011480, 1.944242837392233136, -11.84706149513093365 ) ) ;
#21836=ORIENTED_EDGE ( 'NONE', *, *, #17114, .T. ) ;
#21840=LINE ( 'NONE', #36106, #7607 ) ;
#21841=EDGE_LOOP ( 'NONE', ( #65478, #65311, #10162, #13183 ) ) ;
#21845=DIRECTION ( 'NONE',  ( -1.000000000000000000, 0.000000000000000000, -0.000000000000000000 ) ) ;
#21846=EDGE_LOOP ( 'NONE', ( #40613, #55187, #1988, #749 ) ) ;
#21847=ORIENTED_EDGE ( 'NONE', *, *, #28869, .T. ) ;
#21849=ORIENTED_EDGE ( 'NONE', *, *, #2204, .T. ) ;
#21852=CARTESIAN_POINT ( 'NONE',  ( 35.00000000000000000, 4.705694406421931860E-17, -3.469127814946512892E-15 ) ) ;
#21854=CARTESIAN_POINT ( 'NONE',  ( 35.00000000000000000, 4.705694406421931860E-17, -3.469127814946512892E-15 ) ) ;
#21855=FACE_OUTER_BOUND ( 'NONE', #51460, .T. ) ;
#21857=CYLINDRICAL_SURFACE ( 'NONE', #49317, 12.74999999999999822 ) ;
#21858=VERTEX_POINT ( 'NONE', #12247 ) ;
#21860=VERTEX_POINT ( 'NONE', #966 ) ;
#21861=DIRECTION ( 'NONE',  ( 1.000000000000000000, 0.000000000000000000, 0.000000000000000000 ) ) ;
#21862=EDGE_CURVE ( 'NONE', #19083, #2301, #27532, .T. ) ;
#21864=CARTESIAN_POINT ( 'NONE',  ( 37.00000000000000711, 10.32377448871667625, -6.475373545682339582 ) ) ;
#21865=DIRECTION ( 'NONE',  ( -1.000000000000000000, 0.000000000000000000, 0.000000000000000000 ) ) ;
#21868=ADVANCED_FACE ( 'NONE', ( #31541 ), #21588, .T. ) ;
#21874=CARTESIAN_POINT ( 'NONE',  ( 37.00000000000000711, 10.59380114696469910, -7.094637218249396859 ) ) ;
#21876=CARTESIAN_POINT ( 'NONE',  ( 35.00000000000000000, 3.340853584269691368, 11.26103545359851665 ) ) ;
#21877=ORIENTED_EDGE ( 'NONE', *, *, #62112, .T. ) ;
#21879=CARTESIAN_POINT ( 'NONE',  ( 35.00000000000000000, -0.3025107581130382917, 11.74226168163341022 ) ) ;
#21882=EDGE_CURVE ( 'NONE', #57018, #29075, #46843, .T. ) ;
#21885=CIRCLE ( 'NONE', #15499, 12.75000000000000178 ) ;
#21886=ORIENTED_EDGE ( 'NONE', *, *, #23576, .T. ) ;
#21888=VERTEX_POINT ( 'NONE', #36864 ) ;
#21889=CARTESIAN_POINT ( 'NONE',  ( 10.57567362079633355, 8.112553359107787188, -10.79197710481157557 ) ) ;
#21893=FACE_OUTER_BOUND ( 'NONE', #9577, .T. ) ;
#21895=EDGE_CURVE ( 'NONE', #9063, #50945, #28075, .T. ) ;
#21896=VERTEX_POINT ( 'NONE', #17582 ) ;
#21897=VERTEX_POINT ( 'NONE', #33825 ) ;
#21899=VERTEX_POINT ( 'NONE', #13239 ) ;
#21900=CYLINDRICAL_SURFACE ( 'NONE', #5426, 12.18649999999999878 ) ;
#21901=CARTESIAN_POINT ( 'NONE',  ( 3.375695012145481400, 5.390482730139837031, -12.38384929327539830 ) ) ;
#21902=CARTESIAN_POINT ( 'NONE',  ( 22.57855258442564761, -4.427776684447072952, 12.75322679295976691 ) ) ;
#21905=CYLINDRICAL_SURFACE ( 'NONE', #47256, 6.095312090839646757 ) ;
#21911=CARTESIAN_POINT ( 'NONE',  ( -37.00000000000000711, 11.56998259273177787, 3.827046518385122553 ) ) ;
#21912=CARTESIAN_POINT ( 'NONE',  ( -20.79170840334646542, 11.34110549087207076, -3.921648409140116698 ) ) ;
#21914=CARTESIAN_POINT ( 'NONE',  ( -35.00000000000000000, 0.000000000000000000, 0.000000000000000000 ) ) ;
#21915=EDGE_CURVE ( 'NONE', #53066, #476, #12108, .T. ) ;
#21916=FACE_OUTER_BOUND ( 'NONE', #12984, .T. ) ;
#21917=CARTESIAN_POINT ( 'NONE',  ( 37.00000000000000711, 12.17626345777663488, -0.4993900848167889817 ) ) ;
#21919=EDGE_LOOP ( 'NONE', ( #17910, #2168, #57549, #4295, #4691, #5302, #45839, #23472, #31699, #20603, #20845, #33653, #28464, #56946, #10851, #24962, #53982, #1656, #21010, #59536, #44381, #2368, #51004, #20814, #45536, #9003, #25912, #42254, #62390, #24672, #54862, #63917, #62202, #47679, #44952, #11715, #13762, #63530, #14151, #57156, #15288, #38229, #13650, #34786, #24156, #16701, #22813, #11838, #17480, #36847, #54699, #35651, #64571, #14527, #33270, #10210, #4720, #21673, #36755, #18217, #54303, #43166, #53143, #64898, #38308, #9632, #50187, #25861, #48324, #14418, #47658, #32459, #14816, #38001, #9707, #6968, #8635, #12530, #59569, #23103, #35940, #17046, #18495, #37575, #3803, #8051, #16697, #45391, #55998, #9039, #10854, #39972, #36044, #50384, #21394, #31130, #287, #48521, #1307, #39820, #23437, #48021, #23063, #10467, #54513, #43072, #59955, #52037, #36027, #54790, #55931, #55959, #37530, #37929, #43666, #50687, #13820, #17985, #37673, #61220, #17624, #13661, #48939, #13325, #32307, #23111, #51209, #52687, #17231, #44372, #11598, #23327, #51809, #45064, #20585, #32088, #64879, #5768, #6831, #34320, #5632, #32347, #61637, #16305, #17908, #5843, #24581, #38774, #44340, #1905, #34909, #45599, #787, #56193, #27457, #27872, #10288, #48225, #62791, #1600, #14205, #42896, #19419, #63759, #59811, #40454, #45592, #59658, #36629, #42543, #33734, #6881, #60493, #51680, #7596, #22983, #31635, #36390, #43421, #26572, #26065, #58897, #62305, #45888, #11756, #6048, #23320, #38313, #9727, #29428, #45539, #11268, #2586, #6596, #40094, #9790, #44179, #35581, #36515, #36079, #80, #58735, #58209, #25499, #2438, #37366, #14059, #57959, #36925, #61227, #40946, #62702, #62499, #65785, #43902, #22447, #12332, #62937, #20014, #51092, #51120, #1071, #44460, #39899, #2212, #47904, #16420, #43431, #33624, #58277, #32273, #5939, #27071, #24568, #49235, #51452, #8560, #28669, #16978, #42423, #21321, #10660, #65116, #51767, #45292, #50447, #58862, #43126, #32917, #33582, #13462, #41271, #42566, #36965, #39233, #14216, #14649, #47491, #51022, #65323, #58403, #29392, #61605, #45681, #17185, #27698, #24044, #62509, #4490, #12031, #37955, #65452, #65278, #1645, #25189, #38004, #44395, #34732, #6670, #14696, #41829, #58246, #64313, #35761, #20648, #9883, #23011, #6807, #39863, #4856, #7480, #45695, #6768, #1990, #32765, #19293, #2435, #32150, #51517, #37933, #2700, #3233, #41197, #63847, #8282, #34906, #25254, #56949, #46348, #55331, #5058, #63330, #4116, #36897, #6471, #34351, #4626, #53558, #15862, #17537, #5530, #45450, #56572, #38660, #14839, #57433, #42836, #37004, #46438, #58829, #11600, #50806, #65289, #6176, #13447, #44080, #59703, #980, #62615, #6148, #12883, #31612, #45218, #45981, #35213, #24337, #59109, #25003, #13115, #50290, #63760, #62698, #15196, #16726, #2642, #47649, #20893, #58001, #65683, #62074, #21971, #61282, #18395, #49354, #2283, #32122, #17849, #64201, #26724, #16062, #43928, #18652, #31248, #5490, #16607, #496, #54280, #43445, #58055, #9462, #3534, #30367, #40183, #53034, #32943, #56529, #59768, #46374, #28533, #64486, #21612, #46757, #55944, #53326, #20599, #31770, #60698, #54262, #12703, #544, #20363, #44236, #26684, #1868, #63870 ) ) ;
#21920=CARTESIAN_POINT ( 'NONE',  ( 37.00000000000000711, -6.657191900728386180, -9.677500615117878624 ) ) ;
#21924=ORIENTED_EDGE ( 'NONE', *, *, #34410, .F. ) ;
#21925=EDGE_LOOP ( 'NONE', ( #2432, #1559, #15703, #59250 ) ) ;
#21926=FACE_BOUND ( 'NONE', #8861, .T. ) ;
#21928=CYLINDRICAL_SURFACE ( 'NONE', #33120, 4.000030059823568074 ) ;
#21933=CARTESIAN_POINT ( 'NONE',  ( -37.00000000000000711, 8.839356091080043498, 8.389074212634319849 ) ) ;
#21934=AXIS2_PLACEMENT_3D ( 'NONE', #3754, #44274, #39615 ) ;
#21936=CARTESIAN_POINT ( 'NONE',  ( 37.00000000000000711, 10.63508530065521640, -4.986700593229742573 ) ) ;
#21939=ADVANCED_FACE ( 'NONE', ( #18583 ), #3619, .T. ) ;
#21943=DIRECTION ( 'NONE',  ( -1.000000000000000000, 0.000000000000000000, 0.000000000000000000 ) ) ;
#21944=VERTEX_POINT ( 'NONE', #12555 ) ;
#21945=DIRECTION ( 'NONE',  ( -1.000000000000000000, -0.000000000000000000, 0.000000000000000000 ) ) ;
#21946=( BOUNDED_CURVE ( )  B_SPLINE_CURVE ( 3, ( #34005, #19054, #53331, #48358 ),
 .UNSPECIFIED., .F., .F. ) 
 B_SPLINE_CURVE_WITH_KNOTS ( ( 4, 4 ),
 ( 1.889095289054163906, 1.912960151588308788 ),
 .UNSPECIFIED. ) 
 CURVE ( )  GEOMETRIC_REPRESENTATION_ITEM ( )  RATIONAL_B_SPLINE_CURVE ( ( 1.000000000000000000, 0.9999525395911521564, 0.9999525395911521564, 1.000000000000000000 ) ) 
 REPRESENTATION_ITEM ( '' )  );
#21948=DIRECTION ( 'NONE',  ( 0.000000000000000000, 0.5243256840888502746, 0.8515178078024906450 ) ) ;
#21953=VERTEX_POINT ( 'NONE', #13544 ) ;
#21954=FACE_OUTER_BOUND ( 'NONE', #34215, .T. ) ;
#21955=CARTESIAN_POINT ( 'NONE',  ( 37.00000000000000711, 4.705694406421931860E-17, -3.469127814946512892E-15 ) ) ;
#21956=CARTESIAN_POINT ( 'NONE',  ( -18.58686583997218378, 5.151216734910788908, 12.47858029384653555 ) ) ;
#21957=FACE_OUTER_BOUND ( 'NONE', #46058, .T. ) ;
#21958=CYLINDRICAL_SURFACE ( 'NONE', #16981, 4.999999999999999112 ) ;
#21959=VERTEX_POINT ( 'NONE', #54126 ) ;
#21962=AXIS2_PLACEMENT_3D ( 'NONE', #32599, #62536, #21992 ) ;
#21963=EDGE_CURVE ( 'NONE', #1294, #2632, #15291, .T. ) ;
#21965=EDGE_LOOP ( 'NONE', ( #30795, #32791, #60289, #6277 ) ) ;
#21966=ORIENTED_EDGE ( 'NONE', *, *, #56963, .F. ) ;
#21967=DIRECTION ( 'NONE',  ( 1.000000000000000000, 0.000000000000000000, 0.000000000000000000 ) ) ;
#21968=DIRECTION ( 'NONE',  ( 1.000000000000000000, 0.000000000000000000, 0.000000000000000000 ) ) ;
#21969=CARTESIAN_POINT ( 'NONE',  ( 35.00000000000000000, 12.05416472667167760, 1.791059740004291578 ) ) ;
#21970=DIRECTION ( 'NONE',  ( 0.000000000000000000, -0.01356324068817998940, 0.9999080150203990547 ) ) ;
#21971=ORIENTED_EDGE ( 'NONE', *, *, #29339, .F. ) ;
#21972=ORIENTED_EDGE ( 'NONE', *, *, #8811, .T. ) ;
#21975=CYLINDRICAL_SURFACE ( 'NONE', #58689, 12.18649999999999878 ) ;
#21977=EDGE_LOOP ( 'NONE', ( #43497, #36683, #17414, #14370 ) ) ;
#21978=DIRECTION ( 'NONE',  ( 1.000000000000000000, -0.000000000000000000, 0.000000000000000000 ) ) ;
#21984=DIRECTION ( 'NONE',  ( 1.000000000000000000, 0.000000000000000000, 0.000000000000000000 ) ) ;
#21987=ADVANCED_FACE ( 'NONE', ( #52711 ), #43037, .T. ) ;
#21988=VERTEX_POINT ( 'NONE', #41733 ) ;
#21989=CARTESIAN_POINT ( 'NONE',  ( 11.92370524553500388, 0.08318608274626294874, -13.49997410565396905 ) ) ;
#21990=CARTESIAN_POINT ( 'NONE',  ( -18.20967569695231703, -5.494204602085749123, 12.33373156890061395 ) ) ;
#21992=DIRECTION ( 'NONE',  ( 0.000000000000000000, -0.2355298848897586228, -0.9718671068226442111 ) ) ;
#21995=EDGE_CURVE ( 'NONE', #7316, #20098, #11076, .T. ) ;
#21996=DIRECTION ( 'NONE',  ( 0.000000000000000000, 0.01356324068817998940, -0.9999080150203990547 ) ) ;
#21998=EDGE_LOOP ( 'NONE', ( #26670, #29606, #56459, #26822 ) ) ;
#21999=DIRECTION ( 'NONE',  ( 0.000000000000000000, 0.3807014730195151797, -0.9246979985058750851 ) ) ;
#22000=ORIENTED_EDGE ( 'NONE', *, *, #25667, .F. ) ;
#22002=DIRECTION ( 'NONE',  ( -1.000000000000000000, 0.000000000000000000, -0.000000000000000000 ) ) ;
#22003=EDGE_CURVE ( 'NONE', #35347, #32947, #62331, .T. ) ;
#22004=DIRECTION ( 'NONE',  ( 1.000000000000000000, -0.000000000000000000, 0.000000000000000000 ) ) ;
#22008=CARTESIAN_POINT ( 'NONE',  ( -36.00000000000000711, -10.68873102412847764, 6.950793414699757200 ) ) ;
#22009=ORIENTED_EDGE ( 'NONE', *, *, #49853, .F. ) ;
#22011=CIRCLE ( 'NONE', #47511, 4.999999999999999112 ) ;
#22012=DIRECTION ( 'NONE',  ( -1.000000000000000000, -0.000000000000000000, 0.000000000000000000 ) ) ;
#22013=EDGE_CURVE ( 'NONE', #35492, #15725, #16394, .T. ) ;
#22015=DIRECTION ( 'NONE',  ( 0.000000000000000000, -0.01356324068817991828, 0.9999080150203990547 ) ) ;
#22016=EDGE_CURVE ( 'NONE', #11898, #42832, #4733, .T. ) ;
#22019=DIRECTION ( 'NONE',  ( 0.000000000000000000, -0.01356324068817991828, 0.9999080150203990547 ) ) ;
#22021=EDGE_LOOP ( 'NONE', ( #39554, #47293, #1305, #34094 ) ) ;
#22022=CARTESIAN_POINT ( 'NONE',  ( 24.82652845881425208, -8.390869743685021476, -8.578654028722157321 ) ) ;
#22023=LINE ( 'NONE', #27334, #9663 ) ;
#22024=CARTESIAN_POINT ( 'NONE',  ( -35.00000000000000000, 7.251710744571578715, 9.240395740215660680 ) ) ;
#22026=FACE_OUTER_BOUND ( 'NONE', #6466, .T. ) ;
#22029=VECTOR ( 'NONE', #64574, 1000.000000000000000 ) ;
#22031=ORIENTED_EDGE ( 'NONE', *, *, #24030, .F. ) ;
#22034=CARTESIAN_POINT ( 'NONE',  ( 3.347841273039249721, -10.61118957148187825, 8.345816669330455184 ) ) ;
#22036=EDGE_CURVE ( 'NONE', #30305, #18413, #51732, .T. ) ;
#22044=EDGE_LOOP ( 'NONE', ( #20462, #36546, #31922, #18012 ) ) ;
#22045=VECTOR ( 'NONE', #11211, 1000.000000000000000 ) ;
#22046=ORIENTED_EDGE ( 'NONE', *, *, #30555, .T. ) ;
#22047=CARTESIAN_POINT ( 'NONE',  ( 35.00000000000000000, 4.705694406421931860E-17, -3.469127814946512892E-15 ) ) ;
#22048=EDGE_CURVE ( 'NONE', #34279, #39829, #65218, .T. ) ;
#22049=CIRCLE ( 'NONE', #37991, 12.75000000000000178 ) ;
#22051=DIRECTION ( 'NONE',  ( -1.000000000000000000, 0.000000000000000000, 0.000000000000000000 ) ) ;
#22055=ORIENTED_EDGE ( 'NONE', *, *, #23660, .T. ) ;
#22058=CARTESIAN_POINT ( 'NONE',  ( -26.34600911009608382, 10.72077307324429718, 5.391900231479520578 ) ) ;
#22060=CARTESIAN_POINT ( 'NONE',  ( 25.05309951391468459, 8.823569016628493245, -8.132934882857099979 ) ) ;
#22061=EDGE_CURVE ( 'NONE', #9614, #48986, #7901, .T. ) ;
#22062=VERTEX_POINT ( 'NONE', #36747 ) ;
#22064=ORIENTED_EDGE ( 'NONE', *, *, #31349, .F. ) ;
#22065=CARTESIAN_POINT ( 'NONE',  ( 21.50270529625529647, -11.33978786238144032, -3.930893046708287653 ) ) ;
#22066=CARTESIAN_POINT ( 'NONE',  ( 35.00000000000000000, 4.309077947445811851, 10.92721691015450780 ) ) ;
#22067=CARTESIAN_POINT ( 'NONE',  ( -35.00000000000000000, 0.4993900848167411310, 12.17626345777664021 ) ) ;
#22068=ORIENTED_EDGE ( 'NONE', *, *, #29680, .F. ) ;
#22069=CARTESIAN_POINT ( 'NONE',  ( 35.00000000000000000, 4.705694406421931860E-17, -3.469127814946512892E-15 ) ) ;
#22072=ORIENTED_EDGE ( 'NONE', *, *, #41479, .T. ) ;
#22073=EDGE_LOOP ( 'NONE', ( #15613, #59793, #31016, #10775 ) ) ;
#22076=EDGE_CURVE ( 'NONE', #40304, #44716, #62048, .T. ) ;
#22079=CARTESIAN_POINT ( 'NONE',  ( 35.00000000000000000, -6.917234959366766134, 9.493370459201765144 ) ) ;
#22082=DIRECTION ( 'NONE',  ( 1.000000000000000000, 0.000000000000000000, 0.000000000000000000 ) ) ;
#22086=DIRECTION ( 'NONE',  ( 1.000000000000000000, 0.000000000000000000, 0.000000000000000000 ) ) ;
#22092=ADVANCED_FACE ( 'NONE', ( #1632 ), #21905, .F. ) ;
#22093=CARTESIAN_POINT ( 'NONE',  ( -11.40165637462999904, -7.508992741355383416, 25.00000000000000000 ) ) ;
#22095=CARTESIAN_POINT ( 'NONE',  ( 35.00000000000000000, -11.70009620280412399, -1.039216533672868481 ) ) ;
#22097=DIRECTION ( 'NONE',  ( 0.000000000000000000, -0.3807014730195086849, 0.9246979985058776386 ) ) ;
#22098=CARTESIAN_POINT ( 'NONE',  ( -35.00000000000000000, 9.926225166347114381, -6.280308599560036065 ) ) ;
#22099=DIRECTION ( 'NONE',  ( 0.000000000000000000, 0.1740410799127612429, 0.9847383929261617208 ) ) ;
#22100=CARTESIAN_POINT ( 'NONE',  ( 23.11472949692741352, -3.958498414078114092, -12.90974724811009366 ) ) ;
#22106=DIRECTION ( 'NONE',  ( 0.000000000000000000, -0.9346839223284501008, 0.3554799084909069928 ) ) ;
#22108=FACE_OUTER_BOUND ( 'NONE', #21021, .T. ) ;
#22109=CARTESIAN_POINT ( 'NONE',  ( 12.52750123246316072, 0.4973700281276248192, 13.49083477977253764 ) ) ;
#22111=CIRCLE ( 'NONE', #27421, 5.000000000000000888 ) ;
#22113=CARTESIAN_POINT ( 'NONE',  ( -27.74658222974374411, -12.59936487573947517, -4.856608172635154652 ) ) ;
#22116=ORIENTED_EDGE ( 'NONE', *, *, #55178, .T. ) ;
#22117=DIRECTION ( 'NONE',  ( -1.000000000000000000, 0.000000000000000000, -0.000000000000000000 ) ) ;
#22119=EDGE_CURVE ( 'NONE', #24257, #43073, #15335, .T. ) ;
#22121=EDGE_LOOP ( 'NONE', ( #38980, #44151, #1705, #26842 ) ) ;
#22124=CARTESIAN_POINT ( 'NONE',  ( 35.00000000000000000, 4.705694406421931860E-17, -3.469127814946512892E-15 ) ) ;
#22125=EDGE_LOOP ( 'NONE', ( #11203, #28279, #57988, #757 ) ) ;
#22126=CARTESIAN_POINT ( 'NONE',  ( 37.00000000000000711, 4.705694406421931860E-17, -3.469127814946512892E-15 ) ) ;
#22127=DIRECTION ( 'NONE',  ( 0.000000000000000000, 0.01356324068817991828, -0.9999080150203990547 ) ) ;
#22129=CARTESIAN_POINT ( 'NONE',  ( -37.00000000000000711, 0.000000000000000000, 0.000000000000000000 ) ) ;
#22130=CIRCLE ( 'NONE', #5161, 5.000000000000000000 ) ;
#22135=CARTESIAN_POINT ( 'NONE',  ( -35.00000000000000000, -3.827046518385164742, 11.56998259273176188 ) ) ;
#22136=ORIENTED_EDGE ( 'NONE', *, *, #22619, .T. ) ;
#22138=ADVANCED_FACE ( 'NONE', ( #60088 ), #24177, .T. ) ;
#22139=ORIENTED_EDGE ( 'NONE', *, *, #40536, .T. ) ;
#22140=DIRECTION ( 'NONE',  ( -1.000000000000000000, -0.000000000000000000, 0.000000000000000000 ) ) ;
#22141=VERTEX_POINT ( 'NONE', #43813 ) ;
#22142=AXIS2_PLACEMENT_3D ( 'NONE', #6238, #62393, #16851 ) ;
#22143=CYLINDRICAL_SURFACE ( 'NONE', #28407, 5.000000000000000888 ) ;
#22144=CYLINDRICAL_SURFACE ( 'NONE', #41750, 12.75000000000000178 ) ;
#22147=ORIENTED_EDGE ( 'NONE', *, *, #3894, .F. ) ;
#22148=LINE ( 'NONE', #31476, #36816 ) ;
#22150=ORIENTED_EDGE ( 'NONE', *, *, #47744, .F. ) ;
#22151=VERTEX_POINT ( 'NONE', #19849 ) ;
#22152=DIRECTION ( 'NONE',  ( 0.000000000000000000, -0.01356324068817998940, 0.9999080150203990547 ) ) ;
#22153=EDGE_LOOP ( 'NONE', ( #51963, #54193, #36115, #11900 ) ) ;
#22156=DIRECTION ( 'NONE',  ( 0.000000000000000000, 0.01356324068817998940, -0.9999080150203990547 ) ) ;
#22157=EDGE_CURVE ( 'NONE', #48416, #10957, #10078, .T. ) ;
#22158=DIRECTION ( 'NONE',  ( 1.000000000000000000, -0.000000000000000000, 0.000000000000000000 ) ) ;
#22159=LINE ( 'NONE', #33767, #29866 ) ;
#22161=AXIS2_PLACEMENT_3D ( 'NONE', #28001, #46971, #56958 ) ;
#22163=CARTESIAN_POINT ( 'NONE',  ( 35.00000000000000000, 4.705694406421931860E-17, -3.469127814946512892E-15 ) ) ;
#22164=ORIENTED_EDGE ( 'NONE', *, *, #558, .F. ) ;
#22165=LINE ( 'NONE', #58762, #46487 ) ;
#22166=VERTEX_POINT ( 'NONE', #19193 ) ;
#22167=EDGE_CURVE ( 'NONE', #12197, #58057, #45072, .T. ) ;
#22168=CYLINDRICAL_SURFACE ( 'NONE', #1335, 4.999999999999999112 ) ;
#22170=FACE_OUTER_BOUND ( 'NONE', #23208, .T. ) ;
#22172=VECTOR ( 'NONE', #35203, 1000.000000000000000 ) ;
#22173=EDGE_LOOP ( 'NONE', ( #11870, #27823, #18892, #26069 ) ) ;
#22176=STYLED_ITEM ( 'NONE', ( #49257 ), #30113 ) ;
#22177=ORIENTED_EDGE ( 'NONE', *, *, #7110, .F. ) ;
#22180=VECTOR ( 'NONE', #32534, 1000.000000000000000 ) ;
#22182=DIRECTION ( 'NONE',  ( 1.000000000000000000, -0.000000000000000000, 0.000000000000000000 ) ) ;
#22185=DIRECTION ( 'NONE',  ( 1.000000000000000000, 0.000000000000000000, 0.000000000000000000 ) ) ;
#22186=CARTESIAN_POINT ( 'NONE',  ( -35.00000000000000000, 0.000000000000000000, 0.000000000000000000 ) ) ;
#22187=DIRECTION ( 'NONE',  ( -0.000000000000000000, -1.000000000000000000, -0.000000000000000000 ) ) ;
#22188=EDGE_CURVE ( 'NONE', #55976, #31867, #47212, .T. ) ;
#22190=ADVANCED_FACE ( 'NONE', ( #44444 ), #34482, .T. ) ;
#22191=CARTESIAN_POINT ( 'NONE',  ( -35.00000000000000000, -0.2661492558804205988, 12.18359334611896472 ) ) ;
#22192=ORIENTED_EDGE ( 'NONE', *, *, #29704, .F. ) ;
#22194=ORIENTED_EDGE ( 'NONE', *, *, #63157, .T. ) ;
#22197=DIRECTION ( 'NONE',  ( -1.000000000000000000, 0.000000000000000000, 0.000000000000000000 ) ) ;
#22198=EDGE_CURVE ( 'NONE', #33015, #19363, #3696, .T. ) ;
#22199=DIRECTION ( 'NONE',  ( 1.000000000000000000, 0.000000000000000000, -0.000000000000000000 ) ) ;
#22201=AXIS2_PLACEMENT_3D ( 'NONE', #20216, #19893, #49831 ) ;
#22205=CARTESIAN_POINT ( 'NONE',  ( 35.00000000000000000, 1.262958560998929558, 12.12087942037208066 ) ) ;
#22207=CARTESIAN_POINT ( 'NONE',  ( -35.00000000000000000, -4.983891302653499444, -11.73555825188281609 ) ) ;
#22209=AXIS2_PLACEMENT_3D ( 'NONE', #37878, #42861, #54158 ) ;
#22210=DIRECTION ( 'NONE',  ( -1.000000000000000000, 0.000000000000000000, 0.000000000000000000 ) ) ;
#22212=CARTESIAN_POINT ( 'NONE',  ( -17.08916676964391357, 2.790706569880187615, -13.20909463602864697 ) ) ;
#22213=ORIENTED_EDGE ( 'NONE', *, *, #20340, .F. ) ;
#22214=EDGE_CURVE ( 'NONE', #52362, #53221, #52532, .T. ) ;
#22215=EDGE_CURVE ( 'NONE', #3010, #60035, #18548, .T. ) ;
#22218=ORIENTED_EDGE ( 'NONE', *, *, #62412, .T. ) ;
#22220=EDGE_CURVE ( 'NONE', #45080, #22263, #51490, .T. ) ;
#22221=CARTESIAN_POINT ( 'NONE',  ( 22.80864547236593154, -11.57366291690524029, -6.957251879747434309 ) ) ;
#22222=VECTOR ( 'NONE', #59753, 1000.000000000000000 ) ;
#22223=DIRECTION ( 'NONE',  ( 0.000000000000000000, 0.01356324068818000848, -0.9999080150203990547 ) ) ;
#22224=CARTESIAN_POINT ( 'NONE',  ( 35.00000000000000000, -6.303578524887018197, -10.42955799785318050 ) ) ;
#22227=CYLINDRICAL_SURFACE ( 'NONE', #5747, 12.74999999999999822 ) ;
#22232=DIRECTION ( 'NONE',  ( 0.000000000000000000, -0.8696919319575129315, -0.4935949184179356242 ) ) ;
#22235=DIRECTION ( 'NONE',  ( 1.000000000000000000, 0.000000000000000000, -0.000000000000000000 ) ) ;
#22236=ORIENTED_EDGE ( 'NONE', *, *, #21015, .T. ) ;
#22237=VECTOR ( 'NONE', #13320, 1000.000000000000000 ) ;
#22238=ORIENTED_EDGE ( 'NONE', *, *, #31967, .T. ) ;
#22240=ADVANCED_FACE ( 'NONE', ( #50119 ), #4575, .T. ) ;
#22245=EDGE_CURVE ( 'NONE', #38335, #26398, #54671, .T. ) ;
#22246=DIRECTION ( 'NONE',  ( -1.000000000000000000, 0.000000000000000000, 0.000000000000000000 ) ) ;
#22247=VERTEX_POINT ( 'NONE', #45435 ) ;
#22248=LINE ( 'NONE', #62475, #12584 ) ;
#22250=CARTESIAN_POINT ( 'NONE',  ( 37.00000000000000711, 1.771820996347156507, -11.61175578952786935 ) ) ;
#22252=DIRECTION ( 'NONE',  ( 0.000000000000000000, -0.01356324068817998940, 0.9999080150203990547 ) ) ;
#22253=LINE ( 'NONE', #22933, #61026 ) ;
#22254=CIRCLE ( 'NONE', #1045, 12.74999999999999822 ) ;
#22257=VERTEX_POINT ( 'NONE', #568 ) ;
#22258=CYLINDRICAL_SURFACE ( 'NONE', #8358, 5.000000000000000888 ) ;
#22263=VERTEX_POINT ( 'NONE', #65700 ) ;
#22266=DIRECTION ( 'NONE',  ( 1.000000000000000000, 0.000000000000000000, 0.000000000000000000 ) ) ;
#22267=CARTESIAN_POINT ( 'NONE',  ( 26.17129964821461385, 11.44745868472665684, 3.602463285258926895 ) ) ;
#22268=CIRCLE ( 'NONE', #12710, 5.000000000000000888 ) ;
#22269=CIRCLE ( 'NONE', #27585, 5.000000000000000888 ) ;
#22270=EDGE_CURVE ( 'NONE', #4031, #44052, #20830, .T. ) ;
#22274=PRODUCT_DEFINITION_SHAPE ( 'NONE', 'NONE',  #57568 ) ;
#22276=ADVANCED_FACE ( 'NONE', ( #30471 ), #5896, .T. ) ;
#22280=DIRECTION ( 'NONE',  ( 1.000000000000000000, -0.000000000000000000, -0.000000000000000000 ) ) ;
#22282=DIRECTION ( 'NONE',  ( 0.000000000000000000, -0.01356324068817992175, 0.9999080150203990547 ) ) ;
#22285=ORIENTED_EDGE ( 'NONE', *, *, #42860, .F. ) ;
#22289=VECTOR ( 'NONE', #61748, 1000.000000000000000 ) ;
#22290=ORIENTED_EDGE ( 'NONE', *, *, #15569, .F. ) ;
#22291=CARTESIAN_POINT ( 'NONE',  ( -27.27855387000350262, -12.26939275170277632, 5.631341004100471892 ) ) ;
#22293=EDGE_LOOP ( 'NONE', ( #26456, #25156, #39888, #60091 ) ) ;
#22294=CARTESIAN_POINT ( 'NONE',  ( 35.00000000000000000, 11.81949347079746637, -2.968224442958448783 ) ) ;
#22296=CARTESIAN_POINT ( 'NONE',  ( 24.67819621425959298, 0.8561783389638295549, 11.97593107962119419 ) ) ;
#22297=ORIENTED_EDGE ( 'NONE', *, *, #38518, .F. ) ;
#22298=ORIENTED_EDGE ( 'NONE', *, *, #5249, .F. ) ;
#22299=LINE ( 'NONE', #7334, #64980 ) ;
#22301=CARTESIAN_POINT ( 'NONE',  ( 11.39183535642925804, 0.2409185311480156466, -13.49808056869716033 ) ) ;
#22302=CARTESIAN_POINT ( 'NONE',  ( -17.66721521611205503, -6.974610761929137759, 11.56240511626955758 ) ) ;
#22304=ADVANCED_FACE ( 'NONE', ( #55426 ), #60403, .T. ) ;
#22305=DIRECTION ( 'NONE',  ( 0.000000000000000000, -0.6745969609292555846, -0.7381862504172049810 ) ) ;
#22306=DIRECTION ( 'NONE',  ( -1.000000000000000000, 0.000000000000000000, 0.000000000000000000 ) ) ;
#22309=CARTESIAN_POINT ( 'NONE',  ( 5.587718367926578722, -9.343663864590265433, -7.538223026388563675 ) ) ;
#22310=ORIENTED_EDGE ( 'NONE', *, *, #17491, .T. ) ;
#22311=AXIS2_PLACEMENT_3D ( 'NONE', #42814, #12884, #62431 ) ;
#22312=DIRECTION ( 'NONE',  ( 0.000000000000000000, 0.8696919319575167062, 0.4935949184179292404 ) ) ;
#22320=LINE ( 'NONE', #46313, #52494 ) ;
#22321=EDGE_LOOP ( 'NONE', ( #15698, #52921, #41806, #55269 ) ) ;
#22322=ADVANCED_FACE ( 'NONE', ( #30154 ), #16167, .T. ) ;
#22325=AXIS2_PLACEMENT_3D ( 'NONE', #38009, #43325, #18075 ) ;
#22327=DIRECTION ( 'NONE',  ( 0.000000000000000000, -0.9847383929261634972, 0.1740410799127515284 ) ) ;
#22329=DIRECTION ( 'NONE',  ( 0.000000000000000000, -0.01356324068817991828, 0.9999080150203990547 ) ) ;
#22331=CARTESIAN_POINT ( 'NONE',  ( -19.69476066079020171, -4.201994156881551312, 11.24025111398909615 ) ) ;
#22332=ORIENTED_EDGE ( 'NONE', *, *, #25201, .F. ) ;
#22333=DIRECTION ( 'NONE',  ( 1.000000000000000000, 0.000000000000000000, -0.000000000000000000 ) ) ;
#22335=VECTOR ( 'NONE', #50183, 1000.000000000000000 ) ;
#22336=EDGE_CURVE ( 'NONE', #24509, #55514, #27022, .T. ) ;
#22338=AXIS2_PLACEMENT_3D ( 'NONE', #30276, #38946, #13656 ) ;
#22339=AXIS2_PLACEMENT_3D ( 'NONE', #45506, #50844, #9947 ) ;
#22340=EDGE_CURVE ( 'NONE', #17445, #38122, #49774, .T. ) ;
#22342=CARTESIAN_POINT ( 'NONE',  ( 35.00000000000000000, -4.339012074899872395, 10.91536515067652324 ) ) ;
#22343=DIRECTION ( 'NONE',  ( 0.000000000000000000, -0.01356324068817991828, 0.9999080150203990547 ) ) ;
#22346=CARTESIAN_POINT ( 'NONE',  ( -8.891032880924177206, -11.36194426013948444, -3.860857758255646921 ) ) ;
#22347=CARTESIAN_POINT ( 'NONE',  ( -35.00000000000000000, -10.07641281632181673, 6.036400161834530209 ) ) ;
#22349=AXIS2_PLACEMENT_3D ( 'NONE', #40040, #50037, #19456 ) ;
#22350=EDGE_CURVE ( 'NONE', #59860, #39182, #64182, .T. ) ;
#22352=DIRECTION ( 'NONE',  ( -1.000000000000000000, -0.000000000000000000, 0.000000000000000000 ) ) ;
#22356=EDGE_LOOP ( 'NONE', ( #33151, #45127, #46021, #19688 ) ) ;
#22358=EDGE_CURVE ( 'NONE', #36702, #57461, #33422, .T. ) ;
#22363=VERTEX_POINT ( 'NONE', #25828 ) ;
#22364=DIRECTION ( 'NONE',  ( 0.9759340573753173542, 0.2180658516479614117, 0.000000000000000000 ) ) ;
#22365=VERTEX_POINT ( 'NONE', #31462 ) ;
#22366=VERTEX_POINT ( 'NONE', #5217 ) ;
#22367=B_SPLINE_CURVE_WITH_KNOTS ( 'NONE', 3,
 ( #45734, #10813, #30438, #5526, #31101, #46395, #15141, #20138, #844, #61673, #35424, #36416, #6172, #26434, #1177, #55729, #10159, #22100, #21799, #62644 ),
 .UNSPECIFIED., .F., .F.,
 ( 4, 2, 2, 2, 2, 2, 2, 2, 2, 4 ),
 ( 0.000000000000000000, 0.001078581342907173040, 0.002157162685814346080, 0.003235744028721518686, 0.004314325371628692160, 0.005392906714535864766, 0.005932197385989450636, 0.006471488057443037373, 0.007550069400350215183, 0.008628650743257391259 ),
 .UNSPECIFIED. ) ;
#22370=ADVANCED_FACE ( 'NONE', ( #25484 ), #45773, .T. ) ;
#22371=CARTESIAN_POINT ( 'NONE',  ( 35.00000000000000000, 7.146664589317909488, -9.321877890560465119 ) ) ;
#22376=ORIENTED_EDGE ( 'NONE', *, *, #46484, .T. ) ;
#22377=CARTESIAN_POINT ( 'NONE',  ( 37.00000000000000711, 9.677500615117898164, -6.657191900728355094 ) ) ;
#22380=DIRECTION ( 'NONE',  ( 0.000000000000000000, 0.01356324068817998940, -0.9999080150203990547 ) ) ;
#22383=AXIS2_PLACEMENT_3D ( 'NONE', #39799, #55086, #9515 ) ;
#22384=ORIENTED_EDGE ( 'NONE', *, *, #55425, .T. ) ;
#22385=DIRECTION ( 'NONE',  ( 0.000000000000000000, -0.9970832820307047317, -0.07632122047555413291 ) ) ;
#22386=EDGE_LOOP ( 'NONE', ( #60483, #7037, #30620, #28796 ) ) ;
#22387=CARTESIAN_POINT ( 'NONE',  ( -35.00000000000000000, 0.000000000000000000, 0.000000000000000000 ) ) ;
#22388=CARTESIAN_POINT ( 'NONE',  ( 35.00000000000000000, 9.512294188640899151, -6.891188680298859559 ) ) ;
#22390=AXIS2_PLACEMENT_3D ( 'NONE', #33722, #8458, #43363 ) ;
#22391=VERTEX_POINT ( 'NONE', #52739 ) ;
#22394=AXIS2_PLACEMENT_3D ( 'NONE', #27437, #15815, #46748 ) ;
#22396=CARTESIAN_POINT ( 'NONE',  ( 12.10998784662220551, 10.46621227226785322, -8.526922110106907482 ) ) ;
#22397=ORIENTED_EDGE ( 'NONE', *, *, #61209, .T. ) ;
#22398=ORIENTED_EDGE ( 'NONE', *, *, #46405, .F. ) ;
#22399=AXIS2_PLACEMENT_3D ( 'NONE', #55368, #35403, #9806 ) ;
#22400=DIRECTION ( 'NONE',  ( 0.000000000000000000, 0.9999080150203990547, 0.01356324068817645230 ) ) ;
#22402=VERTEX_POINT ( 'NONE', #62684 ) ;
#22404=CYLINDRICAL_SURFACE ( 'NONE', #60206, 12.18649999999999878 ) ;
#22405=LINE ( 'NONE', #57025, #27714 ) ;
#22409=EDGE_CURVE ( 'NONE', #52056, #42316, #62058, .T. ) ;
#22410=AXIS2_PLACEMENT_3D ( 'NONE', #54242, #49903, #3389 ) ;
#22411=CARTESIAN_POINT ( 'NONE',  ( 35.00000000000000000, -11.37311665002365579, -2.936739658819832677 ) ) ;
#22413=VECTOR ( 'NONE', #40245, 1000.000000000000000 ) ;
#22415=VECTOR ( 'NONE', #24934, 1000.000000000000000 ) ;
#22416=DIRECTION ( 'NONE',  ( -1.000000000000000000, 0.000000000000000000, 0.000000000000000000 ) ) ;
#22417=CARTESIAN_POINT ( 'NONE',  ( -37.00000000000000711, -12.38385022362079724, -3.033604067594711129 ) ) ;
#22418=CIRCLE ( 'NONE', #13913, 4.999999999999999112 ) ;
#22421=CARTESIAN_POINT ( 'NONE',  ( -37.00000000000000711, -12.08216339958899788, -1.591260454995368390 ) ) ;
#22422=EDGE_CURVE ( 'NONE', #4031, #42345, #62912, .T. ) ;
#22425=DIRECTION ( 'NONE',  ( 1.000000000000000000, 0.000000000000000000, -0.000000000000000000 ) ) ;
#22426=EDGE_CURVE ( 'NONE', #38782, #49313, #58946, .T. ) ;
#22427=DIRECTION ( 'NONE',  ( 1.000000000000000000, 0.000000000000000000, 0.000000000000000000 ) ) ;
#22428=AXIS2_PLACEMENT_3D ( 'NONE', #15419, #24407, #60003 ) ;
#22429=EDGE_CURVE ( 'NONE', #54444, #13128, #4787, .T. ) ;
#22430=VERTEX_POINT ( 'NONE', #7844 ) ;
#22432=DIRECTION ( 'NONE',  ( -1.000000000000000000, 0.000000000000000000, 0.000000000000000000 ) ) ;
#22435=AXIS2_PLACEMENT_3D ( 'NONE', #16716, #27035, #51983 ) ;
#22436=CIRCLE ( 'NONE', #53264, 5.000000000000000888 ) ;
#22437=VECTOR ( 'NONE', #37655, 1000.000000000000000 ) ;
#22441=ORIENTED_EDGE ( 'NONE', *, *, #40336, .F. ) ;
#22442=CARTESIAN_POINT ( 'NONE',  ( 19.28625800530496903, -1.699513388191772778, 11.87904264843580471 ) ) ;
#22443=CARTESIAN_POINT ( 'NONE',  ( -17.97167269346459051, 4.327294505063981944, 12.78955090225081648 ) ) ;
#22447=ORIENTED_EDGE ( 'NONE', *, *, #49457, .F. ) ;
#22449=DIRECTION ( 'NONE',  ( 0.000000000000000000, -0.01356324068817998940, 0.9999080150203990547 ) ) ;
#22451=VERTEX_POINT ( 'NONE', #12468 ) ;
#22452=CARTESIAN_POINT ( 'NONE',  ( -37.00000000000000711, -8.699265615722922007, -8.534258022646191932 ) ) ;
#22453=EDGE_CURVE ( 'NONE', #64447, #44513, #42959, .T. ) ;
#22454=VECTOR ( 'NONE', #33446, 1000.000000000000000 ) ;
#22455=VECTOR ( 'NONE', #55970, 1000.000000000000000 ) ;
#22456=B_SPLINE_CURVE_WITH_KNOTS ( 'NONE', 3,
 ( #31135, #61070, #565, #55757, #10189, #61373, #5215, #50451, #50116, #25160, #20828, #29806 ),
 .UNSPECIFIED., .F., .F.,
 ( 4, 2, 2, 2, 2, 4 ),
 ( 0.006656218235223304580, 0.007268574118352267091, 0.007880930001481229602, 0.009105641767739156359, 0.01033035353399708312, 0.01155506530025500814 ),
 .UNSPECIFIED. ) ;
#22458=EDGE_LOOP ( 'NONE', ( #51553, #24774, #64388, #25873 ) ) ;
#22460=ADVANCED_FACE ( 'NONE', ( #32741 ), #57392, .T. ) ;
#22465=CARTESIAN_POINT ( 'NONE',  ( -8.813892140501407013, 7.428019780266606809, -9.432948737998053446 ) ) ;
#22466=AXIS2_PLACEMENT_3D ( 'NONE', #58729, #3528, #14438 ) ;
#22467=EDGE_CURVE ( 'NONE', #53449, #41765, #14284, .T. ) ;
#22468=CARTESIAN_POINT ( 'NONE',  ( -10.64311535907469874, -9.781890035361623603, 9.304428041637393676 ) ) ;
#22470=VERTEX_POINT ( 'NONE', #32102 ) ;
#22472=ORIENTED_EDGE ( 'NONE', *, *, #97, .F. ) ;
#22473=DIRECTION ( 'NONE',  ( 0.000000000000000000, -0.9467777615094604693, -0.3218879778915876844 ) ) ;
#22480=CARTESIAN_POINT ( 'NONE',  ( 35.00000000000000000, -8.839356091080105671, -8.389074212634254124 ) ) ;
#22483=ORIENTED_EDGE ( 'NONE', *, *, #8736, .T. ) ;
#22484=AXIS2_PLACEMENT_3D ( 'NONE', #21852, #36800, #22156 ) ;
#22487=EDGE_LOOP ( 'NONE', ( #1296, #60331, #30732, #21849 ) ) ;
#22488=ORIENTED_EDGE ( 'NONE', *, *, #13841, .T. ) ;
#22491=ORIENTED_EDGE ( 'NONE', *, *, #33036, .F. ) ;
#22495=CYLINDRICAL_SURFACE ( 'NONE', #50731, 12.75000000000000178 ) ;
#22496=CIRCLE ( 'NONE', #2343, 12.75000000000000178 ) ;
#22498=CIRCLE ( 'NONE', #32061, 5.000000000000000888 ) ;
#22499=EDGE_CURVE ( 'NONE', #2584, #44869, #34711, .T. ) ;
#22500=DIRECTION ( 'NONE',  ( -1.000000000000000000, 0.000000000000000000, -0.000000000000000000 ) ) ;
#22512=EDGE_CURVE ( 'NONE', #30999, #9450, #37651, .T. ) ;
#22514=ORIENTED_EDGE ( 'NONE', *, *, #17675, .F. ) ;
#22515=VECTOR ( 'NONE', #26870, 1000.000000000000000 ) ;
#22516=ORIENTED_EDGE ( 'NONE', *, *, #25679, .T. ) ;
#22517=EDGE_CURVE ( 'NONE', #61175, #56695, #48314, .T. ) ;
#22523=VECTOR ( 'NONE', #36942, 1000.000000000000000 ) ;
#22524=CARTESIAN_POINT ( 'NONE',  ( -35.00000000000000000, 11.24036214326520522, 6.018036132182202458 ) ) ;
#22525=LINE ( 'NONE', #32475, #28618 ) ;
#22527=VERTEX_POINT ( 'NONE', #60017 ) ;
#22528=DIRECTION ( 'NONE',  ( -1.000000000000000000, 0.000000000000000000, -0.000000000000000000 ) ) ;
#22530=AXIS2_PLACEMENT_3D ( 'NONE', #30190, #4932, #20205 ) ;
#22535=LINE ( 'NONE', #18203, #55291 ) ;
#22539=ORIENTED_EDGE ( 'NONE', *, *, #63879, .F. ) ;
#22540=LINE ( 'NONE', #63094, #28098 ) ;
#22542=CYLINDRICAL_SURFACE ( 'NONE', #11773, 5.000000000000000888 ) ;
#22543=DIRECTION ( 'NONE',  ( -1.000000000000000000, -0.000000000000000000, 0.000000000000000000 ) ) ;
#22545=EDGE_CURVE ( 'NONE', #17578, #9098, #16443, .T. ) ;
#22546=CIRCLE ( 'NONE', #13002, 12.18650000000000055 ) ;
#22547=VECTOR ( 'NONE', #19575, 1000.000000000000000 ) ;
#22548=ORIENTED_EDGE ( 'NONE', *, *, #29771, .T. ) ;
#22553=ORIENTED_EDGE ( 'NONE', *, *, #10424, .T. ) ;
#22556=CARTESIAN_POINT ( 'NONE',  ( 35.00000000000000000, -12.12087942037208776, 1.262958560998883595 ) ) ;
#22561=FACE_OUTER_BOUND ( 'NONE', #35634, .T. ) ;
#22563=ORIENTED_EDGE ( 'NONE', *, *, #40007, .T. ) ;
#22566=VECTOR ( 'NONE', #19197, 1000.000000000000000 ) ;
#22567=CARTESIAN_POINT ( 'NONE',  ( 21.48552864291340825, -12.93924674466299507, -3.871244808164612916 ) ) ;
#22568=CARTESIAN_POINT ( 'NONE',  ( -37.00000000000000711, 6.102719229070827645, -10.54834585426213422 ) ) ;
#22570=VERTEX_POINT ( 'NONE', #33739 ) ;
#22573=LINE ( 'NONE', #52521, #65781 ) ;
#22575=CIRCLE ( 'NONE', #59731, 5.000000000000000888 ) ;
#22576=ORIENTED_EDGE ( 'NONE', *, *, #40490, .F. ) ;
#22577=DIRECTION ( 'NONE',  ( 0.000000000000000000, 0.2006870767258819854, -0.9796553971857756560 ) ) ;
#22578=ORIENTED_EDGE ( 'NONE', *, *, #54484, .F. ) ;
#22579=ORIENTED_EDGE ( 'NONE', *, *, #51482, .F. ) ;
#22580=CARTESIAN_POINT ( 'NONE',  ( -37.00000000000000711, 0.000000000000000000, 0.000000000000000000 ) ) ;
#22583=DIRECTION ( 'NONE',  ( -1.000000000000000000, -1.836970198721029688E-16, 0.000000000000000000 ) ) ;
#22584=DIRECTION ( 'NONE',  ( 1.000000000000000000, -0.000000000000000000, 0.000000000000000000 ) ) ;
#22585=EDGE_CURVE ( 'NONE', #34249, #60329, #50428, .T. ) ;
#22586=CARTESIAN_POINT ( 'NONE',  ( -19.29830389789112033, -11.99999999999998757, -0.6550734076493088809 ) ) ;
#22587=CYLINDRICAL_SURFACE ( 'NONE', #45777, 12.75000000000000178 ) ;
#22588=CARTESIAN_POINT ( 'NONE',  ( 37.00000000000000711, 4.705694406421931860E-17, -3.469127814946512892E-15 ) ) ;
#22590=EDGE_CURVE ( 'NONE', #22391, #63878, #39058, .T. ) ;
#22592=LINE ( 'NONE', #27562, #32642 ) ;
#22596=CARTESIAN_POINT ( 'NONE',  ( -37.00000000000000711, 0.000000000000000000, 0.000000000000000000 ) ) ;
#22597=FACE_OUTER_BOUND ( 'NONE', #15760, .T. ) ;
#22600=AXIS2_PLACEMENT_3D ( 'NONE', #1386, #27957, #63504 ) ;
#22602=CIRCLE ( 'NONE', #9854, 4.999999999999999112 ) ;
#22604=ORIENTED_EDGE ( 'NONE', *, *, #38585, .F. ) ;
#22605=CARTESIAN_POINT ( 'NONE',  ( 37.00000000000000711, 2.080187960898562061, -12.57916205664482412 ) ) ;
#22609=CARTESIAN_POINT ( 'NONE',  ( 35.00000000000000000, -2.544412758415763864, 11.91791701451268715 ) ) ;
#22614=AXIS2_PLACEMENT_3D ( 'NONE', #17453, #31731, #57699 ) ;
#22616=CARTESIAN_POINT ( 'NONE',  ( -37.00000000000000711, 11.05394794832836958, -5.130401251914614491 ) ) ;
#22618=CARTESIAN_POINT ( 'NONE',  ( 26.25871678826176847, 11.49115831596999371, 3.460539353551113972 ) ) ;
#22619=EDGE_CURVE ( 'NONE', #20683, #23800, #15717, .T. ) ;
#22620=DIRECTION ( 'NONE',  ( 0.000000000000000000, -0.9246979985058680906, -0.3807014730195321661 ) ) ;
#22621=ORIENTED_EDGE ( 'NONE', *, *, #5431, .F. ) ;
#22622=AXIS2_PLACEMENT_3D ( 'NONE', #36305, #56610, #11682 ) ;
#22625=CYLINDRICAL_SURFACE ( 'NONE', #36317, 12.74999999999999822 ) ;
#22627=VERTEX_POINT ( 'NONE', #31388 ) ;
#22628=CARTESIAN_POINT ( 'NONE',  ( -9.345615655111398468, 10.52963412100725016, -8.456574980679686604 ) ) ;
#22629=EDGE_CURVE ( 'NONE', #55862, #13910, #10663, .T. ) ;
#22633=DIRECTION ( 'NONE',  ( 0.000000000000000000, 0.01356324068817998940, -0.9999080150203990547 ) ) ;
#22635=EDGE_CURVE ( 'NONE', #23433, #16276, #61048, .T. ) ;
#22640=AXIS2_PLACEMENT_3D ( 'NONE', #38423, #48424, #53733 ) ;
#22641=ORIENTED_EDGE ( 'NONE', *, *, #10552, .T. ) ;
#22642=ORIENTED_EDGE ( 'NONE', *, *, #34224, .F. ) ;
#22644=CIRCLE ( 'NONE', #21606, 14.99999999999998757 ) ;
#22646=CIRCLE ( 'NONE', #14127, 12.18650000000000055 ) ;
#22647=VERTEX_POINT ( 'NONE', #10768 ) ;
#22648=CYLINDRICAL_SURFACE ( 'NONE', #57013, 5.000000000000000888 ) ;
#22649=LINE ( 'NONE', #37924, #17253 ) ;
#22650=ORIENTED_EDGE ( 'NONE', *, *, #58258, .T. ) ;
#22651=DIRECTION ( 'NONE',  ( 0.000000000000000000, 0.01356324068817998940, -0.9999080150203990547 ) ) ;
#22654=ORIENTED_EDGE ( 'NONE', *, *, #63233, .T. ) ;
#22655=AXIS2_PLACEMENT_3D ( 'NONE', #60282, #45643, #9735 ) ;
#22656=ORIENTED_EDGE ( 'NONE', *, *, #9920, .T. ) ;
#22659=( LENGTH_UNIT ( ) NAMED_UNIT ( * ) SI_UNIT ( .MILLI., .METRE. ) );
#22661=CIRCLE ( 'NONE', #31143, 12.75000000000000178 ) ;
#22663=DIRECTION ( 'NONE',  ( 1.000000000000000000, 0.000000000000000000, 0.000000000000000000 ) ) ;
#22664=CIRCLE ( 'NONE', #5688, 12.74999999999999822 ) ;
#22666=FACE_OUTER_BOUND ( 'NONE', #50007, .T. ) ;
#22668=DIRECTION ( 'NONE',  ( 0.000000000000000000, -0.01356324068817998593, 0.9999080150203990547 ) ) ;
#22669=CARTESIAN_POINT ( 'NONE',  ( 3.720874945556317925, -10.52563386907497645, -5.765812798277466733 ) ) ;
#22671=CARTESIAN_POINT ( 'NONE',  ( -35.00000000000000000, 9.896810808925495806, -7.110831038798170134 ) ) ;
#22673=CIRCLE ( 'NONE', #52436, 12.18650000000000055 ) ;
#22674=ORIENTED_EDGE ( 'NONE', *, *, #32858, .F. ) ;
#22675=DIRECTION ( 'NONE',  ( -1.000000000000000000, 0.000000000000000000, -0.000000000000000000 ) ) ;
#22676=AXIS2_PLACEMENT_3D ( 'NONE', #40904, #44902, #65807 ) ;
#22677=DIRECTION ( 'NONE',  ( -1.000000000000000000, 0.000000000000000000, 0.000000000000000000 ) ) ;
#22683=EDGE_CURVE ( 'NONE', #39152, #41139, #11161, .T. ) ;
#22685=VERTEX_POINT ( 'NONE', #5481 ) ;
#22686=DIRECTION ( 'NONE',  ( 0.000000000000000000, 0.5767582926624911233, 0.8169148498130316405 ) ) ;
#22687=ORIENTED_EDGE ( 'NONE', *, *, #29117, .T. ) ;
#22688=DIRECTION ( 'NONE',  ( 0.000000000000000000, -0.01356324068817991828, 0.9999080150203990547 ) ) ;
#22689=DIRECTION ( 'NONE',  ( 1.000000000000000000, 0.000000000000000000, -0.000000000000000000 ) ) ;
#22690=CARTESIAN_POINT ( 'NONE',  ( -3.551075549032100653, -11.20694143114970309, 7.536131228641787416 ) ) ;
#22691=CYLINDRICAL_SURFACE ( 'NONE', #63973, 12.18650000000000055 ) ;
#22692=EDGE_CURVE ( 'NONE', #42026, #56480, #50611, .T. ) ;
#22693=ORIENTED_EDGE ( 'NONE', *, *, #62730, .F. ) ;
#22695=CIRCLE ( 'NONE', #29052, 5.000000000000000888 ) ;
#22696=DIRECTION ( 'NONE',  ( 1.000000000000000000, 0.000000000000000000, -0.000000000000000000 ) ) ;
#22697=EDGE_CURVE ( 'NONE', #22365, #28181, #20712, .T. ) ;
#22699=AXIS2_PLACEMENT_3D ( 'NONE', #1989, #63465, #43190 ) ;
#22700=CARTESIAN_POINT ( 'NONE',  ( 22.11485272451896122, 12.73694106385319635, -4.489087575610414937 ) ) ;
#22701=DIRECTION ( 'NONE',  ( 1.000000000000000000, 0.000000000000000000, -0.000000000000000000 ) ) ;
#22706=EDGE_CURVE ( 'NONE', #57602, #18732, #55736, .T. ) ;
#22707=AXIS2_PLACEMENT_3D ( 'NONE', #56992, #1125, #31687 ) ;
#22710=CARTESIAN_POINT ( 'NONE',  ( 6.191737802758098930, -8.543386553998011834, 10.45875730708377560 ) ) ;
#22711=VERTEX_POINT ( 'NONE', #15743 ) ;
#22712=CARTESIAN_POINT ( 'NONE',  ( -16.80711177628372610, 7.518039125045333115, -9.354561933223482839 ) ) ;
#22715=AXIS2_PLACEMENT_3D ( 'NONE', #42419, #26495, #46783 ) ;
#22718=VERTEX_POINT ( 'NONE', #56320 ) ;
#22720=ORIENTED_EDGE ( 'NONE', *, *, #18926, .T. ) ;
#22724=ORIENTED_EDGE ( 'NONE', *, *, #16739, .F. ) ;
#22727=DIRECTION ( 'NONE',  ( 0.000000000000000000, -1.000000000000000000, 0.000000000000000000 ) ) ;
#22729=VERTEX_POINT ( 'NONE', #22733 ) ;
#22732=LINE ( 'NONE', #42995, #46879 ) ;
#22733=CARTESIAN_POINT ( 'NONE',  ( -35.00000000000000000, 4.237620530777800987, 11.42599468261430928 ) ) ;
#22734=CARTESIAN_POINT ( 'NONE',  ( -24.45373054277663982, 7.205321492283886187, 9.606256275160440339 ) ) ;
#22735=EDGE_LOOP ( 'NONE', ( #44243, #52124, #55822, #62232 ) ) ;
#22736=CARTESIAN_POINT ( 'NONE',  ( -37.00000000000000711, -11.98254675519230084, 2.220215194441857331 ) ) ;
#22738=VECTOR ( 'NONE', #20307, 1000.000000000000000 ) ;
#22739=CARTESIAN_POINT ( 'NONE',  ( -18.45734883033349405, 13.50390945406918775, 0.07345776429000988594 ) ) ;
#22741=ORIENTED_EDGE ( 'NONE', *, *, #61191, .T. ) ;
#22742=DIRECTION ( 'NONE',  ( 0.000000000000000000, 0.01356324068817998940, -0.9999080150203990547 ) ) ;
#22743=DIRECTION ( 'NONE',  ( 0.000000000000000000, 0.000000000000000000, -1.000000000000000000 ) ) ;
#22745=AXIS2_PLACEMENT_3D ( 'NONE', #8073, #38653, #28342 ) ;
#22750=ORIENTED_EDGE ( 'NONE', *, *, #33177, .F. ) ;
#22752=CIRCLE ( 'NONE', #45002, 12.74999999999999822 ) ;
#22753=VERTEX_POINT ( 'NONE', #47352 ) ;
#22755=ORIENTED_EDGE ( 'NONE', *, *, #37954, .T. ) ;
#22756=EDGE_CURVE ( 'NONE', #59369, #50472, #18639, .T. ) ;
#22757=ORIENTED_EDGE ( 'NONE', *, *, #10118, .T. ) ;
#22758=AXIS2_PLACEMENT_3D ( 'NONE', #18095, #62982, #17444 ) ;
#22759=CARTESIAN_POINT ( 'NONE',  ( -35.00000000000000000, 11.42599468261435192, -4.237620530777677530 ) ) ;
#22765=CARTESIAN_POINT ( 'NONE',  ( -37.00000000000000711, 1.262958560998759472, 12.12087942037210198 ) ) ;
#22767=DIRECTION ( 'NONE',  ( 0.000000000000000000, -1.000000000000000000, 0.000000000000000000 ) ) ;
#22770=CARTESIAN_POINT ( 'NONE',  ( 35.00000000000000000, 7.561043153948098450, 9.557269938331469206 ) ) ;
#22775=CARTESIAN_POINT ( 'NONE',  ( 37.00000000000000711, 4.705694406421931860E-17, -3.469127814946512892E-15 ) ) ;
#22777=DIRECTION ( 'NONE',  ( 0.000000000000000000, -0.01356324068817999114, 0.9999080150203989437 ) ) ;
#22778=DIRECTION ( 'NONE',  ( -1.000000000000000000, 0.000000000000000000, 0.000000000000000000 ) ) ;
#22779=CARTESIAN_POINT ( 'NONE',  ( 11.55599502239090448, 0.7141290965170358218, -11.97894361706956978 ) ) ;
#22780=ORIENTED_EDGE ( 'NONE', *, *, #18112, .F. ) ;
#22783=CYLINDRICAL_SURFACE ( 'NONE', #55871, 12.74999999999999822 ) ;
#22785=AXIS2_PLACEMENT_3D ( 'NONE', #17136, #56386, #10834 ) ;
#22787=DIRECTION ( 'NONE',  ( 0.000000000000000000, -0.01356324068817998940, 0.9999080150203990547 ) ) ;
#22790=CARTESIAN_POINT ( 'NONE',  ( 17.38692437177838102, -10.06616489666143011, 6.600398882461584016 ) ) ;
#22796=DIRECTION ( 'NONE',  ( 0.000000000000000000, 0.4698238015817365332, 0.8827602140260315533 ) ) ;
#22797=ORIENTED_EDGE ( 'NONE', *, *, #10342, .F. ) ;
#22799=DIRECTION ( 'NONE',  ( -1.000000000000000000, 0.000000000000000000, -0.000000000000000000 ) ) ;
#22800=AXIS2_PLACEMENT_3D ( 'NONE', #2540, #22809, #42388 ) ;
#22803=ORIENTED_EDGE ( 'NONE', *, *, #42029, .T. ) ;
#22804=CARTESIAN_POINT ( 'NONE',  ( 35.00000000000000000, 11.72195762423409704, 0.7536123767498881243 ) ) ;
#22809=DIRECTION ( 'NONE',  ( -1.000000000000000000, 0.000000000000000000, 0.000000000000000000 ) ) ;
#22810=FACE_OUTER_BOUND ( 'NONE', #11340, .T. ) ;
#22812=CARTESIAN_POINT ( 'NONE',  ( 8.937200413558842982, 4.476360154859214902, 12.73625532737129795 ) ) ;
#22813=ORIENTED_EDGE ( 'NONE', *, *, #1355, .F. ) ;
#22814=CARTESIAN_POINT ( 'NONE',  ( 24.52288356478241482, -2.685886811157186749, -11.70110727047867805 ) ) ;
#22816=VERTEX_POINT ( 'NONE', #17412 ) ;
#22818=CARTESIAN_POINT ( 'NONE',  ( -27.27855387000350262, 12.26939275170278343, 5.631341004100471892 ) ) ;
#22823=DIRECTION ( 'NONE',  ( -1.000000000000000000, -0.000000000000000000, -0.000000000000000000 ) ) ;
#22826=EDGE_CURVE ( 'NONE', #9772, #27953, #33474, .T. ) ;
#22827=CYLINDRICAL_SURFACE ( 'NONE', #19150, 5.000000000000000888 ) ;
#22828=DIRECTION ( 'NONE',  ( 0.000000000000000000, -0.01356324068817998767, 0.9999080150203990547 ) ) ;
#22829=ORIENTED_EDGE ( 'NONE', *, *, #51808, .F. ) ;
#22833=ORIENTED_EDGE ( 'NONE', *, *, #54836, .T. ) ;
#22835=CARTESIAN_POINT ( 'NONE',  ( -37.00000000000000711, 0.000000000000000000, 0.000000000000000000 ) ) ;
#22836=CARTESIAN_POINT ( 'NONE',  ( 8.937200413559450496, 4.243630616744383133, 12.81805183698073947 ) ) ;
#22838=CARTESIAN_POINT ( 'NONE',  ( -35.00000000000000000, 0.000000000000000000, 0.000000000000000000 ) ) ;
#22839=CARTESIAN_POINT ( 'NONE',  ( -29.14293782047111847, 1.979001771404295784, 13.38056321518360292 ) ) ;
#22840=EDGE_CURVE ( 'NONE', #1587, #64727, #22852, .T. ) ;
#22843=DIRECTION ( 'NONE',  ( 0.000000000000000000, -0.01356324068817998940, 0.9999080150203990547 ) ) ;
#22847=LINE ( 'NONE', #52770, #29970 ) ;
#22848=CARTESIAN_POINT ( 'NONE',  ( 35.00000000000000000, 4.705694406421931860E-17, -3.469127814946512892E-15 ) ) ;
#22851=FACE_OUTER_BOUND ( 'NONE', #34409, .T. ) ;
#22852=CIRCLE ( 'NONE', #23903, 4.999999999999999112 ) ;
#22854=ORIENTED_EDGE ( 'NONE', *, *, #40900, .T. ) ;
#22856=EDGE_CURVE ( 'NONE', #10868, #11758, #16433, .T. ) ;
#22858=DIRECTION ( 'NONE',  ( 0.000000000000000000, -0.4134677391718577510, -0.9105187689795923855 ) ) ;
#22859=DIRECTION ( 'NONE',  ( 0.000000000000000000, 0.01356324068817998940, -0.9999080150203990547 ) ) ;
#22861=CARTESIAN_POINT ( 'NONE',  ( -37.00000000000000711, 0.000000000000000000, 0.000000000000000000 ) ) ;
#22863=ORIENTED_EDGE ( 'NONE', *, *, #10014, .T. ) ;
#22865=CARTESIAN_POINT ( 'NONE',  ( 17.95036338764469619, 10.25346347048778739, 8.788876757364576520 ) ) ;
#22866=CARTESIAN_POINT ( 'NONE',  ( -29.65781431629226361, -0.5515374799640114789, -13.49546472197990532 ) ) ;
#22868=CIRCLE ( 'NONE', #21787, 5.000000000000000888 ) ;
#22870=CARTESIAN_POINT ( 'NONE',  ( -37.00000000000000711, 8.146229107149400406, 9.063649021438985542 ) ) ;
#22874=CARTESIAN_POINT ( 'NONE',  ( 35.00000000000000000, 4.705694406421931860E-17, -3.469127814946512892E-15 ) ) ;
#22875=ORIENTED_EDGE ( 'NONE', *, *, #6546, .T. ) ;
#22876=DIRECTION ( 'NONE',  ( 1.000000000000000000, 0.000000000000000000, 0.000000000000000000 ) ) ;
#22878=CARTESIAN_POINT ( 'NONE',  ( -37.00000000000000711, 12.08216339958900676, 1.591260454995285789 ) ) ;
#22881=ADVANCED_FACE ( 'NONE', ( #33992 ), #54306, .T. ) ;
#22883=ORIENTED_EDGE ( 'NONE', *, *, #45577, .T. ) ;
#22885=ORIENTED_EDGE ( 'NONE', *, *, #64119, .T. ) ;
#22887=DIRECTION ( 'NONE',  ( -1.000000000000000000, 0.000000000000000000, -0.000000000000000000 ) ) ;
#22889=DIRECTION ( 'NONE',  ( -0.000000000000000000, -0.000000000000000000, -1.000000000000000000 ) ) ;
#22890=DIRECTION ( 'NONE',  ( -0.000000000000000000, -1.000000000000000000, -0.000000000000000000 ) ) ;
#22892=DIRECTION ( 'NONE',  ( 0.000000000000000000, -0.8369827122275401710, -0.5472293298355185298 ) ) ;
#22894=VERTEX_POINT ( 'NONE', #44299 ) ;
#22895=EDGE_CURVE ( 'NONE', #55534, #2111, #36652, .T. ) ;
#22896=DIRECTION ( 'NONE',  ( 0.000000000000000000, 0.01356324068818000328, -0.9999080150203990547 ) ) ;
#22897=ORIENTED_EDGE ( 'NONE', *, *, #6171, .T. ) ;
#22898=AXIS2_PLACEMENT_3D ( 'NONE', #44379, #34724, #23465 ) ;
#22901=EDGE_CURVE ( 'NONE', #53784, #62115, #7734, .T. ) ;
#22902=CARTESIAN_POINT ( 'NONE',  ( 35.00000000000000000, 7.971186206369472060, -9.217970097227754067 ) ) ;
#22903=ORIENTED_EDGE ( 'NONE', *, *, #31967, .F. ) ;
#22907=ORIENTED_EDGE ( 'NONE', *, *, #29784, .T. ) ;
#22908=ORIENTED_EDGE ( 'NONE', *, *, #30287, .F. ) ;
#22910=ADVANCED_FACE ( 'NONE', ( #43315 ), #53654, .T. ) ;
#22911=EDGE_LOOP ( 'NONE', ( #12613, #20328, #49494, #49657 ) ) ;
#22913=EDGE_LOOP ( 'NONE', ( #24258, #55285, #34126, #41826 ) ) ;
#22914=VERTEX_POINT ( 'NONE', #43645 ) ;
#22917=AXIS2_PLACEMENT_3D ( 'NONE', #41811, #47151, #62104 ) ;
#22918=FACE_OUTER_BOUND ( 'NONE', #22356, .T. ) ;
#22920=DIRECTION ( 'NONE',  ( 0.000000000000000000, 0.8989688749565173387, 0.4380125133593943398 ) ) ;
#22922=( BOUNDED_CURVE ( )  B_SPLINE_CURVE ( 3, ( #54363, #28104, #18118, #48397 ),
 .UNSPECIFIED., .F., .F. ) 
 B_SPLINE_CURVE_WITH_KNOTS ( ( 4, 4 ),
 ( 6.141081411243264121, 6.425289203115908343 ),
 .UNSPECIFIED. ) 
 CURVE ( )  GEOMETRIC_REPRESENTATION_ITEM ( )  RATIONAL_B_SPLINE_CURVE ( ( 1.000000000000000000, 0.9932801471353227551, 0.9932801471353227551, 1.000000000000000000 ) ) 
 REPRESENTATION_ITEM ( '' )  );
#22923=EDGE_LOOP ( 'NONE', ( #23286, #37709, #18529, #32208 ) ) ;
#22925=EDGE_CURVE ( 'NONE', #1336, #7715, #19225, .T. ) ;
#22928=ADVANCED_FACE ( 'NONE', ( #64263 ), #23055, .F. ) ;
#22933=CARTESIAN_POINT ( 'NONE',  ( -35.00000000000000000, -8.927548052240956267, 8.295159312811819063 ) ) ;
#22935=ADVANCED_FACE ( 'NONE', ( #3114 ), #23376, .T. ) ;
#22937=LINE ( 'NONE', #62483, #2539 ) ;
#22938=EDGE_CURVE ( 'NONE', #44205, #62469, #9029, .T. ) ;
#22940=( BOUNDED_CURVE ( )  B_SPLINE_CURVE ( 3, ( #61105, #51486, #5932, #4931 ),
 .UNSPECIFIED., .F., .F. ) 
 B_SPLINE_CURVE_WITH_KNOTS ( ( 4, 4 ),
 ( 0.5962944384795770825, 0.6311393659967107217 ),
 .UNSPECIFIED. ) 
 CURVE ( )  GEOMETRIC_REPRESENTATION_ITEM ( )  RATIONAL_B_SPLINE_CURVE ( ( 1.000000000000000000, 0.9998988218115538729, 0.9998988218115538729, 1.000000000000000000 ) ) 
 REPRESENTATION_ITEM ( '' )  );
#22944=CARTESIAN_POINT ( 'NONE',  ( 12.14692673679996737, -13.20602977273170175, -2.806489945550152854 ) ) ;
#22945=EDGE_CURVE ( 'NONE', #64097, #7860, #34329, .T. ) ;
#22948=ORIENTED_EDGE ( 'NONE', *, *, #14154, .F. ) ;
#22949=DIRECTION ( 'NONE',  ( 0.000000000000000000, -0.01356324068817991828, 0.9999080150203990547 ) ) ;
#22950=DIRECTION ( 'NONE',  ( 0.000000000000000000, 0.8696919319575165952, 0.4935949184179292404 ) ) ;
#22952=DIRECTION ( 'NONE',  ( -1.000000000000000000, 0.000000000000000000, 0.000000000000000000 ) ) ;
#22953=AXIS2_PLACEMENT_3D ( 'NONE', #59961, #59627, #14053 ) ;
#22954=LINE ( 'NONE', #63811, #34995 ) ;
#22955=ORIENTED_EDGE ( 'NONE', *, *, #21624, .T. ) ;
#22956=DIRECTION ( 'NONE',  ( 1.000000000000000000, 0.000000000000000000, -0.000000000000000000 ) ) ;
#22959=EDGE_CURVE ( 'NONE', #61226, #57314, #728, .T. ) ;
#22960=ORIENTED_EDGE ( 'NONE', *, *, #40864, .T. ) ;
#22961=CARTESIAN_POINT ( 'NONE',  ( 2.354167843600960097, -6.278647867796540716, 25.00000000000000000 ) ) ;
#22963=DIRECTION ( 'NONE',  ( -1.000000000000000000, 0.000000000000000000, 0.000000000000000000 ) ) ;
#22966=DIRECTION ( 'NONE',  ( 0.000000000000000000, 0.01356324068817998940, -0.9999080150203990547 ) ) ;
#22968=VERTEX_POINT ( 'NONE', #20342 ) ;
#22969=EDGE_CURVE ( 'NONE', #10113, #19062, #56847, .T. ) ;
#22971=EDGE_LOOP ( 'NONE', ( #46178, #7056, #43470, #64652 ) ) ;
#22973=CARTESIAN_POINT ( 'NONE',  ( 35.00000000000000000, 4.705694406421931860E-17, -3.469127814946512892E-15 ) ) ;
#22974=ORIENTED_EDGE ( 'NONE', *, *, #12161, .T. ) ;
#22975=CIRCLE ( 'NONE', #59060, 12.18649999999999878 ) ;
#22976=CARTESIAN_POINT ( 'NONE',  ( 145.1370849898475797, 3.309064568108273190E-14, 0.000000000000000000 ) ) ;
#22978=ORIENTED_EDGE ( 'NONE', *, *, #61348, .F. ) ;
#22979=VECTOR ( 'NONE', #37318, 1000.000000000000000 ) ;
#22981=FACE_OUTER_BOUND ( 'NONE', #37794, .T. ) ;
#22983=ORIENTED_EDGE ( 'NONE', *, *, #35744, .F. ) ;
#22985=ADVANCED_FACE ( 'NONE', ( #34640 ), #35298, .T. ) ;
#22986=ORIENTED_EDGE ( 'NONE', *, *, #45621, .T. ) ;
#22987=ORIENTED_EDGE ( 'NONE', *, *, #43142, .F. ) ;
#22989=EDGE_CURVE ( 'NONE', #42463, #21230, #65310, .T. ) ;
#22991=DIRECTION ( 'NONE',  ( 1.000000000000000000, 0.000000000000000000, 0.000000000000000000 ) ) ;
#22992=DIRECTION ( 'NONE',  ( -1.000000000000000000, 0.000000000000000000, 0.000000000000000000 ) ) ;
#22993=CARTESIAN_POINT ( 'NONE',  ( 35.00000000000000000, -8.830544224263011444, -9.196955404009264257 ) ) ;
#22994=CYLINDRICAL_SURFACE ( 'NONE', #23896, 5.000000000000000888 ) ;
#22995=CARTESIAN_POINT ( 'NONE',  ( -27.58700550753028224, -9.955571130810017877, -6.705838893603189632 ) ) ;
#22996=ORIENTED_EDGE ( 'NONE', *, *, #56579, .T. ) ;
#23001=ORIENTED_EDGE ( 'NONE', *, *, #59024, .F. ) ;
#23007=VERTEX_POINT ( 'NONE', #26003 ) ;
#23009=ADVANCED_FACE ( 'NONE', ( #40957 ), #25330, .T. ) ;
#23011=ORIENTED_EDGE ( 'NONE', *, *, #58192, .F. ) ;
#23013=DIRECTION ( 'NONE',  ( 0.000000000000000000, 0.3218879778915905154, -0.9467777615094595811 ) ) ;
#23015=ADVANCED_FACE ( 'NONE', ( #54936 ), #46287, .T. ) ;
#23017=CARTESIAN_POINT ( 'NONE',  ( -18.25006854224444908, -9.443202773001939221, 7.404452808139724063 ) ) ;
#23019=CIRCLE ( 'NONE', #57006, 5.000000000000000888 ) ;
#23022=EDGE_CURVE ( 'NONE', #11696, #28136, #8000, .T. ) ;
#23026=DIRECTION ( 'NONE',  ( 1.000000000000000000, -0.000000000000000000, 0.000000000000000000 ) ) ;
#23027=CARTESIAN_POINT ( 'NONE',  ( 6.507052240825795586, -8.968520638857693683, -7.975644518742436517 ) ) ;
#23033=EDGE_CURVE ( 'NONE', #12853, #53880, #43006, .T. ) ;
#23036=DIRECTION ( 'NONE',  ( 1.000000000000000000, 0.000000000000000000, 0.000000000000000000 ) ) ;
#23039=LINE ( 'NONE', #27350, #41559 ) ;
#23040=VERTEX_POINT ( 'NONE', #45607 ) ;
#23041=CARTESIAN_POINT ( 'NONE',  ( -36.00000000000000711, -0.9416912585473466990, -12.71517666308949046 ) ) ;
#23042=EDGE_CURVE ( 'NONE', #54738, #22141, #53664, .T. ) ;
#23043=ORIENTED_EDGE ( 'NONE', *, *, #60890, .F. ) ;
#23044=ORIENTED_EDGE ( 'NONE', *, *, #11568, .T. ) ;
#23047=ORIENTED_EDGE ( 'NONE', *, *, #39112, .F. ) ;
#23051=FACE_OUTER_BOUND ( 'NONE', #41012, .T. ) ;
#23052=ORIENTED_EDGE ( 'NONE', *, *, #26876, .T. ) ;
#23055=CYLINDRICAL_SURFACE ( 'NONE', #64228, 14.19297241773857188 ) ;
#23059=ADVANCED_FACE ( 'NONE', ( #15663 ), #50303, .T. ) ;
#23060=ADVANCED_FACE ( 'NONE', ( #45290 ), #30970, .T. ) ;
#23061=EDGE_LOOP ( 'NONE', ( #9207, #22693, #53401, #43485 ) ) ;
#23062=CARTESIAN_POINT ( 'NONE',  ( -18.00215407324301964, 13.42696834491351154, 1.444777302739133296 ) ) ;
#23063=ORIENTED_EDGE ( 'NONE', *, *, #30117, .F. ) ;
#23064=AXIS2_PLACEMENT_3D ( 'NONE', #54231, #14301, #28617 ) ;
#23066=DIRECTION ( 'NONE',  ( 1.000000000000000000, 0.000000000000000000, 0.000000000000000000 ) ) ;
#23067=EDGE_CURVE ( 'NONE', #60414, #7557, #50478, .T. ) ;
#23068=DIRECTION ( 'NONE',  ( 0.000000000000000000, -0.01356324068817999114, 0.9999080150203989437 ) ) ;
#23069=CARTESIAN_POINT ( 'NONE',  ( 37.00000000000000711, -7.474872387601069867, -9.060822531526026680 ) ) ;
#23073=ORIENTED_EDGE ( 'NONE', *, *, #16660, .F. ) ;
#23074=DIRECTION ( 'NONE',  ( 1.000000000000000000, 0.000000000000000000, 0.000000000000000000 ) ) ;
#23084=CARTESIAN_POINT ( 'NONE',  ( 37.00000000000000711, -8.551552972817137999, -8.052525312709853722 ) ) ;
#23085=VERTEX_POINT ( 'NONE', #36284 ) ;
#23086=CARTESIAN_POINT ( 'NONE',  ( 37.00000000000000711, 7.215058775251253387, -9.821084925794595577 ) ) ;
#23091=DIRECTION ( 'NONE',  ( 0.000000000000000000, -0.01356324068817998940, 0.9999080150203990547 ) ) ;
#23092=CARTESIAN_POINT ( 'NONE',  ( 9.268253959421528521, 2.865053375548464398, -11.65528265421164811 ) ) ;
#23093=ORIENTED_EDGE ( 'NONE', *, *, #47364, .T. ) ;
#23095=CARTESIAN_POINT ( 'NONE',  ( -35.00000000000000000, 10.64792938439755332, 5.927257550915355999 ) ) ;
#23098=CIRCLE ( 'NONE', #5035, 12.74999999999999822 ) ;
#23099=CARTESIAN_POINT ( 'NONE',  ( 37.00000000000000711, 9.700295462048767803, 7.376655759824772396 ) ) ;
#23101=ADVANCED_FACE ( 'NONE', ( #16990 ), #57242, .T. ) ;
#23103=ORIENTED_EDGE ( 'NONE', *, *, #53839, .F. ) ;
#23105=CARTESIAN_POINT ( 'NONE',  ( -35.00000000000000000, 4.725891942574755866, 10.75351884295729477 ) ) ;
#23107=ORIENTED_EDGE ( 'NONE', *, *, #38757, .T. ) ;
#23109=DIRECTION ( 'NONE',  ( 0.000000000000000000, 0.01356324068817991828, -0.9999080150203990547 ) ) ;
#23111=ORIENTED_EDGE ( 'NONE', *, *, #65051, .F. ) ;
#23113=ADVANCED_FACE ( 'NONE', ( #57579 ), #6706, .T. ) ;
#23114=EDGE_LOOP ( 'NONE', ( #9316, #46498, #37679, #40366 ) ) ;
#23115=CARTESIAN_POINT ( 'NONE',  ( -35.00000000000000000, 7.745827850123011338, 10.12742074351899291 ) ) ;
#23118=CARTESIAN_POINT ( 'NONE',  ( 35.00000000000000000, 11.71932350927024657, -3.511386971104992760 ) ) ;
#23119=DIRECTION ( 'NONE',  ( 0.000000000000000000, -0.01356324068817999114, 0.9999080150203989437 ) ) ;
#23122=ORIENTED_EDGE ( 'NONE', *, *, #41970, .F. ) ;
#23124=EDGE_CURVE ( 'NONE', #20489, #65370, #11210, .T. ) ;
#23126=LINE ( 'NONE', #33436, #63554 ) ;
#23127=ORIENTED_EDGE ( 'NONE', *, *, #44434, .T. ) ;
#23130=CARTESIAN_POINT ( 'NONE',  ( -16.31771647384731949, 8.296044977521708219, 10.65025654402225364 ) ) ;
#23132=VECTOR ( 'NONE', #20922, 1000.000000000000000 ) ;
#23133=CARTESIAN_POINT ( 'NONE',  ( -25.06408389988974150, 11.89233385548744693, 6.391198624005284934 ) ) ;
#23134=CARTESIAN_POINT ( 'NONE',  ( 22.57855258442565116, 3.026812727784649493, 11.61199400236328749 ) ) ;
#23136=LINE ( 'NONE', #53414, #14985 ) ;
#23137=ORIENTED_EDGE ( 'NONE', *, *, #33420, .F. ) ;
#23138=AXIS2_PLACEMENT_3D ( 'NONE', #7878, #27817, #53435 ) ;
#23141=DIRECTION ( 'NONE',  ( 0.000000000000000000, -0.01356324068817998940, 0.9999080150203990547 ) ) ;
#23142=VERTEX_POINT ( 'NONE', #26983 ) ;
#23146=DIRECTION ( 'NONE',  ( 1.000000000000000000, 0.000000000000000000, 0.000000000000000000 ) ) ;
#23147=VECTOR ( 'NONE', #7436, 1000.000000000000000 ) ;
#23149=LINE ( 'NONE', #59073, #10801 ) ;
#23151=DIRECTION ( 'NONE',  ( -1.000000000000000000, 0.000000000000000000, 0.000000000000000000 ) ) ;
#23153=VECTOR ( 'NONE', #61083, 1000.000000000000000 ) ;
#23154=DIRECTION ( 'NONE',  ( -1.000000000000000000, 0.000000000000000000, 0.000000000000000000 ) ) ;
#23155=ORIENTED_EDGE ( 'NONE', *, *, #8866, .F. ) ;
#23156=CARTESIAN_POINT ( 'NONE',  ( -35.00000000000000000, -12.18632975068352842, -0.06441628369849203284 ) ) ;
#23157=EDGE_LOOP ( 'NONE', ( #20802, #7332, #327, #25116 ) ) ;
#23159=EDGE_CURVE ( 'NONE', #27199, #56769, #55300, .T. ) ;
#23161=CARTESIAN_POINT ( 'NONE',  ( 35.00000000000000000, -0.06441628369827803735, 12.18632975068352309 ) ) ;
#23162=ADVANCED_FACE ( 'NONE', ( #41931 ), #62216, .T. ) ;
#23164=CARTESIAN_POINT ( 'NONE',  ( 47.00000000000000711, 4.705694406421931860E-17, -3.469127814946512892E-15 ) ) ;
#23165=ORIENTED_EDGE ( 'NONE', *, *, #33733, .F. ) ;
#23169=CARTESIAN_POINT ( 'NONE',  ( 35.00000000000000000, -8.854740511458901508, -7.717887834988215623 ) ) ;
#23170=VERTEX_POINT ( 'NONE', #47278 ) ;
#23173=FACE_OUTER_BOUND ( 'NONE', #44092, .T. ) ;
#23175=CARTESIAN_POINT ( 'NONE',  ( 37.00000000000000711, 11.73555825188276280, -4.983891302653623789 ) ) ;
#23176=CIRCLE ( 'NONE', #61417, 12.75000000000000178 ) ;
#23177=ADVANCED_FACE ( 'NONE', ( #33607 ), #59528, .T. ) ;
#23179=CARTESIAN_POINT ( 'NONE',  ( -37.00000000000000711, 10.92721691015462149, -4.309077947445535628 ) ) ;
#23180=AXIS2_PLACEMENT_3D ( 'NONE', #62833, #22952, #11638 ) ;
#23181=VECTOR ( 'NONE', #60667, 1000.000000000000000 ) ;
#23182=EDGE_CURVE ( 'NONE', #14607, #35879, #59212, .T. ) ;
#23183=ORIENTED_EDGE ( 'NONE', *, *, #10293, .F. ) ;
#23186=ORIENTED_EDGE ( 'NONE', *, *, #45109, .T. ) ;
#23187=VECTOR ( 'NONE', #26414, 1000.000000000000000 ) ;
#23190=DIRECTION ( 'NONE',  ( 0.000000000000000000, 0.01356324068817992522, -0.9999080150203990547 ) ) ;
#23191=DIRECTION ( 'NONE',  ( -0.000000000000000000, -0.000000000000000000, -1.000000000000000000 ) ) ;
#23193=CARTESIAN_POINT ( 'NONE',  ( 35.00000000000000000, 4.705694406421931860E-17, -3.469127814946512892E-15 ) ) ;
#23196=ORIENTED_EDGE ( 'NONE', *, *, #52870, .T. ) ;
#23197=DIRECTION ( 'NONE',  ( 1.000000000000000000, -0.000000000000000000, 0.000000000000000000 ) ) ;
#23199=CARTESIAN_POINT ( 'NONE',  ( 16.78263030916553333, -10.48479066935623827, 5.836879698929882565 ) ) ;
#23204=EDGE_CURVE ( 'NONE', #57229, #62196, #12641, .T. ) ;
#23208=EDGE_LOOP ( 'NONE', ( #41157, #39555, #35719, #23730 ) ) ;
#23210=ORIENTED_EDGE ( 'NONE', *, *, #42387, .T. ) ;
#23212=LINE ( 'NONE', #8247, #30033 ) ;
#23215=LINE ( 'NONE', #58824, #52140 ) ;
#23216=VERTEX_POINT ( 'NONE', #23635 ) ;
#23219=AXIS2_PLACEMENT_3D ( 'NONE', #47764, #37112, #11844 ) ;
#23220=DIRECTION ( 'NONE',  ( 0.000000000000000000, 0.8169148498130297531, -0.5767582926624941209 ) ) ;
#23222=ORIENTED_EDGE ( 'NONE', *, *, #11874, .T. ) ;
#23224=ORIENTED_EDGE ( 'NONE', *, *, #45884, .T. ) ;
#23225=CARTESIAN_POINT ( 'NONE',  ( -35.00000000000000000, 10.14433819232434253, 6.753013023069750709 ) ) ;
#23230=AXIS2_PLACEMENT_3D ( 'NONE', #53432, #32771, #23482 ) ;
#23233=DIRECTION ( 'NONE',  ( -1.000000000000000000, 0.000000000000000000, 0.000000000000000000 ) ) ;
#23234=CIRCLE ( 'NONE', #12621, 4.999999999999999112 ) ;
#23235=AXIS2_PLACEMENT_3D ( 'NONE', #53242, #17339, #33612 ) ;
#23240=CYLINDRICAL_SURFACE ( 'NONE', #58275, 4.999999999999999112 ) ;
#23241=CARTESIAN_POINT ( 'NONE',  ( 27.85039655636127875, 11.11615754980423176, 4.533728555765254242 ) ) ;
#23245=FACE_OUTER_BOUND ( 'NONE', #56508, .T. ) ;
#23247=ORIENTED_EDGE ( 'NONE', *, *, #64470, .T. ) ;
#23249=ORIENTED_EDGE ( 'NONE', *, *, #56323, .T. ) ;
#23250=CARTESIAN_POINT ( 'NONE',  ( 37.00000000000000711, -7.971186206369407223, 9.217970097227803805 ) ) ;
#23252=CARTESIAN_POINT ( 'NONE',  ( 11.02943363989745684, -13.39302490721040151, -1.700353917502927859 ) ) ;
#23255=ORIENTED_EDGE ( 'NONE', *, *, #54154, .T. ) ;
#23258=DIRECTION ( 'NONE',  ( 0.000000000000000000, -0.6745969609292717939, -0.7381862504171901040 ) ) ;
#23259=CARTESIAN_POINT ( 'NONE',  ( -35.00000000000000000, 1.771820996347319710, -11.61175578952784448 ) ) ;
#23261=CIRCLE ( 'NONE', #33883, 12.75000000000000178 ) ;
#23263=CARTESIAN_POINT ( 'NONE',  ( -4.989057617119008192, -0.9162120371760335003, -13.46887357958837406 ) ) ;
#23264=ORIENTED_EDGE ( 'NONE', *, *, #29345, .T. ) ;
#23265=CIRCLE ( 'NONE', #3112, 5.000000000000000888 ) ;
#23266=EDGE_CURVE ( 'NONE', #65690, #54019, #3792, .T. ) ;
#23268=EDGE_CURVE ( 'NONE', #55634, #47275, #18664, .T. ) ;
#23271=EDGE_LOOP ( 'NONE', ( #22948, #30966, #16916, #10558 ) ) ;
#23273=LINE ( 'NONE', #53209, #63641 ) ;
#23274=CIRCLE ( 'NONE', #33898, 5.000000000000001776 ) ;
#23275=ORIENTED_EDGE ( 'NONE', *, *, #19749, .F. ) ;
#23276=CYLINDRICAL_SURFACE ( 'NONE', #4326, 12.18649999999999878 ) ;
#23279=DIRECTION ( 'NONE',  ( 1.000000000000000000, 0.000000000000000000, -0.000000000000000000 ) ) ;
#23283=EDGE_CURVE ( 'NONE', #27444, #59695, #63225, .T. ) ;
#23284=VERTEX_POINT ( 'NONE', #32923 ) ;
#23285=AXIS2_PLACEMENT_3D ( 'NONE', #59720, #14148, #34440 ) ;
#23286=ORIENTED_EDGE ( 'NONE', *, *, #1493, .F. ) ;
#23287=DIRECTION ( 'NONE',  ( 1.000000000000000000, 0.000000000000000000, 0.000000000000000000 ) ) ;
#23289=B_SPLINE_CURVE_WITH_KNOTS ( 'NONE', 3,
 ( #16813, #58051, #51759, #37090, #32427, #1212, #6202, #12466, #26464, #46750, #57390, #11817, #52417, #27130, #47427, #47739 ),
 .UNSPECIFIED., .F., .F.,
 ( 4, 2, 2, 2, 2, 2, 2, 4 ),
 ( 0.000000000000000000, 0.001204540821560086709, 0.002409081643120173418, 0.003613622464680259910, 0.004818163286240346836, 0.007227244929360519821, 0.008431785750920607614, 0.009636326572480693672 ),
 .UNSPECIFIED. ) ;
#23290=DIRECTION ( 'NONE',  ( -1.000000000000000000, 0.000000000000000000, 0.000000000000000000 ) ) ;
#23291=ORIENTED_EDGE ( 'NONE', *, *, #57289, .T. ) ;
#23292=DIRECTION ( 'NONE',  ( -1.000000000000000000, 0.000000000000000000, 0.000000000000000000 ) ) ;
#23293=EDGE_CURVE ( 'NONE', #54167, #64126, #27966, .T. ) ;
#23295=ORIENTED_EDGE ( 'NONE', *, *, #53276, .T. ) ;
#23296=( BOUNDED_CURVE ( )  B_SPLINE_CURVE ( 3, ( #65510, #54600, #9024, #23680 ),
 .UNSPECIFIED., .F., .F. ) 
 B_SPLINE_CURVE_WITH_KNOTS ( ( 4, 4 ),
 ( 1.254278954140350288, 1.289274629942205985 ),
 .UNSPECIFIED. ) 
 CURVE ( )  GEOMETRIC_REPRESENTATION_ITEM ( )  RATIONAL_B_SPLINE_CURVE ( ( 1.000000000000000000, 0.9998979444935354177, 0.9998979444935354177, 1.000000000000000000 ) ) 
 REPRESENTATION_ITEM ( '' )  );
#23299=CARTESIAN_POINT ( 'NONE',  ( -37.00000000000000711, 0.000000000000000000, 0.000000000000000000 ) ) ;
#23301=ORIENTED_EDGE ( 'NONE', *, *, #44113, .T. ) ;
#23303=DIRECTION ( 'NONE',  ( 0.000000000000000000, -0.8009703041134103030, -0.5987040770935764256 ) ) ;
#23304=ORIENTED_EDGE ( 'NONE', *, *, #44799, .F. ) ;
#23305=CARTESIAN_POINT ( 'NONE',  ( -47.00000000000000711, 0.000000000000000000, 0.000000000000000000 ) ) ;
#23310=AXIS2_PLACEMENT_3D ( 'NONE', #39770, #3888, #63712 ) ;
#23311=DIRECTION ( 'NONE',  ( -1.000000000000000000, 0.000000000000000000, -0.000000000000000000 ) ) ;
#23313=FACE_OUTER_BOUND ( 'NONE', #44160, .T. ) ;
#23314=ORIENTED_EDGE ( 'NONE', *, *, #11714, .F. ) ;
#23315=CARTESIAN_POINT ( 'NONE',  ( -37.00000000000000711, 10.28547182238008162, 5.672855678558722303 ) ) ;
#23318=LINE ( 'NONE', #33936, #32744 ) ;
#23320=ORIENTED_EDGE ( 'NONE', *, *, #61590, .F. ) ;
#23321=CARTESIAN_POINT ( 'NONE',  ( 24.90079489126682688, 10.54408982692485530, -8.432554294912229409 ) ) ;
#23325=VERTEX_POINT ( 'NONE', #34248 ) ;
#23326=EDGE_CURVE ( 'NONE', #35454, #61571, #46258, .T. ) ;
#23327=ORIENTED_EDGE ( 'NONE', *, *, #42456, .F. ) ;
#23328=CARTESIAN_POINT ( 'NONE',  ( 35.00000000000000000, 4.705694406421931860E-17, -3.469127814946512892E-15 ) ) ;
#23329=CIRCLE ( 'NONE', #54131, 12.74999999999999822 ) ;
#23330=ORIENTED_EDGE ( 'NONE', *, *, #20063, .T. ) ;
#23331=CARTESIAN_POINT ( 'NONE',  ( -26.43107551473783090, -12.39219842031925012, 5.356174113667619530 ) ) ;
#23332=DIRECTION ( 'NONE',  ( 0.000000000000000000, 0.8827602140260297769, -0.4698238015817396418 ) ) ;
#23333=CARTESIAN_POINT ( 'NONE',  ( 35.00000000000000000, 4.705694406421931860E-17, -3.469127814946512892E-15 ) ) ;
#23334=CARTESIAN_POINT ( 'NONE',  ( -3.456237872026009850, 8.328074767851541438, 8.678162217191049521 ) ) ;
#23335=CARTESIAN_POINT ( 'NONE',  ( 37.00000000000000711, 11.53507381115583108, 2.216820770815121744 ) ) ;
#23336=ORIENTED_EDGE ( 'NONE', *, *, #18100, .T. ) ;
#23337=EDGE_CURVE ( 'NONE', #2788, #31673, #2750, .T. ) ;
#23338=CIRCLE ( 'NONE', #52010, 5.000000000000000000 ) ;
#23345=CARTESIAN_POINT ( 'NONE',  ( -19.69476066079020171, -4.201994156881551312, 25.00000000000000000 ) ) ;
#23352=CYLINDRICAL_SURFACE ( 'NONE', #42701, 12.18649999999999878 ) ;
#23353=CIRCLE ( 'NONE', #60518, 5.000000000000000888 ) ;
#23354=CYLINDRICAL_SURFACE ( 'NONE', #22745, 12.18649999999999878 ) ;
#23355=FACE_OUTER_BOUND ( 'NONE', #33478, .T. ) ;
#23357=DIRECTION ( 'NONE',  ( 1.000000000000000000, 0.000000000000000000, -0.000000000000000000 ) ) ;
#23358=CARTESIAN_POINT ( 'NONE',  ( 35.00000000000000000, 12.16632754454236398, -0.7008968033239244555 ) ) ;
#23360=ORIENTED_EDGE ( 'NONE', *, *, #55111, .F. ) ;
#23361=ORIENTED_EDGE ( 'NONE', *, *, #30900, .T. ) ;
#23362=CARTESIAN_POINT ( 'NONE',  ( 29.28325686113022641, -11.61404609382441855, 6.885459852046807327 ) ) ;
#23363=EDGE_CURVE ( 'NONE', #33997, #32649, #48966, .T. ) ;
#23364=AXIS2_PLACEMENT_3D ( 'NONE', #4901, #28845, #40445 ) ;
#23366=ORIENTED_EDGE ( 'NONE', *, *, #48885, .T. ) ;
#23369=CARTESIAN_POINT ( 'NONE',  ( 2.711717199018286450, 2.143848034498841315, 13.33439168509460337 ) ) ;
#23371=CARTESIAN_POINT ( 'NONE',  ( 35.00000000000000000, -3.287724142101329683, 11.73463472867578972 ) ) ;
#23372=DIRECTION ( 'NONE',  ( -0.000000000000000000, -0.000000000000000000, -1.000000000000000000 ) ) ;
#23373=ORIENTED_EDGE ( 'NONE', *, *, #9452, .F. ) ;
#23374=DIRECTION ( 'NONE',  ( 1.000000000000000000, 0.000000000000000000, 0.000000000000000000 ) ) ;
#23375=DIRECTION ( 'NONE',  ( -1.000000000000000000, 0.000000000000000000, 0.000000000000000000 ) ) ;
#23376=CYLINDRICAL_SURFACE ( 'NONE', #17533, 6.183183579532408380 ) ;
#23377=CYLINDRICAL_SURFACE ( 'NONE', #49999, 12.75000000000000178 ) ;
#23381=ORIENTED_EDGE ( 'NONE', *, *, #9673, .T. ) ;
#23385=CARTESIAN_POINT ( 'NONE',  ( 21.47577844137839520, -11.77878740299461313, -2.329267728435745255 ) ) ;
#23387=FACE_OUTER_BOUND ( 'NONE', #49942, .T. ) ;
#23388=DIRECTION ( 'NONE',  ( 1.000000000000000000, 0.000000000000000000, 0.000000000000000000 ) ) ;
#23391=CARTESIAN_POINT ( 'NONE',  ( -10.87317010465706346, -6.818838523886362246, -11.65834341784620065 ) ) ;
#23392=DIRECTION ( 'NONE',  ( 0.000000000000000000, -0.2006870767258961963, 0.9796553971857727694 ) ) ;
#23394=DIRECTION ( 'NONE',  ( -1.000000000000000000, 0.000000000000000000, 0.000000000000000000 ) ) ;
#23396=ORIENTED_EDGE ( 'NONE', *, *, #21808, .F. ) ;
#23397=CARTESIAN_POINT ( 'NONE',  ( 24.82652845881425208, 8.390869743685042792, -8.578654028722157321 ) ) ;
#23399=CARTESIAN_POINT ( 'NONE',  ( 35.00000000000000000, -8.551552972817137999, -8.052525312709853722 ) ) ;
#23401=DIRECTION ( 'NONE',  ( 0.000000000000000000, 0.01356324068817991828, -0.9999080150203990547 ) ) ;
#23402=DIRECTION ( 'NONE',  ( 0.000000000000000000, -0.9246979985058680906, -0.3807014730195321661 ) ) ;
#23404=EDGE_CURVE ( 'NONE', #22451, #34672, #25585, .T. ) ;
#23409=VERTEX_POINT ( 'NONE', #58067 ) ;
#23410=CARTESIAN_POINT ( 'NONE',  ( -37.00000000000000711, 0.000000000000000000, 0.000000000000000000 ) ) ;
#23412=DIRECTION ( 'NONE',  ( -1.000000000000000000, 0.000000000000000000, -0.000000000000000000 ) ) ;
#23413=EDGE_CURVE ( 'NONE', #33694, #37925, #35638, .T. ) ;
#23414=DIRECTION ( 'NONE',  ( -1.000000000000000000, -0.000000000000000000, -0.000000000000000000 ) ) ;
#23418=CARTESIAN_POINT ( 'NONE',  ( -10.74967964958609201, -6.109637884495152882, 12.04509226909001640 ) ) ;
#23419=EDGE_CURVE ( 'NONE', #60081, #10789, #64273, .T. ) ;
#23424=AXIS2_PLACEMENT_3D ( 'NONE', #62539, #37279, #47599 ) ;
#23428=CIRCLE ( 'NONE', #25560, 5.000000000000000000 ) ;
#23433=VERTEX_POINT ( 'NONE', #64658 ) ;
#23434=CARTESIAN_POINT ( 'NONE',  ( 37.00000000000000711, 11.73463472867580393, 3.287724142101285274 ) ) ;
#23437=ORIENTED_EDGE ( 'NONE', *, *, #44167, .F. ) ;
#23439=EDGE_CURVE ( 'NONE', #55813, #50026, #26071, .T. ) ;
#23440=CIRCLE ( 'NONE', #38340, 12.75000000000000178 ) ;
#23441=AXIS2_PLACEMENT_3D ( 'NONE', #11956, #8289, #18281 ) ;
#23442=VECTOR ( 'NONE', #15574, 1000.000000000000000 ) ;
#23444=EDGE_CURVE ( 'NONE', #8833, #15077, #38837, .T. ) ;
#23445=CARTESIAN_POINT ( 'NONE',  ( 35.00000000000000000, 4.705694406421931860E-17, -3.469127814946512892E-15 ) ) ;
#23446=DIRECTION ( 'NONE',  ( -1.000000000000000000, 0.000000000000000000, -0.000000000000000000 ) ) ;
#23447=DIRECTION ( 'NONE',  ( 0.000000000000000000, 0.3807014730195220631, -0.9246979985058721985 ) ) ;
#23449=CIRCLE ( 'NONE', #98, 12.75000000000000178 ) ;
#23451=CARTESIAN_POINT ( 'NONE',  ( -37.00000000000000711, 0.000000000000000000, 0.000000000000000000 ) ) ;
#23452=ORIENTED_EDGE ( 'NONE', *, *, #17613, .F. ) ;
#23456=EDGE_LOOP ( 'NONE', ( #48338, #38565, #13301, #5166 ) ) ;
#23457=ORIENTED_EDGE ( 'NONE', *, *, #23124, .T. ) ;
#23458=CARTESIAN_POINT ( 'NONE',  ( -25.37500095553464163, 11.65763308310754809, 6.809669256228112033 ) ) ;
#23459=VECTOR ( 'NONE', #17901, 1000.000000000000000 ) ;
#23461=CARTESIAN_POINT ( 'NONE',  ( -26.42332584564274711, 12.40027562897680369, 5.341196054782874292 ) ) ;
#23465=DIRECTION ( 'NONE',  ( 0.000000000000000000, -0.8989688749565110104, -0.4380125133594070519 ) ) ;
#23468=VECTOR ( 'NONE', #22197, 1000.000000000000000 ) ;
#23469=DIRECTION ( 'NONE',  ( 0.000000000000000000, -1.000000000000000000, 0.000000000000000000 ) ) ;
#23470=DIRECTION ( 'NONE',  ( 0.000000000000000000, 0.01356324068817992695, -0.9999080150203990547 ) ) ;
#23472=ORIENTED_EDGE ( 'NONE', *, *, #39535, .F. ) ;
#23473=CIRCLE ( 'NONE', #31946, 12.00000000000000000 ) ;
#23475=VERTEX_POINT ( 'NONE', #4170 ) ;
#23476=CIRCLE ( 'NONE', #28785, 15.00000000000000000 ) ;
#23477=CARTESIAN_POINT ( 'NONE',  ( 35.00000000000000000, -2.216820770815006725, 11.53507381115585417 ) ) ;
#23481=DIRECTION ( 'NONE',  ( -1.000000000000000000, 0.000000000000000000, -0.000000000000000000 ) ) ;
#23482=DIRECTION ( 'NONE',  ( 0.000000000000000000, -0.8009703041134232926, -0.5987040770935588840 ) ) ;
#23483=DIRECTION ( 'NONE',  ( 1.000000000000000000, 0.000000000000000000, 0.000000000000000000 ) ) ;
#23484=CIRCLE ( 'NONE', #60635, 12.74999999999999822 ) ;
#23485=EDGE_CURVE ( 'NONE', #21858, #34626, #60053, .T. ) ;
#23486=VERTEX_POINT ( 'NONE', #3541 ) ;
#23487=DIRECTION ( 'NONE',  ( 0.000000000000000000, 0.9346839223284527653, -0.3554799084909002205 ) ) ;
#23488=ORIENTED_EDGE ( 'NONE', *, *, #8067, .T. ) ;
#23493=AXIS2_PLACEMENT_3D ( 'NONE', #35986, #16043, #1764 ) ;
#23494=DIRECTION ( 'NONE',  ( -1.000000000000000000, 0.000000000000000000, 0.000000000000000000 ) ) ;
#23495=ADVANCED_FACE ( 'NONE', ( #4510 ), #43741, .T. ) ;
#23496=VECTOR ( 'NONE', #27658, 1000.000000000000000 ) ;
#23497=FACE_OUTER_BOUND ( 'NONE', #2355, .T. ) ;
#23500=CARTESIAN_POINT ( 'NONE',  ( 37.00000000000000711, -7.608228585767796481, -10.23119532541070420 ) ) ;
#23504=EDGE_CURVE ( 'NONE', #12570, #37018, #45188, .T. ) ;
#23505=ORIENTED_EDGE ( 'NONE', *, *, #61763, .T. ) ;
#23507=DIRECTION ( 'NONE',  ( -1.000000000000000000, 0.000000000000000000, 0.000000000000000000 ) ) ;
#23508=DIRECTION ( 'NONE',  ( -1.000000000000000000, 0.000000000000000000, 0.000000000000000000 ) ) ;
#23513=AXIS2_PLACEMENT_3D ( 'NONE', #14249, #29530, #4283 ) ;
#23515=CARTESIAN_POINT ( 'NONE',  ( -28.19906601428456838, -11.19867358001292068, -4.323235035335756038 ) ) ;
#23519=CIRCLE ( 'NONE', #19298, 5.000000000000000000 ) ;
#23521=ORIENTED_EDGE ( 'NONE', *, *, #7413, .T. ) ;
#23523=CYLINDRICAL_SURFACE ( 'NONE', #48013, 17.25474371510545879 ) ;
#23524=CARTESIAN_POINT ( 'NONE',  ( -36.00000000000000711, -1.738225594539906771, -12.63095688309031139 ) ) ;
#23527=CARTESIAN_POINT ( 'NONE',  ( 36.00000000000000711, -9.913596905230170009, -8.017674001891752056 ) ) ;
#23529=EDGE_CURVE ( 'NONE', #4710, #31308, #62189, .T. ) ;
#23531=ORIENTED_EDGE ( 'NONE', *, *, #473, .T. ) ;
#23537=DIRECTION ( 'NONE',  ( 0.000000000000000000, -0.9246979985058763063, -0.3807014730195120711 ) ) ;
#23538=FACE_OUTER_BOUND ( 'NONE', #27045, .T. ) ;
#23539=DIRECTION ( 'NONE',  ( -1.000000000000000000, -0.000000000000000000, 0.000000000000000000 ) ) ;
#23540=CARTESIAN_POINT ( 'NONE',  ( 35.00000000000000000, 4.705694406421931860E-17, -3.469127814946512892E-15 ) ) ;
#23541=AXIS2_PLACEMENT_3D ( 'NONE', #30580, #46878, #15617 ) ;
#23542=ORIENTED_EDGE ( 'NONE', *, *, #18776, .F. ) ;
#23545=VERTEX_POINT ( 'NONE', #55024 ) ;
#23546=DIRECTION ( 'NONE',  ( 1.000000000000000000, -0.000000000000000000, 0.000000000000000000 ) ) ;
#23547=EDGE_CURVE ( 'NONE', #58033, #14694, #15423, .T. ) ;
#23549=CARTESIAN_POINT ( 'NONE',  ( 3.459614771489464946, -11.09853614738469396, -7.685863346768205595 ) ) ;
#23550=AXIS2_PLACEMENT_3D ( 'NONE', #17002, #37281, #12014 ) ;
#23553=ORIENTED_EDGE ( 'NONE', *, *, #19244, .T. ) ;
#23554=DIRECTION ( 'NONE',  ( 0.000000000000000000, -0.04924826701373154203, -0.9987865678893285137 ) ) ;
#23557=VERTEX_POINT ( 'NONE', #18508 ) ;
#23559=CARTESIAN_POINT ( 'NONE',  ( -37.00000000000000711, 0.000000000000000000, 0.000000000000000000 ) ) ;
#23560=LINE ( 'NONE', #23225, #19556 ) ;
#23565=CARTESIAN_POINT ( 'NONE',  ( -35.00000000000000000, 10.59380114696480391, -7.094637218249239652 ) ) ;
#23568=CARTESIAN_POINT ( 'NONE',  ( 35.00000000000000000, 10.28547182238015978, 5.672855678558568648 ) ) ;
#23571=EDGE_CURVE ( 'NONE', #4661, #14900, #9456, .T. ) ;
#23572=VERTEX_POINT ( 'NONE', #19797 ) ;
#23573=LINE ( 'NONE', #8589, #50726 ) ;
#23574=DIRECTION ( 'NONE',  ( 0.000000000000000000, 0.8515178078024886466, -0.5243256840888532722 ) ) ;
#23575=AXIS2_PLACEMENT_3D ( 'NONE', #59872, #60179, #25588 ) ;
#23576=EDGE_CURVE ( 'NONE', #2181, #58998, #13344, .T. ) ;
#23578=CARTESIAN_POINT ( 'NONE',  ( 35.00000000000000000, -11.74614673114903596, -0.01609748574441245694 ) ) ;
#23579=CIRCLE ( 'NONE', #57347, 12.75000000000000178 ) ;
#23580=CARTESIAN_POINT ( 'NONE',  ( 28.16476997869163412, 10.96217668651337007, 4.899552670153406453 ) ) ;
#23581=CARTESIAN_POINT ( 'NONE',  ( -35.00000000000000000, 11.60979404548639948, -3.704519465651187282 ) ) ;
#23582=AXIS2_PLACEMENT_3D ( 'NONE', #53348, #17101, #7121 ) ;
#23583=DIRECTION ( 'NONE',  ( 0.000000000000000000, 0.9651210252299785575, 0.2618041379715665973 ) ) ;
#23584=CARTESIAN_POINT ( 'NONE',  ( 35.00000000000000000, 4.732539170486261604, -11.23004253107766282 ) ) ;
#23585=CYLINDRICAL_SURFACE ( 'NONE', #28908, 4.999999999999999112 ) ;
#23587=EDGE_CURVE ( 'NONE', #10033, #35942, #39612, .T. ) ;
#23590=ORIENTED_EDGE ( 'NONE', *, *, #37390, .T. ) ;
#23591=DIRECTION ( 'NONE',  ( 0.000000000000000000, -0.9467777615094604693, -0.3218879778915875178 ) ) ;
#23593=DIRECTION ( 'NONE',  ( 0.000000000000000000, 0.9246979985058709772, 0.3807014730195252827 ) ) ;
#23594=CARTESIAN_POINT ( 'NONE',  ( -10.61476244842199002, -9.390648123693877025, 9.710410838802262745 ) ) ;
#23595=CARTESIAN_POINT ( 'NONE',  ( -35.00000000000000000, 11.66664283989679696, 5.143145423404321903 ) ) ;
#23596=EDGE_CURVE ( 'NONE', #10568, #12727, #57936, .T. ) ;
#23597=EDGE_LOOP ( 'NONE', ( #21218, #47341, #41597, #36958 ) ) ;
#23598=CARTESIAN_POINT ( 'NONE',  ( -27.45775109278351067, 8.499184579339635448, -8.471355351200609007 ) ) ;
#23601=CARTESIAN_POINT ( 'NONE',  ( -35.00000000000000000, 0.000000000000000000, 0.000000000000000000 ) ) ;
#23602=DIRECTION ( 'NONE',  ( -1.000000000000000000, 0.000000000000000000, 0.000000000000000000 ) ) ;
#23603=AXIS2_PLACEMENT_3D ( 'NONE', #1546, #22799, #21821 ) ;
#23604=VECTOR ( 'NONE', #53845, 1000.000000000000000 ) ;
#23605=ADVANCED_FACE ( 'NONE', ( #54397 ), #813, .F. ) ;
#23606=DIRECTION ( 'NONE',  ( 0.000000000000000000, 0.04924826701374583615, 0.9987865678893277366 ) ) ;
#23607=EDGE_LOOP ( 'NONE', ( #17435, #24856, #38991, #15564 ) ) ;
#23608=DIRECTION ( 'NONE',  ( -1.000000000000000000, 0.000000000000000000, 0.000000000000000000 ) ) ;
#23610=CARTESIAN_POINT ( 'NONE',  ( 47.00000000000000711, 4.705694406421931860E-17, -3.469127814946512892E-15 ) ) ;
#23611=CIRCLE ( 'NONE', #32073, 12.74999999999999822 ) ;
#23613=VERTEX_POINT ( 'NONE', #56010 ) ;
#23614=CARTESIAN_POINT ( 'NONE',  ( -9.765880726038068005, 12.49572852913685139, -5.113274341876826057 ) ) ;
#23618=DIRECTION ( 'NONE',  ( 1.000000000000000000, 0.000000000000000000, 0.000000000000000000 ) ) ;
#23624=ORIENTED_EDGE ( 'NONE', *, *, #38187, .T. ) ;
#23625=CARTESIAN_POINT ( 'NONE',  ( -35.00000000000000000, -6.415447294506628317, -11.01837265713079894 ) ) ;
#23626=ADVANCED_FACE ( 'NONE', ( #60677 ), #51704, .T. ) ;
#23627=CARTESIAN_POINT ( 'NONE',  ( -35.00000000000000000, -12.16893194857547478, -3.805206332242601963 ) ) ;
#23628=ORIENTED_EDGE ( 'NONE', *, *, #65601, .F. ) ;
#23629=CARTESIAN_POINT ( 'NONE',  ( 35.00000000000000000, -0.8294751490778421443, 12.15823808070322976 ) ) ;
#23630=CIRCLE ( 'NONE', #12986, 12.18649999999999878 ) ;
#23633=CARTESIAN_POINT ( 'NONE',  ( 35.00000000000000000, 4.705694406421931860E-17, -3.469127814946512892E-15 ) ) ;
#23635=CARTESIAN_POINT ( 'NONE',  ( -35.00000000000000000, 12.54989509947650994, 2.250029553613800637 ) ) ;
#23636=ORIENTED_EDGE ( 'NONE', *, *, #379, .F. ) ;
#23638=CARTESIAN_POINT ( 'NONE',  ( -17.96927786591848886, -9.630624776632364714, 7.160636282608096259 ) ) ;
#23640=ORIENTED_EDGE ( 'NONE', *, *, #8257, .F. ) ;
#23641=DIRECTION ( 'NONE',  ( 1.000000000000000000, 0.000000000000000000, -0.000000000000000000 ) ) ;
#23642=ORIENTED_EDGE ( 'NONE', *, *, #43914, .F. ) ;
#23643=CIRCLE ( 'NONE', #22600, 5.000000000000001776 ) ;
#23644=VERTEX_POINT ( 'NONE', #163 ) ;
#23647=LINE ( 'NONE', #49579, #35790 ) ;
#23653=CARTESIAN_POINT ( 'NONE',  ( 37.00000000000000711, 5.015831474386306610, -10.62137734850269943 ) ) ;
#23654=ORIENTED_EDGE ( 'NONE', *, *, #21555, .T. ) ;
#23655=DIRECTION ( 'NONE',  ( 1.000000000000000000, 0.000000000000000000, 0.000000000000000000 ) ) ;
#23656=ORIENTED_EDGE ( 'NONE', *, *, #36566, .T. ) ;
#23660=EDGE_CURVE ( 'NONE', #3297, #21470, #13380, .T. ) ;
#23666=ORIENTED_EDGE ( 'NONE', *, *, #9633, .T. ) ;
#23669=ADVANCED_FACE ( 'NONE', ( #41701 ), #505, .T. ) ;
#23671=CIRCLE ( 'NONE', #50200, 12.74999999999999822 ) ;
#23675=CARTESIAN_POINT ( 'NONE',  ( -28.71060117729524919, 3.670315194194619490, 12.99175741217617563 ) ) ;
#23676=CARTESIAN_POINT ( 'NONE',  ( 35.00000000000000000, -4.946702696913249042, -11.13736569743272753 ) ) ;
#23678=CARTESIAN_POINT ( 'NONE',  ( 35.00000000000000000, 4.705694406421931860E-17, -3.469127814946512892E-15 ) ) ;
#23679=CARTESIAN_POINT ( 'NONE',  ( 12.52750123246316072, 0.4973700281276248192, 25.00000000000000000 ) ) ;
#23680=CARTESIAN_POINT ( 'NONE',  ( -19.47984447937493613, -3.750539801530005768, -12.96855624952674724 ) ) ;
#23682=CARTESIAN_POINT ( 'NONE',  ( -30.18541646480305829, -1.811670027856088439, 13.38380110246788490 ) ) ;
#23683=EDGE_CURVE ( 'NONE', #14200, #2755, #3756, .T. ) ;
#23684=EDGE_CURVE ( 'NONE', #40131, #52526, #21775, .T. ) ;
#23685=EDGE_CURVE ( 'NONE', #22527, #45722, #15446, .T. ) ;
#23687=DIRECTION ( 'NONE',  ( 0.000000000000000000, -0.1118654143051685257, -0.9937233664769752339 ) ) ;
#23691=AXIS2_PLACEMENT_3D ( 'NONE', #31532, #56840, #31220 ) ;
#23692=CIRCLE ( 'NONE', #15164, 4.999999999999999112 ) ;
#23694=CIRCLE ( 'NONE', #23751, 15.00000000000000000 ) ;
#23695=ORIENTED_EDGE ( 'NONE', *, *, #34452, .T. ) ;
#23696=LINE ( 'NONE', #2433, #44788 ) ;
#23698=EDGE_LOOP ( 'NONE', ( #19118, #42731, #42184, #34642 ) ) ;
#23702=CARTESIAN_POINT ( 'NONE',  ( -27.45775109278351067, 11.83395752356219077, -1.989333891161980894 ) ) ;
#23704=AXIS2_PLACEMENT_3D ( 'NONE', #46563, #16959, #45919 ) ;
#23705=ORIENTED_EDGE ( 'NONE', *, *, #2124, .T. ) ;
#23706=ORIENTED_EDGE ( 'NONE', *, *, #40490, .T. ) ;
#23707=CARTESIAN_POINT ( 'NONE',  ( 29.34908395106651469, -11.50269583891679659, 7.070024793111046257 ) ) ;
#23709=DIRECTION ( 'NONE',  ( -1.000000000000000000, 0.000000000000000000, -0.000000000000000000 ) ) ;
#23711=EDGE_CURVE ( 'NONE', #52094, #44262, #44147, .T. ) ;
#23712=ORIENTED_EDGE ( 'NONE', *, *, #45998, .T. ) ;
#23714=B_SPLINE_CURVE_WITH_KNOTS ( 'NONE', 3,
 ( #37532, #16923, #26566, #52188, #52829, #32202, #36203, #51855, #52525, #46857, #1651, #26250, #10955, #1322, #46220, #62150, #57173, #661 ),
 .UNSPECIFIED., .F., .F.,
 ( 4, 2, 2, 2, 2, 2, 2, 2, 4 ),
 ( 7.770031522344853663E-18, 0.002493514729510051386, 0.003116893411887563473, 0.003740272094265075127, 0.004987029459020096700, 0.006233786823775119140, 0.007480544188530139846, 0.008727301553285160551, 0.009974058918040182992 ),
 .UNSPECIFIED. ) ;
#23717=CARTESIAN_POINT ( 'NONE',  ( 17.54591139300511671, 9.528221380451970646, 7.352565480027280387 ) ) ;
#23718=ORIENTED_EDGE ( 'NONE', *, *, #27254, .F. ) ;
#23719=DIRECTION ( 'NONE',  ( 1.000000000000000000, 0.000000000000000000, -0.000000000000000000 ) ) ;
#23721=CIRCLE ( 'NONE', #56615, 5.000000000000000000 ) ;
#23723=CARTESIAN_POINT ( 'NONE',  ( -29.43980975494970309, -3.641506875706030488, -11.43413432115371364 ) ) ;
#23724=FACE_OUTER_BOUND ( 'NONE', #17199, .T. ) ;
#23725=ORIENTED_EDGE ( 'NONE', *, *, #30086, .T. ) ;
#23727=ORIENTED_EDGE ( 'NONE', *, *, #41903, .T. ) ;
#23728=DIRECTION ( 'NONE',  ( -1.000000000000000000, 0.000000000000000000, 0.000000000000000000 ) ) ;
#23730=ORIENTED_EDGE ( 'NONE', *, *, #37449, .T. ) ;
#23731=CARTESIAN_POINT ( 'NONE',  ( 21.74356534222384596, -11.95363809093303686, -1.123395297719272712 ) ) ;
#23733=DIRECTION ( 'NONE',  ( 0.000000000000000000, 0.3554799084908970563, 0.9346839223284539866 ) ) ;
#23734=AXIS2_PLACEMENT_3D ( 'NONE', #10062, #5389, #30631 ) ;
#23735=DIRECTION ( 'NONE',  ( 1.000000000000000000, 0.000000000000000000, 0.000000000000000000 ) ) ;
#23737=DIRECTION ( 'NONE',  ( -1.000000000000000000, 0.000000000000000000, 0.000000000000000000 ) ) ;
#23739=EDGE_LOOP ( 'NONE', ( #56201, #53289, #41511, #59052 ) ) ;
#23741=ORIENTED_EDGE ( 'NONE', *, *, #19527, .T. ) ;
#23742=EDGE_CURVE ( 'NONE', #30009, #50989, #50578, .T. ) ;
#23743=CIRCLE ( 'NONE', #51373, 4.999999999999999112 ) ;
#23749=CARTESIAN_POINT ( 'NONE',  ( -35.00000000000000000, -12.74921544981111055, 0.1414404973751688388 ) ) ;
#23750=CARTESIAN_POINT ( 'NONE',  ( -7.181456785175555524, -8.540743096806455270, -10.45493698471458188 ) ) ;
#23751=AXIS2_PLACEMENT_3D ( 'NONE', #2015, #17315, #57560 ) ;
#23752=LINE ( 'NONE', #27728, #35498 ) ;
#23753=ORIENTED_EDGE ( 'NONE', *, *, #25978, .F. ) ;
#23755=CARTESIAN_POINT ( 'NONE',  ( 22.57855258442565116, 3.026812727784649493, 25.00000000000000000 ) ) ;
#23756=CIRCLE ( 'NONE', #60902, 12.18650000000000055 ) ;
#23758=DIRECTION ( 'NONE',  ( -1.000000000000000000, 0.000000000000000000, 0.000000000000000000 ) ) ;
#23759=EDGE_CURVE ( 'NONE', #16732, #27686, #632, .T. ) ;
#23760=AXIS2_PLACEMENT_3D ( 'NONE', #54834, #30210, #54517 ) ;
#23762=AXIS2_PLACEMENT_3D ( 'NONE', #21407, #25405, #25743 ) ;
#23765=CARTESIAN_POINT ( 'NONE',  ( -10.33756816907811782, -3.910582247997075989, 12.92259563996709026 ) ) ;
#23766=AXIS2_PLACEMENT_3D ( 'NONE', #50883, #51227, #35882 ) ;
#23767=EDGE_CURVE ( 'NONE', #62086, #48650, #33574, .T. ) ;
#23768=CARTESIAN_POINT ( 'NONE',  ( -9.037010005417281278, -3.102636015309993223, 13.14221497168421848 ) ) ;
#23769=ORIENTED_EDGE ( 'NONE', *, *, #13216, .F. ) ;
#23772=DIRECTION ( 'NONE',  ( 0.000000000000000000, 0.01356324068817998940, -0.9999080150203990547 ) ) ;
#23773=AXIS2_PLACEMENT_3D ( 'NONE', #61809, #37183, #11918 ) ;
#23774=CARTESIAN_POINT ( 'NONE',  ( -24.97643703457612929, 7.232049057323012065, 9.582644723418388466 ) ) ;
#23778=DIRECTION ( 'NONE',  ( 0.000000000000000000, 0.01356324068817991481, -0.9999080150203990547 ) ) ;
#23780=VERTEX_POINT ( 'NONE', #47035 ) ;
#23781=CARTESIAN_POINT ( 'NONE',  ( 145.1370849898475797, 3.309064568108273190E-14, 0.000000000000000000 ) ) ;
#23783=ORIENTED_EDGE ( 'NONE', *, *, #62463, .F. ) ;
#23784=VECTOR ( 'NONE', #7158, 1000.000000000000000 ) ;
#23785=AXIS2_PLACEMENT_3D ( 'NONE', #4960, #4644, #9260 ) ;
#23786=ORIENTED_EDGE ( 'NONE', *, *, #20024, .F. ) ;
#23787=DIRECTION ( 'NONE',  ( 0.000000000000000000, -0.01356324068818000328, 0.9999080150203990547 ) ) ;
#23788=ADVANCED_FACE ( 'NONE', ( #21771 ), #7777, .T. ) ;
#23789=ORIENTED_EDGE ( 'NONE', *, *, #31498, .T. ) ;
#23791=EDGE_CURVE ( 'NONE', #14430, #42534, #30377, .T. ) ;
#23792=CARTESIAN_POINT ( 'NONE',  ( -35.00000000000000000, 12.31350058095527977, -3.307597835713114609 ) ) ;
#23794=LINE ( 'NONE', #44364, #59512 ) ;
#23795=CIRCLE ( 'NONE', #19512, 5.000000000000000888 ) ;
#23797=AXIS2_PLACEMENT_3D ( 'NONE', #28469, #48776, #59727 ) ;
#23798=DIRECTION ( 'NONE',  ( -1.000000000000000000, 0.000000000000000000, 0.000000000000000000 ) ) ;
#23800=VERTEX_POINT ( 'NONE', #28063 ) ;
#23802=CARTESIAN_POINT ( 'NONE',  ( 35.00000000000000000, 4.705694406421931860E-17, -3.469127814946512892E-15 ) ) ;
#23805=CIRCLE ( 'NONE', #29111, 5.000000000000000000 ) ;
#23808=ORIENTED_EDGE ( 'NONE', *, *, #12796, .F. ) ;
#23809=CARTESIAN_POINT ( 'NONE',  ( -17.98414573016741613, 7.072294406407991119, 11.50157350705893755 ) ) ;
#23814=CARTESIAN_POINT ( 'NONE',  ( 35.00000000000000000, 4.705694406421931860E-17, -3.469127814946512892E-15 ) ) ;
#23815=CARTESIAN_POINT ( 'NONE',  ( -35.00000000000000000, 11.66953048682404415, -3.511814412391998541 ) ) ;
#23816=VERTEX_POINT ( 'NONE', #62617 ) ;
#23817=DIRECTION ( 'NONE',  ( 1.000000000000000000, 0.000000000000000000, 0.000000000000000000 ) ) ;
#23819=DIRECTION ( 'NONE',  ( 1.000000000000000000, 0.000000000000000000, 0.000000000000000000 ) ) ;
#23825=CARTESIAN_POINT ( 'NONE',  ( 35.00000000000000000, 8.146229107149526527, 9.063649021438864750 ) ) ;
#23826=EDGE_CURVE ( 'NONE', #4279, #33015, #18747, .T. ) ;
#23828=DIRECTION ( 'NONE',  ( 0.000000000000000000, -0.01356324068817991828, 0.9999080150203990547 ) ) ;
#23830=CARTESIAN_POINT ( 'NONE',  ( -37.00000000000000711, 0.000000000000000000, 0.000000000000000000 ) ) ;
#23831=VERTEX_POINT ( 'NONE', #48673 ) ;
#23833=CARTESIAN_POINT ( 'NONE',  ( -37.00000000000000711, 10.43555801961483098, -5.391785509270847321 ) ) ;
#23834=AXIS2_PLACEMENT_3D ( 'NONE', #38742, #18794, #14431 ) ;
#23837=DIRECTION ( 'NONE',  ( 0.000000000000000000, -0.01356324068817991828, 0.9999080150203990547 ) ) ;
#23839=DIRECTION ( 'NONE',  ( -0.000000000000000000, -0.000000000000000000, -1.000000000000000000 ) ) ;
#23842=VECTOR ( 'NONE', #64681, 1000.000000000000000 ) ;
#23843=CARTESIAN_POINT ( 'NONE',  ( -9.860341104261298284, -4.079292048029911300, -11.29117792640004936 ) ) ;
#23845=EDGE_CURVE ( 'NONE', #38680, #25311, #29126, .T. ) ;
#23846=DIRECTION ( 'NONE',  ( -1.000000000000000000, -0.000000000000000000, 0.000000000000000000 ) ) ;
#23847=DIRECTION ( 'NONE',  ( -1.000000000000000000, 0.000000000000000000, 0.000000000000000000 ) ) ;
#23848=ORIENTED_EDGE ( 'NONE', *, *, #33750, .T. ) ;
#23849=VECTOR ( 'NONE', #40659, 1000.000000000000000 ) ;
#23850=CARTESIAN_POINT ( 'NONE',  ( 3.459614771489464946, -11.09853614738469396, 25.00000000000000000 ) ) ;
#23851=DIRECTION ( 'NONE',  ( -1.000000000000000000, 0.000000000000000000, 0.000000000000000000 ) ) ;
#23853=AXIS2_PLACEMENT_3D ( 'NONE', #54785, #64095, #9202 ) ;
#23856=ORIENTED_EDGE ( 'NONE', *, *, #56796, .T. ) ;
#23858=CARTESIAN_POINT ( 'NONE',  ( 29.60251855095053486, 10.89349753539994836, 7.986429861213258263 ) ) ;
#23863=DIRECTION ( 'NONE',  ( 0.000000000000000000, 0.01356324068817998940, -0.9999080150203990547 ) ) ;
#23864=CARTESIAN_POINT ( 'NONE',  ( 18.84867683979356201, -5.944105725974474730, 12.12095735156416509 ) ) ;
#23868=VECTOR ( 'NONE', #63787, 1000.000000000000000 ) ;
#23869=DIRECTION ( 'NONE',  ( 0.000000000000000000, -0.9796553971857722143, -0.2006870767258996102 ) ) ;
#23870=EDGE_LOOP ( 'NONE', ( #12111, #30742, #14681, #59341 ) ) ;
#23872=EDGE_CURVE ( 'NONE', #60517, #56420, #51620, .T. ) ;
#23873=CARTESIAN_POINT ( 'NONE',  ( 17.27839441901508621, -10.52068335315807524, 5.771933972472480967 ) ) ;
#23876=CARTESIAN_POINT ( 'NONE',  ( 37.00000000000000711, -8.573591947375261313, 8.029056188533775895 ) ) ;
#23877=DIRECTION ( 'NONE',  ( 1.000000000000000000, -0.000000000000000000, 0.000000000000000000 ) ) ;
#23878=CARTESIAN_POINT ( 'NONE',  ( -29.95631573795198577, 0.8334892910201414651, -11.97922705870643334 ) ) ;
#23879=CARTESIAN_POINT ( 'NONE',  ( 9.575800908719084958, 13.45729701195361372, -1.072919909436246266 ) ) ;
#23881=VECTOR ( 'NONE', #16593, 1000.000000000000000 ) ;
#23882=ORIENTED_EDGE ( 'NONE', *, *, #30315, .T. ) ;
#23883=ORIENTED_EDGE ( 'NONE', *, *, #2071, .T. ) ;
#23885=CARTESIAN_POINT ( 'NONE',  ( -36.00000000000000711, -12.66641127287624968, -1.457575200925676828 ) ) ;
#23887=VERTEX_POINT ( 'NONE', #64277 ) ;
#23889=VECTOR ( 'NONE', #527, 1000.000000000000000 ) ;
#23891=CARTESIAN_POINT ( 'NONE',  ( -35.00000000000000000, 0.000000000000000000, 0.000000000000000000 ) ) ;
#23892=VERTEX_POINT ( 'NONE', #34343 ) ;
#23895=EDGE_CURVE ( 'NONE', #11924, #20989, #25070, .T. ) ;
#23896=AXIS2_PLACEMENT_3D ( 'NONE', #28302, #63859, #53907 ) ;
#23897=DIRECTION ( 'NONE',  ( 1.000000000000000000, 0.000000000000000000, 0.000000000000000000 ) ) ;
#23898=EDGE_LOOP ( 'NONE', ( #8005, #47522, #51701, #47340 ) ) ;
#23899=VERTEX_POINT ( 'NONE', #13722 ) ;
#23901=CARTESIAN_POINT ( 'NONE',  ( 12.47628546223243617, 0.000000000000000000, 13.50000000000000178 ) ) ;
#23902=ADVANCED_FACE ( 'NONE', ( #34007 ), #44312, .T. ) ;
#23903=AXIS2_PLACEMENT_3D ( 'NONE', #27696, #6131, #26392 ) ;
#23904=DIRECTION ( 'NONE',  ( 0.000000000000000000, -0.2355298848897378339, -0.9718671068226493182 ) ) ;
#23907=CARTESIAN_POINT ( 'NONE',  ( -37.00000000000000711, 0.000000000000000000, 0.000000000000000000 ) ) ;
#23908=CARTESIAN_POINT ( 'NONE',  ( -35.00000000000000000, 11.50504120060943158, 4.018060380616439886 ) ) ;
#23911=LINE ( 'NONE', #53173, #41153 ) ;
#23912=CARTESIAN_POINT ( 'NONE',  ( -14.51274404441612376, 7.865079314623513618, 9.063796499285235342 ) ) ;
#23914=DIRECTION ( 'NONE',  ( 1.000000000000000000, 0.000000000000000000, 0.000000000000000000 ) ) ;
#23918=CARTESIAN_POINT ( 'NONE',  ( -29.43980975494970309, -3.641506875706030488, 25.00000000000000000 ) ) ;
#23922=CARTESIAN_POINT ( 'NONE',  ( -17.67947061630126271, 7.441336280027901040, -9.417258690134145738 ) ) ;
#23923=ORIENTED_EDGE ( 'NONE', *, *, #42113, .F. ) ;
#23924=DIRECTION ( 'NONE',  ( 0.000000000000000000, 0.4380125133593912312, -0.8989688749565187820 ) ) ;
#23927=CARTESIAN_POINT ( 'NONE',  ( -35.00000000000000000, -11.81949347079749124, 2.968224442958359965 ) ) ;
#23930=CARTESIAN_POINT ( 'NONE',  ( 35.00000000000000000, -1.262958560998847624, -12.12087942037209665 ) ) ;
#23934=EDGE_CURVE ( 'NONE', #36243, #23284, #26115, .T. ) ;
#23936=AXIS2_PLACEMENT_3D ( 'NONE', #15954, #51248, #46561 ) ;
#23937=ORIENTED_EDGE ( 'NONE', *, *, #29146, .F. ) ;
#23938=CARTESIAN_POINT ( 'NONE',  ( -19.02967556479663713, 11.99999999999999645, 1.585036030062028271E-15 ) ) ;
#23941=DIRECTION ( 'NONE',  ( 0.000000000000000000, -0.5767582926625031137, -0.8169148498130233138 ) ) ;
#23942=CYLINDRICAL_SURFACE ( 'NONE', #37355, 12.74999999999999822 ) ;
#23944=VECTOR ( 'NONE', #2722, 1000.000000000000000 ) ;
#23945=EDGE_LOOP ( 'NONE', ( #60937, #63206, #62749, #57928 ) ) ;
#23946=ORIENTED_EDGE ( 'NONE', *, *, #43009, .F. ) ;
#23949=CARTESIAN_POINT ( 'NONE',  ( -37.00000000000000711, 0.000000000000000000, 0.000000000000000000 ) ) ;
#23950=LINE ( 'NONE', #3687, #13021 ) ;
#23951=FACE_OUTER_BOUND ( 'NONE', #65387, .T. ) ;
#23953=CARTESIAN_POINT ( 'NONE',  ( -35.00000000000000000, -6.564808257521844048, 10.93004082984016279 ) ) ;
#23954=EDGE_CURVE ( 'NONE', #19473, #19363, #63260, .T. ) ;
#23955=ORIENTED_EDGE ( 'NONE', *, *, #24021, .T. ) ;
#23957=ORIENTED_EDGE ( 'NONE', *, *, #53041, .F. ) ;
#23959=CARTESIAN_POINT ( 'NONE',  ( -35.00000000000000000, 0.000000000000000000, 0.000000000000000000 ) ) ;
#23960=EDGE_CURVE ( 'NONE', #44463, #52168, #60095, .T. ) ;
#23962=FACE_OUTER_BOUND ( 'NONE', #13903, .T. ) ;
#23963=DIRECTION ( 'NONE',  ( 1.000000000000000000, -0.000000000000000000, 0.000000000000000000 ) ) ;
#23964=VERTEX_POINT ( 'NONE', #34972 ) ;
#23966=CARTESIAN_POINT ( 'NONE',  ( 37.00000000000000711, -12.73293890771483561, -0.6593684648220077271 ) ) ;
#23967=DIRECTION ( 'NONE',  ( 1.000000000000000000, 0.000000000000000000, 0.000000000000000000 ) ) ;
#23968=ORIENTED_EDGE ( 'NONE', *, *, #1859, .T. ) ;
#23971=EDGE_LOOP ( 'NONE', ( #13566, #48740, #16926, #35295 ) ) ;
#23972=EDGE_CURVE ( 'NONE', #15089, #61328, #6072, .T. ) ;
#23974=SURFACE_SIDE_STYLE ('',( #28948 ) ) ;
#23975=VERTEX_POINT ( 'NONE', #30006 ) ;
#23980=CARTESIAN_POINT ( 'NONE',  ( -21.17861794710831091, 13.00977982294135593, -3.604945070120774808 ) ) ;
#23983=VERTEX_POINT ( 'NONE', #56605 ) ;
#23986=DIRECTION ( 'NONE',  ( 0.9261641133930337277, 0.000000000000000000, -0.3771207168306929813 ) ) ;
#23987=CARTESIAN_POINT ( 'NONE',  ( -18.74580655112670868, -4.843304743421753322, -12.60275085743400680 ) ) ;
#23988=ORIENTED_EDGE ( 'NONE', *, *, #47884, .T. ) ;
#23989=DIRECTION ( 'NONE',  ( 1.000000000000000000, 0.000000000000000000, -0.000000000000000000 ) ) ;
#23990=CARTESIAN_POINT ( 'NONE',  ( 28.25627792643572889, 10.45952599874087063, 5.894934686502148580 ) ) ;
#23992=VECTOR ( 'NONE', #55939, 1000.000000000000000 ) ;
#23996=ORIENTED_EDGE ( 'NONE', *, *, #51164, .F. ) ;
#23997=CARTESIAN_POINT ( 'NONE',  ( 35.00000000000000000, -8.496612874013090178, 9.506317355798454827 ) ) ;
#23998=CARTESIAN_POINT ( 'NONE',  ( 37.00000000000000711, 4.705694406421931860E-17, -3.469127814946512892E-15 ) ) ;
#23999=CARTESIAN_POINT ( 'NONE',  ( -30.03609618253042868, 0.3802027729374650722, 13.49649232113790909 ) ) ;
#24001=CARTESIAN_POINT ( 'NONE',  ( 13.19552928342135090, 11.39730694699084523, -3.781285820845986301 ) ) ;
#24007=DIRECTION ( 'NONE',  ( 1.000000000000000000, 0.000000000000000000, 0.000000000000000000 ) ) ;
#24009=CARTESIAN_POINT ( 'NONE',  ( -35.00000000000000000, -5.921969905510425569, 10.14408668126211488 ) ) ;
#24011=CARTESIAN_POINT ( 'NONE',  ( 7.195572628608377208, -7.349260008028998037, -9.497068771844457302 ) ) ;
#24013=EDGE_CURVE ( 'NONE', #23085, #3506, #27198, .T. ) ;
#24014=AXIS2_PLACEMENT_3D ( 'NONE', #12011, #21335, #62879 ) ;
#24015=EDGE_LOOP ( 'NONE', ( #65092, #29023, #49642, #11256 ) ) ;
#24021=EDGE_CURVE ( 'NONE', #20717, #17286, #36301, .T. ) ;
#24022=LINE ( 'NONE', #19026, #14079 ) ;
#24025=EDGE_CURVE ( 'NONE', #65378, #64221, #61140, .T. ) ;
#24028=ORIENTED_EDGE ( 'NONE', *, *, #63637, .T. ) ;
#24030=EDGE_CURVE ( 'NONE', #41230, #17964, #31325, .T. ) ;
#24033=CARTESIAN_POINT ( 'NONE',  ( -35.00000000000000000, -7.251710744571512102, -9.240395740215712195 ) ) ;
#24035=DIRECTION ( 'NONE',  ( 1.000000000000000000, -0.000000000000000000, 0.000000000000000000 ) ) ;
#24036=ORIENTED_EDGE ( 'NONE', *, *, #9649, .T. ) ;
#24037=CARTESIAN_POINT ( 'NONE',  ( 35.00000000000000000, 4.705694406421931860E-17, -3.469127814946512892E-15 ) ) ;
#24041=DIRECTION ( 'NONE',  ( 0.000000000000000000, -0.01356324068817998940, 0.9999080150203990547 ) ) ;
#24042=ORIENTED_EDGE ( 'NONE', *, *, #27432, .T. ) ;
#24043=DIRECTION ( 'NONE',  ( -1.000000000000000000, 0.000000000000000000, 0.000000000000000000 ) ) ;
#24044=ORIENTED_EDGE ( 'NONE', *, *, #21332, .F. ) ;
#24045=CARTESIAN_POINT ( 'NONE',  ( -37.00000000000000711, -10.49591321039677005, -5.273331777780449592 ) ) ;
#24046=ORIENTED_EDGE ( 'NONE', *, *, #27243, .T. ) ;
#24048=CARTESIAN_POINT ( 'NONE',  ( -35.00000000000000000, 0.000000000000000000, 0.000000000000000000 ) ) ;
#24051=CARTESIAN_POINT ( 'NONE',  ( 37.00000000000000711, 4.705694406421931860E-17, -3.469127814946512892E-15 ) ) ;
#24053=DIRECTION ( 'NONE',  ( 1.000000000000000000, -0.000000000000000000, 0.000000000000000000 ) ) ;
#24055=VERTEX_POINT ( 'NONE', #61249 ) ;
#24056=EDGE_CURVE ( 'NONE', #28113, #5802, #35954, .T. ) ;
#24058=CARTESIAN_POINT ( 'NONE',  ( 35.00000000000000000, 4.705694406421931860E-17, -3.469127814946512892E-15 ) ) ;
#24062=CARTESIAN_POINT ( 'NONE',  ( -37.00000000000000711, 0.000000000000000000, 0.000000000000000000 ) ) ;
#24063=DIRECTION ( 'NONE',  ( 0.000000000000000000, 0.01356324068817992175, -0.9999080150203990547 ) ) ;
#24064=CARTESIAN_POINT ( 'NONE',  ( 47.00000000000000711, 4.705694406421931860E-17, -3.469127814946512892E-15 ) ) ;
#24066=CIRCLE ( 'NONE', #47420, 4.999999999999999112 ) ;
#24067=CARTESIAN_POINT ( 'NONE',  ( 25.05309951391468459, 25.00000000000000000, -8.132934882857099979 ) ) ;
#24068=CIRCLE ( 'NONE', #4940, 4.999999999999999112 ) ;
#24069=ORIENTED_EDGE ( 'NONE', *, *, #39904, .T. ) ;
#24070=DIRECTION ( 'NONE',  ( 0.000000000000000000, -0.01356324068818000848, 0.9999080150203990547 ) ) ;
#24072=DIRECTION ( 'NONE',  ( -0.000000000000000000, -1.000000000000000000, -0.000000000000000000 ) ) ;
#24075=( BOUNDED_CURVE ( )  B_SPLINE_CURVE ( 3, ( #19883, #61746, #51484, #40142 ),
 .UNSPECIFIED., .F., .F. ) 
 B_SPLINE_CURVE_WITH_KNOTS ( ( 4, 4 ),
 ( 5.102875344919000966, 5.142681165258892406 ),
 .UNSPECIFIED. ) 
 CURVE ( )  GEOMETRIC_REPRESENTATION_ITEM ( )  RATIONAL_B_SPLINE_CURVE ( ( 1.000000000000000000, 0.9998679624143003153, 0.9998679624143003153, 1.000000000000000000 ) ) 
 REPRESENTATION_ITEM ( '' )  );
#24076=CARTESIAN_POINT ( 'NONE',  ( -6.736209972540539326, -1.198479029871813095, 13.44688918519066334 ) ) ;
#24077=CARTESIAN_POINT ( 'NONE',  ( -35.00000000000000000, 11.70009620280411688, 1.039216533672945753 ) ) ;
#24078=ORIENTED_EDGE ( 'NONE', *, *, #15747, .T. ) ;
#24080=CARTESIAN_POINT ( 'NONE',  ( -35.00000000000000000, 11.30684963584389280, 4.545979934229452901 ) ) ;
#24081=CARTESIAN_POINT ( 'NONE',  ( 3.624631522511398529, 4.203481679627634193, 11.24801011402735362 ) ) ;
#24083=EDGE_CURVE ( 'NONE', #61832, #39576, #42043, .T. ) ;
#24084=CARTESIAN_POINT ( 'NONE',  ( -35.00000000000000000, -4.018060380616481631, 11.50504120060941915 ) ) ;
#24085=DIRECTION ( 'NONE',  ( 1.000000000000000000, 0.000000000000000000, 0.000000000000000000 ) ) ;
#24089=CARTESIAN_POINT ( 'NONE',  ( -37.00000000000000711, -10.63508530065525370, 4.986700593229667078 ) ) ;
#24092=DIRECTION ( 'NONE',  ( 1.000000000000000000, 0.000000000000000000, 0.000000000000000000 ) ) ;
#24094=EDGE_CURVE ( 'NONE', #59597, #60093, #27064, .T. ) ;
#24096=ORIENTED_EDGE ( 'NONE', *, *, #9009, .F. ) ;
#24097=AXIS2_PLACEMENT_3D ( 'NONE', #42747, #21510, #46440 ) ;
#24098=DIRECTION ( 'NONE',  ( 1.000000000000000000, 0.000000000000000000, 0.000000000000000000 ) ) ;
#24099=AXIS2_PLACEMENT_3D ( 'NONE', #8019, #17660, #53229 ) ;
#24100=VERTEX_POINT ( 'NONE', #56941 ) ;
#24101=FACE_OUTER_BOUND ( 'NONE', #1945, .T. ) ;
#24108=ORIENTED_EDGE ( 'NONE', *, *, #36212, .F. ) ;
#24110=EDGE_CURVE ( 'NONE', #25348, #33198, #61907, .T. ) ;
#24111=ORIENTED_EDGE ( 'NONE', *, *, #29300, .F. ) ;
#24113=ORIENTED_EDGE ( 'NONE', *, *, #63099, .T. ) ;
#24115=DIRECTION ( 'NONE',  ( -1.000000000000000000, 0.000000000000000000, 0.000000000000000000 ) ) ;
#24116=EDGE_CURVE ( 'NONE', #47989, #48505, #63968, .T. ) ;
#24118=CARTESIAN_POINT ( 'NONE',  ( -24.80857425325906718, 8.631266723926000139, 10.38663870023611757 ) ) ;
#24119=CARTESIAN_POINT ( 'NONE',  ( 23.74857913196462178, -3.119318027837767460, 11.59209599145404646 ) ) ;
#24120=CARTESIAN_POINT ( 'NONE',  ( -35.00000000000000000, 11.38112321385055026, -2.905556151562505462 ) ) ;
#24121=ADVANCED_FACE ( 'NONE', ( #11678 ), #31634, .T. ) ;
#24122=CARTESIAN_POINT ( 'NONE',  ( 34.00000000000000000, 11.99999999999999822, 1.469576158976822172E-15 ) ) ;
#24123=ADVANCED_FACE ( 'NONE', ( #57593 ), #17680, .T. ) ;
#24124=VERTEX_POINT ( 'NONE', #37941 ) ;
#24125=ORIENTED_EDGE ( 'NONE', *, *, #42763, .T. ) ;
#24127=ADVANCED_FACE ( 'NONE', ( #58234 ), #51944, .T. ) ;
#24130=LINE ( 'NONE', #38436, #8314 ) ;
#24133=CARTESIAN_POINT ( 'NONE',  ( -35.00000000000000000, -10.91072401419407001, -5.428340790341820821 ) ) ;
#24134=LINE ( 'NONE', #8844, #56462 ) ;
#24135=DIRECTION ( 'NONE',  ( 0.000000000000000000, 0.01356324068817998940, -0.9999080150203990547 ) ) ;
#24137=AXIS2_PLACEMENT_3D ( 'NONE', #24062, #65272, #9390 ) ;
#24138=ORIENTED_EDGE ( 'NONE', *, *, #25371, .F. ) ;
#24139=DIRECTION ( 'NONE',  ( 0.000000000000000000, -0.04924826701373159060, -0.9987865678893284027 ) ) ;
#24141=AXIS2_PLACEMENT_3D ( 'NONE', #17267, #63137, #37867 ) ;
#24142=ADVANCED_FACE ( 'NONE', ( #18984 ), #13333, .T. ) ;
#24143=ORIENTED_EDGE ( 'NONE', *, *, #58947, .F. ) ;
#24144=CARTESIAN_POINT ( 'NONE',  ( -35.00000000000000000, -2.696588552978969933, -12.46157735505192221 ) ) ;
#24145=AXIS2_PLACEMENT_3D ( 'NONE', #42085, #16175, #31775 ) ;
#24146=CARTESIAN_POINT ( 'NONE',  ( -5.806076944307488219, -1.481863301461679772, -11.90854409942760661 ) ) ;
#24147=DIRECTION ( 'NONE',  ( 0.000000000000000000, -0.01356324068817991828, 0.9999080150203990547 ) ) ;
#24149=CARTESIAN_POINT ( 'NONE',  ( 47.00000000000000711, 4.705694406421931860E-17, -3.469127814946512892E-15 ) ) ;
#24151=FACE_OUTER_BOUND ( 'NONE', #13487, .T. ) ;
#24154=CARTESIAN_POINT ( 'NONE',  ( 37.00000000000000711, -7.561043153948031836, -9.557269938331533154 ) ) ;
#24155=CARTESIAN_POINT ( 'NONE',  ( 37.00000000000000711, 5.556331110570566167, 11.47561260193570654 ) ) ;
#24156=ORIENTED_EDGE ( 'NONE', *, *, #47884, .F. ) ;
#24158=FACE_OUTER_BOUND ( 'NONE', #48711, .T. ) ;
#24163=CARTESIAN_POINT ( 'NONE',  ( 2.798553295784531159, 25.00000000000000000, 7.462808788758677814 ) ) ;
#24166=CARTESIAN_POINT ( 'NONE',  ( -9.733281154747491115, -12.57221497072713490, -4.922044890244330340 ) ) ;
#24167=AXIS2_PLACEMENT_3D ( 'NONE', #58308, #3788, #38682 ) ;
#24169=ORIENTED_EDGE ( 'NONE', *, *, #58012, .T. ) ;
#24171=CARTESIAN_POINT ( 'NONE',  ( -7.181456785175555524, 8.540743096806467705, -10.45493698471458188 ) ) ;
#24172=CIRCLE ( 'NONE', #61477, 4.999999999999999112 ) ;
#24173=DIRECTION ( 'NONE',  ( -1.000000000000000000, 0.000000000000000000, 0.000000000000000000 ) ) ;
#24176=CARTESIAN_POINT ( 'NONE',  ( 35.00000000000000000, 4.705694406421931860E-17, -3.469127814946512892E-15 ) ) ;
#24177=CYLINDRICAL_SURFACE ( 'NONE', #17477, 12.18650000000000055 ) ;
#24179=ORIENTED_EDGE ( 'NONE', *, *, #28234, .T. ) ;
#24181=LINE ( 'NONE', #60744, #50191 ) ;
#24182=ORIENTED_EDGE ( 'NONE', *, *, #30960, .T. ) ;
#24183=AXIS2_PLACEMENT_3D ( 'NONE', #16116, #31416, #6156 ) ;
#24185=EDGE_CURVE ( 'NONE', #32335, #21666, #13974, .T. ) ;
#24186=DIRECTION ( 'NONE',  ( 0.000000000000000000, -0.9105187689795911643, 0.4134677391718608597 ) ) ;
#24187=AXIS2_PLACEMENT_3D ( 'NONE', #44153, #18890, #24192 ) ;
#24189=DIRECTION ( 'NONE',  ( 1.000000000000000000, -0.000000000000000000, 0.000000000000000000 ) ) ;
#24190=ORIENTED_EDGE ( 'NONE', *, *, #23419, .T. ) ;
#24192=DIRECTION ( 'NONE',  ( 0.000000000000000000, 0.01356324068817998940, -0.9999080150203990547 ) ) ;
#24193=LINE ( 'NONE', #54798, #35020 ) ;
#24194=EDGE_LOOP ( 'NONE', ( #56195, #41028, #9433, #25331 ) ) ;
#24196=ADVANCED_FACE ( 'NONE', ( #23313 ), #22994, .T. ) ;
#24197=CARTESIAN_POINT ( 'NONE',  ( 37.00000000000000711, -10.64792938439759595, -5.927257550915285833 ) ) ;
#24198=DIRECTION ( 'NONE',  ( 0.000000000000000000, 0.01356324068817998940, -0.9999080150203989437 ) ) ;
#24199=ORIENTED_EDGE ( 'NONE', *, *, #15516, .T. ) ;
#24200=CARTESIAN_POINT ( 'NONE',  ( -27.71554010819489378, -10.41834511119169626, -5.961899762888907439 ) ) ;
#24203=CYLINDRICAL_SURFACE ( 'NONE', #30490, 5.000000000000000888 ) ;
#24208=ORIENTED_EDGE ( 'NONE', *, *, #48826, .F. ) ;
#24210=CARTESIAN_POINT ( 'NONE',  ( -17.88840112149050654, 6.209967363062701473, 10.27068265694474292 ) ) ;
#24217=CARTESIAN_POINT ( 'NONE',  ( -8.891032880924177206, 11.36194426013951997, -3.860857758255646921 ) ) ;
#24218=AXIS2_PLACEMENT_3D ( 'NONE', #49729, #59706, #58747 ) ;
#24222=EDGE_CURVE ( 'NONE', #21760, #25143, #40876, .T. ) ;
#24227=DIRECTION ( 'NONE',  ( 0.000000000000000000, 0.8169148498130295311, -0.5767582926624942319 ) ) ;
#24230=CARTESIAN_POINT ( 'NONE',  ( -35.00000000000000000, 5.927257550915472351, -10.64792938439748937 ) ) ;
#24231=DIRECTION ( 'NONE',  ( -1.000000000000000000, 0.000000000000000000, -0.000000000000000000 ) ) ;
#24233=CARTESIAN_POINT ( 'NONE',  ( -35.00000000000000000, 5.927257550915472351, -10.64792938439748937 ) ) ;
#24236=ORIENTED_EDGE ( 'NONE', *, *, #4032, .F. ) ;
#24242=EDGE_CURVE ( 'NONE', #23409, #61480, #20705, .T. ) ;
#24243=ADVANCED_FACE ( 'NONE', ( #19312 ), #39583, .T. ) ;
#24245=EDGE_CURVE ( 'NONE', #14872, #42626, #10071, .T. ) ;
#24247=EDGE_LOOP ( 'NONE', ( #42409, #58592, #14622, #3219 ) ) ;
#24250=FACE_OUTER_BOUND ( 'NONE', #28921, .T. ) ;
#24251=DIRECTION ( 'NONE',  ( -1.000000000000000000, -0.000000000000000000, 0.000000000000000000 ) ) ;
#24257=VERTEX_POINT ( 'NONE', #9304 ) ;
#24258=ORIENTED_EDGE ( 'NONE', *, *, #37587, .F. ) ;
#24265=EDGE_CURVE ( 'NONE', #58366, #26477, #24930, .T. ) ;
#24267=AXIS2_PLACEMENT_3D ( 'NONE', #54264, #14640, #4726 ) ;
#24268=VERTEX_POINT ( 'NONE', #46230 ) ;
#24269=CIRCLE ( 'NONE', #38070, 5.000000000000000888 ) ;
#24272=CARTESIAN_POINT ( 'NONE',  ( 35.00000000000000000, 9.506317355798490354, 8.496612874013052874 ) ) ;
#24283=ORIENTED_EDGE ( 'NONE', *, *, #5963, .T. ) ;
#24284=CARTESIAN_POINT ( 'NONE',  ( -37.00000000000000711, -8.573591947375380329, 8.029056188533655103 ) ) ;
#24286=DIRECTION ( 'NONE',  ( 0.000000000000000000, 0.01356324068817992175, -0.9999080150203990547 ) ) ;
#24289=EDGE_CURVE ( 'NONE', #27612, #53714, #29199, .T. ) ;
#24290=DIRECTION ( 'NONE',  ( 0.000000000000000000, -0.6745969609292717939, -0.7381862504171902151 ) ) ;
#24291=VERTEX_POINT ( 'NONE', #50237 ) ;
#24293=CARTESIAN_POINT ( 'NONE',  ( -17.66784097051423075, -6.970076762182745078, -11.56512672300377886 ) ) ;
#24295=CARTESIAN_POINT ( 'NONE',  ( -35.00000000000000000, 2.772148766916116891, 11.86701198550357361 ) ) ;
#24297=CARTESIAN_POINT ( 'NONE',  ( -35.00000000000000000, 11.73555825188283386, -4.983891302653459476 ) ) ;
#24298=ORIENTED_EDGE ( 'NONE', *, *, #18030, .T. ) ;
#24299=ORIENTED_EDGE ( 'NONE', *, *, #9834, .T. ) ;
#24300=LINE ( 'NONE', #14628, #44946 ) ;
#24302=AXIS2_PLACEMENT_3D ( 'NONE', #61331, #40384, #16112 ) ;
#24303=EDGE_LOOP ( 'NONE', ( #18691, #59593, #52812, #25655 ) ) ;
#24304=CARTESIAN_POINT ( 'NONE',  ( 9.687175622948609899, 25.00000000000000000, -0.5854820436212360146 ) ) ;
#24307=CARTESIAN_POINT ( 'NONE',  ( -3.472933359965475475, 10.12749893407059254, 6.449612554627071503 ) ) ;
#24308=CARTESIAN_POINT ( 'NONE',  ( 13.36879067795435283, 11.08032463289294256, -4.612831250830367935 ) ) ;
#24310=DIRECTION ( 'NONE',  ( 0.000000000000000000, 0.7617968321374856133, 0.6478160128811973895 ) ) ;
#24311=DIRECTION ( 'NONE',  ( -1.000000000000000000, -0.000000000000000000, 0.000000000000000000 ) ) ;
#24312=CIRCLE ( 'NONE', #9394, 5.000000000000000888 ) ;
#24313=ADVANCED_FACE ( 'NONE', ( #30575 ), #4348, .T. ) ;
#24317=CIRCLE ( 'NONE', #52997, 12.74999999999999822 ) ;
#24318=CARTESIAN_POINT ( 'NONE',  ( 37.00000000000000711, -6.547236723513950807, 9.752226076388957665 ) ) ;
#24320=CARTESIAN_POINT ( 'NONE',  ( -37.00000000000000711, 0.000000000000000000, 0.000000000000000000 ) ) ;
#24321=AXIS2_PLACEMENT_3D ( 'NONE', #28720, #44028, #49373 ) ;
#24323=ORIENTED_EDGE ( 'NONE', *, *, #34026, .T. ) ;
#24324=CARTESIAN_POINT ( 'NONE',  ( 11.07172588725403273, -11.87906629146547210, -1.711250688108173712 ) ) ;
#24325=ORIENTED_EDGE ( 'NONE', *, *, #26344, .T. ) ;
#24330=EDGE_LOOP ( 'NONE', ( #53421, #38017, #20318, #16500 ) ) ;
#24331=ORIENTED_EDGE ( 'NONE', *, *, #30160, .F. ) ;
#24332=VERTEX_POINT ( 'NONE', #35878 ) ;
#24335=AXIS2_PLACEMENT_3D ( 'NONE', #18621, #44184, #35507 ) ;
#24336=CARTESIAN_POINT ( 'NONE',  ( -35.00000000000000000, 9.512294188641000403, -6.891188680298720115 ) ) ;
#24337=ORIENTED_EDGE ( 'NONE', *, *, #1365, .F. ) ;
#24339=DIRECTION ( 'NONE',  ( -1.000000000000000000, -1.836970198721029688E-16, 0.000000000000000000 ) ) ;
#24341=CARTESIAN_POINT ( 'NONE',  ( -35.00000000000000000, -7.718225330433740261, -9.430788938294131896 ) ) ;
#24343=DIRECTION ( 'NONE',  ( 0.000000000000000000, 0.01356324068818000328, -0.9999080150203990547 ) ) ;
#24346=CARTESIAN_POINT ( 'NONE',  ( -32.16141091265169649, 25.00000000000000000, 5.384978440493686236 ) ) ;
#24347=CARTESIAN_POINT ( 'NONE',  ( -35.00000000000000000, -12.49688848680886188, 2.527899948230592830 ) ) ;
#24348=EDGE_LOOP ( 'NONE', ( #4420, #63566, #5314, #56087 ) ) ;
#24354=CARTESIAN_POINT ( 'NONE',  ( 13.24596223717851373, -11.31509987884708046, -4.002165216063023223 ) ) ;
#24355=CIRCLE ( 'NONE', #29615, 5.000000000000000000 ) ;
#24356=LINE ( 'NONE', #55272, #28738 ) ;
#24358=EDGE_CURVE ( 'NONE', #64321, #10113, #26025, .T. ) ;
#24360=CARTESIAN_POINT ( 'NONE',  ( -7.721880503586887379, -2.140633088631647585, -13.33031841795283512 ) ) ;
#24362=DIRECTION ( 'NONE',  ( -1.000000000000000000, 0.000000000000000000, 0.000000000000000000 ) ) ;
#24364=CIRCLE ( 'NONE', #8426, 12.18650000000000233 ) ;
#24365=ORIENTED_EDGE ( 'NONE', *, *, #48152, .F. ) ;
#24366=CYLINDRICAL_SURFACE ( 'NONE', #17875, 4.725920239717170901 ) ;
#24373=DIRECTION ( 'NONE',  ( 0.000000000000000000, 0.01356324068817991828, -0.9999080150203990547 ) ) ;
#24375=DIRECTION ( 'NONE',  ( 0.000000000000000000, -0.01356324068817999114, 0.9999080150203989437 ) ) ;
#24376=DIRECTION ( 'NONE',  ( 0.000000000000000000, 0.01356324068817991828, -0.9999080150203990547 ) ) ;
#24377=EDGE_CURVE ( 'NONE', #416, #24479, #30903, .T. ) ;
#24380=CARTESIAN_POINT ( 'NONE',  ( -35.00000000000000000, 11.01837265713082203, -6.415447294506590126 ) ) ;
#24383=CARTESIAN_POINT ( 'NONE',  ( -18.06762394718330711, -4.853757295686705220, 12.59799896500893190 ) ) ;
#24384=ORIENTED_EDGE ( 'NONE', *, *, #36263, .T. ) ;
#24385=CIRCLE ( 'NONE', #29689, 12.18650000000000411 ) ;
#24386=CIRCLE ( 'NONE', #55342, 12.18650000000000055 ) ;
#24387=EDGE_CURVE ( 'NONE', #46364, #46522, #5899, .T. ) ;
#24388=AXIS2_PLACEMENT_3D ( 'NONE', #49669, #43681, #29063 ) ;
#24391=VERTEX_POINT ( 'NONE', #10298 ) ;
#24395=DIRECTION ( 'NONE',  ( 0.9703875065674330003, 0.000000000000000000, 0.2415534870330798278 ) ) ;
#24396=AXIS2_PLACEMENT_3D ( 'NONE', #28273, #48569, #3019 ) ;
#24397=ADVANCED_FACE ( 'NONE', ( #42180 ), #57852, .T. ) ;
#24398=DIRECTION ( 'NONE',  ( 1.000000000000000000, 0.000000000000000000, -0.000000000000000000 ) ) ;
#24399=CARTESIAN_POINT ( 'NONE',  ( 6.361445718264521432, -4.355102044641763648, 25.00000000000000000 ) ) ;
#24400=AXIS2_PLACEMENT_3D ( 'NONE', #15081, #20742, #35361 ) ;
#24402=CARTESIAN_POINT ( 'NONE',  ( -37.00000000000000711, 2.143131898507868297E-16, 1.750000000000000000 ) ) ;
#24404=LINE ( 'NONE', #54023, #8459 ) ;
#24405=VERTEX_POINT ( 'NONE', #21261 ) ;
#24406=CARTESIAN_POINT ( 'NONE',  ( 8.437200413559441614, 4.215340780676140930, 12.82799475126035560 ) ) ;
#24407=DIRECTION ( 'NONE',  ( 0.5417962735734949131, 0.000000000000000000, -0.8405098440481674205 ) ) ;
#24408=ORIENTED_EDGE ( 'NONE', *, *, #34224, .T. ) ;
#24409=CIRCLE ( 'NONE', #3222, 5.000000000000000888 ) ;
#24410=ORIENTED_EDGE ( 'NONE', *, *, #28061, .F. ) ;
#24411=ORIENTED_EDGE ( 'NONE', *, *, #63802, .F. ) ;
#24413=VERTEX_POINT ( 'NONE', #7272 ) ;
#24414=LINE ( 'NONE', #4149, #18578 ) ;
#24416=CYLINDRICAL_SURFACE ( 'NONE', #11021, 5.000000000000000888 ) ;
#24421=ORIENTED_EDGE ( 'NONE', *, *, #33784, .T. ) ;
#24423=ORIENTED_EDGE ( 'NONE', *, *, #47234, .F. ) ;
#24425=ORIENTED_EDGE ( 'NONE', *, *, #15098, .F. ) ;
#24430=EDGE_CURVE ( 'NONE', #5232, #27547, #27557, .T. ) ;
#24431=CIRCLE ( 'NONE', #45653, 5.000000000000000888 ) ;
#24432=AXIS2_PLACEMENT_3D ( 'NONE', #39420, #29760, #59721 ) ;
#24433=CARTESIAN_POINT ( 'NONE',  ( 23.55819837055134158, -3.414313941384615081, 11.50760599575436949 ) ) ;
#24435=DIRECTION ( 'NONE',  ( -1.000000000000000000, 0.000000000000000000, -0.000000000000000000 ) ) ;
#24436=ORIENTED_EDGE ( 'NONE', *, *, #39937, .T. ) ;
#24437=ORIENTED_EDGE ( 'NONE', *, *, #12276, .T. ) ;
#24439=VERTEX_POINT ( 'NONE', #31564 ) ;
#24440=ORIENTED_EDGE ( 'NONE', *, *, #7151, .T. ) ;
#24444=DIRECTION ( 'NONE',  ( -0.000000000000000000, -0.000000000000000000, -1.000000000000000000 ) ) ;
#24446=CIRCLE ( 'NONE', #15942, 5.000000000000000888 ) ;
#24447=DIRECTION ( 'NONE',  ( 0.6147887355352468219, -0.7886918350401329603, 0.000000000000000000 ) ) ;
#24448=ADVANCED_FACE ( 'NONE', ( #47855 ), #51867, .T. ) ;
#24449=CARTESIAN_POINT ( 'NONE',  ( 26.34661844826604593, -13.08594712317289321, 3.317828791472332117 ) ) ;
#24451=VERTEX_POINT ( 'NONE', #16934 ) ;
#24453=EDGE_CURVE ( 'NONE', #57089, #19006, #25306, .T. ) ;
#24454=ORIENTED_EDGE ( 'NONE', *, *, #61949, .T. ) ;
#24456=CARTESIAN_POINT ( 'NONE',  ( 35.00000000000000000, -10.91072401419414462, -5.428340790341669830 ) ) ;
#24458=DIRECTION ( 'NONE',  ( 0.000000000000000000, -0.01356324068817992001, 0.9999080150203990547 ) ) ;
#24460=CARTESIAN_POINT ( 'NONE',  ( -35.00000000000000000, 3.307597835713244283, 12.31350058095524247 ) ) ;
#24461=ADVANCED_FACE ( 'NONE', ( #1332 ), #11295, .T. ) ;
#24462=CARTESIAN_POINT ( 'NONE',  ( 6.918530584243898218, -8.212880376810627325, -10.72188286460056439 ) ) ;
#24463=EDGE_CURVE ( 'NONE', #8336, #52191, #50804, .T. ) ;
#24465=CARTESIAN_POINT ( 'NONE',  ( 35.00000000000000000, 10.63508530065521640, -4.986700593229742573 ) ) ;
#24466=CARTESIAN_POINT ( 'NONE',  ( 9.575800908719084958, -11.95193887484098028, -1.072919909436247154 ) ) ;
#24468=ORIENTED_EDGE ( 'NONE', *, *, #50266, .T. ) ;
#24469=LINE ( 'NONE', #64060, #46284 ) ;
#24471=DIRECTION ( 'NONE',  ( 0.000000000000000000, -0.01356324068817998593, 0.9999080150203990547 ) ) ;
#24472=ADVANCED_FACE ( 'NONE', ( #6005 ), #62163, .T. ) ;
#24473=AXIS2_PLACEMENT_3D ( 'NONE', #1920, #58440, #33150 ) ;
#24474=CIRCLE ( 'NONE', #56334, 12.74999999999999822 ) ;
#24476=ADVANCED_FACE ( 'NONE', ( #12267 ), #41535, .T. ) ;
#24479=VERTEX_POINT ( 'NONE', #1974 ) ;
#24483=EDGE_CURVE ( 'NONE', #41989, #26974, #57180, .T. ) ;
#24488=DIRECTION ( 'NONE',  ( 1.000000000000000000, 0.000000000000000000, -0.000000000000000000 ) ) ;
#24492=DIRECTION ( 'NONE',  ( 1.000000000000000000, 0.000000000000000000, 0.000000000000000000 ) ) ;
#24493=ORIENTED_EDGE ( 'NONE', *, *, #53609, .T. ) ;
#24497=CARTESIAN_POINT ( 'NONE',  ( 35.00000000000000000, -7.718225330433870823, -9.430788938294027091 ) ) ;
#24498=CARTESIAN_POINT ( 'NONE',  ( 37.00000000000000711, -8.017674001891711200, 9.913596905230193101 ) ) ;
#24500=DIRECTION ( 'NONE',  ( 0.000000000000000000, 0.01356324068817998940, -0.9999080150203990547 ) ) ;
#24501=CARTESIAN_POINT ( 'NONE',  ( -35.00000000000000000, -11.91791701451264629, -2.544412758415973030 ) ) ;
#24502=AXIS2_PLACEMENT_3D ( 'NONE', #5424, #91, #25361 ) ;
#24505=VERTEX_POINT ( 'NONE', #61828 ) ;
#24506=EDGE_LOOP ( 'NONE', ( #19274, #5018, #55955, #64851 ) ) ;
#24507=CARTESIAN_POINT ( 'NONE',  ( -18.24855926006501505, -5.449082428673613698, -10.69225419630004481 ) ) ;
#24509=VERTEX_POINT ( 'NONE', #56872 ) ;
#24510=CARTESIAN_POINT ( 'NONE',  ( 3.423896178748679020, -10.94279856996580413, -7.910751437345123982 ) ) ;
#24511=EDGE_CURVE ( 'NONE', #62855, #22570, #33791, .T. ) ;
#24512=EDGE_CURVE ( 'NONE', #15438, #11272, #56105, .T. ) ;
#24513=CARTESIAN_POINT ( 'NONE',  ( -17.83419946441818027, -9.720786832536937538, 9.367833439828872955 ) ) ;
#24515=DIRECTION ( 'NONE',  ( -1.000000000000000000, -0.000000000000000000, 0.000000000000000000 ) ) ;
#24516=CARTESIAN_POINT ( 'NONE',  ( 12.64346310766591586, 9.915289356383874875, -6.770812359651990242 ) ) ;
#24517=DIRECTION ( 'NONE',  ( -1.000000000000000000, -1.836970198721029688E-16, -0.000000000000000000 ) ) ;
#24519=VERTEX_POINT ( 'NONE', #46871 ) ;
#24521=DIRECTION ( 'NONE',  ( 1.000000000000000000, -0.000000000000000000, 0.000000000000000000 ) ) ;
#24522=EDGE_CURVE ( 'NONE', #30009, #37953, #55021, .T. ) ;
#24523=ORIENTED_EDGE ( 'NONE', *, *, #9414, .T. ) ;
#24524=FACE_OUTER_BOUND ( 'NONE', #39841, .T. ) ;
#24529=VECTOR ( 'NONE', #41810, 1000.000000000000000 ) ;
#24532=AXIS2_PLACEMENT_3D ( 'NONE', #1297, #36848, #26542 ) ;
#24533=EDGE_CURVE ( 'NONE', #26974, #40555, #31881, .T. ) ;
#24534=CARTESIAN_POINT ( 'NONE',  ( -14.11589373245165469, 8.250315036047107142, -10.68561190601526256 ) ) ;
#24535=EDGE_LOOP ( 'NONE', ( #33110, #43, #32992, #64185 ) ) ;
#24537=CIRCLE ( 'NONE', #7382, 4.999999999999999112 ) ;
#24539=DIRECTION ( 'NONE',  ( 1.000000000000000000, 0.000000000000000000, -0.000000000000000000 ) ) ;
#24541=CYLINDRICAL_SURFACE ( 'NONE', #16823, 4.999999999999999112 ) ;
#24542=CARTESIAN_POINT ( 'NONE',  ( -20.74400292461320916, 13.15690609773952602, -3.073985401093241254 ) ) ;
#24543=CARTESIAN_POINT ( 'NONE',  ( 24.18616158388540782, -2.148571468477003865, 13.33263367692836177 ) ) ;
#24544=DIRECTION ( 'NONE',  ( -1.000000000000000000, 0.000000000000000000, 0.000000000000000000 ) ) ;
#24545=CARTESIAN_POINT ( 'NONE',  ( -35.00000000000000000, -8.766823244862047559, 7.817610399097479679 ) ) ;
#24547=CIRCLE ( 'NONE', #44752, 5.000000000000000888 ) ;
#24548=ORIENTED_EDGE ( 'NONE', *, *, #62647, .T. ) ;
#24549=CIRCLE ( 'NONE', #61703, 12.18650000000000055 ) ;
#24550=AXIS2_PLACEMENT_3D ( 'NONE', #58311, #38008, #22743 ) ;
#24551=VERTEX_POINT ( 'NONE', #3943 ) ;
#24554=ADVANCED_FACE ( 'NONE', ( #13262 ), #37870, .T. ) ;
#24555=CARTESIAN_POINT ( 'NONE',  ( 35.00000000000000000, 4.705694406421931860E-17, -3.469127814946512892E-15 ) ) ;
#24556=FACE_OUTER_BOUND ( 'NONE', #24330, .T. ) ;
#24557=CARTESIAN_POINT ( 'NONE',  ( 37.00000000000000711, -11.59095880812006385, 1.903127969211307224 ) ) ;
#24558=ORIENTED_EDGE ( 'NONE', *, *, #51591, .T. ) ;
#24559=CARTESIAN_POINT ( 'NONE',  ( 145.1370849898475797, 3.309064568108273190E-14, 0.000000000000000000 ) ) ;
#24560=CARTESIAN_POINT ( 'NONE',  ( -29.92777678363736626, -3.750539801530011985, -11.39883551934752681 ) ) ;
#24561=AXIS2_PLACEMENT_3D ( 'NONE', #39826, #13880, #29509 ) ;
#24562=DIRECTION ( 'NONE',  ( 1.000000000000000000, 0.000000000000000000, 0.000000000000000000 ) ) ;
#24564=EDGE_CURVE ( 'NONE', #34567, #8663, #63503, .T. ) ;
#24566=AXIS2_PLACEMENT_3D ( 'NONE', #33537, #28867, #29506 ) ;
#24568=ORIENTED_EDGE ( 'NONE', *, *, #23439, .F. ) ;
#24569=CARTESIAN_POINT ( 'NONE',  ( -35.00000000000000000, 0.000000000000000000, 0.000000000000000000 ) ) ;
#24572=CIRCLE ( 'NONE', #43694, 12.18650000000000233 ) ;
#24574=CARTESIAN_POINT ( 'NONE',  ( -36.00000000000000711, 5.556331110570408960, 11.47561260193578825 ) ) ;
#24575=CARTESIAN_POINT ( 'NONE',  ( -2.816255946208519934, -7.711081843936708147, 11.08213906273405769 ) ) ;
#24576=LINE ( 'NONE', #28918, #59624 ) ;
#24577=CIRCLE ( 'NONE', #11791, 12.75000000000000178 ) ;
#24579=VECTOR ( 'NONE', #63088, 1000.000000000000000 ) ;
#24581=ORIENTED_EDGE ( 'NONE', *, *, #30455, .F. ) ;
#24583=ORIENTED_EDGE ( 'NONE', *, *, #11458, .T. ) ;
#24585=DIRECTION ( 'NONE',  ( 1.000000000000000000, 0.000000000000000000, 0.000000000000000000 ) ) ;
#24586=CARTESIAN_POINT ( 'NONE',  ( -35.00000000000000000, 11.44858830469740241, -2.627174906296955381 ) ) ;
#24587=LINE ( 'NONE', #59508, #19460 ) ;
#24588=DIRECTION ( 'NONE',  ( 1.000000000000000000, 0.000000000000000000, 0.000000000000000000 ) ) ;
#24589=LINE ( 'NONE', #44867, #8371 ) ;
#24590=CARTESIAN_POINT ( 'NONE',  ( -18.77940254910617668, -11.98723174400094393, 0.6435659898533969692 ) ) ;
#24595=VECTOR ( 'NONE', #9798, 1000.000000000000000 ) ;
#24596=CIRCLE ( 'NONE', #58555, 5.000000000000000888 ) ;
#24597=DIRECTION ( 'NONE',  ( -1.000000000000000000, 0.000000000000000000, 0.000000000000000000 ) ) ;
#24598=EDGE_CURVE ( 'NONE', #18920, #48103, #7268, .T. ) ;
#24599=ORIENTED_EDGE ( 'NONE', *, *, #39092, .T. ) ;
#24600=AXIS2_PLACEMENT_3D ( 'NONE', #19158, #50086, #4545 ) ;
#24601=FACE_BOUND ( 'NONE', #4336, .T. ) ;
#24603=ORIENTED_EDGE ( 'NONE', *, *, #7803, .F. ) ;
#24605=FACE_OUTER_BOUND ( 'NONE', #16495, .T. ) ;
#24607=ORIENTED_EDGE ( 'NONE', *, *, #37642, .F. ) ;
#24608=AXIS2_PLACEMENT_3D ( 'NONE', #44614, #24043, #33359 ) ;
#24609=EDGE_LOOP ( 'NONE', ( #44121, #30260, #37335, #52992 ) ) ;
#24611=EDGE_LOOP ( 'NONE', ( #58543, #20237, #64500, #53806 ) ) ;
#24613=EDGE_CURVE ( 'NONE', #63532, #58825, #23176, .T. ) ;
#24616=ORIENTED_EDGE ( 'NONE', *, *, #63921, .T. ) ;
#24617=CARTESIAN_POINT ( 'NONE',  ( 35.00000000000000000, 3.640372113593551173, -12.21925492305363470 ) ) ;
#24619=DIRECTION ( 'NONE',  ( -0.000000000000000000, -1.000000000000000000, -0.000000000000000000 ) ) ;
#24620=CARTESIAN_POINT ( 'NONE',  ( -35.00000000000000000, 9.677500615117999416, -6.657191900728212985 ) ) ;
#24621=VERTEX_POINT ( 'NONE', #7960 ) ;
#24623=AXIS2_PLACEMENT_3D ( 'NONE', #55038, #6814, #21098 ) ;
#24624=ORIENTED_EDGE ( 'NONE', *, *, #37551, .T. ) ;
#24625=DIRECTION ( 'NONE',  ( -1.000000000000000000, 0.000000000000000000, 0.000000000000000000 ) ) ;
#24626=DIRECTION ( 'NONE',  ( 0.000000000000000000, -0.01356324068817991828, 0.9999080150203990547 ) ) ;
#24628=EDGE_CURVE ( 'NONE', #10393, #6306, #59309, .T. ) ;
#24631=CARTESIAN_POINT ( 'NONE',  ( -37.00000000000000711, 2.216820770815248309, -11.53507381115581332 ) ) ;
#24637=CIRCLE ( 'NONE', #61785, 5.000000000000000888 ) ;
#24641=DIRECTION ( 'NONE',  ( 1.000000000000000000, 0.000000000000000000, 0.000000000000000000 ) ) ;
#24645=CARTESIAN_POINT ( 'NONE',  ( 12.60640452496583030, 11.71824542652569079, -2.591698231487439497 ) ) ;
#24647=CARTESIAN_POINT ( 'NONE',  ( -37.00000000000000711, -3.916263239775430005, 11.07407352312211302 ) ) ;
#24648=FACE_OUTER_BOUND ( 'NONE', #58744, .T. ) ;
#24649=FACE_OUTER_BOUND ( 'NONE', #7165, .T. ) ;
#24650=VECTOR ( 'NONE', #28378, 1000.000000000000000 ) ;
#24658=ADVANCED_FACE ( 'NONE', ( #59152 ), #13563, .T. ) ;
#24660=CARTESIAN_POINT ( 'NONE',  ( -27.45775109278351067, 25.00000000000000000, -8.471355351200609007 ) ) ;
#24661=EDGE_CURVE ( 'NONE', #46638, #61418, #45471, .T. ) ;
#24662=ORIENTED_EDGE ( 'NONE', *, *, #57584, .F. ) ;
#24663=CARTESIAN_POINT ( 'NONE',  ( -37.00000000000000711, -6.036400161834495570, -10.07641281632183983 ) ) ;
#24665=FACE_OUTER_BOUND ( 'NONE', #46579, .T. ) ;
#24667=CARTESIAN_POINT ( 'NONE',  ( 16.78263030916553333, 25.00000000000000000, 5.836879698929882565 ) ) ;
#24670=ORIENTED_EDGE ( 'NONE', *, *, #33623, .F. ) ;
#24671=CIRCLE ( 'NONE', #8868, 5.000000000000000888 ) ;
#24672=ORIENTED_EDGE ( 'NONE', *, *, #39937, .F. ) ;
#24675=DIRECTION ( 'NONE',  ( 0.000000000000000000, -0.01356324068817998940, 0.9999080150203990547 ) ) ;
#24676=LINE ( 'NONE', #4407, #43800 ) ;
#24677=AXIS2_PLACEMENT_3D ( 'NONE', #58359, #12779, #28105 ) ;
#24680=FACE_OUTER_BOUND ( 'NONE', #36954, .T. ) ;
#24681=DIRECTION ( 'NONE',  ( 0.000000000000000000, -0.5243256840888443904, -0.8515178078024941977 ) ) ;
#24682=CARTESIAN_POINT ( 'NONE',  ( 37.00000000000000711, 4.705694406421931860E-17, -3.469127814946512892E-15 ) ) ;
#24683=EDGE_CURVE ( 'NONE', #56961, #57088, #19564, .T. ) ;
#24685=CARTESIAN_POINT ( 'NONE',  ( 16.78263030916553333, 25.00000000000000000, 5.836879698929882565 ) ) ;
#24687=DIRECTION ( 'NONE',  ( -1.000000000000000000, 0.000000000000000000, 0.000000000000000000 ) ) ;
#24689=ORIENTED_EDGE ( 'NONE', *, *, #2489, .F. ) ;
#24690=CARTESIAN_POINT ( 'NONE',  ( -37.00000000000000711, 6.950793414699792727, 10.68873102412845100 ) ) ;
#24694=DIRECTION ( 'NONE',  ( 0.000000000000000000, -0.6943713148249691658, 0.7196168960969744344 ) ) ;
#24695=CIRCLE ( 'NONE', #21518, 5.000000000000000888 ) ;
#24696=DIRECTION ( 'NONE',  ( 0.000000000000000000, -0.7381862504172023165, 0.6745969609292585822 ) ) ;
#24698=DIRECTION ( 'NONE',  ( 1.000000000000000000, 0.000000000000000000, -0.000000000000000000 ) ) ;
#24703=CARTESIAN_POINT ( 'NONE',  ( 36.00000000000000711, -12.42372387097884001, -2.865935305911582631 ) ) ;
#24704=DIRECTION ( 'NONE',  ( 0.000000000000000000, -0.9937233664769749009, 0.1118654143051720229 ) ) ;
#24706=AXIS2_PLACEMENT_3D ( 'NONE', #21672, #62525, #41926 ) ;
#24707=VERTEX_POINT ( 'NONE', #60771 ) ;
#24708=CARTESIAN_POINT ( 'NONE',  ( 11.31411741755062295, -13.43902530517520866, -1.288601721348704654 ) ) ;
#24709=VERTEX_POINT ( 'NONE', #24872 ) ;
#24711=EDGE_CURVE ( 'NONE', #29943, #57229, #51495, .T. ) ;
#24712=ORIENTED_EDGE ( 'NONE', *, *, #52579, .T. ) ;
#24713=DIRECTION ( 'NONE',  ( 0.000000000000000000, -0.01356324068817992175, 0.9999080150203990547 ) ) ;
#24714=DIRECTION ( 'NONE',  ( 0.000000000000000000, 0.01356324068817998940, -0.9999080150203990547 ) ) ;
#24716=LINE ( 'NONE', #40984, #16361 ) ;
#24717=DIRECTION ( 'NONE',  ( 0.000000000000000000, 0.01356324068817998940, -0.9999080150203990547 ) ) ;
#24719=EDGE_CURVE ( 'NONE', #8244, #11975, #14224, .T. ) ;
#24720=CARTESIAN_POINT ( 'NONE',  ( 35.00000000000000000, -12.49688848680881748, 2.527899948230766913 ) ) ;
#24721=FACE_OUTER_BOUND ( 'NONE', #13345, .T. ) ;
#24724=DIRECTION ( 'NONE',  ( -0.6147887355352408267, -0.7886918350401376232, 0.000000000000000000 ) ) ;
#24726=CARTESIAN_POINT ( 'NONE',  ( -18.17110097162331428, -4.731948580995131159, 12.64413186530607014 ) ) ;
#24727=ORIENTED_EDGE ( 'NONE', *, *, #32131, .F. ) ;
#24728=VECTOR ( 'NONE', #19437, 1000.000000000000000 ) ;
#24729=EDGE_CURVE ( 'NONE', #62669, #43307, #29523, .T. ) ;
#24733=CARTESIAN_POINT ( 'NONE',  ( -35.00000000000000000, 0.8294751490781091530, -12.15823808070321732 ) ) ;
#24735=CARTESIAN_POINT ( 'NONE',  ( -10.89134765133834293, -7.913666455164804603, -10.93997517974822387 ) ) ;
#24736=DIRECTION ( 'NONE',  ( 0.000000000000000000, -0.7381862504172023165, 0.6745969609292585822 ) ) ;
#24738=LINE ( 'NONE', #10093, #20280 ) ;
#24740=DIRECTION ( 'NONE',  ( 1.000000000000000000, 0.000000000000000000, 0.000000000000000000 ) ) ;
#24741=VECTOR ( 'NONE', #40590, 1000.000000000000000 ) ;
#24742=EDGE_CURVE ( 'NONE', #26468, #24709, #864, .T. ) ;
#24743=CIRCLE ( 'NONE', #61901, 5.000000000000000888 ) ;
#24746=EDGE_LOOP ( 'NONE', ( #41017, #11064, #45378, #28636 ) ) ;
#24748=DIRECTION ( 'NONE',  ( 1.000000000000000000, -0.000000000000000000, -0.000000000000000000 ) ) ;
#24749=AXIS2_PLACEMENT_3D ( 'NONE', #18516, #59069, #13477 ) ;
#24750=DIRECTION ( 'NONE',  ( 0.000000000000000000, 0.4134677391718510897, 0.9105187689795954942 ) ) ;
#24751=ORIENTED_EDGE ( 'NONE', *, *, #53839, .T. ) ;
#24752=CARTESIAN_POINT ( 'NONE',  ( 8.936348816238876225, 2.397984168018178153, 13.28748829145446919 ) ) ;
#24754=ORIENTED_EDGE ( 'NONE', *, *, #39399, .T. ) ;
#24755=EDGE_LOOP ( 'NONE', ( #62322, #51675, #7678, #54075 ) ) ;
#24757=VECTOR ( 'NONE', #65356, 1000.000000000000000 ) ;
#24758=ORIENTED_EDGE ( 'NONE', *, *, #54972, .T. ) ;
#24759=DIRECTION ( 'NONE',  ( 0.000000000000000000, 0.5472293298355273006, -0.8369827122275342868 ) ) ;
#24760=DIRECTION ( 'NONE',  ( 0.000000000000000000, -0.9903235168508564001, -0.1387779952735713473 ) ) ;
#24761=CARTESIAN_POINT ( 'NONE',  ( -35.00000000000000000, 0.000000000000000000, 0.000000000000000000 ) ) ;
#24764=CARTESIAN_POINT ( 'NONE',  ( 22.88594695219327235, 3.421158645304719137, -13.05931366970166962 ) ) ;
#24766=ORIENTED_EDGE ( 'NONE', *, *, #50382, .T. ) ;
#24767=EDGE_CURVE ( 'NONE', #31684, #31935, #34824, .T. ) ;
#24768=DIRECTION ( 'NONE',  ( 0.000000000000000000, -0.01356324068817998940, 0.9999080150203990547 ) ) ;
#24770=AXIS2_PLACEMENT_3D ( 'NONE', #44865, #45197, #3349 ) ;
#24771=CYLINDRICAL_SURFACE ( 'NONE', #29573, 4.999999999999999112 ) ;
#24772=ORIENTED_EDGE ( 'NONE', *, *, #21642, .T. ) ;
#24773=AXIS2_PLACEMENT_3D ( 'NONE', #58739, #33749, #39397 ) ;
#24774=ORIENTED_EDGE ( 'NONE', *, *, #7957, .F. ) ;
#24777=CIRCLE ( 'NONE', #33264, 12.74999999999999822 ) ;
#24779=CIRCLE ( 'NONE', #59807, 4.999999999999999112 ) ;
#24781=CARTESIAN_POINT ( 'NONE',  ( -35.00000000000000000, -11.54110654723650420, 2.185196060783841432 ) ) ;
#24782=DIRECTION ( 'NONE',  ( -1.000000000000000000, -0.000000000000000000, 0.000000000000000000 ) ) ;
#24783=DIRECTION ( 'NONE',  ( 0.000000000000000000, 0.01356324068817992175, -0.9999080150203990547 ) ) ;
#24784=ORIENTED_EDGE ( 'NONE', *, *, #47600, .F. ) ;
#24786=DIRECTION ( 'NONE',  ( -1.000000000000000000, 0.000000000000000000, 0.000000000000000000 ) ) ;
#24787=ORIENTED_EDGE ( 'NONE', *, *, #58195, .F. ) ;
#24788=CIRCLE ( 'NONE', #4630, 5.000000000000000888 ) ;
#24789=ADVANCED_FACE ( 'NONE', ( #61096 ), #59791, .T. ) ;
#24790=VERTEX_POINT ( 'NONE', #50792 ) ;
#24793=CARTESIAN_POINT ( 'NONE',  ( 18.70366329277965178, -2.125550911571206569, 11.85937264694274518 ) ) ;
#24794=CARTESIAN_POINT ( 'NONE',  ( -35.00000000000000000, 10.54834585426219995, 6.102719229070713070 ) ) ;
#24795=CIRCLE ( 'NONE', #39636, 5.000000000000001776 ) ;
#24796=CARTESIAN_POINT ( 'NONE',  ( -11.40165637463000259, -7.158503671335326501, -9.641458581199431777 ) ) ;
#24797=DIRECTION ( 'NONE',  ( -1.000000000000000000, 0.000000000000000000, 0.000000000000000000 ) ) ;
#24798=EDGE_LOOP ( 'NONE', ( #21265, #56917, #22136, #35413, #14297, #23264, #1496, #30316, #63325, #28593, #21340, #1041 ) ) ;
#24801=CIRCLE ( 'NONE', #32238, 12.18650000000000411 ) ;
#24804=FACE_OUTER_BOUND ( 'NONE', #42886, .T. ) ;
#24805=CARTESIAN_POINT ( 'NONE',  ( 6.680451748998780026, -7.311972598139333535, 9.517076143087459528 ) ) ;
#24806=VECTOR ( 'NONE', #41188, 1000.000000000000000 ) ;
#24808=CARTESIAN_POINT ( 'NONE',  ( 7.182606707284545422, -7.361254329974325827, -11.31839762553341622 ) ) ;
#24809=FACE_OUTER_BOUND ( 'NONE', #65249, .T. ) ;
#24812=ORIENTED_EDGE ( 'NONE', *, *, #12305, .T. ) ;
#24813=VECTOR ( 'NONE', #28506, 1000.000000000000000 ) ;
#24814=CARTESIAN_POINT ( 'NONE',  ( -21.17861794710831091, 11.44571409049744304, -3.604945070120774808 ) ) ;
#24816=AXIS2_PLACEMENT_3D ( 'NONE', #51031, #9793, #50047 ) ;
#24821=CARTESIAN_POINT ( 'NONE',  ( -28.06993472828175484, -9.866117616252182643, -6.837783180416262319 ) ) ;
#24823=CARTESIAN_POINT ( 'NONE',  ( -37.00000000000000711, 4.018060380616562455, -11.50504120060938718 ) ) ;
#24827=ORIENTED_EDGE ( 'NONE', *, *, #8513, .F. ) ;
#24829=CARTESIAN_POINT ( 'NONE',  ( 47.00000000000000711, 4.705694406421931860E-17, -3.469127814946512892E-15 ) ) ;
#24831=AXIS2_PLACEMENT_3D ( 'NONE', #30758, #35742, #51074 ) ;
#24834=VECTOR ( 'NONE', #8088, 1000.000000000000000 ) ;
#24835=EDGE_CURVE ( 'NONE', #13080, #26919, #5242, .T. ) ;
#24837=EDGE_LOOP ( 'NONE', ( #41638, #60898, #23996, #39890 ) ) ;
#24838=CARTESIAN_POINT ( 'NONE',  ( -35.00000000000000000, 11.02904044024209185, -4.041347439435899247 ) ) ;
#24842=CARTESIAN_POINT ( 'NONE',  ( 0.2851083653049530375, -0.4107471485392680810, -13.49374991542258151 ) ) ;
#24844=AXIS2_PLACEMENT_3D ( 'NONE', #40137, #20198, #14534 ) ;
#24845=CARTESIAN_POINT ( 'NONE',  ( 35.00000000000000000, 4.705694406421931860E-17, -3.469127814946512892E-15 ) ) ;
#24850=DIRECTION ( 'NONE',  ( -1.000000000000000000, 0.000000000000000000, 0.000000000000000000 ) ) ;
#24852=FACE_OUTER_BOUND ( 'NONE', #21497, .T. ) ;
#24856=ORIENTED_EDGE ( 'NONE', *, *, #29067, .T. ) ;
#24858=( BOUNDED_CURVE ( )  B_SPLINE_CURVE ( 3, ( #49779, #29804, #20167, #4228 ),
 .UNSPECIFIED., .F., .F. ) 
 B_SPLINE_CURVE_WITH_KNOTS ( ( 4, 4 ),
 ( 0.3740640042953261024, 0.4316535298590248870 ),
 .UNSPECIFIED. ) 
 CURVE ( )  GEOMETRIC_REPRESENTATION_ITEM ( )  RATIONAL_B_SPLINE_CURVE ( ( 1.000000000000000000, 0.9997236396413186066, 0.9997236396413186066, 1.000000000000000000 ) ) 
 REPRESENTATION_ITEM ( '' )  );
#24859=LINE ( 'NONE', #55772, #23153 ) ;
#24860=CARTESIAN_POINT ( 'NONE',  ( 35.00000000000000000, -6.711949091238068377, 10.84030624090613060 ) ) ;
#24861=EDGE_CURVE ( 'NONE', #12647, #36193, #1971, .T. ) ;
#24863=B_SPLINE_CURVE_WITH_KNOTS ( 'NONE', 3,
 ( #48632, #18039, #58279, #59263, #12697, #53290, #38301, #33654, #13046, #53944, #33331, #53631, #28338, #48970, #3089, #38648, #63907, #8385, #3427, #9677, #39947, #29969, #24324, #39287, #44589, #34304 ),
 .UNSPECIFIED., .F., .F.,
 ( 4, 2, 2, 2, 2, 2, 2, 2, 2, 2, 2, 2, 4 ),
 ( 0.000000000000000000, 0.001208835475306771490, 0.001813253212960158969, 0.002417670950613546449, 0.003626506425920317939, 0.004230924163573704551, 0.004835341901227091163, 0.005439759638880478643, 0.006044177376533865255, 0.006648595114187251867, 0.007253012851840638479, 0.008461848327147414306, 0.009670683802454189265 ),
 .UNSPECIFIED. ) ;
#24864=ORIENTED_EDGE ( 'NONE', *, *, #6444, .F. ) ;
#24866=AXIS2_PLACEMENT_3D ( 'NONE', #29544, #56131, #45496 ) ;
#24867=ORIENTED_EDGE ( 'NONE', *, *, #64686, .F. ) ;
#24868=DIRECTION ( 'NONE',  ( 0.000000000000000000, -0.3807014730195285579, 0.9246979985058696450 ) ) ;
#24870=CYLINDRICAL_SURFACE ( 'NONE', #57530, 12.75000000000000178 ) ;
#24872=CARTESIAN_POINT ( 'NONE',  ( 37.00000000000000711, -0.6593684648219547695, 12.73293890771483561 ) ) ;
#24873=EDGE_CURVE ( 'NONE', #18117, #11339, #42323, .T. ) ;
#24875=ORIENTED_EDGE ( 'NONE', *, *, #15821, .F. ) ;
#24879=DIRECTION ( 'NONE',  ( -1.000000000000000000, 0.000000000000000000, 0.000000000000000000 ) ) ;
#24881=CARTESIAN_POINT ( 'NONE',  ( 10.33819151767390743, 13.43558936918568136, -1.319127422667911276 ) ) ;
#24882=CARTESIAN_POINT ( 'NONE',  ( 24.36133864597850263, -0.004336254571473984777, 13.50457224143761259 ) ) ;
#24883=FACE_OUTER_BOUND ( 'NONE', #19064, .T. ) ;
#24884=CARTESIAN_POINT ( 'NONE',  ( -37.00000000000000711, 11.66664283989680051, 5.143145423404323680 ) ) ;
#24885=CYLINDRICAL_SURFACE ( 'NONE', #6606, 8.049672981451799103 ) ;
#24886=AXIS2_PLACEMENT_3D ( 'NONE', #11589, #6291, #26554 ) ;
#24887=ORIENTED_EDGE ( 'NONE', *, *, #48375, .F. ) ;
#24889=VERTEX_POINT ( 'NONE', #62384 ) ;
#24890=FACE_OUTER_BOUND ( 'NONE', #59611, .T. ) ;
#24892=CIRCLE ( 'NONE', #18556, 4.999999999999999112 ) ;
#24893=CARTESIAN_POINT ( 'NONE',  ( -35.00000000000000000, 0.000000000000000000, 0.000000000000000000 ) ) ;
#24897=CARTESIAN_POINT ( 'NONE',  ( -37.00000000000000711, -10.01317267707891467, 6.946017217729903770 ) ) ;
#24899=CARTESIAN_POINT ( 'NONE',  ( 9.040406806271612083, 3.542740750417936901, 11.46777809083421218 ) ) ;
#24901=EDGE_CURVE ( 'NONE', #5918, #36872, #62505, .T. ) ;
#24902=VECTOR ( 'NONE', #25613, 1000.000000000000000 ) ;
#24903=LINE ( 'NONE', #18632, #49987 ) ;
#24904=ORIENTED_EDGE ( 'NONE', *, *, #19410, .F. ) ;
#24905=CARTESIAN_POINT ( 'NONE',  ( -36.00000000000000711, 2.696588552979058750, 12.46157735505190267 ) ) ;
#24906=ORIENTED_EDGE ( 'NONE', *, *, #11337, .F. ) ;
#24908=DIRECTION ( 'NONE',  ( 0.000000000000000000, 0.01356324068817998940, -0.9999080150203990547 ) ) ;
#24909=AXIS2_PLACEMENT_3D ( 'NONE', #35370, #15734, #60992 ) ;
#24910=EDGE_CURVE ( 'NONE', #7095, #56961, #31075, .T. ) ;
#24911=CARTESIAN_POINT ( 'NONE',  ( 35.00000000000000000, -7.379373053628789592, 10.39746860227898217 ) ) ;
#24915=ORIENTED_EDGE ( 'NONE', *, *, #15976, .T. ) ;
#24916=EDGE_LOOP ( 'NONE', ( #16257, #58074, #24928, #28368 ) ) ;
#24919=ORIENTED_EDGE ( 'NONE', *, *, #48571, .T. ) ;
#24921=DIRECTION ( 'NONE',  ( -1.000000000000000000, 0.000000000000000000, 0.000000000000000000 ) ) ;
#24922=AXIS2_PLACEMENT_3D ( 'NONE', #24647, #58340, #13111 ) ;
#24924=DIRECTION ( 'NONE',  ( -1.000000000000000000, 0.000000000000000000, 0.000000000000000000 ) ) ;
#24926=CARTESIAN_POINT ( 'NONE',  ( -37.00000000000000711, -6.415447294506628317, -11.01837265713080072 ) ) ;
#24928=ORIENTED_EDGE ( 'NONE', *, *, #43068, .F. ) ;
#24929=EDGE_CURVE ( 'NONE', #32830, #65463, #2008, .T. ) ;
#24930=CIRCLE ( 'NONE', #58943, 12.75000000000000178 ) ;
#24932=VERTEX_POINT ( 'NONE', #61739 ) ;
#24933=ORIENTED_EDGE ( 'NONE', *, *, #36645, .F. ) ;
#24934=DIRECTION ( 'NONE',  ( 1.000000000000000000, 0.000000000000000000, -0.000000000000000000 ) ) ;
#24939=CARTESIAN_POINT ( 'NONE',  ( 37.00000000000000711, -7.817492529713787164, 9.348667969174485393 ) ) ;
#24940=FACE_OUTER_BOUND ( 'NONE', #64467, .T. ) ;
#24942=EDGE_CURVE ( 'NONE', #27683, #23780, #41121, .T. ) ;
#24950=VERTEX_POINT ( 'NONE', #57766 ) ;
#24951=EDGE_LOOP ( 'NONE', ( #50885, #26335, #43049, #5753 ) ) ;
#24953=EDGE_CURVE ( 'NONE', #17964, #21760, #48721, .T. ) ;
#24959=EDGE_CURVE ( 'NONE', #6900, #43286, #31488, .T. ) ;
#24961=CARTESIAN_POINT ( 'NONE',  ( -37.00000000000000711, 0.000000000000000000, 0.000000000000000000 ) ) ;
#24962=ORIENTED_EDGE ( 'NONE', *, *, #50277, .F. ) ;
#24963=CARTESIAN_POINT ( 'NONE',  ( -35.00000000000000000, -3.645068577060105230, 11.16627499335654150 ) ) ;
#24964=FACE_OUTER_BOUND ( 'NONE', #24837, .T. ) ;
#24966=AXIS2_PLACEMENT_3D ( 'NONE', #10040, #15352, #14667 ) ;
#24968=CARTESIAN_POINT ( 'NONE',  ( 35.00000000000000000, -10.92721691015452912, 4.309077947445766554 ) ) ;
#24969=DIRECTION ( 'NONE',  ( -1.000000000000000000, 0.000000000000000000, 0.000000000000000000 ) ) ;
#24970=DIRECTION ( 'NONE',  ( -0.000000000000000000, -1.000000000000000000, -0.000000000000000000 ) ) ;
#24972=ORIENTED_EDGE ( 'NONE', *, *, #45655, .F. ) ;
#24975=ORIENTED_EDGE ( 'NONE', *, *, #6642, .T. ) ;
#24978=DIRECTION ( 'NONE',  ( -1.000000000000000000, 0.000000000000000000, -0.000000000000000000 ) ) ;
#24980=CARTESIAN_POINT ( 'NONE',  ( 10.55727017642485954, 11.97188460455015502, -0.8507229460849952130 ) ) ;
#24981=ORIENTED_EDGE ( 'NONE', *, *, #17374, .T. ) ;
#24982=DIRECTION ( 'NONE',  ( 0.000000000000000000, 0.7790879021242528291, -0.6269146997507959451 ) ) ;
#24983=DIRECTION ( 'NONE',  ( -1.000000000000000000, -0.000000000000000000, 0.000000000000000000 ) ) ;
#24985=CARTESIAN_POINT ( 'NONE',  ( -35.00000000000000000, 11.16627499335650242, 3.645068577060221582 ) ) ;
#24986=AXIS2_PLACEMENT_3D ( 'NONE', #35631, #65245, #19713 ) ;
#24987=EDGE_CURVE ( 'NONE', #3409, #16590, #58262, .T. ) ;
#24990=DIRECTION ( 'NONE',  ( -1.000000000000000000, 0.000000000000000000, 0.000000000000000000 ) ) ;
#24993=DIRECTION ( 'NONE',  ( -1.000000000000000000, 0.000000000000000000, 0.000000000000000000 ) ) ;
#24995=CIRCLE ( 'NONE', #37751, 5.000000000000000888 ) ;
#24996=EDGE_LOOP ( 'NONE', ( #58817, #5996, #13797, #25901 ) ) ;
#24999=DIRECTION ( 'NONE',  ( 1.000000000000000000, 0.000000000000000000, 0.000000000000000000 ) ) ;
#25001=DIRECTION ( 'NONE',  ( -1.000000000000000000, -0.000000000000000000, 0.000000000000000000 ) ) ;
#25003=ORIENTED_EDGE ( 'NONE', *, *, #10667, .F. ) ;
#25004=EDGE_CURVE ( 'NONE', #19021, #20284, #15554, .T. ) ;
#25005=ORIENTED_EDGE ( 'NONE', *, *, #18707, .T. ) ;
#25006=ORIENTED_EDGE ( 'NONE', *, *, #11573, .T. ) ;
#25008=EDGE_CURVE ( 'NONE', #65378, #63878, #44468, .T. ) ;
#25011=CARTESIAN_POINT ( 'NONE',  ( 35.00000000000000000, -10.92721691015452912, 4.309077947445766554 ) ) ;
#25012=DIRECTION ( 'NONE',  ( -1.000000000000000000, 0.000000000000000000, 0.000000000000000000 ) ) ;
#25014=ORIENTED_EDGE ( 'NONE', *, *, #5113, .T. ) ;
#25018=DIRECTION ( 'NONE',  ( -1.000000000000000000, 0.000000000000000000, 0.000000000000000000 ) ) ;
#25019=DIRECTION ( 'NONE',  ( 1.000000000000000000, 0.000000000000000000, -0.000000000000000000 ) ) ;
#25022=EDGE_LOOP ( 'NONE', ( #53442, #39992, #59746, #35926 ) ) ;
#25023=DIRECTION ( 'NONE',  ( 0.000000000000000000, -0.01356324068817992175, 0.9999080150203990547 ) ) ;
#25024=ORIENTED_EDGE ( 'NONE', *, *, #31987, .F. ) ;
#25025=CARTESIAN_POINT ( 'NONE',  ( 37.00000000000000711, -10.14433819232439049, -6.753013023069681431 ) ) ;
#25027=EDGE_CURVE ( 'NONE', #36952, #25258, #24312, .T. ) ;
#25028=AXIS2_PLACEMENT_3D ( 'NONE', #37928, #38924, #54219 ) ;
#25029=LINE ( 'NONE', #4425, #2162 ) ;
#25032=CYLINDRICAL_SURFACE ( 'NONE', #56922, 5.000000000000000888 ) ;
#25034=CARTESIAN_POINT ( 'NONE',  ( -37.00000000000000711, -0.01609748574453131326, 11.74614673114904129 ) ) ;
#25035=CARTESIAN_POINT ( 'NONE',  ( -4.590058209962335489, 6.612760447609789871, 25.00000000000000000 ) ) ;
#25038=EDGE_CURVE ( 'NONE', #1795, #27199, #8187, .T. ) ;
#25039=CARTESIAN_POINT ( 'NONE',  ( -35.00000000000000000, 2.021542716731397071, 12.01765980939842748 ) ) ;
#25041=DIRECTION ( 'NONE',  ( 1.000000000000000000, 0.000000000000000000, -0.000000000000000000 ) ) ;
#25042=EDGE_LOOP ( 'NONE', ( #57772, #34685, #42837, #57405 ) ) ;
#25043=EDGE_CURVE ( 'NONE', #173, #38028, #45518, .T. ) ;
#25048=DIRECTION ( 'NONE',  ( 1.000000000000000000, 0.000000000000000000, -0.000000000000000000 ) ) ;
#25051=CARTESIAN_POINT ( 'NONE',  ( 37.00000000000000711, 11.23004253107771255, 4.732539170486137259 ) ) ;
#25055=DIRECTION ( 'NONE',  ( -1.000000000000000000, 0.000000000000000000, 0.000000000000000000 ) ) ;
#25057=ORIENTED_EDGE ( 'NONE', *, *, #52715, .F. ) ;
#25058=CIRCLE ( 'NONE', #33559, 12.18650000000000055 ) ;
#25059=EDGE_CURVE ( 'NONE', #54185, #38600, #21051, .T. ) ;
#25064=DIRECTION ( 'NONE',  ( -1.000000000000000000, 0.000000000000000000, 0.000000000000000000 ) ) ;
#25065=ORIENTED_EDGE ( 'NONE', *, *, #23960, .T. ) ;
#25069=EDGE_CURVE ( 'NONE', #29278, #29745, #40197, .T. ) ;
#25070=CIRCLE ( 'NONE', #10198, 12.18650000000000411 ) ;
#25072=CYLINDRICAL_SURFACE ( 'NONE', #33123, 12.18650000000000055 ) ;
#25073=DIRECTION ( 'NONE',  ( 0.000000000000000000, -0.9105187689795911643, 0.4134677391718608597 ) ) ;
#25074=VERTEX_POINT ( 'NONE', #61616 ) ;
#25077=CYLINDRICAL_SURFACE ( 'NONE', #60474, 17.25474371510545879 ) ;
#25079=CARTESIAN_POINT ( 'NONE',  ( 35.00000000000000000, 5.636262487437473823, 10.80478261802175233 ) ) ;
#25083=ADVANCED_FACE ( 'NONE', ( #17398 ), #41331, .T. ) ;
#25084=EDGE_LOOP ( 'NONE', ( #48755, #23196, #23275, #20215 ) ) ;
#25085=ORIENTED_EDGE ( 'NONE', *, *, #13216, .T. ) ;
#25086=EDGE_CURVE ( 'NONE', #53149, #10035, #63551, .T. ) ;
#25091=DIRECTION ( 'NONE',  ( -1.000000000000000000, 0.000000000000000000, 0.000000000000000000 ) ) ;
#25093=CARTESIAN_POINT ( 'NONE',  ( 35.00000000000000000, 4.705694406421931860E-17, -3.469127814946512892E-15 ) ) ;
#25094=CYLINDRICAL_SURFACE ( 'NONE', #39349, 12.74999999999999822 ) ;
#25096=FACE_OUTER_BOUND ( 'NONE', #61398, .T. ) ;
#25098=CARTESIAN_POINT ( 'NONE',  ( -36.00000000000000711, -11.66664283989676321, -5.143145423404404504 ) ) ;
#25103=EDGE_CURVE ( 'NONE', #2444, #38347, #41671, .T. ) ;
#25104=CARTESIAN_POINT ( 'NONE',  ( 35.00000000000000000, 5.927257550915316919, -10.64792938439757641 ) ) ;
#25106=AXIS2_PLACEMENT_3D ( 'NONE', #3520, #17804, #33426 ) ;
#25108=CARTESIAN_POINT ( 'NONE',  ( -36.00000000000000711, 2.080187960898736588, -12.57916205664479214 ) ) ;
#25109=VERTEX_POINT ( 'NONE', #61964 ) ;
#25111=AXIS2_PLACEMENT_3D ( 'NONE', #12439, #31740, #53364 ) ;
#25112=VERTEX_POINT ( 'NONE', #1461 ) ;
#25116=ORIENTED_EDGE ( 'NONE', *, *, #49877, .T. ) ;
#25117=DIRECTION ( 'NONE',  ( 1.000000000000000000, 0.000000000000000000, -0.000000000000000000 ) ) ;
#25119=DIRECTION ( 'NONE',  ( 0.000000000000000000, -1.000000000000000000, 0.000000000000000000 ) ) ;
#25120=CARTESIAN_POINT ( 'NONE',  ( 17.09299993145517860, 9.325632684014761864, 7.625298650601195050 ) ) ;
#25122=CARTESIAN_POINT ( 'NONE',  ( -10.37734985215438499, -3.972422271833704777, -11.32510580359292618 ) ) ;
#25123=DIRECTION ( 'NONE',  ( 0.3771207168306929813, -0.000000000000000000, 0.9261641133930337277 ) ) ;
#25125=EDGE_LOOP ( 'NONE', ( #23968, #38597, #12629, #60193 ) ) ;
#25127=CARTESIAN_POINT ( 'NONE',  ( -35.00000000000000000, -9.700295462048607931, -7.376655759824990000 ) ) ;
#25128=CARTESIAN_POINT ( 'NONE',  ( -35.00000000000000000, 0.000000000000000000, 0.000000000000000000 ) ) ;
#25131=EDGE_CURVE ( 'NONE', #56567, #44942, #42298, .T. ) ;
#25132=CARTESIAN_POINT ( 'NONE',  ( 35.00000000000000000, 0.4993900848169179896, 12.17626345777662600 ) ) ;
#25133=DIRECTION ( 'NONE',  ( 1.000000000000000000, 0.000000000000000000, -0.000000000000000000 ) ) ;
#25135=ORIENTED_EDGE ( 'NONE', *, *, #22590, .T. ) ;
#25139=EDGE_CURVE ( 'NONE', #16920, #53925, #37333, .T. ) ;
#25140=AXIS2_PLACEMENT_3D ( 'NONE', #56584, #21978, #11344 ) ;
#25142=DIRECTION ( 'NONE',  ( 0.000000000000000000, 0.01356324068817998940, -0.9999080150203990547 ) ) ;
#25143=VERTEX_POINT ( 'NONE', #32342 ) ;
#25144=CARTESIAN_POINT ( 'NONE',  ( 37.00000000000000711, 8.699265615723106748, 8.534258022645994757 ) ) ;
#25145=CARTESIAN_POINT ( 'NONE',  ( 34.00000000000000000, 15.00000000000000000, 1.836970198721028406E-15 ) ) ;
#25147=EDGE_LOOP ( 'NONE', ( #30087, #21206, #1849, #32121 ) ) ;
#25148=DIRECTION ( 'NONE',  ( 0.000000000000000000, 0.01356324068818000328, -0.9999080150203990547 ) ) ;
#25149=DIRECTION ( 'NONE',  ( 0.000000000000000000, 0.01356324068817992175, -0.9999080150203990547 ) ) ;
#25151=ADVANCED_FACE ( 'NONE', ( #7080 ), #57970, .T. ) ;
#25152=DIRECTION ( 'NONE',  ( 0.000000000000000000, 0.01356324068817998940, -0.9999080150203989437 ) ) ;
#25153=ORIENTED_EDGE ( 'NONE', *, *, #53859, .F. ) ;
#25156=ORIENTED_EDGE ( 'NONE', *, *, #30362, .T. ) ;
#25158=CARTESIAN_POINT ( 'NONE',  ( -8.891032880924177206, 12.93614229090409395, -3.860857758255646921 ) ) ;
#25159=CARTESIAN_POINT ( 'NONE',  ( 37.00000000000000711, -2.905556151562703082, -11.38112321385050052 ) ) ;
#25160=CARTESIAN_POINT ( 'NONE',  ( 9.879977921069958313, 7.798719617128603510, -11.02431057014362992 ) ) ;
#25162=CARTESIAN_POINT ( 'NONE',  ( -18.01037762727211700, 3.267117315390755117, 13.10031058145693983 ) ) ;
#25163=DIRECTION ( 'NONE',  ( 1.000000000000000000, -0.000000000000000000, 0.000000000000000000 ) ) ;
#25164=ORIENTED_EDGE ( 'NONE', *, *, #17512, .F. ) ;
#25165=CYLINDRICAL_SURFACE ( 'NONE', #8754, 12.18650000000000055 ) ;
#25166=ORIENTED_EDGE ( 'NONE', *, *, #32170, .T. ) ;
#25168=DIRECTION ( 'NONE',  ( 0.000000000000000000, 0.01356324068817991828, -0.9999080150203990547 ) ) ;
#25169=ORIENTED_EDGE ( 'NONE', *, *, #12852, .F. ) ;
#25170=CARTESIAN_POINT ( 'NONE',  ( -35.00000000000000000, -11.47561260193580779, 5.556331110570367215 ) ) ;
#25171=CARTESIAN_POINT ( 'NONE',  ( -27.27855387000350262, -12.26939275170277632, 5.631341004100471892 ) ) ;
#25172=AXIS2_PLACEMENT_3D ( 'NONE', #29675, #19736, #60606 ) ;
#25173=CYLINDRICAL_SURFACE ( 'NONE', #45638, 5.000000000000000888 ) ;
#25174=EDGE_LOOP ( 'NONE', ( #56687, #6404, #23725, #47792 ) ) ;
#25177=EDGE_CURVE ( 'NONE', #5644, #29486, #51909, .T. ) ;
#25178=ORIENTED_EDGE ( 'NONE', *, *, #10821, .F. ) ;
#25179=CARTESIAN_POINT ( 'NONE',  ( 23.91335571186425923, -9.465411751381743954, -7.380766550276687710 ) ) ;
#25180=CIRCLE ( 'NONE', #16690, 5.000000000000000000 ) ;
#25184=EDGE_CURVE ( 'NONE', #25258, #57134, #50205, .T. ) ;
#25185=CARTESIAN_POINT ( 'NONE',  ( -36.00000000000000711, -10.93004082984014147, -6.564808257521885793 ) ) ;
#25186=DIRECTION ( 'NONE',  ( 1.000000000000000000, 0.000000000000000000, -0.000000000000000000 ) ) ;
#25188=DIRECTION ( 'NONE',  ( 1.000000000000000000, 0.000000000000000000, 0.000000000000000000 ) ) ;
#25189=ORIENTED_EDGE ( 'NONE', *, *, #2612, .F. ) ;
#25191=DIRECTION ( 'NONE',  ( 0.000000000000000000, 0.01356324068817992175, -0.9999080150203990547 ) ) ;
#25193=CARTESIAN_POINT ( 'NONE',  ( 12.51553973845115841, 11.51522108451853121, -7.048732632201635262 ) ) ;
#25194=DIRECTION ( 'NONE',  ( 0.000000000000000000, -0.01356324068817992175, 0.9999080150203990547 ) ) ;
#25195=DIRECTION ( 'NONE',  ( -1.000000000000000000, 0.000000000000000000, 0.000000000000000000 ) ) ;
#25196=CARTESIAN_POINT ( 'NONE',  ( 35.00000000000000000, 3.093009498343925134, -11.78745411414841016 ) ) ;
#25198=EDGE_CURVE ( 'NONE', #60941, #58003, #976, .T. ) ;
#25199=ORIENTED_EDGE ( 'NONE', *, *, #36684, .T. ) ;
#25201=EDGE_CURVE ( 'NONE', #65337, #36759, #45200, .T. ) ;
#25202=ORIENTED_EDGE ( 'NONE', *, *, #19878, .F. ) ;
#25203=CARTESIAN_POINT ( 'NONE',  ( -3.552846699730117574, -9.406274435376895227, 7.462624784235579511 ) ) ;
#25204=DIRECTION ( 'NONE',  ( -1.000000000000000000, 0.000000000000000000, 0.000000000000000000 ) ) ;
#25205=CARTESIAN_POINT ( 'NONE',  ( -17.57509096728301046, 6.782429754866558191, -11.67417802825193895 ) ) ;
#25207=EDGE_CURVE ( 'NONE', #52121, #36243, #35971, .T. ) ;
#25209=EDGE_LOOP ( 'NONE', ( #49391, #51343, #58626, #24772 ) ) ;
#25212=DIRECTION ( 'NONE',  ( -1.000000000000000000, 0.000000000000000000, 0.000000000000000000 ) ) ;
#25214=CIRCLE ( 'NONE', #7216, 12.75000000000000178 ) ;
#25216=CARTESIAN_POINT ( 'NONE',  ( -17.25801985322950216, -6.481189176515793626, 10.10068109367541034 ) ) ;
#25217=LINE ( 'NONE', #57132, #3238 ) ;
#25218=VERTEX_POINT ( 'NONE', #63573 ) ;
#25219=EDGE_CURVE ( 'NONE', #56892, #48293, #54030, .T. ) ;
#25221=EDGE_LOOP ( 'NONE', ( #61299, #56342, #3629, #47542 ) ) ;
#25223=DIRECTION ( 'NONE',  ( 1.000000000000000000, 0.000000000000000000, 0.000000000000000000 ) ) ;
#25224=CIRCLE ( 'NONE', #51781, 12.18650000000000055 ) ;
#25227=ORIENTED_EDGE ( 'NONE', *, *, #2419, .F. ) ;
#25228=AXIS2_PLACEMENT_3D ( 'NONE', #48881, #28914, #49223 ) ;
#25235=LINE ( 'NONE', #61146, #26827 ) ;
#25238=CARTESIAN_POINT ( 'NONE',  ( 35.00000000000000000, -4.986700593229777212, -10.63508530065520219 ) ) ;
#25239=FACE_OUTER_BOUND ( 'NONE', #43389, .T. ) ;
#25240=CARTESIAN_POINT ( 'NONE',  ( -18.56512981111246319, -11.93407345808114073, 1.298380824258862587 ) ) ;
#25241=ORIENTED_EDGE ( 'NONE', *, *, #46475, .F. ) ;
#25244=DIRECTION ( 'NONE',  ( 0.000000000000000000, -0.01356324068817991828, 0.9999080150203990547 ) ) ;
#25246=VERTEX_POINT ( 'NONE', #2443 ) ;
#25248=VERTEX_POINT ( 'NONE', #24926 ) ;
#25249=DIRECTION ( 'NONE',  ( 1.000000000000000000, 0.000000000000000000, 0.000000000000000000 ) ) ;
#25250=CARTESIAN_POINT ( 'NONE',  ( 6.520882551146788941, -4.687253057175320592, -12.66502263360881564 ) ) ;
#25254=ORIENTED_EDGE ( 'NONE', *, *, #34136, .F. ) ;
#25255=FACE_OUTER_BOUND ( 'NONE', #25642, .T. ) ;
#25258=VERTEX_POINT ( 'NONE', #42981 ) ;
#25259=ORIENTED_EDGE ( 'NONE', *, *, #64177, .F. ) ;
#25261=CARTESIAN_POINT ( 'NONE',  ( 36.00000000000000711, -10.68873102412837639, 6.950793414699901085 ) ) ;
#25263=AXIS2_PLACEMENT_3D ( 'NONE', #43084, #5663, #16272 ) ;
#25264=EDGE_CURVE ( 'NONE', #5329, #29772, #10483, .T. ) ;
#25266=DIRECTION ( 'NONE',  ( 1.000000000000000000, 0.000000000000000000, -0.000000000000000000 ) ) ;
#25268=ORIENTED_EDGE ( 'NONE', *, *, #8600, .F. ) ;
#25269=CARTESIAN_POINT ( 'NONE',  ( 35.00000000000000000, -8.534258022646033837, 8.699265615723071221 ) ) ;
#25270=ORIENTED_EDGE ( 'NONE', *, *, #44434, .F. ) ;
#25271=CYLINDRICAL_SURFACE ( 'NONE', #54003, 3.309571291727934295 ) ;
#25272=CARTESIAN_POINT ( 'NONE',  ( 35.00000000000000000, 4.705694406421931860E-17, -3.469127814946512892E-15 ) ) ;
#25273=CIRCLE ( 'NONE', #32698, 12.18649999999999878 ) ;
#25276=DIRECTION ( 'NONE',  ( -0.000000000000000000, -0.000000000000000000, -1.000000000000000000 ) ) ;
#25281=VERTEX_POINT ( 'NONE', #19618 ) ;
#25283=ORIENTED_EDGE ( 'NONE', *, *, #54721, .F. ) ;
#25285=DIRECTION ( 'NONE',  ( -1.000000000000000000, -0.000000000000000000, -0.000000000000000000 ) ) ;
#25286=CARTESIAN_POINT ( 'NONE',  ( -20.79170840334646542, -12.91784323155722269, -3.921648409140116698 ) ) ;
#25287=CARTESIAN_POINT ( 'NONE',  ( -47.00000000000000711, 0.000000000000000000, 0.000000000000000000 ) ) ;
#25292=CARTESIAN_POINT ( 'NONE',  ( -37.00000000000000711, 0.000000000000000000, 0.000000000000000000 ) ) ;
#25293=DIRECTION ( 'NONE',  ( 1.000000000000000000, 0.000000000000000000, -0.000000000000000000 ) ) ;
#25294=DIRECTION ( 'NONE',  ( 0.000000000000000000, -0.01356324068817991828, 0.9999080150203990547 ) ) ;
#25295=DIRECTION ( 'NONE',  ( -1.000000000000000000, -1.836970198721029688E-16, -0.000000000000000000 ) ) ;
#25297=CYLINDRICAL_SURFACE ( 'NONE', #43507, 5.000000000000000888 ) ;
#25298=AXIS2_PLACEMENT_3D ( 'NONE', #53905, #22992, #8033 ) ;
#25300=FACE_OUTER_BOUND ( 'NONE', #34240, .T. ) ;
#25302=CARTESIAN_POINT ( 'NONE',  ( 37.00000000000000711, 4.705694406421931860E-17, -3.469127814946512892E-15 ) ) ;
#25305=EDGE_CURVE ( 'NONE', #38593, #47315, #58289, .T. ) ;
#25306=CIRCLE ( 'NONE', #32731, 12.18649999999999878 ) ;
#25307=ORIENTED_EDGE ( 'NONE', *, *, #27736, .F. ) ;
#25308=EDGE_CURVE ( 'NONE', #41673, #4686, #24589, .T. ) ;
#25311=VERTEX_POINT ( 'NONE', #14583 ) ;
#25314=LINE ( 'NONE', #51596, #18382 ) ;
#25315=EDGE_CURVE ( 'NONE', #51800, #30093, #24355, .T. ) ;
#25316=CIRCLE ( 'NONE', #18972, 5.000000000000000000 ) ;
#25317=LINE ( 'NONE', #45591, #44563 ) ;
#25319=ORIENTED_EDGE ( 'NONE', *, *, #7215, .T. ) ;
#25320=CIRCLE ( 'NONE', #1986, 5.000000000000000888 ) ;
#25323=DIRECTION ( 'NONE',  ( 0.000000000000000000, 0.9551603052523468529, -0.2960891610144545938 ) ) ;
#25325=DIRECTION ( 'NONE',  ( 0.000000000000000000, 0.01356324068817999808, -0.9999080150203990547 ) ) ;
#25328=FACE_OUTER_BOUND ( 'NONE', #14176, .T. ) ;
#25330=CYLINDRICAL_SURFACE ( 'NONE', #34505, 4.999999999999999112 ) ;
#25331=ORIENTED_EDGE ( 'NONE', *, *, #1738, .F. ) ;
#25336=DIRECTION ( 'NONE',  ( 1.000000000000000000, 0.000000000000000000, 0.000000000000000000 ) ) ;
#25337=DIRECTION ( 'NONE',  ( -1.000000000000000000, -1.836970198721029688E-16, -0.000000000000000000 ) ) ;
#25341=EDGE_CURVE ( 'NONE', #57308, #57915, #61518, .T. ) ;
#25342=AXIS2_PLACEMENT_3D ( 'NONE', #47871, #11955, #51887 ) ;
#25343=CARTESIAN_POINT ( 'NONE',  ( 37.00000000000000711, 4.705694406421931860E-17, -3.469127814946512892E-15 ) ) ;
#25346=CARTESIAN_POINT ( 'NONE',  ( 36.00000000000000711, -7.238157050195554554, 10.49626516989278180 ) ) ;
#25347=CARTESIAN_POINT ( 'NONE',  ( 6.412959687766495165, -9.124421398965553820, 9.956605555149330655 ) ) ;
#25348=VERTEX_POINT ( 'NONE', #62134 ) ;
#25351=VECTOR ( 'NONE', #37372, 1000.000000000000000 ) ;
#25353=ORIENTED_EDGE ( 'NONE', *, *, #916, .F. ) ;
#25354=ORIENTED_EDGE ( 'NONE', *, *, #23204, .F. ) ;
#25355=EDGE_CURVE ( 'NONE', #4031, #22247, #8227, .T. ) ;
#25359=CARTESIAN_POINT ( 'NONE',  ( 0.2851083653049504285, -0.4107471485392698018, 13.49374991542258151 ) ) ;
#25361=DIRECTION ( 'NONE',  ( 0.000000000000000000, 0.8169148498130255343, -0.5767582926624997830 ) ) ;
#25362=ADVANCED_FACE ( 'NONE', ( #25239 ), #56842, .T. ) ;
#25363=CARTESIAN_POINT ( 'NONE',  ( 6.361445718264521432, -4.355102044641763648, 25.00000000000000000 ) ) ;
#25366=ORIENTED_EDGE ( 'NONE', *, *, #21915, .T. ) ;
#25368=CARTESIAN_POINT ( 'NONE',  ( 35.00000000000000000, -10.75351884295723970, 4.725891942574862448 ) ) ;
#25371=EDGE_CURVE ( 'NONE', #28701, #38380, #32790, .T. ) ;
#25372=ORIENTED_EDGE ( 'NONE', *, *, #61870, .F. ) ;
#25373=CIRCLE ( 'NONE', #48739, 12.18649999999999878 ) ;
#25375=DIRECTION ( 'NONE',  ( -1.000000000000000000, -0.000000000000000000, 0.000000000000000000 ) ) ;
#25376=CARTESIAN_POINT ( 'NONE',  ( -37.00000000000000711, 0.4993900848167411310, 12.17626345777664021 ) ) ;
#25378=ORIENTED_EDGE ( 'NONE', *, *, #58557, .F. ) ;
#25380=LINE ( 'NONE', #56647, #40996 ) ;
#25381=DIRECTION ( 'NONE',  ( -0.2415534870330798278, 0.000000000000000000, 0.9703875065674330003 ) ) ;
#25382=EDGE_CURVE ( 'NONE', #12285, #50930, #32835, .T. ) ;
#25385=DIRECTION ( 'NONE',  ( -0.000000000000000000, -0.000000000000000000, -1.000000000000000000 ) ) ;
#25387=ORIENTED_EDGE ( 'NONE', *, *, #26109, .T. ) ;
#25388=VECTOR ( 'NONE', #14542, 1000.000000000000000 ) ;
#25389=DIRECTION ( 'NONE',  ( 0.000000000000000000, 0.01356324068817998940, -0.9999080150203990547 ) ) ;
#25390=CARTESIAN_POINT ( 'NONE',  ( 2.320974307000889247, 2.464467181831794917, -11.75030150517671679 ) ) ;
#25391=DIRECTION ( 'NONE',  ( 0.000000000000000000, 0.01356324068817998940, -0.9999080150203990547 ) ) ;
#25392=EDGE_LOOP ( 'NONE', ( #11400, #1722, #15923, #20501 ) ) ;
#25393=EDGE_CURVE ( 'NONE', #15725, #35492, #58351, .T. ) ;
#25395=DIRECTION ( 'NONE',  ( -1.000000000000000000, 0.000000000000000000, -0.000000000000000000 ) ) ;
#25396=EDGE_LOOP ( 'NONE', ( #7301, #18145, #33342, #13948 ) ) ;
#25397=EDGE_LOOP ( 'NONE', ( #22897, #25610 ) ) ;
#25399=AXIS2_PLACEMENT_3D ( 'NONE', #24163, #63408, #28495 ) ;
#25400=AXIS2_PLACEMENT_3D ( 'NONE', #45512, #10589, #10936 ) ;
#25401=EDGE_LOOP ( 'NONE', ( #3515, #29346, #32957, #59190 ) ) ;
#25402=DIRECTION ( 'NONE',  ( 1.000000000000000000, -0.000000000000000000, 0.000000000000000000 ) ) ;
#25403=CARTESIAN_POINT ( 'NONE',  ( 37.00000000000000711, 4.705694406421931860E-17, -3.469127814946512892E-15 ) ) ;
#25405=DIRECTION ( 'NONE',  ( -1.000000000000000000, 0.000000000000000000, -0.000000000000000000 ) ) ;
#25409=CARTESIAN_POINT ( 'NONE',  ( 24.85730486487263491, 0.07226432089349320298, -13.50554067701254546 ) ) ;
#25412=DIRECTION ( 'NONE',  ( 0.000000000000000000, -0.9970832820307047317, -0.07632122047555403577 ) ) ;
#25413=ORIENTED_EDGE ( 'NONE', *, *, #45284, .T. ) ;
#25414=FACE_OUTER_BOUND ( 'NONE', #48898, .T. ) ;
#25415=VERTEX_POINT ( 'NONE', #26547 ) ;
#25417=B_SPLINE_CURVE_WITH_KNOTS ( 'NONE', 3,
 ( #55941, #10701, #61566, #21339, #5408, #20038, #5752, #26018, #30347, #41621 ),
 .UNSPECIFIED., .F., .F.,
 ( 4, 2, 2, 2, 4 ),
 ( 8.673617379884034509E-19, 0.0007817650899998000594, 0.001563530179999599251, 0.002345295269999397251, 0.003127060359999195467 ),
 .UNSPECIFIED. ) ;
#25419=DIRECTION ( 'NONE',  ( -1.000000000000000000, 0.000000000000000000, 0.000000000000000000 ) ) ;
#25421=CARTESIAN_POINT ( 'NONE',  ( 37.00000000000000711, 4.705694406421931860E-17, -3.469127814946512892E-15 ) ) ;
#25423=CYLINDRICAL_SURFACE ( 'NONE', #3705, 12.74999999999999822 ) ;
#25424=CARTESIAN_POINT ( 'NONE',  ( 10.75853767213705225, 7.830989516993144051, 9.092612561015865680 ) ) ;
#25426=ORIENTED_EDGE ( 'NONE', *, *, #64861, .F. ) ;
#25427=ADVANCED_FACE ( 'NONE', ( #61150 ), #15579, .T. ) ;
#25429=DIRECTION ( 'NONE',  ( 1.000000000000000000, 0.000000000000000000, -0.000000000000000000 ) ) ;
#25431=ORIENTED_EDGE ( 'NONE', *, *, #52189, .F. ) ;
#25433=CARTESIAN_POINT ( 'NONE',  ( 35.00000000000000000, -9.430788938293991563, 7.718225330433904574 ) ) ;
#25436=CARTESIAN_POINT ( 'NONE',  ( 17.75904445597924308, 6.994922235104493957, 9.764648471568612820 ) ) ;
#25438=DIRECTION ( 'NONE',  ( -1.000000000000000000, 0.000000000000000000, -0.000000000000000000 ) ) ;
#25439=AXIS2_PLACEMENT_3D ( 'NONE', #55812, #4946, #26517 ) ;
#25441=( BOUNDED_CURVE ( )  B_SPLINE_CURVE ( 3, ( #24814, #14163, #44410, #3580 ),
 .UNSPECIFIED., .F., .F. ) 
 B_SPLINE_CURVE_WITH_KNOTS ( ( 4, 4 ),
 ( 1.875920997006544022, 1.903716271183292008 ),
 .UNSPECIFIED. ) 
 CURVE ( )  GEOMETRIC_REPRESENTATION_ITEM ( )  RATIONAL_B_SPLINE_CURVE ( ( 1.000000000000000000, 0.9999356195973556627, 0.9999356195973556627, 1.000000000000000000 ) ) 
 REPRESENTATION_ITEM ( '' )  );
#25442=AXIS2_PLACEMENT_3D ( 'NONE', #49371, #3817, #24070 ) ;
#25443=VERTEX_POINT ( 'NONE', #57143 ) ;
#25444=CARTESIAN_POINT ( 'NONE',  ( 37.00000000000000711, 4.705694406421931860E-17, -3.469127814946512892E-15 ) ) ;
#25445=EDGE_CURVE ( 'NONE', #36611, #12850, #26533, .T. ) ;
#25446=DIRECTION ( 'NONE',  ( 1.000000000000000000, 0.000000000000000000, 0.000000000000000000 ) ) ;
#25447=DIRECTION ( 'NONE',  ( 0.000000000000000000, -0.3218879778916041157, 0.9467777615094549182 ) ) ;
#25449=CARTESIAN_POINT ( 'NONE',  ( 37.00000000000000711, 11.65150730582934635, 1.488153103997001514 ) ) ;
#25451=AXIS2_PLACEMENT_3D ( 'NONE', #55980, #10415, #45026 ) ;
#25452=DIRECTION ( 'NONE',  ( -1.000000000000000000, -0.000000000000000000, 0.000000000000000000 ) ) ;
#25453=CARTESIAN_POINT ( 'NONE',  ( 1.010855698802849201, 0.1373453909157727193, -12.00331048781906595 ) ) ;
#25455=EDGE_LOOP ( 'NONE', ( #63439, #33608, #23247, #64218 ) ) ;
#25457=CARTESIAN_POINT ( 'NONE',  ( 37.00000000000000711, 1.039216533672905785, -11.70009620280412221 ) ) ;
#25458=DIRECTION ( 'NONE',  ( -1.000000000000000000, -1.836970198721029688E-16, -0.000000000000000000 ) ) ;
#25459=AXIS2_PLACEMENT_3D ( 'NONE', #330, #16919, #61472 ) ;
#25460=ADVANCED_FACE ( 'NONE', ( #5282 ), #21568, .T. ) ;
#25463=DIRECTION ( 'NONE',  ( 0.000000000000000000, 0.01356324068818000848, -0.9999080150203990547 ) ) ;
#25465=CARTESIAN_POINT ( 'NONE',  ( -17.16761170699768968, -6.928568383034877876, -11.59115056719998371 ) ) ;
#25468=VERTEX_POINT ( 'NONE', #31209 ) ;
#25473=EDGE_LOOP ( 'NONE', ( #57760, #949, #56702, #3932 ) ) ;
#25474=DIRECTION ( 'NONE',  ( 0.000000000000000000, -0.9346839223284579834, 0.3554799084908868423 ) ) ;
#25476=EDGE_CURVE ( 'NONE', #8907, #56961, #65341, .T. ) ;
#25478=EDGE_LOOP ( 'NONE', ( #42588, #45964, #34942, #59338 ) ) ;
#25481=CARTESIAN_POINT ( 'NONE',  ( -35.00000000000000000, -12.16632754454237464, 0.7008968033238341944 ) ) ;
#25483=LINE ( 'NONE', #24501, #29060 ) ;
#25484=FACE_OUTER_BOUND ( 'NONE', #49062, .T. ) ;
#25487=DIRECTION ( 'NONE',  ( -1.000000000000000000, 0.000000000000000000, 0.000000000000000000 ) ) ;
#25489=DIRECTION ( 'NONE',  ( -0.000000000000000000, -0.000000000000000000, -1.000000000000000000 ) ) ;
#25490=VECTOR ( 'NONE', #38411, 1000.000000000000000 ) ;
#25492=CARTESIAN_POINT ( 'NONE',  ( -18.25006854224444908, -9.443202773001939221, 9.647586298549914119 ) ) ;
#25494=ORIENTED_EDGE ( 'NONE', *, *, #57021, .T. ) ;
#25496=ADVANCED_FACE ( 'NONE', ( #10575 ), #51515, .T. ) ;
#25497=CARTESIAN_POINT ( 'NONE',  ( 12.57012137786681549, 11.47155630137818072, -3.539951925651088960 ) ) ;
#25498=FACE_BOUND ( 'NONE', #42412, .T. ) ;
#25499=ORIENTED_EDGE ( 'NONE', *, *, #16395, .F. ) ;
#25502=VERTEX_POINT ( 'NONE', #25898 ) ;
#25503=VECTOR ( 'NONE', #59780, 1000.000000000000000 ) ;
#25505=DIRECTION ( 'NONE',  ( -1.000000000000000000, 0.000000000000000000, 0.000000000000000000 ) ) ;
#25509=EDGE_CURVE ( 'NONE', #48505, #42153, #14562, .T. ) ;
#25510=CARTESIAN_POINT ( 'NONE',  ( -36.00000000000000711, -10.23119532541078236, 7.608228585767692564 ) ) ;
#25511=CARTESIAN_POINT ( 'NONE',  ( 37.00000000000000711, -8.029056188533749250, -8.573591947375291511 ) ) ;
#25512=VECTOR ( 'NONE', #39966, 1000.000000000000000 ) ;
#25514=DIRECTION ( 'NONE',  ( 0.000000000000000000, -0.01356324068817998940, 0.9999080150203990547 ) ) ;
#25515=CARTESIAN_POINT ( 'NONE',  ( 35.00000000000000000, -5.672855678558609505, 10.28547182238013669 ) ) ;
#25516=ADVANCED_FACE ( 'NONE', ( #52797 ), #7228, .T. ) ;
#25517=CARTESIAN_POINT ( 'NONE',  ( -35.00000000000000000, 0.000000000000000000, 0.000000000000000000 ) ) ;
#25518=CARTESIAN_POINT ( 'NONE',  ( 11.92883720626436350, 13.27018586330439831, -2.496723423483149684 ) ) ;
#25519=DIRECTION ( 'NONE',  ( -1.000000000000000000, -0.000000000000000000, 0.000000000000000000 ) ) ;
#25521=CARTESIAN_POINT ( 'NONE',  ( -36.00000000000000711, 9.076753354954126607, -8.954052073409506818 ) ) ;
#25522=CARTESIAN_POINT ( 'NONE',  ( 37.00000000000000711, 11.54110654723649176, -2.185196060783925809 ) ) ;
#25523=EDGE_CURVE ( 'NONE', #12164, #42779, #36010, .T. ) ;
#25526=ORIENTED_EDGE ( 'NONE', *, *, #39502, .F. ) ;
#25528=LINE ( 'NONE', #51493, #30135 ) ;
#25529=ORIENTED_EDGE ( 'NONE', *, *, #8175, .T. ) ;
#25530=CARTESIAN_POINT ( 'NONE',  ( -35.00000000000000000, 0.000000000000000000, 0.000000000000000000 ) ) ;
#25531=CYLINDRICAL_SURFACE ( 'NONE', #54267, 5.000000000000000888 ) ;
#25535=ORIENTED_EDGE ( 'NONE', *, *, #32996, .T. ) ;
#25536=DIRECTION ( 'NONE',  ( -0.000000000000000000, -1.000000000000000000, -0.000000000000000000 ) ) ;
#25539=CARTESIAN_POINT ( 'NONE',  ( 24.82652845881425208, 25.00000000000000000, -8.578654028722157321 ) ) ;
#25541=ADVANCED_FACE ( 'NONE', ( #12226 ), #8225, .T. ) ;
#25543=CARTESIAN_POINT ( 'NONE',  ( 8.937200413559441614, 4.646453064669045396, -12.67647346021110266 ) ) ;
#25545=FACE_OUTER_BOUND ( 'NONE', #34503, .T. ) ;
#25546=VERTEX_POINT ( 'NONE', #47809 ) ;
#25553=CIRCLE ( 'NONE', #34042, 12.75000000000000178 ) ;
#25559=ORIENTED_EDGE ( 'NONE', *, *, #18450, .F. ) ;
#25560=AXIS2_PLACEMENT_3D ( 'NONE', #10203, #40805, #65710 ) ;
#25561=DIRECTION ( 'NONE',  ( 1.000000000000000000, 0.000000000000000000, 0.000000000000000000 ) ) ;
#25563=FACE_OUTER_BOUND ( 'NONE', #49934, .T. ) ;
#25567=CARTESIAN_POINT ( 'NONE',  ( -7.382824176484668044, -1.433652869056799339, 11.91442981667273315 ) ) ;
#25570=CARTESIAN_POINT ( 'NONE',  ( -8.580377709536596953, -8.097098178811418023, -8.863927581768100694 ) ) ;
#25575=VECTOR ( 'NONE', #27490, 1000.000000000000000 ) ;
#25576=AXIS2_PLACEMENT_3D ( 'NONE', #65380, #65696, #40439 ) ;
#25577=ORIENTED_EDGE ( 'NONE', *, *, #10709, .T. ) ;
#25580=DIRECTION ( 'NONE',  ( 1.000000000000000000, -0.000000000000000000, 0.000000000000000000 ) ) ;
#25581=EDGE_CURVE ( 'NONE', #47524, #51686, #13717, .T. ) ;
#25582=DIRECTION ( 'NONE',  ( -1.000000000000000000, 0.000000000000000000, 0.000000000000000000 ) ) ;
#25583=AXIS2_PLACEMENT_3D ( 'NONE', #6154, #826, #21440 ) ;
#25584=LINE ( 'NONE', #40887, #57323 ) ;
#25585=LINE ( 'NONE', #27455, #17581 ) ;
#25586=ORIENTED_EDGE ( 'NONE', *, *, #28018, .F. ) ;
#25588=DIRECTION ( 'NONE',  ( 0.000000000000000000, 0.01356324068817998940, -0.9999080150203990547 ) ) ;
#25589=EDGE_CURVE ( 'NONE', #27033, #25959, #41334, .T. ) ;
#25590=ORIENTED_EDGE ( 'NONE', *, *, #13165, .F. ) ;
#25591=DIRECTION ( 'NONE',  ( 0.000000000000000000, 0.5767582926624970074, 0.8169148498130275327 ) ) ;
#25592=ORIENTED_EDGE ( 'NONE', *, *, #65440, .F. ) ;
#25593=ORIENTED_EDGE ( 'NONE', *, *, #62206, .T. ) ;
#25594=ORIENTED_EDGE ( 'NONE', *, *, #42678, .F. ) ;
#25596=CARTESIAN_POINT ( 'NONE',  ( -35.00000000000000000, 0.000000000000000000, 0.000000000000000000 ) ) ;
#25600=DIRECTION ( 'NONE',  ( 0.000000000000000000, 0.7381862504171925465, -0.6745969609292691294 ) ) ;
#25601=EDGE_CURVE ( 'NONE', #58571, #7860, #7358, .T. ) ;
#25602=DIRECTION ( 'NONE',  ( 0.000000000000000000, 0.8369827122275362852, 0.5472293298355244140 ) ) ;
#25603=ORIENTED_EDGE ( 'NONE', *, *, #2915, .T. ) ;
#25605=ORIENTED_EDGE ( 'NONE', *, *, #5447, .F. ) ;
#25606=CARTESIAN_POINT ( 'NONE',  ( 37.00000000000000711, -0.7536123767497623360, 11.72195762423410237 ) ) ;
#25609=ADVANCED_FACE ( 'NONE', ( #27510 ), #7916, .T. ) ;
#25610=ORIENTED_EDGE ( 'NONE', *, *, #51656, .T. ) ;
#25613=DIRECTION ( 'NONE',  ( -1.000000000000000000, 0.000000000000000000, 0.000000000000000000 ) ) ;
#25614=ORIENTED_EDGE ( 'NONE', *, *, #65648, .F. ) ;
#25615=LINE ( 'NONE', #36582, #65113 ) ;
#25616=EDGE_CURVE ( 'NONE', #62364, #59342, #9432, .T. ) ;
#25618=ORIENTED_EDGE ( 'NONE', *, *, #27172, .T. ) ;
#25619=CARTESIAN_POINT ( 'NONE',  ( -24.29873642282455393, -10.29150269569643150, 8.745998899381449476 ) ) ;
#25620=CARTESIAN_POINT ( 'NONE',  ( 35.00000000000000000, -11.23004253107767880, -4.732539170486222524 ) ) ;
#25623=DIRECTION ( 'NONE',  ( 0.000000000000000000, 0.01356324068817998940, -0.9999080150203990547 ) ) ;
#25624=ORIENTED_EDGE ( 'NONE', *, *, #45293, .T. ) ;
#25626=CARTESIAN_POINT ( 'NONE',  ( 35.00000000000000000, -9.908974237959688125, -6.307491713048997362 ) ) ;
#25629=AXIS2_PLACEMENT_3D ( 'NONE', #32322, #31661, #7060 ) ;
#25630=AXIS2_PLACEMENT_3D ( 'NONE', #30128, #50430, #45410 ) ;
#25632=( BOUNDED_CURVE ( )  B_SPLINE_CURVE ( 3, ( #190, #19151, #35419, #49744 ),
 .UNSPECIFIED., .F., .F. ) 
 B_SPLINE_CURVE_WITH_KNOTS ( ( 4, 4 ),
 ( 1.242321100838241765, 1.259206054522467477 ),
 .UNSPECIFIED. ) 
 CURVE ( )  GEOMETRIC_REPRESENTATION_ITEM ( )  RATIONAL_B_SPLINE_CURVE ( ( 1.000000000000000000, 0.9999762416693727118, 0.9999762416693727118, 1.000000000000000000 ) ) 
 REPRESENTATION_ITEM ( '' )  );
#25633=CYLINDRICAL_SURFACE ( 'NONE', #10487, 12.74999999999999822 ) ;
#25635=DIRECTION ( 'NONE',  ( -1.000000000000000000, 0.000000000000000000, -0.000000000000000000 ) ) ;
#25636=DIRECTION ( 'NONE',  ( 0.000000000000000000, 0.01356324068817998940, -0.9999080150203989437 ) ) ;
#25637=VECTOR ( 'NONE', #48016, 1000.000000000000000 ) ;
#25638=ADVANCED_FACE ( 'NONE', ( #63732 ), #18213, .T. ) ;
#25639=AXIS2_PLACEMENT_3D ( 'NONE', #52314, #6753, #27660 ) ;
#25642=EDGE_LOOP ( 'NONE', ( #29364, #47467, #13617, #2020 ) ) ;
#25643=DIRECTION ( 'NONE',  ( -1.000000000000000000, -0.000000000000000000, 0.000000000000000000 ) ) ;
#25646=VECTOR ( 'NONE', #10050, 1000.000000000000000 ) ;
#25647=CARTESIAN_POINT ( 'NONE',  ( -10.90165637462999726, -7.508992741355383416, 25.00000000000000000 ) ) ;
#25651=ORIENTED_EDGE ( 'NONE', *, *, #8928, .T. ) ;
#25652=CARTESIAN_POINT ( 'NONE',  ( -37.00000000000000711, 0.000000000000000000, 0.000000000000000000 ) ) ;
#25653=CARTESIAN_POINT ( 'NONE',  ( 37.00000000000000711, 1.591260454995240714, -12.08216339958901564 ) ) ;
#25654=EDGE_CURVE ( 'NONE', #10868, #7257, #56207, .T. ) ;
#25655=ORIENTED_EDGE ( 'NONE', *, *, #20580, .F. ) ;
#25656=CARTESIAN_POINT ( 'NONE',  ( 37.00000000000000711, -8.258652103341374229, 8.352657516904754331 ) ) ;
#25657=DIRECTION ( 'NONE',  ( 0.000000000000000000, -0.4935949184179135862, 0.8696919319575254770 ) ) ;
#25658=AXIS2_PLACEMENT_3D ( 'NONE', #25596, #51861, #41202 ) ;
#25660=ORIENTED_EDGE ( 'NONE', *, *, #2192, .F. ) ;
#25664=ORIENTED_EDGE ( 'NONE', *, *, #24245, .T. ) ;
#25665=AXIS2_PLACEMENT_3D ( 'NONE', #34327, #3451, #43986 ) ;
#25666=CYLINDRICAL_SURFACE ( 'NONE', #4454, 13.50000000000000178 ) ;
#25667=EDGE_CURVE ( 'NONE', #28861, #48679, #18563, .T. ) ;
#25671=CARTESIAN_POINT ( 'NONE',  ( -35.00000000000000000, -7.882940143791844712, 10.02106554660705839 ) ) ;
#25672=CARTESIAN_POINT ( 'NONE',  ( -37.00000000000000711, 0.000000000000000000, 0.000000000000000000 ) ) ;
#25674=DIRECTION ( 'NONE',  ( 0.000000000000000000, 0.01356324068817992175, -0.9999080150203990547 ) ) ;
#25676=CARTESIAN_POINT ( 'NONE',  ( 35.00000000000000000, -9.557269938331497627, 7.561043153948066475 ) ) ;
#25677=CIRCLE ( 'NONE', #4472, 5.000000000000000888 ) ;
#25678=DIRECTION ( 'NONE',  ( 1.000000000000000000, 0.000000000000000000, 0.000000000000000000 ) ) ;
#25679=EDGE_CURVE ( 'NONE', #50432, #53297, #49140, .T. ) ;
#25681=DIRECTION ( 'NONE',  ( 1.000000000000000000, 0.000000000000000000, 0.000000000000000000 ) ) ;
#25682=DIRECTION ( 'NONE',  ( 1.000000000000000000, 0.000000000000000000, -0.000000000000000000 ) ) ;
#25683=ORIENTED_EDGE ( 'NONE', *, *, #54655, .T. ) ;
#25684=DIRECTION ( 'NONE',  ( -1.000000000000000000, 0.000000000000000000, 0.000000000000000000 ) ) ;
#25685=ORIENTED_EDGE ( 'NONE', *, *, #1755, .F. ) ;
#25686=CARTESIAN_POINT ( 'NONE',  ( 10.12522915465333462, -13.48295319373161760, -0.6855729276752927648 ) ) ;
#25687=ORIENTED_EDGE ( 'NONE', *, *, #61486, .T. ) ;
#25688=ADVANCED_FACE ( 'NONE', ( #28833 ), #14182, .T. ) ;
#25689=DIRECTION ( 'NONE',  ( 1.000000000000000000, 0.000000000000000000, 0.000000000000000000 ) ) ;
#25690=EDGE_LOOP ( 'NONE', ( #44245, #36099, #6436, #12096 ) ) ;
#25691=DIRECTION ( 'NONE',  ( -1.000000000000000000, 0.000000000000000000, 0.000000000000000000 ) ) ;
#25692=DIRECTION ( 'NONE',  ( -1.000000000000000000, 0.000000000000000000, 0.000000000000000000 ) ) ;
#25693=DIRECTION ( 'NONE',  ( -1.000000000000000000, 0.000000000000000000, -0.000000000000000000 ) ) ;
#25696=CIRCLE ( 'NONE', #35211, 5.000000000000000888 ) ;
#25698=EDGE_LOOP ( 'NONE', ( #22650, #14933, #40263, #12062 ) ) ;
#25699=FACE_OUTER_BOUND ( 'NONE', #45103, .T. ) ;
#25700=AXIS2_PLACEMENT_3D ( 'NONE', #16477, #31737, #36745 ) ;
#25701=EDGE_CURVE ( 'NONE', #8767, #4893, #14744, .T. ) ;
#25702=ORIENTED_EDGE ( 'NONE', *, *, #39710, .T. ) ;
#25704=AXIS2_PLACEMENT_3D ( 'NONE', #2725, #8027, #58911 ) ;
#25705=ADVANCED_FACE ( 'NONE', ( #35100 ), #29792, .F. ) ;
#25706=PLANE ( 'NONE',  #10087 ) ;
#25708=ORIENTED_EDGE ( 'NONE', *, *, #33239, .F. ) ;
#25709=AXIS2_PLACEMENT_3D ( 'NONE', #33553, #53843, #23583 ) ;
#25713=DIRECTION ( 'NONE',  ( 0.000000000000000000, 0.01356324068817998940, -0.9999080150203990547 ) ) ;
#25714=DIRECTION ( 'NONE',  ( 0.000000000000000000, -0.01356324068818000328, 0.9999080150203990547 ) ) ;
#25716=CARTESIAN_POINT ( 'NONE',  ( 35.00000000000000000, 5.428340790341703581, -10.91072401419412685 ) ) ;
#25720=EDGE_CURVE ( 'NONE', #45412, #51182, #40098, .T. ) ;
#25723=B_SPLINE_CURVE_WITH_KNOTS ( 'NONE', 3,
 ( #37579, #11965, #17298, #17633, #31908, #57876, #2342, #52868, #37896, #32246, #7298, #43202, #42206, #62495, #63478, #27583 ),
 .UNSPECIFIED., .F., .F.,
 ( 4, 2, 2, 2, 2, 2, 2, 4 ),
 ( 2.485638410533990448E-17, 0.002410354704749657039, 0.003615532057124472981, 0.004820709409499289791, 0.006025886761874103999, 0.007231064114248917339, 0.008436241466623731547, 0.009641418818998544887 ),
 .UNSPECIFIED. ) ;
#25725=CARTESIAN_POINT ( 'NONE',  ( -37.00000000000000711, 0.000000000000000000, 0.000000000000000000 ) ) ;
#25729=CARTESIAN_POINT ( 'NONE',  ( 34.38695973621796043, 25.00000000000000000, 3.530690241644829364 ) ) ;
#25730=ORIENTED_EDGE ( 'NONE', *, *, #59024, .T. ) ;
#25731=CARTESIAN_POINT ( 'NONE',  ( -18.58686583997225839, 5.151216734910813777, 10.83812558286603789 ) ) ;
#25732=CARTESIAN_POINT ( 'NONE',  ( 35.00000000000000000, -11.65150730582935523, -1.488153103996925797 ) ) ;
#25733=EDGE_LOOP ( 'NONE', ( #50760, #24523, #17841, #48545 ) ) ;
#25734=EDGE_CURVE ( 'NONE', #23284, #59054, #30701, .T. ) ;
#25737=CIRCLE ( 'NONE', #62893, 5.000000000000000000 ) ;
#25738=VECTOR ( 'NONE', #9503, 1000.000000000000000 ) ;
#25739=ADVANCED_FACE ( 'NONE', ( #9851 ), #29470, .T. ) ;
#25740=ORIENTED_EDGE ( 'NONE', *, *, #18582, .F. ) ;
#25743=DIRECTION ( 'NONE',  ( 0.000000000000000000, -0.01356324068817998940, 0.9999080150203990547 ) ) ;
#25744=CARTESIAN_POINT ( 'NONE',  ( 9.150528470156286787, 5.807572156255496054, 10.50730673458101450 ) ) ;
#25749=CARTESIAN_POINT ( 'NONE',  ( 24.90067624556555259, -0.3238485137761343835, -13.50202336863869235 ) ) ;
#25750=DIRECTION ( 'NONE',  ( -0.000000000000000000, -1.000000000000000000, -0.000000000000000000 ) ) ;
#25752=CARTESIAN_POINT ( 'NONE',  ( 47.00000000000000711, 4.705694406421931860E-17, -3.469127814946512892E-15 ) ) ;
#25753=EDGE_CURVE ( 'NONE', #19363, #26831, #65047, .T. ) ;
#25756=ORIENTED_EDGE ( 'NONE', *, *, #57044, .F. ) ;
#25757=ORIENTED_EDGE ( 'NONE', *, *, #50128, .F. ) ;
#25760=CARTESIAN_POINT ( 'NONE',  ( -27.45775109278351067, 10.51123867646838583, -8.471355351200609007 ) ) ;
#25761=CARTESIAN_POINT ( 'NONE',  ( 37.00000000000000711, 9.621072037176993774, -8.366449238204399563 ) ) ;
#25763=DIRECTION ( 'NONE',  ( 1.000000000000000000, 0.000000000000000000, 0.000000000000000000 ) ) ;
#25764=ORIENTED_EDGE ( 'NONE', *, *, #33828, .T. ) ;
#25765=AXIS2_PLACEMENT_3D ( 'NONE', #40140, #45465, #30500 ) ;
#25766=ORIENTED_EDGE ( 'NONE', *, *, #24021, .F. ) ;
#25769=EDGE_CURVE ( 'NONE', #7682, #37677, #60431, .T. ) ;
#25771=CIRCLE ( 'NONE', #4561, 5.000000000000000888 ) ;
#25772=ORIENTED_EDGE ( 'NONE', *, *, #61991, .F. ) ;
#25773=CARTESIAN_POINT ( 'NONE',  ( -37.00000000000000711, 3.340853584269533716, 11.26103545359857350 ) ) ;
#25774=CARTESIAN_POINT ( 'NONE',  ( 35.00000000000000000, -11.17622378668003691, 3.614449339633606595 ) ) ;
#25779=VECTOR ( 'NONE', #23851, 1000.000000000000000 ) ;
#25780=DIRECTION ( 'NONE',  ( 0.000000000000000000, 0.4134677391718449835, 0.9105187689795983808 ) ) ;
#25781=AXIS2_PLACEMENT_3D ( 'NONE', #9115, #30049, #29394 ) ;
#25782=ADVANCED_FACE ( 'NONE', ( #56054 ), #6193, .T. ) ;
#25784=ADVANCED_FACE ( 'NONE', ( #15808 ), #60731, .T. ) ;
#25788=CARTESIAN_POINT ( 'NONE',  ( -35.00000000000000000, -9.321877890560388735, -7.146664589318012517 ) ) ;
#25789=CIRCLE ( 'NONE', #31097, 5.000000000000001776 ) ;
#25790=DIRECTION ( 'NONE',  ( 1.000000000000000000, 0.000000000000000000, 0.000000000000000000 ) ) ;
#25791=PLANE ( 'NONE',  #57644 ) ;
#25792=CARTESIAN_POINT ( 'NONE',  ( -36.00000000000000711, 6.564808257521927537, -10.93004082984011482 ) ) ;
#25793=CARTESIAN_POINT ( 'NONE',  ( 0.6605806670570022465, -0.1501238075117865833, -12.00189431062279688 ) ) ;
#25794=CIRCLE ( 'NONE', #36418, 5.000000000000000000 ) ;
#25796=VERTEX_POINT ( 'NONE', #20818 ) ;
#25798=CARTESIAN_POINT ( 'NONE',  ( -37.00000000000000711, 0.000000000000000000, 0.000000000000000000 ) ) ;
#25803=DIRECTION ( 'NONE',  ( 1.000000000000000000, 0.000000000000000000, 0.000000000000000000 ) ) ;
#25804=VERTEX_POINT ( 'NONE', #50755 ) ;
#25805=DIRECTION ( 'NONE',  ( -1.000000000000000000, -0.000000000000000000, 0.000000000000000000 ) ) ;
#25808=ORIENTED_EDGE ( 'NONE', *, *, #51482, .T. ) ;
#25811=CARTESIAN_POINT ( 'NONE',  ( 35.00000000000000000, 0.1414404973753909389, 12.74921544981110344 ) ) ;
#25813=ADVANCED_FACE ( 'NONE', ( #46418 ), #36764, .T. ) ;
#25815=DIRECTION ( 'NONE',  ( -1.000000000000000000, 0.000000000000000000, 0.000000000000000000 ) ) ;
#25821=EDGE_LOOP ( 'NONE', ( #11651, #44880, #33232, #39771 ) ) ;
#25823=( BOUNDED_CURVE ( )  B_SPLINE_CURVE ( 3, ( #43791, #54095, #60068, #14487 ),
 .UNSPECIFIED., .F., .F. ) 
 B_SPLINE_CURVE_WITH_KNOTS ( ( 4, 4 ),
 ( 5.002748361502479924, 5.006749598811624402 ),
 .UNSPECIFIED. ) 
 CURVE ( )  GEOMETRIC_REPRESENTATION_ITEM ( )  RATIONAL_B_SPLINE_CURVE ( ( 1.000000000000000000, 0.9999986658421111674, 0.9999986658421111674, 1.000000000000000000 ) ) 
 REPRESENTATION_ITEM ( '' )  );
#25827=VECTOR ( 'NONE', #35974, 1000.000000000000000 ) ;
#25828=CARTESIAN_POINT ( 'NONE',  ( 37.00000000000000711, -5.814360711498364864, -10.70999494708490829 ) ) ;
#25830=EDGE_CURVE ( 'NONE', #31862, #38335, #37064, .T. ) ;
#25832=CARTESIAN_POINT ( 'NONE',  ( -35.00000000000000000, -8.839356091079983102, -8.389074212634382022 ) ) ;
#25833=VECTOR ( 'NONE', #40847, 1000.000000000000000 ) ;
#25834=ORIENTED_EDGE ( 'NONE', *, *, #7077, .T. ) ;
#25840=DIRECTION ( 'NONE',  ( -1.000000000000000000, 0.000000000000000000, -0.000000000000000000 ) ) ;
#25844=DIRECTION ( 'NONE',  ( 1.000000000000000000, 0.000000000000000000, 0.000000000000000000 ) ) ;
#25846=ORIENTED_EDGE ( 'NONE', *, *, #51205, .F. ) ;
#25848=VERTEX_POINT ( 'NONE', #61061 ) ;
#25849=CARTESIAN_POINT ( 'NONE',  ( 29.10683426066285051, -10.83754748704998505, 8.060616254555327487 ) ) ;
#25851=CARTESIAN_POINT ( 'NONE',  ( 21.97522221603474080, -11.76847154110449623, -2.374955909613984506 ) ) ;
#25852=DIRECTION ( 'NONE',  ( 0.000000000000000000, -0.01356324068817998940, 0.9999080150203990547 ) ) ;
#25854=ADVANCED_FACE ( 'NONE', ( #55748 ), #5206, .T. ) ;
#25855=CARTESIAN_POINT ( 'NONE',  ( -28.80182618048087662, 2.759540267861917862, 11.68534817325614661 ) ) ;
#25856=DIRECTION ( 'NONE',  ( -1.000000000000000000, 0.000000000000000000, 0.000000000000000000 ) ) ;
#25859=ADVANCED_FACE ( 'NONE', ( #61363 ), #30459, .T. ) ;
#25861=ORIENTED_EDGE ( 'NONE', *, *, #57818, .F. ) ;
#25862=CARTESIAN_POINT ( 'NONE',  ( -37.00000000000000711, -7.379373053628941470, 10.39746860227888270 ) ) ;
#25863=ADVANCED_FACE ( 'NONE', ( #61696 ), #16156, .T. ) ;
#25864=DIRECTION ( 'NONE',  ( 0.000000000000000000, 0.01356324068817991828, -0.9999080150203990547 ) ) ;
#25865=CARTESIAN_POINT ( 'NONE',  ( 36.00000000000000711, 3.640372113593552061, -12.21925492305363647 ) ) ;
#25867=CARTESIAN_POINT ( 'NONE',  ( -9.142358947343478093, 11.11112337110911774, -4.548091552537131932 ) ) ;
#25868=DIRECTION ( 'NONE',  ( -1.000000000000000000, 0.000000000000000000, 0.000000000000000000 ) ) ;
#25870=DIRECTION ( 'NONE',  ( -1.000000000000000000, 0.000000000000000000, 0.000000000000000000 ) ) ;
#25872=CIRCLE ( 'NONE', #63016, 12.18650000000000055 ) ;
#25873=ORIENTED_EDGE ( 'NONE', *, *, #4380, .T. ) ;
#25874=DIRECTION ( 'NONE',  ( -1.000000000000000000, -0.000000000000000000, -0.000000000000000000 ) ) ;
#25875=EDGE_CURVE ( 'NONE', #21538, #54100, #37080, .T. ) ;
#25876=ORIENTED_EDGE ( 'NONE', *, *, #1884, .T. ) ;
#25878=DIRECTION ( 'NONE',  ( 1.000000000000000000, 0.000000000000000000, 0.000000000000000000 ) ) ;
#25879=AXIS2_PLACEMENT_3D ( 'NONE', #26510, #61420, #920 ) ;
#25883=AXIS2_PLACEMENT_3D ( 'NONE', #8865, #64063, #3583 ) ;
#25890=EDGE_CURVE ( 'NONE', #60382, #31853, #4241, .T. ) ;
#25892=ORIENTED_EDGE ( 'NONE', *, *, #50552, .T. ) ;
#25893=AXIS2_PLACEMENT_3D ( 'NONE', #23830, #34092, #58411 ) ;
#25894=DIRECTION ( 'NONE',  ( -1.000000000000000000, 0.000000000000000000, -0.000000000000000000 ) ) ;
#25895=EDGE_LOOP ( 'NONE', ( #2923, #23093, #31640, #43105 ) ) ;
#25896=DIRECTION ( 'NONE',  ( -1.000000000000000000, 0.000000000000000000, -0.000000000000000000 ) ) ;
#25898=CARTESIAN_POINT ( 'NONE',  ( -37.00000000000000711, -1.286231064351400555, 12.68495603654571369 ) ) ;
#25899=FACE_OUTER_BOUND ( 'NONE', #57597, .T. ) ;
#25900=AXIS2_PLACEMENT_3D ( 'NONE', #38843, #54472, #63756 ) ;
#25901=ORIENTED_EDGE ( 'NONE', *, *, #51289, .T. ) ;
#25903=CARTESIAN_POINT ( 'NONE',  ( -29.06834935496808470, 3.365517089803128137, 11.52551889874833080 ) ) ;
#25904=EDGE_LOOP ( 'NONE', ( #3190, #8820, #36540, #48666 ) ) ;
#25909=FACE_OUTER_BOUND ( 'NONE', #55848, .T. ) ;
#25911=DIRECTION ( 'NONE',  ( 0.000000000000000000, -0.01356324068817991828, 0.9999080150203990547 ) ) ;
#25912=ORIENTED_EDGE ( 'NONE', *, *, #51716, .F. ) ;
#25913=EDGE_CURVE ( 'NONE', #42570, #10611, #55158, .T. ) ;
#25914=VECTOR ( 'NONE', #30778, 1000.000000000000000 ) ;
#25915=CARTESIAN_POINT ( 'NONE',  ( -9.145100072270180291, -9.360112017720965127, -7.518496054314849353 ) ) ;
#25918=ADVANCED_FACE ( 'NONE', ( #13374 ), #29011, .T. ) ;
#25919=DIRECTION ( 'NONE',  ( 0.000000000000000000, -0.3554799084909035511, -0.9346839223284514331 ) ) ;
#25920=CARTESIAN_POINT ( 'NONE',  ( 19.28625800530496903, 1.699513388191793428, 11.87904264843580471 ) ) ;
#25921=ORIENTED_EDGE ( 'NONE', *, *, #46024, .T. ) ;
#25923=FACE_OUTER_BOUND ( 'NONE', #33568, .T. ) ;
#25924=AXIS2_PLACEMENT_3D ( 'NONE', #45419, #14495, #35098 ) ;
#25926=FACE_OUTER_BOUND ( 'NONE', #10247, .T. ) ;
#25928=VERTEX_POINT ( 'NONE', #13692 ) ;
#25929=AXIS2_PLACEMENT_3D ( 'NONE', #9481, #50081, #44403 ) ;
#25933=DIRECTION ( 'NONE',  ( 0.000000000000000000, 0.6745969609292663538, 0.7381862504171952111 ) ) ;
#25935=AXIS2_PLACEMENT_3D ( 'NONE', #37378, #833, #27087 ) ;
#25940=AXIS2_PLACEMENT_3D ( 'NONE', #48049, #2510, #42357 ) ;
#25944=DIRECTION ( 'NONE',  ( 1.000000000000000000, 0.000000000000000000, 0.000000000000000000 ) ) ;
#25945=ORIENTED_EDGE ( 'NONE', *, *, #32170, .F. ) ;
#25946=CARTESIAN_POINT ( 'NONE',  ( 35.00000000000000000, -9.926225166346981155, 6.280308599560240346 ) ) ;
#25947=ORIENTED_EDGE ( 'NONE', *, *, #5335, .F. ) ;
#25948=DIRECTION ( 'NONE',  ( -1.000000000000000000, 0.000000000000000000, 0.000000000000000000 ) ) ;
#25950=CARTESIAN_POINT ( 'NONE',  ( -3.476444485811618801, 10.54985286295970504, 8.431306331566823076 ) ) ;
#25952=CARTESIAN_POINT ( 'NONE',  ( -37.00000000000000711, -11.65150730582933392, -1.488153103997089888 ) ) ;
#25953=B_SPLINE_CURVE_WITH_KNOTS ( 'NONE', 3,
 ( #59488, #60140, #29867, #19592, #9572, #29235, #28904, #50177, #4637, #49214, #39192, #13592, #59822, #65438, #24899, #19902, #40165, #13914 ),
 .UNSPECIFIED., .F., .F.,
 ( 4, 2, 2, 2, 2, 2, 2, 2, 4 ),
 ( 1.788112030672749005E-18, 0.0007433925613402978666, 0.001486785122680593998, 0.002230177684020890130, 0.002973570245361186262, 0.003716962806701481527, 0.004460355368041777659, 0.005203747929382072056, 0.005947140490722368188 ),
 .UNSPECIFIED. ) ;
#25956=CARTESIAN_POINT ( 'NONE',  ( 145.1370849898475797, 3.309064568108273190E-14, 0.000000000000000000 ) ) ;
#25959=VERTEX_POINT ( 'NONE', #59270 ) ;
#25960=DIRECTION ( 'NONE',  ( -1.000000000000000000, -0.000000000000000000, 0.000000000000000000 ) ) ;
#25964=CARTESIAN_POINT ( 'NONE',  ( 10.86013604962553991, -13.40624585479074327, -1.591185651104887411 ) ) ;
#25965=CARTESIAN_POINT ( 'NONE',  ( -35.00000000000000000, -8.854740511458796703, -7.717887834988336415 ) ) ;
#25967=VERTEX_POINT ( 'NONE', #28345 ) ;
#25968=AXIS2_PLACEMENT_3D ( 'NONE', #40700, #10426, #51013 ) ;
#25969=AXIS2_PLACEMENT_3D ( 'NONE', #9188, #65371, #29466 ) ;
#25970=DIRECTION ( 'NONE',  ( 1.000000000000000000, 0.000000000000000000, 0.000000000000000000 ) ) ;
#25971=FACE_OUTER_BOUND ( 'NONE', #7109, .T. ) ;
#25972=CARTESIAN_POINT ( 'NONE',  ( 22.83374636504741773, 9.761338926624789636, -6.987695329749072037 ) ) ;
#25973=CYLINDRICAL_SURFACE ( 'NONE', #21029, 12.75000000000000178 ) ;
#25974=EDGE_CURVE ( 'NONE', #10303, #42026, #57893, .T. ) ;
#25975=FACE_OUTER_BOUND ( 'NONE', #55543, .T. ) ;
#25977=DIRECTION ( 'NONE',  ( 0.000000000000000000, -0.01356324068817991828, 0.9999080150203990547 ) ) ;
#25978=EDGE_CURVE ( 'NONE', #32947, #42367, #46408, .T. ) ;
#25980=CARTESIAN_POINT ( 'NONE',  ( -35.00000000000000000, 10.28547182238008162, 5.672855678558722303 ) ) ;
#25982=EDGE_CURVE ( 'NONE', #56883, #62291, #38159, .T. ) ;
#25983=VERTEX_POINT ( 'NONE', #62668 ) ;
#25984=EDGE_LOOP ( 'NONE', ( #39881, #3857, #14914, #29747 ) ) ;
#25985=FACE_OUTER_BOUND ( 'NONE', #46201, .T. ) ;
#25987=DIRECTION ( 'NONE',  ( 1.000000000000000000, 0.000000000000000000, 0.000000000000000000 ) ) ;
#25988=FACE_OUTER_BOUND ( 'NONE', #29976, .T. ) ;
#25992=VERTEX_POINT ( 'NONE', #53637 ) ;
#25995=VECTOR ( 'NONE', #2495, 1000.000000000000000 ) ;
#25996=DIRECTION ( 'NONE',  ( 0.000000000000000000, -0.3554799084909036067, -0.9346839223284515441 ) ) ;
#26003=CARTESIAN_POINT ( 'NONE',  ( -37.00000000000000711, -12.68495603654570836, -1.286231064351444742 ) ) ;
#26004=ORIENTED_EDGE ( 'NONE', *, *, #44218, .F. ) ;
#26008=EDGE_LOOP ( 'NONE', ( #48570, #50931, #3205, #51706, #48330, #17429, #4065, #49625, #41861, #33137, #41287, #9084, #56667, #25526, #54387, #47115, #16661, #30618, #16906, #23628, #57780, #39034, #6760, #2475, #46310, #46136, #62298, #6308, #4441, #18335, #53532, #65397, #31712, #18814, #64076, #15158, #27089, #6243, #60907, #23937, #24727, #4673, #32067, #54325, #13693, #34057, #2958, #8255, #47149, #39498, #1085, #51368, #40960, #44295, #23155, #48973, #39931, #59758, #47156, #62195, #54555, #41100, #64267, #2856, #57613, #17885, #57912, #7183, #9588, #29828, #19457, #2195, #63964, #47003, #28600, #28410, #60773, #8483, #45079, #32377, #31695, #30090, #21924, #55890, #47026, #29242, #27295, #47332, #2034, #61438, #63011, #5731, #64265, #65584, #16157, #44669, #65219, #50526, #53086, #21636, #9082, #36770, #61314, #895, #49528, #8966, #11886, #33948, #41876, #46355, #57712, #48822, #49644, #25772, #34311, #7308, #34596, #48506, #49426, #10953, #52065, #22780, #34756, #31189, #50968, #15313, #21598, #51115, #65195, #19773, #12255, #17696, #25202, #37800, #37526, #60840, #31407, #7310, #41550, #43510, #22147, #24411, #20525, #14293, #55603, #18164, #32340, #35674, #56805, #39446, #15650, #59924, #45852, #53580, #61965, #5866, #41998, #33371, #25740, #34400, #9052, #50860, #60420, #38842, #57269, #2596, #51827, #64502, #48277, #52856, #14576, #16110, #3724, #44447, #59431, #11227, #40424, #26212, #18829, #15584, #51311, #56865, #40376, #59361, #42905, #1734, #34390, #1967, #62222, #43556, #19399, #51306, #38615, #15797, #41847, #41354, #25846, #10416, #22621, #27603, #55204, #22068, #6772, #55150, #59229, #23043, #41982, #62703, #11049, #56173, #56576, #18503, #9995, #53436, #17196, #22750, #17003, #31466, #47822, #35286, #9624, #43122, #64804, #46324, #31246, #3376, #54212, #14198, #13489, #41528, #12475, #19427, #27682, #59232, #59537, #15448, #42372, #49353, #24425, #20436, #61076, #37349, #11235, #26486, #35010, #61203, #30535, #20945, #60897, #4439, #36720, #6091, #44063, #54563, #55182, #51135, #51025, #49954, #47306, #3343, #57296, #49096, #20563, #36691, #58185, #11670, #53519, #26446, #50024, #9523, #37958, #50309, #29376, #10049, #9368, #19402, #28501, #36837, #38993, #53946, #37191, #33467, #39869, #61582, #34844, #47338, #29176, #43835, #56925, #26460, #25178, #11216, #8613, #21680, #30333, #33437, #57908, #363, #15971, #22009, #44056, #29223, #44252, #30162, #30920, #23786, #26634, #43296, #25378, #59530, #36818, #42475, #40549, #59370, #1954, #8393, #5915, #42490, #30832, #51355, #49203, #31499, #3578, #5499, #50329, #40155, #15476, #8538, #58291, #38586, #3013, #56854, #8908, #29121, #17883, #6977, #6686, #56583, #1960, #63650, #64052, #26875, #50870, #43941, #8735, #51829, #16783, #30799, #49358, #23047, #6875, #40008, #34166, #29635, #30697, #9619, #57519, #27826, #6310, #63424, #62060, #64011, #65002, #65154, #47327, #39418, #673, #5760, #18680, #12017, #10945, #11822, #33692, #27845, #32940, #20903, #32626, #59407, #64824, #1, #37178, #31037, #45708, #62039, #8957, #45775, #57408, #44545, #33256, #7319, #15346, #7509, #13256, #61132, #4667, #8143, #23808, #25372, #20672, #55209, #12781, #156, #1811, #59630, #59852 ) ) ;
#26009=EDGE_LOOP ( 'NONE', ( #63350, #41635, #28795, #18896 ) ) ;
#26010=CARTESIAN_POINT ( 'NONE',  ( 10.13605210956113822, -11.98069853244876803, -0.6880458654474965741 ) ) ;
#26012=DIRECTION ( 'NONE',  ( -1.000000000000000000, -1.836970198721029688E-16, 0.000000000000000000 ) ) ;
#26015=CARTESIAN_POINT ( 'NONE',  ( 9.215727626607732148, 1.931385612058147849, 11.84600384405800000 ) ) ;
#26017=CARTESIAN_POINT ( 'NONE',  ( 8.437200413559441614, 4.673024714880076758, -11.05476227139408252 ) ) ;
#26018=CARTESIAN_POINT ( 'NONE',  ( -18.56056789867630030, 4.666091029268902624, -12.67058235225230511 ) ) ;
#26019=VERTEX_POINT ( 'NONE', #9348 ) ;
#26022=VERTEX_POINT ( 'NONE', #39628 ) ;
#26023=CARTESIAN_POINT ( 'NONE',  ( -35.00000000000000000, 11.39945968423479883, -5.710938531231587234 ) ) ;
#26024=CYLINDRICAL_SURFACE ( 'NONE', #53527, 12.18650000000000055 ) ;
#26025=CIRCLE ( 'NONE', #55733, 5.000000000000000888 ) ;
#26027=ORIENTED_EDGE ( 'NONE', *, *, #15444, .T. ) ;
#26028=DIRECTION ( 'NONE',  ( -1.000000000000000000, 0.000000000000000000, 0.000000000000000000 ) ) ;
#26029=CARTESIAN_POINT ( 'NONE',  ( -35.00000000000000000, -11.23004253107761130, -4.732539170486383284 ) ) ;
#26030=CYLINDRICAL_SURFACE ( 'NONE', #15310, 12.75000000000000178 ) ;
#26034=EDGE_LOOP ( 'NONE', ( #48639, #60190, #52149, #2973 ) ) ;
#26035=CARTESIAN_POINT ( 'NONE',  ( -17.82060864339548090, -5.188839051198853802, -10.82117449455721570 ) ) ;
#26039=CYLINDRICAL_SURFACE ( 'NONE', #26043, 4.999999999999999112 ) ;
#26043=AXIS2_PLACEMENT_3D ( 'NONE', #25368, #19417, #20058 ) ;
#26044=EDGE_CURVE ( 'NONE', #15993, #64802, #54920, .T. ) ;
#26045=EDGE_CURVE ( 'NONE', #17119, #37122, #55248, .T. ) ;
#26049=CYLINDRICAL_SURFACE ( 'NONE', #45872, 12.75000000000000178 ) ;
#26056=EDGE_CURVE ( 'NONE', #56916, #53395, #32888, .T. ) ;
#26058=CARTESIAN_POINT ( 'NONE',  ( -15.45667515140707415, 7.965149195100730495, 10.89992138575203029 ) ) ;
#26059=CARTESIAN_POINT ( 'NONE',  ( 17.77583356546081106, -10.71851000382461017, 8.238550139072438938 ) ) ;
#26060=ORIENTED_EDGE ( 'NONE', *, *, #50558, .T. ) ;
#26062=EDGE_CURVE ( 'NONE', #59647, #62046, #22268, .T. ) ;
#26064=DIRECTION ( 'NONE',  ( 1.000000000000000000, 0.000000000000000000, -0.000000000000000000 ) ) ;
#26065=ORIENTED_EDGE ( 'NONE', *, *, #21027, .F. ) ;
#26067=DIRECTION ( 'NONE',  ( 0.000000000000000000, 0.01356324068817991828, -0.9999080150203990547 ) ) ;
#26068=ORIENTED_EDGE ( 'NONE', *, *, #16143, .F. ) ;
#26069=ORIENTED_EDGE ( 'NONE', *, *, #33920, .F. ) ;
#26071=CIRCLE ( 'NONE', #22898, 5.000000000000001776 ) ;
#26072=FACE_OUTER_BOUND ( 'NONE', #63336, .T. ) ;
#26073=ORIENTED_EDGE ( 'NONE', *, *, #45712, .T. ) ;
#26083=CARTESIAN_POINT ( 'NONE',  ( 35.00000000000000000, 4.705694406421931860E-17, -3.469127814946512892E-15 ) ) ;
#26084=ORIENTED_EDGE ( 'NONE', *, *, #37561, .T. ) ;
#26085=FACE_OUTER_BOUND ( 'NONE', #55753, .T. ) ;
#26086=ORIENTED_EDGE ( 'NONE', *, *, #50509, .F. ) ;
#26087=DIRECTION ( 'NONE',  ( -1.000000000000000000, 0.000000000000000000, 0.000000000000000000 ) ) ;
#26089=ORIENTED_EDGE ( 'NONE', *, *, #22016, .F. ) ;
#26093=VECTOR ( 'NONE', #50170, 1000.000000000000000 ) ;
#26094=EDGE_LOOP ( 'NONE', ( #54251, #12026, #26027, #24468 ) ) ;
#26095=DIRECTION ( 'NONE',  ( 0.000000000000000000, -0.01356324068817992175, 0.9999080150203990547 ) ) ;
#26096=DIRECTION ( 'NONE',  ( 0.000000000000000000, -0.01356324068818000328, 0.9999080150203990547 ) ) ;
#26097=DIRECTION ( 'NONE',  ( 0.000000000000000000, -0.1118654143051685257, -0.9937233664769753450 ) ) ;
#26105=CARTESIAN_POINT ( 'NONE',  ( 37.00000000000000711, 4.705694406421931860E-17, -3.469127814946512892E-15 ) ) ;
#26107=CARTESIAN_POINT ( 'NONE',  ( 18.77703285501462815, 0.5575356882853835794, 11.99009668352191760 ) ) ;
#26109=EDGE_CURVE ( 'NONE', #37925, #29278, #25317, .T. ) ;
#26110=CARTESIAN_POINT ( 'NONE',  ( -10.25776720149870336, -3.790424196025902859, -11.38713284139628712 ) ) ;
#26111=DIRECTION ( 'NONE',  ( 0.000000000000000000, 0.01356324068817998940, -0.9999080150203990547 ) ) ;
#26113=ORIENTED_EDGE ( 'NONE', *, *, #29562, .F. ) ;
#26114=DIRECTION ( 'NONE',  ( 0.000000000000000000, -0.01356324068817998940, 0.9999080150203990547 ) ) ;
#26115=CIRCLE ( 'NONE', #22953, 12.75000000000000178 ) ;
#26116=CARTESIAN_POINT ( 'NONE',  ( 37.00000000000000711, 7.110831038798420600, 9.896810808925309288 ) ) ;
#26117=EDGE_CURVE ( 'NONE', #54418, #10113, #32264, .T. ) ;
#26118=CARTESIAN_POINT ( 'NONE',  ( -35.00000000000000000, -5.428340790341781741, 10.91072401419408777 ) ) ;
#26119=DIRECTION ( 'NONE',  ( 0.000000000000000000, 0.01356324068817992175, -0.9999080150203990547 ) ) ;
#26120=ADVANCED_FACE ( 'NONE', ( #52580 ), #37250, .T. ) ;
#26122=DIRECTION ( 'NONE',  ( -0.9029087107030919768, 0.4298323628305345534, 0.000000000000000000 ) ) ;
#26123=EDGE_CURVE ( 'NONE', #50717, #42378, #5284, .T. ) ;
#26125=LINE ( 'NONE', #56734, #6979 ) ;
#26129=CARTESIAN_POINT ( 'NONE',  ( 10.28941146347812108, 1.468011129749627663, -13.42080671719455509 ) ) ;
#26130=CARTESIAN_POINT ( 'NONE',  ( 37.00000000000000711, -4.561791185930327508, 11.90598845858538013 ) ) ;
#26131=VERTEX_POINT ( 'NONE', #51266 ) ;
#26132=CARTESIAN_POINT ( 'NONE',  ( -17.69283485052123694, -9.508998116294153036, -9.587601754173576296 ) ) ;
#26133=CARTESIAN_POINT ( 'NONE',  ( -27.69376440589343247, -12.79244479394529144, -4.322498630235340755 ) ) ;
#26134=ADVANCED_FACE ( 'NONE', ( #11981 ), #31604, .T. ) ;
#26136=EDGE_LOOP ( 'NONE', ( #40226, #32352, #52699, #65366 ) ) ;
#26137=CARTESIAN_POINT ( 'NONE',  ( -9.197602943758385052, -12.97439165539571526, -3.730917860933688157 ) ) ;
#26139=B_SPLINE_CURVE_WITH_KNOTS ( 'NONE', 3,
 ( #9233, #28878, #39500, #50153, #24210, #39170, #44171, #13568, #58850, #19568, #59463, #49509, #13888, #38863, #48849, #3949, #8271, #3647, #44476, #29514, #23912, #64754 ),
 .UNSPECIFIED., .F., .F.,
 ( 4, 2, 2, 2, 2, 2, 2, 2, 2, 2, 4 ),
 ( 0.002692368623994594382, 0.003420944312408854843, 0.004149520000823115305, 0.004878095689237376201, 0.005606671377651636229, 0.005970959221858770580, 0.006335247066065904931, 0.006699534910273039282, 0.007063822754480173632, 0.007792398442894443202, 0.008520974131308712771 ),
 .UNSPECIFIED. ) ;
#26140=DIRECTION ( 'NONE',  ( -1.000000000000000000, 0.000000000000000000, -0.000000000000000000 ) ) ;
#26141=ADVANCED_FACE ( 'NONE', ( #42220 ), #36924, .T. ) ;
#26144=DIRECTION ( 'NONE',  ( -1.000000000000000000, 0.000000000000000000, 0.000000000000000000 ) ) ;
#26146=AXIS2_PLACEMENT_3D ( 'NONE', #22069, #52680, #1492 ) ;
#26147=DIRECTION ( 'NONE',  ( -1.000000000000000000, 0.000000000000000000, 0.000000000000000000 ) ) ;
#26148=ORIENTED_EDGE ( 'NONE', *, *, #30507, .T. ) ;
#26151=CARTESIAN_POINT ( 'NONE',  ( -37.00000000000000711, -11.42599468261432527, 4.237620530777758354 ) ) ;
#26152=DIRECTION ( 'NONE',  ( 1.000000000000000000, 0.000000000000000000, 0.000000000000000000 ) ) ;
#26153=AXIS2_PLACEMENT_3D ( 'NONE', #37658, #27339, #16710 ) ;
#26155=CARTESIAN_POINT ( 'NONE',  ( -9.391855009251028008, 8.630551682975259098, -8.347810229187485831 ) ) ;
#26160=ORIENTED_EDGE ( 'NONE', *, *, #11098, .F. ) ;
#26164=DIRECTION ( 'NONE',  ( 1.000000000000000000, 0.000000000000000000, 0.000000000000000000 ) ) ;
#26166=DIRECTION ( 'NONE',  ( 1.000000000000000000, 0.000000000000000000, 0.000000000000000000 ) ) ;
#26168=FACE_OUTER_BOUND ( 'NONE', #27551, .T. ) ;
#26169=CARTESIAN_POINT ( 'NONE',  ( -24.55259447788195359, -9.550149982066713505, 7.269203354856432320 ) ) ;
#26170=DIRECTION ( 'NONE',  ( 0.000000000000000000, -0.4698238015817428059, -0.8827602140260282226 ) ) ;
#26171=EDGE_LOOP ( 'NONE', ( #24208, #46932, #65492, #53054 ) ) ;
#26173=LINE ( 'NONE', #46444, #53437 ) ;
#26175=DIRECTION ( 'NONE',  ( 0.000000000000000000, -0.01356324068817998940, 0.9999080150203990547 ) ) ;
#26179=EDGE_CURVE ( 'NONE', #325, #17303, #56571, .T. ) ;
#26182=CARTESIAN_POINT ( 'NONE',  ( 3.459614771489464946, -11.09853614738469396, -7.685863346768205595 ) ) ;
#26183=ORIENTED_EDGE ( 'NONE', *, *, #17590, .F. ) ;
#26184=DIRECTION ( 'NONE',  ( 0.000000000000000000, -0.8169148498130212044, 0.5767582926625060002 ) ) ;
#26187=DIRECTION ( 'NONE',  ( 0.000000000000000000, 0.01356324068817992175, -0.9999080150203990547 ) ) ;
#26188=LINE ( 'NONE', #45467, #14819 ) ;
#26190=FACE_OUTER_BOUND ( 'NONE', #1756, .T. ) ;
#26191=ADVANCED_FACE ( 'NONE', ( #25988 ), #26964, .T. ) ;
#26193=CARTESIAN_POINT ( 'NONE',  ( 36.00000000000000711, 12.16893194857555116, 3.805206332242343947 ) ) ;
#26194=ORIENTED_EDGE ( 'NONE', *, *, #27308, .T. ) ;
#26195=VERTEX_POINT ( 'NONE', #21308 ) ;
#26196=DIRECTION ( 'NONE',  ( 1.000000000000000000, 0.000000000000000000, -0.000000000000000000 ) ) ;
#26197=AXIS2_PLACEMENT_3D ( 'NONE', #25403, #30394, #35025 ) ;
#26198=ORIENTED_EDGE ( 'NONE', *, *, #63275, .T. ) ;
#26200=CARTESIAN_POINT ( 'NONE',  ( -15.46066504888353954, 7.965027411696084414, -10.90001387300706526 ) ) ;
#26202=CARTESIAN_POINT ( 'NONE',  ( 35.00000000000000000, 4.705694406421931860E-17, -3.469127814946512892E-15 ) ) ;
#26203=EDGE_CURVE ( 'NONE', #61612, #28181, #61877, .T. ) ;
#26205=DIRECTION ( 'NONE',  ( 0.000000000000000000, 0.01356324068817998940, -0.9999080150203990547 ) ) ;
#26206=DIRECTION ( 'NONE',  ( 1.000000000000000000, 0.000000000000000000, 0.000000000000000000 ) ) ;
#26208=CARTESIAN_POINT ( 'NONE',  ( 37.00000000000000711, 11.56998259273182583, 3.827046518384956020 ) ) ;
#26212=ORIENTED_EDGE ( 'NONE', *, *, #29363, .F. ) ;
#26213=CYLINDRICAL_SURFACE ( 'NONE', #53028, 12.74999999999999822 ) ;
#26214=VERTEX_POINT ( 'NONE', #46920 ) ;
#26215=DIRECTION ( 'NONE',  ( -1.000000000000000000, 0.000000000000000000, 0.000000000000000000 ) ) ;
#26219=CARTESIAN_POINT ( 'NONE',  ( -7.000263073075360332, -1.818388804573970452, 11.86162824919947312 ) ) ;
#26221=ORIENTED_EDGE ( 'NONE', *, *, #15529, .T. ) ;
#26222=ORIENTED_EDGE ( 'NONE', *, *, #52709, .F. ) ;
#26223=CARTESIAN_POINT ( 'NONE',  ( -35.00000000000000000, -7.817492529713920391, 9.348667969174380588 ) ) ;
#26225=ORIENTED_EDGE ( 'NONE', *, *, #54203, .F. ) ;
#26226=DIRECTION ( 'NONE',  ( -1.000000000000000000, 0.000000000000000000, 0.000000000000000000 ) ) ;
#26227=CARTESIAN_POINT ( 'NONE',  ( 3.489700430103022555, 6.891615640558352851, -11.63886720449249346 ) ) ;
#26228=FACE_OUTER_BOUND ( 'NONE', #41580, .T. ) ;
#26229=CARTESIAN_POINT ( 'NONE',  ( 3.459614771489464946, -11.09853614738469396, 25.00000000000000000 ) ) ;
#26230=CARTESIAN_POINT ( 'NONE',  ( 22.88594695219327235, 3.421158645304719137, 11.50198563395281148 ) ) ;
#26232=CARTESIAN_POINT ( 'NONE',  ( 37.00000000000000711, -10.75351884295723970, 4.725891942574862448 ) ) ;
#26233=CARTESIAN_POINT ( 'NONE',  ( -10.69899791063849648, -4.515810463815420839, 11.12485491063779897 ) ) ;
#26236=VERTEX_POINT ( 'NONE', #7666 ) ;
#26237=AXIS2_PLACEMENT_3D ( 'NONE', #20623, #61178, #40898 ) ;
#26238=CARTESIAN_POINT ( 'NONE',  ( -36.00000000000000711, 11.59605747147786836, 5.300372733891682842 ) ) ;
#26239=CARTESIAN_POINT ( 'NONE',  ( -35.00000000000000000, 10.75351884295727700, -4.725891942574793170 ) ) ;
#26240=EDGE_LOOP ( 'NONE', ( #64200, #47777, #18383, #16369 ) ) ;
#26241=AXIS2_PLACEMENT_3D ( 'NONE', #2716, #63506, #12985 ) ;
#26245=LINE ( 'NONE', #35556, #61968 ) ;
#26249=ORIENTED_EDGE ( 'NONE', *, *, #7922, .T. ) ;
#26250=CARTESIAN_POINT ( 'NONE',  ( 2.284736133211987319, 2.405285213157656976, 13.28910238183927639 ) ) ;
#26252=FACE_OUTER_BOUND ( 'NONE', #57063, .T. ) ;
#26253=ORIENTED_EDGE ( 'NONE', *, *, #22003, .T. ) ;
#26254=VERTEX_POINT ( 'NONE', #23953 ) ;
#26255=ORIENTED_EDGE ( 'NONE', *, *, #24289, .T. ) ;
#26261=DIRECTION ( 'NONE',  ( -1.000000000000000000, -0.000000000000000000, 0.000000000000000000 ) ) ;
#26262=ORIENTED_EDGE ( 'NONE', *, *, #32541, .T. ) ;
#26266=FACE_OUTER_BOUND ( 'NONE', #4418, .T. ) ;
#26269=DIRECTION ( 'NONE',  ( -0.000000000000000000, -1.000000000000000000, -0.000000000000000000 ) ) ;
#26271=CARTESIAN_POINT ( 'NONE',  ( -35.00000000000000000, 12.26766708251996540, -3.473736367725128726 ) ) ;
#26275=CARTESIAN_POINT ( 'NONE',  ( -35.00000000000000000, -10.63508530065525370, 4.986700593229667078 ) ) ;
#26278=LINE ( 'NONE', #25620, #38289 ) ;
#26280=CYLINDRICAL_SURFACE ( 'NONE', #27729, 5.000000000000000888 ) ;
#26282=EDGE_CURVE ( 'NONE', #36705, #44008, #58549, .T. ) ;
#26283=EDGE_CURVE ( 'NONE', #55188, #13695, #53081, .T. ) ;
#26285=DIRECTION ( 'NONE',  ( -1.000000000000000000, 0.000000000000000000, 0.000000000000000000 ) ) ;
#26289=CARTESIAN_POINT ( 'NONE',  ( 37.00000000000000711, 9.821084925794670184, 7.215058775251142364 ) ) ;
#26290=ADVANCED_FACE ( 'NONE', ( #9599 ), #54856, .T. ) ;
#26291=CARTESIAN_POINT ( 'NONE',  ( 16.78263030916553333, 25.00000000000000000, 5.836879698929882565 ) ) ;
#26292=DIRECTION ( 'NONE',  ( 1.000000000000000000, 0.000000000000000000, 0.000000000000000000 ) ) ;
#26294=CARTESIAN_POINT ( 'NONE',  ( -19.68842116273439657, -11.76428741321061899, -2.390220401484857149 ) ) ;
#26295=CARTESIAN_POINT ( 'NONE',  ( 37.00000000000000711, 4.705694406421931860E-17, -3.469127814946512892E-15 ) ) ;
#26296=ADVANCED_FACE ( 'NONE', ( #65146 ), #13938, .T. ) ;
#26298=ADVANCED_FACE ( 'NONE', ( #45201 ), #14584, .T. ) ;
#26302=CARTESIAN_POINT ( 'NONE',  ( -37.00000000000000711, -6.950793414699719008, -10.68873102412850074 ) ) ;
#26305=ORIENTED_EDGE ( 'NONE', *, *, #11458, .F. ) ;
#26307=CARTESIAN_POINT ( 'NONE',  ( 26.34661844826604593, -11.53221627053866527, 3.317828791472333005 ) ) ;
#26309=DIRECTION ( 'NONE',  ( 0.000000000000000000, 0.8989688749565142301, 0.4380125133594005016 ) ) ;
#26311=DIRECTION ( 'NONE',  ( 0.000000000000000000, 0.01356324068817998940, -0.9999080150203990547 ) ) ;
#26313=AXIS2_PLACEMENT_3D ( 'NONE', #51356, #27356, #31377 ) ;
#26317=CARTESIAN_POINT ( 'NONE',  ( -47.00000000000000711, 0.000000000000000000, 0.000000000000000000 ) ) ;
#26320=ORIENTED_EDGE ( 'NONE', *, *, #48480, .T. ) ;
#26323=DIRECTION ( 'NONE',  ( 0.000000000000000000, 0.01356324068817998940, -0.9999080150203990547 ) ) ;
#26325=CARTESIAN_POINT ( 'NONE',  ( -35.00000000000000000, 0.000000000000000000, 0.000000000000000000 ) ) ;
#26328=CARTESIAN_POINT ( 'NONE',  ( -37.00000000000000711, -0.3025107581132014389, 11.74226168163341200 ) ) ;
#26331=CYLINDRICAL_SURFACE ( 'NONE', #43718, 12.74999999999999822 ) ;
#26332=VERTEX_POINT ( 'NONE', #4317 ) ;
#26333=CARTESIAN_POINT ( 'NONE',  ( -36.00000000000000711, -7.608228585767650820, -10.23119532541081078 ) ) ;
#26335=ORIENTED_EDGE ( 'NONE', *, *, #58452, .T. ) ;
#26338=ORIENTED_EDGE ( 'NONE', *, *, #46571, .F. ) ;
#26340=FACE_OUTER_BOUND ( 'NONE', #33661, .T. ) ;
#26343=DIRECTION ( 'NONE',  ( 1.000000000000000000, 0.000000000000000000, 0.000000000000000000 ) ) ;
#26344=EDGE_CURVE ( 'NONE', #3284, #21988, #4169, .T. ) ;
#26346=CARTESIAN_POINT ( 'NONE',  ( 6.361445718264521432, -4.355102044641763648, 12.77822703589027320 ) ) ;
#26349=DIRECTION ( 'NONE',  ( 1.000000000000000000, 0.000000000000000000, 0.000000000000000000 ) ) ;
#26351=DIRECTION ( 'NONE',  ( -1.000000000000000000, 0.000000000000000000, 0.000000000000000000 ) ) ;
#26355=AXIS2_PLACEMENT_3D ( 'NONE', #42505, #26261, #16615 ) ;
#26356=VECTOR ( 'NONE', #25295, 1000.000000000000000 ) ;
#26357=CARTESIAN_POINT ( 'NONE',  ( 3.618571554686948577, 8.318316264554038497, 8.649151353875890180 ) ) ;
#26358=CARTESIAN_POINT ( 'NONE',  ( 37.00000000000000711, 10.07641281632177588, -6.036400161834603928 ) ) ;
#26359=CARTESIAN_POINT ( 'NONE',  ( -37.00000000000000711, -10.64792938439751424, -5.927257550915432383 ) ) ;
#26365=EDGE_CURVE ( 'NONE', #62061, #41285, #51993, .T. ) ;
#26366=ORIENTED_EDGE ( 'NONE', *, *, #13430, .T. ) ;
#26367=CARTESIAN_POINT ( 'NONE',  ( -18.08686583997218733, 5.151216734910788908, 12.47858029384653733 ) ) ;
#26368=CARTESIAN_POINT ( 'NONE',  ( 6.788772321873702609, -6.731768924035796964, 11.70805477083968782 ) ) ;
#26372=CARTESIAN_POINT ( 'NONE',  ( -9.810797966268966164, 12.34121403900716984, -5.475695573403694283 ) ) ;
#26376=EDGE_LOOP ( 'NONE', ( #64627, #38131, #58238, #50321 ) ) ;
#26378=ORIENTED_EDGE ( 'NONE', *, *, #16393, .T. ) ;
#26379=EDGE_LOOP ( 'NONE', ( #879, #35259, #39572, #17219 ) ) ;
#26382=CYLINDRICAL_SURFACE ( 'NONE', #54977, 13.50000000000000178 ) ;
#26383=CIRCLE ( 'NONE', #44452, 4.999999999999999112 ) ;
#26384=VERTEX_POINT ( 'NONE', #9277 ) ;
#26385=FACE_OUTER_BOUND ( 'NONE', #13519, .T. ) ;
#26387=CARTESIAN_POINT ( 'NONE',  ( -37.00000000000000711, 3.213188559034398040, -11.29812557209473667 ) ) ;
#26388=CARTESIAN_POINT ( 'NONE',  ( -47.00000000000000711, 0.000000000000000000, 0.000000000000000000 ) ) ;
#26389=ORIENTED_EDGE ( 'NONE', *, *, #64345, .T. ) ;
#26392=DIRECTION ( 'NONE',  ( 0.000000000000000000, -0.7381862504171878836, 0.6745969609292743474 ) ) ;
#26395=CARTESIAN_POINT ( 'NONE',  ( -28.15409021793930933, 11.30913317806512985, -4.025053242516860585 ) ) ;
#26397=LINE ( 'NONE', #62609, #61422 ) ;
#26398=VERTEX_POINT ( 'NONE', #35204 ) ;
#26399=ORIENTED_EDGE ( 'NONE', *, *, #48260, .T. ) ;
#26401=CARTESIAN_POINT ( 'NONE',  ( -35.00000000000000000, 0.000000000000000000, 0.000000000000000000 ) ) ;
#26402=AXIS2_PLACEMENT_3D ( 'NONE', #32130, #27159, #17181 ) ;
#26403=DIRECTION ( 'NONE',  ( 0.000000000000000000, 0.01356324068817998940, -0.9999080150203989437 ) ) ;
#26405=DIRECTION ( 'NONE',  ( 1.000000000000000000, -0.000000000000000000, 0.000000000000000000 ) ) ;
#26407=DIRECTION ( 'NONE',  ( -1.000000000000000000, -0.000000000000000000, 0.000000000000000000 ) ) ;
#26410=ADVANCED_FACE ( 'NONE', ( #34862 ), #40191, .T. ) ;
#26412=ORIENTED_EDGE ( 'NONE', *, *, #29617, .F. ) ;
#26414=DIRECTION ( 'NONE',  ( 1.000000000000000000, 0.000000000000000000, 0.000000000000000000 ) ) ;
#26416=EDGE_CURVE ( 'NONE', #8847, #8493, #64728, .T. ) ;
#26417=ORIENTED_EDGE ( 'NONE', *, *, #33147, .T. ) ;
#26418=LINE ( 'NONE', #20453, #14732 ) ;
#26419=DIRECTION ( 'NONE',  ( -1.000000000000000000, 0.000000000000000000, -0.000000000000000000 ) ) ;
#26421=DIRECTION ( 'NONE',  ( 0.000000000000000000, 0.9651210252299803338, 0.2618041379715600470 ) ) ;
#26424=EDGE_CURVE ( 'NONE', #52497, #41192, #16039, .T. ) ;
#26425=LINE ( 'NONE', #20785, #46108 ) ;
#26426=VERTEX_POINT ( 'NONE', #52507 ) ;
#26428=DIRECTION ( 'NONE',  ( 1.000000000000000000, 0.000000000000000000, 0.000000000000000000 ) ) ;
#26430=DIRECTION ( 'NONE',  ( -1.000000000000000000, -0.000000000000000000, 0.000000000000000000 ) ) ;
#26433=AXIS2_PLACEMENT_3D ( 'NONE', #22079, #16457, #53343 ) ;
#26434=CARTESIAN_POINT ( 'NONE',  ( 24.05910844200719367, -2.469428917447811678, -13.27331698206481292 ) ) ;
#26436=CYLINDRICAL_SURFACE ( 'NONE', #29909, 12.74999999999999822 ) ;
#26437=VERTEX_POINT ( 'NONE', #16903 ) ;
#26438=DIRECTION ( 'NONE',  ( -0.000000000000000000, -0.000000000000000000, -1.000000000000000000 ) ) ;
#26440=CYLINDRICAL_SURFACE ( 'NONE', #28955, 5.000000000000000888 ) ;
#26442=CIRCLE ( 'NONE', #46628, 12.18649999999999878 ) ;
#26443=CARTESIAN_POINT ( 'NONE',  ( 9.382075856650567758, 2.626741102731213306, -13.24370663063512765 ) ) ;
#26446=ORIENTED_EDGE ( 'NONE', *, *, #49969, .F. ) ;
#26447=CARTESIAN_POINT ( 'NONE',  ( -17.56015734194049216, -5.645012286831811998, -12.26409170071914012 ) ) ;
#26450=ORIENTED_EDGE ( 'NONE', *, *, #61641, .T. ) ;
#26452=CARTESIAN_POINT ( 'NONE',  ( 35.00000000000000000, 10.75351884295727345, -4.725891942574794058 ) ) ;
#26454=AXIS2_PLACEMENT_3D ( 'NONE', #35068, #61339, #26114 ) ;
#26456=ORIENTED_EDGE ( 'NONE', *, *, #54178, .F. ) ;
#26458=EDGE_CURVE ( 'NONE', #21944, #18385, #60525, .T. ) ;
#26460=ORIENTED_EDGE ( 'NONE', *, *, #50156, .F. ) ;
#26462=CYLINDRICAL_SURFACE ( 'NONE', #18130, 12.75000000000000178 ) ;
#26464=CARTESIAN_POINT ( 'NONE',  ( -4.050991451692300238, -11.17498730987891875, 7.585040469053804912 ) ) ;
#26465=DIRECTION ( 'NONE',  ( 0.000000000000000000, 0.000000000000000000, -1.000000000000000000 ) ) ;
#26466=LINE ( 'NONE', #46754, #57354 ) ;
#26467=ORIENTED_EDGE ( 'NONE', *, *, #2867, .T. ) ;
#26468=VERTEX_POINT ( 'NONE', #21229 ) ;
#26469=CARTESIAN_POINT ( 'NONE',  ( -29.60265935865812637, -3.677894516095094879, 12.98940028976120509 ) ) ;
#26472=DIRECTION ( 'NONE',  ( -1.000000000000000000, 0.000000000000000000, 0.000000000000000000 ) ) ;
#26474=CIRCLE ( 'NONE', #63628, 12.74999999999999822 ) ;
#26476=CARTESIAN_POINT ( 'NONE',  ( -35.00000000000000000, -10.49626516989265923, -7.238157050195740183 ) ) ;
#26477=VERTEX_POINT ( 'NONE', #37174 ) ;
#26480=ADVANCED_FACE ( 'NONE', ( #35847 ), #30869, .T. ) ;
#26481=CARTESIAN_POINT ( 'NONE',  ( 37.00000000000000711, 4.705694406421931860E-17, -3.469127814946512892E-15 ) ) ;
#26482=VERTEX_POINT ( 'NONE', #31535 ) ;
#26484=CARTESIAN_POINT ( 'NONE',  ( 29.23219761849493281, -9.462903118444481620, 9.637299545766000008 ) ) ;
#26486=ORIENTED_EDGE ( 'NONE', *, *, #5687, .F. ) ;
#26487=DIRECTION ( 'NONE',  ( -1.000000000000000000, 0.000000000000000000, 0.000000000000000000 ) ) ;
#26488=DIRECTION ( 'NONE',  ( 0.000000000000000000, -0.01356324068817992175, 0.9999080150203990547 ) ) ;
#26489=CARTESIAN_POINT ( 'NONE',  ( 12.52750123246316072, 0.4973700281276248192, 11.98968819674307618 ) ) ;
#26490=DIRECTION ( 'NONE',  ( 0.000000000000000000, -0.01356324068817998940, 0.9999080150203990547 ) ) ;
#26491=VECTOR ( 'NONE', #62200, 1000.000000000000000 ) ;
#26492=DIRECTION ( 'NONE',  ( 0.000000000000000000, 0.1387779952735819222, -0.9903235168508549569 ) ) ;
#26494=EDGE_CURVE ( 'NONE', #4396, #15089, #4292, .T. ) ;
#26495=DIRECTION ( 'NONE',  ( 1.000000000000000000, 0.000000000000000000, -0.000000000000000000 ) ) ;
#26496=AXIS2_PLACEMENT_3D ( 'NONE', #64316, #48714, #63645 ) ;
#26497=ORIENTED_EDGE ( 'NONE', *, *, #2001, .F. ) ;
#26499=ADVANCED_FACE ( 'NONE', ( #38496 ), #58464, .T. ) ;
#26500=CARTESIAN_POINT ( 'NONE',  ( 35.00000000000000000, 10.14408668126221613, 5.921969905510239940 ) ) ;
#26502=CARTESIAN_POINT ( 'NONE',  ( -35.00000000000000000, 0.000000000000000000, 0.000000000000000000 ) ) ;
#26503=DIRECTION ( 'NONE',  ( -1.000000000000000000, 0.000000000000000000, 0.000000000000000000 ) ) ;
#26504=CARTESIAN_POINT ( 'NONE',  ( 35.00000000000000000, -4.824807283154205706, -11.80185301892979055 ) ) ;
#26506=LINE ( 'NONE', #26193, #31896 ) ;
#26508=ORIENTED_EDGE ( 'NONE', *, *, #20813, .T. ) ;
#26510=CARTESIAN_POINT ( 'NONE',  ( -37.00000000000000711, 0.000000000000000000, 0.000000000000000000 ) ) ;
#26512=ORIENTED_EDGE ( 'NONE', *, *, #11976, .T. ) ;
#26513=CARTESIAN_POINT ( 'NONE',  ( 12.93723047338301058, 4.476360154859203355, 25.00000000000000000 ) ) ;
#26514=CARTESIAN_POINT ( 'NONE',  ( -14.74485252626585741, 7.912425174792709015, -10.93822032635975994 ) ) ;
#26517=DIRECTION ( 'NONE',  ( 0.000000000000000000, 0.9246979985058709772, 0.3807014730195252272 ) ) ;
#26518=ORIENTED_EDGE ( 'NONE', *, *, #8039, .F. ) ;
#26520=DIRECTION ( 'NONE',  ( 1.000000000000000000, 0.000000000000000000, 0.000000000000000000 ) ) ;
#26522=DIRECTION ( 'NONE',  ( 0.000000000000000000, 0.1387779952735818945, -0.9903235168508549569 ) ) ;
#26524=DIRECTION ( 'NONE',  ( -1.000000000000000000, 0.000000000000000000, -0.000000000000000000 ) ) ;
#26526=ORIENTED_EDGE ( 'NONE', *, *, #35088, .T. ) ;
#26527=AXIS2_PLACEMENT_3D ( 'NONE', #53269, #26680, #2411 ) ;
#26529=ORIENTED_EDGE ( 'NONE', *, *, #51797, .T. ) ;
#26531=CARTESIAN_POINT ( 'NONE',  ( -35.00000000000000000, 12.21925492305362049, 3.640372113593593806 ) ) ;
#26533=LINE ( 'NONE', #31522, #4191 ) ;
#26534=DIRECTION ( 'NONE',  ( 1.000000000000000000, 0.000000000000000000, 0.000000000000000000 ) ) ;
#26536=EDGE_CURVE ( 'NONE', #46522, #61135, #24446, .T. ) ;
#26539=ORIENTED_EDGE ( 'NONE', *, *, #9452, .T. ) ;
#26540=CARTESIAN_POINT ( 'NONE',  ( -30.18541646480307250, -1.190103380016452217, 11.94300686747243745 ) ) ;
#26542=DIRECTION ( 'NONE',  ( 0.000000000000000000, -0.01356324068817991828, 0.9999080150203990547 ) ) ;
#26544=CARTESIAN_POINT ( 'NONE',  ( 35.00000000000000000, 10.39746860227901060, 7.379373053628749624 ) ) ;
#26547=CARTESIAN_POINT ( 'NONE',  ( 35.00000000000000000, -12.42372387097884179, -2.865935305911583519 ) ) ;
#26548=CARTESIAN_POINT ( 'NONE',  ( -35.00000000000000000, 0.000000000000000000, 0.000000000000000000 ) ) ;
#26549=ORIENTED_EDGE ( 'NONE', *, *, #13151, .T. ) ;
#26550=ADVANCED_FACE ( 'NONE', ( #22561 ), #27870, .T. ) ;
#26552=CIRCLE ( 'NONE', #37131, 4.999999999999999112 ) ;
#26553=VERTEX_POINT ( 'NONE', #7241 ) ;
#26554=DIRECTION ( 'NONE',  ( 0.000000000000000000, -0.01356324068817998940, 0.9999080150203990547 ) ) ;
#26557=EDGE_CURVE ( 'NONE', #34540, #39315, #12411, .T. ) ;
#26561=DIRECTION ( 'NONE',  ( 1.000000000000000000, 0.000000000000000000, 0.000000000000000000 ) ) ;
#26564=ORIENTED_EDGE ( 'NONE', *, *, #40860, .T. ) ;
#26566=CARTESIAN_POINT ( 'NONE',  ( 3.489268527502659811, 6.893366482496841918, 11.63752349626312288 ) ) ;
#26567=EDGE_CURVE ( 'NONE', #39182, #5675, #63692, .T. ) ;
#26568=ORIENTED_EDGE ( 'NONE', *, *, #50566, .T. ) ;
#26569=LINE ( 'NONE', #11286, #23132 ) ;
#26572=ORIENTED_EDGE ( 'NONE', *, *, #60296, .F. ) ;
#26578=DIRECTION ( 'NONE',  ( 0.000000000000000000, 0.5987040770935676548, -0.8009703041134167423 ) ) ;
#26579=AXIS2_PLACEMENT_3D ( 'NONE', #18644, #59506, #13934 ) ;
#26580=VERTEX_POINT ( 'NONE', #48179 ) ;
#26582=ORIENTED_EDGE ( 'NONE', *, *, #36510, .T. ) ;
#26584=EDGE_CURVE ( 'NONE', #4143, #39990, #30790, .T. ) ;
#26585=CARTESIAN_POINT ( 'NONE',  ( -35.00000000000000000, -10.49591321039677005, -5.273331777780449592 ) ) ;
#26587=ADVANCED_FACE ( 'NONE', ( #38828 ), #57820, .T. ) ;
#26589=CARTESIAN_POINT ( 'NONE',  ( 35.00000000000000000, 5.130401251914885385, 11.05394794832823813 ) ) ;
#26590=DIRECTION ( 'NONE',  ( -1.000000000000000000, -1.836970198721029688E-16, 0.000000000000000000 ) ) ;
#26592=ORIENTED_EDGE ( 'NONE', *, *, #44339, .T. ) ;
#26594=EDGE_CURVE ( 'NONE', #25848, #45204, #7446, .T. ) ;
#26595=( BOUNDED_CURVE ( )  B_SPLINE_CURVE ( 3, ( #47171, #21889, #62421, #52489 ),
 .UNSPECIFIED., .F., .F. ) 
 B_SPLINE_CURVE_WITH_KNOTS ( ( 4, 4 ),
 ( 0.9133032884833093279, 0.9519776552476308940 ),
 .UNSPECIFIED. ) 
 CURVE ( )  GEOMETRIC_REPRESENTATION_ITEM ( )  RATIONAL_B_SPLINE_CURVE ( ( 1.000000000000000000, 0.9998753616634872277, 0.9998753616634872277, 1.000000000000000000 ) ) 
 REPRESENTATION_ITEM ( '' )  );
#26597=DIRECTION ( 'NONE',  ( 0.000000000000000000, -0.01356324068817998940, 0.9999080150203990547 ) ) ;
#26600=ADVANCED_FACE ( 'NONE', ( #20172 ), #55427, .F. ) ;
#26606=VECTOR ( 'NONE', #65260, 1000.000000000000000 ) ;
#26609=AXIS2_PLACEMENT_3D ( 'NONE', #14840, #41106, #29821 ) ;
#26610=CARTESIAN_POINT ( 'NONE',  ( -20.92021774235402276, 12.94977746786777395, -3.816457577290518266 ) ) ;
#26612=CIRCLE ( 'NONE', #51070, 12.18649999999999878 ) ;
#26614=LINE ( 'NONE', #58114, #11011 ) ;
#26615=CARTESIAN_POINT ( 'NONE',  ( 35.00000000000000000, -1.456211999474423369, -11.65554240571057143 ) ) ;
#26616=AXIS2_PLACEMENT_3D ( 'NONE', #28910, #9576, #35178 ) ;
#26617=EDGE_CURVE ( 'NONE', #44861, #2869, #55341, .T. ) ;
#26618=CIRCLE ( 'NONE', #16026, 5.000000000000000000 ) ;
#26620=ORIENTED_EDGE ( 'NONE', *, *, #25103, .T. ) ;
#26621=ADVANCED_FACE ( 'NONE', ( #60742 ), #60089, .T. ) ;
#26625=DIRECTION ( 'NONE',  ( 1.000000000000000000, 0.000000000000000000, 0.000000000000000000 ) ) ;
#26626=DIRECTION ( 'NONE',  ( -1.000000000000000000, -0.000000000000000000, -0.000000000000000000 ) ) ;
#26628=EDGE_CURVE ( 'NONE', #7491, #48365, #13802, .T. ) ;
#26630=ORIENTED_EDGE ( 'NONE', *, *, #56639, .T. ) ;
#26631=CARTESIAN_POINT ( 'NONE',  ( -35.00000000000000000, -1.771820996347237331, 11.61175578952785692 ) ) ;
#26634=ORIENTED_EDGE ( 'NONE', *, *, #15262, .F. ) ;
#26635=LINE ( 'NONE', #46929, #758 ) ;
#26637=AXIS2_PLACEMENT_3D ( 'NONE', #30980, #62223, #61556 ) ;
#26638=DIRECTION ( 'NONE',  ( 1.000000000000000000, 0.000000000000000000, -0.000000000000000000 ) ) ;
#26640=CARTESIAN_POINT ( 'NONE',  ( 47.00000000000000711, 4.705694406421931860E-17, -3.469127814946512892E-15 ) ) ;
#26644=AXIS2_PLACEMENT_3D ( 'NONE', #38912, #54206, #8649 ) ;
#26646=EDGE_CURVE ( 'NONE', #32268, #36353, #12760, .T. ) ;
#26647=ORIENTED_EDGE ( 'NONE', *, *, #46386, .T. ) ;
#26648=CARTESIAN_POINT ( 'NONE',  ( 35.00000000000000000, 6.657191900728455458, 9.677500615117825333 ) ) ;
#26650=ADVANCED_FACE ( 'NONE', ( #8895 ), #18878, .T. ) ;
#26651=CARTESIAN_POINT ( 'NONE',  ( 37.00000000000000711, 4.705694406421931860E-17, -3.469127814946512892E-15 ) ) ;
#26653=CARTESIAN_POINT ( 'NONE',  ( -35.00000000000000000, 7.238157050195777487, -10.49626516989263614 ) ) ;
#26654=CARTESIAN_POINT ( 'NONE',  ( 8.437200413559441614, 4.476360154859203355, 11.13383131558893346 ) ) ;
#26657=VERTEX_POINT ( 'NONE', #23879 ) ;
#26660=EDGE_LOOP ( 'NONE', ( #46389, #22055, #9497, #46924 ) ) ;
#26661=DIRECTION ( 'NONE',  ( -1.000000000000000000, 0.000000000000000000, 0.000000000000000000 ) ) ;
#26663=CIRCLE ( 'NONE', #11785, 4.999999999999998224 ) ;
#26664=ORIENTED_EDGE ( 'NONE', *, *, #16291, .T. ) ;
#26667=CARTESIAN_POINT ( 'NONE',  ( -35.00000000000000000, -8.699265615722922007, -8.534258022646191932 ) ) ;
#26668=CARTESIAN_POINT ( 'NONE',  ( 37.00000000000000711, 4.705694406421931860E-17, -3.469127814946512892E-15 ) ) ;
#26669=ADVANCED_FACE ( 'NONE', ( #44445 ), #40111, .T. ) ;
#26670=ORIENTED_EDGE ( 'NONE', *, *, #51670, .T. ) ;
#26672=AXIS2_PLACEMENT_3D ( 'NONE', #42365, #7144, #52717 ) ;
#26673=VECTOR ( 'NONE', #56727, 1000.000000000000000 ) ;
#26674=AXIS2_PLACEMENT_3D ( 'NONE', #48625, #38639, #48960 ) ;
#26675=ORIENTED_EDGE ( 'NONE', *, *, #20799, .T. ) ;
#26676=CARTESIAN_POINT ( 'NONE',  ( -19.47984447937493613, -3.750539801530005768, -11.39883551934754102 ) ) ;
#26677=ADVANCED_FACE ( 'NONE', ( #39803 ), #55089, .T. ) ;
#26678=AXIS2_PLACEMENT_3D ( 'NONE', #47125, #36475, #26488 ) ;
#26680=DIRECTION ( 'NONE',  ( -1.000000000000000000, 0.000000000000000000, -0.000000000000000000 ) ) ;
#26681=CYLINDRICAL_SURFACE ( 'NONE', #27085, 12.18649999999999878 ) ;
#26683=CARTESIAN_POINT ( 'NONE',  ( -14.11589373245165469, 8.250315036047107142, 25.00000000000000000 ) ) ;
#26684=ORIENTED_EDGE ( 'NONE', *, *, #63346, .F. ) ;
#26686=CIRCLE ( 'NONE', #6477, 12.74999999999999822 ) ;
#26689=AXIS2_PLACEMENT_3D ( 'NONE', #25965, #50585, #35257 ) ;
#26693=CARTESIAN_POINT ( 'NONE',  ( -35.00000000000000000, 8.624332853796195408, -9.390600770287898413 ) ) ;
#26694=DIRECTION ( 'NONE',  ( 1.000000000000000000, 0.000000000000000000, 0.000000000000000000 ) ) ;
#26696=CARTESIAN_POINT ( 'NONE',  ( -35.00000000000000000, 1.463443770872774774, 12.09831040184924866 ) ) ;
#26697=VECTOR ( 'NONE', #42417, 1000.000000000000000 ) ;
#26700=CARTESIAN_POINT ( 'NONE',  ( 35.00000000000000000, 12.46157735505189024, -2.696588552979104492 ) ) ;
#26702=EDGE_CURVE ( 'NONE', #47803, #4063, #65062, .T. ) ;
#26703=ORIENTED_EDGE ( 'NONE', *, *, #40168, .T. ) ;
#26706=EDGE_LOOP ( 'NONE', ( #9250, #32520, #59922, #62870 ) ) ;
#26708=AXIS2_PLACEMENT_3D ( 'NONE', #24586, #38310, #19614 ) ;
#26709=LINE ( 'NONE', #1459, #33055 ) ;
#26711=DIRECTION ( 'NONE',  ( -1.000000000000000000, 0.000000000000000000, 0.000000000000000000 ) ) ;
#26713=ORIENTED_EDGE ( 'NONE', *, *, #15533, .T. ) ;
#26716=AXIS2_PLACEMENT_3D ( 'NONE', #11360, #62231, #42250 ) ;
#26717=B_SPLINE_CURVE_WITH_KNOTS ( 'NONE', 3,
 ( #1446, #53940, #58619, #8380, #53627, #64234, #18709, #3421, #33650, #12692, #13039, #23027, #13363, #28654, #9035, #24011, #63903, #8065, #14011, #33325, #48628, #29313 ),
 .UNSPECIFIED., .F., .F.,
 ( 4, 2, 2, 2, 2, 2, 2, 2, 2, 2, 4 ),
 ( 0.000000000000000000, 0.0006972416122780116313, 0.001394483224556023263, 0.002788966449112044790, 0.004183449673668066318, 0.004880691285946077949, 0.005577932898224087846, 0.006972416122780110241, 0.008366899347336134371, 0.009761382571892159368, 0.01115586579644818437 ),
 .UNSPECIFIED. ) ;
#26719=ORIENTED_EDGE ( 'NONE', *, *, #61614, .F. ) ;
#26720=CARTESIAN_POINT ( 'NONE',  ( -25.28055712087207496, -6.343239884292907860, 10.19231694478317785 ) ) ;
#26722=CARTESIAN_POINT ( 'NONE',  ( 35.00000000000000000, 0.6593684648220492495, -12.73293890771483738 ) ) ;
#26723=CARTESIAN_POINT ( 'NONE',  ( 8.621148270653568702, 25.00000000000000000, -5.251012286260225537 ) ) ;
#26724=ORIENTED_EDGE ( 'NONE', *, *, #2640, .F. ) ;
#26725=DIRECTION ( 'NONE',  ( -0.000000000000000000, -1.000000000000000000, -0.000000000000000000 ) ) ;
#26728=CARTESIAN_POINT ( 'NONE',  ( -25.19743177864295447, 5.013274974602487610, 10.93390578225709397 ) ) ;
#26731=DIRECTION ( 'NONE',  ( -1.000000000000000000, 0.000000000000000000, 0.000000000000000000 ) ) ;
#26732=EDGE_CURVE ( 'NONE', #40151, #743, #26466, .T. ) ;
#26733=VERTEX_POINT ( 'NONE', #20509 ) ;
#26735=ORIENTED_EDGE ( 'NONE', *, *, #49036, .F. ) ;
#26737=VECTOR ( 'NONE', #22823, 1000.000000000000000 ) ;
#26739=ADVANCED_FACE ( 'NONE', ( #30784 ), #61378, .T. ) ;
#26741=ORIENTED_EDGE ( 'NONE', *, *, #34192, .T. ) ;
#26742=CARTESIAN_POINT ( 'NONE',  ( 35.00000000000000000, 4.705694406421931860E-17, -3.469127814946512892E-15 ) ) ;
#26747=VERTEX_POINT ( 'NONE', #5218 ) ;
#26748=AXIS2_PLACEMENT_3D ( 'NONE', #33434, #3186, #61633 ) ;
#26750=CIRCLE ( 'NONE', #63905, 12.18650000000000233 ) ;
#26751=DIRECTION ( 'NONE',  ( 1.000000000000000000, -0.000000000000000000, 0.000000000000000000 ) ) ;
#26753=CARTESIAN_POINT ( 'NONE',  ( 37.00000000000000711, 12.08151691381189963, -4.074242145636052470 ) ) ;
#26755=FACE_OUTER_BOUND ( 'NONE', #53636, .T. ) ;
#26757=CARTESIAN_POINT ( 'NONE',  ( 35.00000000000000000, 4.705694406421931860E-17, -3.469127814946512892E-15 ) ) ;
#26758=DIRECTION ( 'NONE',  ( 0.9703875065674330003, 0.000000000000000000, 0.2415534870330798278 ) ) ;
#26759=ORIENTED_EDGE ( 'NONE', *, *, #37561, .F. ) ;
#26761=CARTESIAN_POINT ( 'NONE',  ( -4.045887249688725262, -9.479482157611457183, 7.361438422396102688 ) ) ;
#26763=EDGE_CURVE ( 'NONE', #136, #43267, #21273, .T. ) ;
#26764=CIRCLE ( 'NONE', #63922, 12.18649999999999878 ) ;
#26765=CARTESIAN_POINT ( 'NONE',  ( 12.52750123246316072, 0.4973700281276248192, -11.98968819674306374 ) ) ;
#26768=LINE ( 'NONE', #27099, #46846 ) ;
#26769=CARTESIAN_POINT ( 'NONE',  ( 12.19544574952904803, 0.02891895647919810047, -11.99999999999999645 ) ) ;
#26770=VERTEX_POINT ( 'NONE', #61711 ) ;
#26775=VECTOR ( 'NONE', #25682, 1000.000000000000000 ) ;
#26776=LINE ( 'NONE', #42364, #19272 ) ;
#26777=CARTESIAN_POINT ( 'NONE',  ( -27.27855387000350262, -12.26939275170277632, 5.631341004100471892 ) ) ;
#26778=EDGE_CURVE ( 'NONE', #62894, #9194, #51763, .T. ) ;
#26779=ORIENTED_EDGE ( 'NONE', *, *, #49302, .F. ) ;
#26780=DIRECTION ( 'NONE',  ( 1.000000000000000000, -0.000000000000000000, 0.000000000000000000 ) ) ;
#26781=CARTESIAN_POINT ( 'NONE',  ( 29.03457606387295087, 25.00000000000000000, 10.97436308512422265 ) ) ;
#26783=DIRECTION ( 'NONE',  ( -1.000000000000000000, 0.000000000000000000, -0.000000000000000000 ) ) ;
#26786=CARTESIAN_POINT ( 'NONE',  ( -35.00000000000000000, 0.000000000000000000, 0.000000000000000000 ) ) ;
#26787=FACE_OUTER_BOUND ( 'NONE', #45312, .T. ) ;
#26796=CARTESIAN_POINT ( 'NONE',  ( 37.00000000000000711, 4.705694406421931860E-17, -3.469127814946512892E-15 ) ) ;
#26798=DIRECTION ( 'NONE',  ( 0.000000000000000000, 0.4935949184179261873, -0.8696919319575183716 ) ) ;
#26800=CARTESIAN_POINT ( 'NONE',  ( -9.808575974122994978, 9.959513386048705286, -6.707583712996705749 ) ) ;
#26808=ORIENTED_EDGE ( 'NONE', *, *, #29801, .F. ) ;
#26809=AXIS2_PLACEMENT_3D ( 'NONE', #20675, #5726, #25996 ) ;
#26811=AXIS2_PLACEMENT_3D ( 'NONE', #34058, #54372, #19447 ) ;
#26812=CARTESIAN_POINT ( 'NONE',  ( -17.90332768477131609, 4.129650048207996527, 11.26888906344803587 ) ) ;
#26813=CIRCLE ( 'NONE', #15073, 12.18650000000000233 ) ;
#26814=DIRECTION ( 'NONE',  ( -1.000000000000000000, 0.000000000000000000, 0.000000000000000000 ) ) ;
#26816=DIRECTION ( 'NONE',  ( -1.000000000000000000, 0.000000000000000000, -0.000000000000000000 ) ) ;
#26819=ORIENTED_EDGE ( 'NONE', *, *, #62677, .T. ) ;
#26820=VERTEX_POINT ( 'NONE', #37094 ) ;
#26822=ORIENTED_EDGE ( 'NONE', *, *, #58759, .F. ) ;
#26825=LINE ( 'NONE', #47126, #15061 ) ;
#26827=VECTOR ( 'NONE', #45507, 1000.000000000000000 ) ;
#26828=CARTESIAN_POINT ( 'NONE',  ( 35.00000000000000000, -7.817610399097575602, -8.766823244861962294 ) ) ;
#26830=DIRECTION ( 'NONE',  ( 1.000000000000000000, 0.000000000000000000, -0.000000000000000000 ) ) ;
#26831=VERTEX_POINT ( 'NONE', #57393 ) ;
#26833=DIRECTION ( 'NONE',  ( 0.000000000000000000, -0.01356324068817992175, 0.9999080150203990547 ) ) ;
#26834=ORIENTED_EDGE ( 'NONE', *, *, #54520, .F. ) ;
#26835=VECTOR ( 'NONE', #27544, 1000.000000000000000 ) ;
#26838=CARTESIAN_POINT ( 'NONE',  ( -9.340672490813821227, 10.24685145699743494, -6.257124625858472733 ) ) ;
#26840=DIRECTION ( 'NONE',  ( 1.000000000000000000, 0.000000000000000000, 0.000000000000000000 ) ) ;
#26841=DIRECTION ( 'NONE',  ( -1.000000000000000000, 0.000000000000000000, 0.000000000000000000 ) ) ;
#26842=ORIENTED_EDGE ( 'NONE', *, *, #18122, .F. ) ;
#26843=ADVANCED_FACE ( 'NONE', ( #22810 ), #48083, .T. ) ;
#26845=DIRECTION ( 'NONE',  ( 0.000000000000000000, -0.01356324068817999808, 0.9999080150203990547 ) ) ;
#26846=VECTOR ( 'NONE', #32462, 1000.000000000000000 ) ;
#26847=EDGE_LOOP ( 'NONE', ( #16273, #53161, #61074, #40563 ) ) ;
#26848=CARTESIAN_POINT ( 'NONE',  ( -35.00000000000000000, -11.13736569743278082, 4.946702696913133579 ) ) ;
#26853=CIRCLE ( 'NONE', #47043, 12.18650000000000233 ) ;
#26854=FACE_OUTER_BOUND ( 'NONE', #61691, .T. ) ;
#26856=DIRECTION ( 'NONE',  ( 0.000000000000000000, -0.01356324068817998940, 0.9999080150203990547 ) ) ;
#26858=AXIS2_PLACEMENT_3D ( 'NONE', #52137, #56816, #1272 ) ;
#26859=CIRCLE ( 'NONE', #56581, 5.000000000000000888 ) ;
#26860=EDGE_CURVE ( 'NONE', #50602, #12850, #53125, .T. ) ;
#26861=CARTESIAN_POINT ( 'NONE',  ( -35.00000000000000000, -11.65150730582933392, -1.488153103997089888 ) ) ;
#26864=EDGE_CURVE ( 'NONE', #31963, #2241, #47741, .T. ) ;
#26865=AXIS2_PLACEMENT_3D ( 'NONE', #759, #22012, #11695 ) ;
#26866=DIRECTION ( 'NONE',  ( 1.000000000000000000, 0.000000000000000000, 0.000000000000000000 ) ) ;
#26867=ORIENTED_EDGE ( 'NONE', *, *, #61393, .T. ) ;
#26868=EDGE_CURVE ( 'NONE', #11644, #63443, #32932, .T. ) ;
#26869=CARTESIAN_POINT ( 'NONE',  ( -25.54417658651491863, -4.240019242199836391, 11.22596262356930197 ) ) ;
#26870=DIRECTION ( 'NONE',  ( 1.000000000000000000, 0.000000000000000000, 0.000000000000000000 ) ) ;
#26871=DIRECTION ( 'NONE',  ( 0.000000000000000000, 0.01356324068817991828, -0.9999080150203990547 ) ) ;
#26875=ORIENTED_EDGE ( 'NONE', *, *, #15162, .F. ) ;
#26876=EDGE_CURVE ( 'NONE', #37186, #54640, #43728, .T. ) ;
#26877=ORIENTED_EDGE ( 'NONE', *, *, #26628, .F. ) ;
#26880=CARTESIAN_POINT ( 'NONE',  ( 3.355386238882536620, 7.941827888624184872, 9.005989223246164244 ) ) ;
#26881=CARTESIAN_POINT ( 'NONE',  ( 2.700868940011170949, 3.106162501881789773, -13.16183552361884779 ) ) ;
#26882=CARTESIAN_POINT ( 'NONE',  ( 22.21053567399755835, -13.47268488964859046, -0.8606552803710496580 ) ) ;
#26883=CARTESIAN_POINT ( 'NONE',  ( -37.00000000000000711, 0.000000000000000000, 0.000000000000000000 ) ) ;
#26886=AXIS2_PLACEMENT_3D ( 'NONE', #55630, #35648, #46305 ) ;
#26888=CARTESIAN_POINT ( 'NONE',  ( -11.14943813774385539, -5.657473984827134039, 10.59121631773951222 ) ) ;
#26889=ORIENTED_EDGE ( 'NONE', *, *, #25139, .F. ) ;
#26892=DIRECTION ( 'NONE',  ( 1.000000000000000000, 0.000000000000000000, 0.000000000000000000 ) ) ;
#26893=CARTESIAN_POINT ( 'NONE',  ( 22.02145101462502197, -12.24345070192289775, -5.700244587874106372 ) ) ;
#26901=DIRECTION ( 'NONE',  ( 1.000000000000000000, 0.000000000000000000, 0.000000000000000000 ) ) ;
#26902=ORIENTED_EDGE ( 'NONE', *, *, #46756, .F. ) ;
#26903=ORIENTED_EDGE ( 'NONE', *, *, #26365, .T. ) ;
#26905=CARTESIAN_POINT ( 'NONE',  ( 35.00000000000000000, 9.821084925794670184, 7.215058775251142364 ) ) ;
#26908=CIRCLE ( 'NONE', #43893, 12.18649999999999878 ) ;
#26909=CIRCLE ( 'NONE', #57721, 12.74999999999999822 ) ;
#26910=ORIENTED_EDGE ( 'NONE', *, *, #21503, .F. ) ;
#26911=VERTEX_POINT ( 'NONE', #43066 ) ;
#26913=DIRECTION ( 'NONE',  ( 0.000000000000000000, 0.01356324068817992175, -0.9999080150203990547 ) ) ;
#26915=CIRCLE ( 'NONE', #64066, 12.18650000000000055 ) ;
#26916=CARTESIAN_POINT ( 'NONE',  ( -19.61329546411680624, -11.94675665305282841, -1.284421273215466508 ) ) ;
#26918=CARTESIAN_POINT ( 'NONE',  ( 36.00000000000000711, 9.913596905230228629, 8.017674001891673896 ) ) ;
#26919=VERTEX_POINT ( 'NONE', #17153 ) ;
#26920=LINE ( 'NONE', #42183, #29025 ) ;
#26924=FACE_OUTER_BOUND ( 'NONE', #41953, .T. ) ;
#26926=CARTESIAN_POINT ( 'NONE',  ( 37.00000000000000711, -8.496612874013091954, 9.506317355798454827 ) ) ;
#26927=DIRECTION ( 'NONE',  ( 0.000000000000000000, 0.01356324068817992175, -0.9999080150203990547 ) ) ;
#26928=DIRECTION ( 'NONE',  ( 0.000000000000000000, -0.01356324068817991828, 0.9999080150203990547 ) ) ;
#26930=EDGE_CURVE ( 'NONE', #48396, #50472, #28429, .T. ) ;
#26931=VERTEX_POINT ( 'NONE', #12158 ) ;
#26933=AXIS2_PLACEMENT_3D ( 'NONE', #26388, #11419, #16080 ) ;
#26937=FACE_OUTER_BOUND ( 'NONE', #28140, .T. ) ;
#26938=DIRECTION ( 'NONE',  ( -0.000000000000000000, -1.000000000000000000, -0.000000000000000000 ) ) ;
#26940=ORIENTED_EDGE ( 'NONE', *, *, #56271, .F. ) ;
#26941=EDGE_CURVE ( 'NONE', #63262, #16803, #1372, .T. ) ;
#26942=FACE_OUTER_BOUND ( 'NONE', #7046, .T. ) ;
#26945=DIRECTION ( 'NONE',  ( 0.000000000000000000, 0.9551603052523489623, -0.2960891610144475439 ) ) ;
#26948=DIRECTION ( 'NONE',  ( 0.000000000000000000, -0.01356324068817998940, 0.9999080150203990547 ) ) ;
#26949=ORIENTED_EDGE ( 'NONE', *, *, #32115, .F. ) ;
#26953=VECTOR ( 'NONE', #58809, 1000.000000000000000 ) ;
#26954=AXIS2_PLACEMENT_3D ( 'NONE', #49805, #64114, #18595 ) ;
#26955=CIRCLE ( 'NONE', #43955, 4.999999999999999112 ) ;
#26957=ORIENTED_EDGE ( 'NONE', *, *, #47772, .T. ) ;
#26959=AXIS2_PLACEMENT_3D ( 'NONE', #47078, #52057, #52396 ) ;
#26961=LINE ( 'NONE', #21969, #11991 ) ;
#26962=EDGE_CURVE ( 'NONE', #20989, #815, #57400, .T. ) ;
#26964=CYLINDRICAL_SURFACE ( 'NONE', #2096, 12.74999999999999822 ) ;
#26965=ORIENTED_EDGE ( 'NONE', *, *, #28261, .T. ) ;
#26967=AXIS2_PLACEMENT_3D ( 'NONE', #41072, #36750, #40412 ) ;
#26968=ORIENTED_EDGE ( 'NONE', *, *, #55702, .F. ) ;
#26970=DIRECTION ( 'NONE',  ( 1.000000000000000000, 0.000000000000000000, -0.000000000000000000 ) ) ;
#26971=ADVANCED_FACE ( 'NONE', ( #64008 ), #33740, .T. ) ;
#26972=CIRCLE ( 'NONE', #56753, 12.18649999999999878 ) ;
#26973=DIRECTION ( 'NONE',  ( -0.000000000000000000, -0.000000000000000000, -1.000000000000000000 ) ) ;
#26974=VERTEX_POINT ( 'NONE', #8817 ) ;
#26975=EDGE_CURVE ( 'NONE', #28034, #51695, #44693, .T. ) ;
#26977=EDGE_CURVE ( 'NONE', #24332, #6547, #18148, .T. ) ;
#26979=ORIENTED_EDGE ( 'NONE', *, *, #26977, .T. ) ;
#26980=CARTESIAN_POINT ( 'NONE',  ( -37.00000000000000711, 3.287724142101577485, -11.73463472867572932 ) ) ;
#26981=CIRCLE ( 'NONE', #24844, 12.74999999999999822 ) ;
#26983=CARTESIAN_POINT ( 'NONE',  ( -35.00000000000000000, 11.81949347079751256, -2.968224442958276921 ) ) ;
#26984=VERTEX_POINT ( 'NONE', #50380 ) ;
#26986=CARTESIAN_POINT ( 'NONE',  ( -35.00000000000000000, 5.556331110570408960, 11.47561260193578825 ) ) ;
#26987=EDGE_LOOP ( 'NONE', ( #40289, #58254, #35105, #32523, #52893, #17874 ) ) ;
#26988=CARTESIAN_POINT ( 'NONE',  ( 35.00000000000000000, 12.60630747491662973, -1.908798535168425792 ) ) ;
#26989=ORIENTED_EDGE ( 'NONE', *, *, #44290, .F. ) ;
#26990=CARTESIAN_POINT ( 'NONE',  ( -17.77096676138755527, -6.470721604686525907, 11.85175806654005903 ) ) ;
#26991=DIRECTION ( 'NONE',  ( 1.000000000000000000, -0.000000000000000000, 0.000000000000000000 ) ) ;
#26992=DIRECTION ( 'NONE',  ( 0.000000000000000000, 0.01356324068817991828, -0.9999080150203990547 ) ) ;
#26995=CARTESIAN_POINT ( 'NONE',  ( 35.00000000000000000, 3.340853584269691368, 11.26103545359851665 ) ) ;
#26998=LINE ( 'NONE', #52285, #13072 ) ;
#27000=ORIENTED_EDGE ( 'NONE', *, *, #47667, .F. ) ;
#27001=FACE_OUTER_BOUND ( 'NONE', #33330, .T. ) ;
#27002=DIRECTION ( 'NONE',  ( 1.000000000000000000, -0.000000000000000000, 0.000000000000000000 ) ) ;
#27005=CARTESIAN_POINT ( 'NONE',  ( -17.67713918426279918, 7.443964916031736045, 9.415221461658108026 ) ) ;
#27007=CARTESIAN_POINT ( 'NONE',  ( -21.24030193723618609, 25.00000000000000000, -5.230344621181295395 ) ) ;
#27009=ORIENTED_EDGE ( 'NONE', *, *, #10726, .T. ) ;
#27010=ADVANCED_FACE ( 'NONE', ( #3526 ), #4498, .T. ) ;
#27011=ORIENTED_EDGE ( 'NONE', *, *, #32266, .T. ) ;
#27012=DIRECTION ( 'NONE',  ( -1.000000000000000000, -0.000000000000000000, -0.000000000000000000 ) ) ;
#27015=CARTESIAN_POINT ( 'NONE',  ( 35.00000000000000000, 4.705694406421931860E-17, -3.469127814946512892E-15 ) ) ;
#27016=CARTESIAN_POINT ( 'NONE',  ( -3.491682519919724115, -11.78917057717144345, 6.588009498355533289 ) ) ;
#27017=DIRECTION ( 'NONE',  ( 0.000000000000000000, -0.01356324068818000848, 0.9999080150203990547 ) ) ;
#27018=ORIENTED_EDGE ( 'NONE', *, *, #12007, .T. ) ;
#27019=CIRCLE ( 'NONE', #63083, 12.75000000000000178 ) ;
#27022=CIRCLE ( 'NONE', #34458, 12.18650000000000055 ) ;
#27024=DIRECTION ( 'NONE',  ( -1.000000000000000000, 0.000000000000000000, 0.000000000000000000 ) ) ;
#27026=DIRECTION ( 'NONE',  ( 0.000000000000000000, -0.6745969609292555846, -0.7381862504172049810 ) ) ;
#27027=CARTESIAN_POINT ( 'NONE',  ( 37.00000000000000711, -7.146664589317845540, 9.321877890560507751 ) ) ;
#27028=ADVANCED_FACE ( 'NONE', ( #64643 ), #38748, .T. ) ;
#27032=VECTOR ( 'NONE', #39837, 1000.000000000000000 ) ;
#27033=VERTEX_POINT ( 'NONE', #9784 ) ;
#27034=DIRECTION ( 'NONE',  ( 0.000000000000000000, 0.01356324068817992175, -0.9999080150203990547 ) ) ;
#27035=DIRECTION ( 'NONE',  ( -0.6845106172691086677, 0.000000000000000000, -0.7290028908350527637 ) ) ;
#27040=FACE_OUTER_BOUND ( 'NONE', #14364, .T. ) ;
#27041=VERTEX_POINT ( 'NONE', #44367 ) ;
#27045=EDGE_LOOP ( 'NONE', ( #23122, #40099, #4581, #418 ) ) ;
#27046=ADVANCED_FACE ( 'NONE', ( #19115 ), #25094, .T. ) ;
#27049=EDGE_LOOP ( 'NONE', ( #59286, #52429, #64425, #65605 ) ) ;
#27050=EDGE_CURVE ( 'NONE', #14653, #46044, #59538, .T. ) ;
#27051=CARTESIAN_POINT ( 'NONE',  ( -26.56525829975939956, -10.48173858536018699, 5.842830346974275280 ) ) ;
#27053=DIRECTION ( 'NONE',  ( -1.000000000000000000, -1.836970198721029688E-16, 0.000000000000000000 ) ) ;
#27055=EDGE_LOOP ( 'NONE', ( #1781, #27076, #15542, #37802 ) ) ;
#27056=DIRECTION ( 'NONE',  ( 1.000000000000000000, 0.000000000000000000, -0.000000000000000000 ) ) ;
#27059=CARTESIAN_POINT ( 'NONE',  ( -24.31558339428802640, 8.695784598849996883, 8.272409342072648997 ) ) ;
#27061=ADVANCED_FACE ( 'NONE', ( #51690 ), #55997, .T. ) ;
#27062=CARTESIAN_POINT ( 'NONE',  ( -28.23735777670677294, 10.53122157488975574, -5.761455423850979862 ) ) ;
#27064=CIRCLE ( 'NONE', #15382, 4.999999999999999112 ) ;
#27067=CARTESIAN_POINT ( 'NONE',  ( 35.00000000000000000, 9.217970097227839332, 7.971186206369370808 ) ) ;
#27071=ORIENTED_EDGE ( 'NONE', *, *, #30507, .F. ) ;
#27072=LINE ( 'NONE', #42019, #32482 ) ;
#27073=DIRECTION ( 'NONE',  ( -1.000000000000000000, -0.000000000000000000, 0.000000000000000000 ) ) ;
#27075=ORIENTED_EDGE ( 'NONE', *, *, #19364, .F. ) ;
#27076=ORIENTED_EDGE ( 'NONE', *, *, #28261, .F. ) ;
#27080=CARTESIAN_POINT ( 'NONE',  ( -27.01437459610461644, 10.69338818478080455, -8.240233560378637634 ) ) ;
#27081=CARTESIAN_POINT ( 'NONE',  ( 35.00000000000000000, -1.908798535168467536, -12.60630747491662618 ) ) ;
#27082=DIRECTION ( 'NONE',  ( 1.000000000000000000, 0.000000000000000000, 0.000000000000000000 ) ) ;
#27083=CARTESIAN_POINT ( 'NONE',  ( -35.00000000000000000, 2.936739658820028520, -11.37311665002360783 ) ) ;
#27085=AXIS2_PLACEMENT_3D ( 'NONE', #16032, #11381, #36660 ) ;
#27086=EDGE_CURVE ( 'NONE', #64921, #34336, #10434, .T. ) ;
#27087=DIRECTION ( 'NONE',  ( 0.000000000000000000, -0.04924826701375277505, -0.9987865678893275145 ) ) ;
#27089=ORIENTED_EDGE ( 'NONE', *, *, #46763, .F. ) ;
#27092=VECTOR ( 'NONE', #3446, 1000.000000000000000 ) ;
#27093=FACE_OUTER_BOUND ( 'NONE', #41603, .T. ) ;
#27094=EDGE_CURVE ( 'NONE', #50042, #12300, #45690, .T. ) ;
#27096=DIRECTION ( 'NONE',  ( 0.000000000000000000, -0.01356324068817991828, 0.9999080150203990547 ) ) ;
#27098=CIRCLE ( 'NONE', #17569, 4.999999999999999112 ) ;
#27099=CARTESIAN_POINT ( 'NONE',  ( -35.00000000000000000, -7.561043153947899498, -9.557269938331636183 ) ) ;
#27101=EDGE_CURVE ( 'NONE', #15014, #12978, #6423, .T. ) ;
#27102=ADVANCED_FACE ( 'NONE', ( #40707 ), #30400, .T. ) ;
#27103=VERTEX_POINT ( 'NONE', #493 ) ;
#27104=DIRECTION ( 'NONE',  ( -1.000000000000000000, 0.000000000000000000, 0.000000000000000000 ) ) ;
#27106=DIRECTION ( 'NONE',  ( -1.000000000000000000, 0.000000000000000000, -0.000000000000000000 ) ) ;
#27107=DIRECTION ( 'NONE',  ( 1.000000000000000000, 0.000000000000000000, -0.000000000000000000 ) ) ;
#27109=AXIS2_PLACEMENT_3D ( 'NONE', #28362, #58980, #39308 ) ;
#27110=CARTESIAN_POINT ( 'NONE',  ( 10.67917606476195580, 1.165423783710027861, -13.45046084793106367 ) ) ;
#27111=CARTESIAN_POINT ( 'NONE',  ( -25.47095544430322889, -11.72962784578977313, 6.684589422636681988 ) ) ;
#27112=ORIENTED_EDGE ( 'NONE', *, *, #56167, .T. ) ;
#27113=CARTESIAN_POINT ( 'NONE',  ( 18.73707042796466027, -5.248124276600211857, 10.80148738011064680 ) ) ;
#27114=DIRECTION ( 'NONE',  ( -1.000000000000000000, 0.000000000000000000, 0.000000000000000000 ) ) ;
#27119=CARTESIAN_POINT ( 'NONE',  ( -35.00000000000000000, 0.000000000000000000, 0.000000000000000000 ) ) ;
#27120=DIRECTION ( 'NONE',  ( 0.000000000000000000, 0.000000000000000000, -1.000000000000000000 ) ) ;
#27122=DIRECTION ( 'NONE',  ( 1.000000000000000000, -0.000000000000000000, 0.000000000000000000 ) ) ;
#27126=EDGE_CURVE ( 'NONE', #48166, #33099, #34032, .T. ) ;
#27127=FACE_OUTER_BOUND ( 'NONE', #64351, .T. ) ;
#27129=DIRECTION ( 'NONE',  ( 0.000000000000000000, 0.01356324068817992001, -0.9999080150203990547 ) ) ;
#27130=CARTESIAN_POINT ( 'NONE',  ( -3.221163217498328901, -8.204480317174903448, 10.72779841256758360 ) ) ;
#27133=CARTESIAN_POINT ( 'NONE',  ( -35.00000000000000000, -9.217970097227665249, -7.971186206369574201 ) ) ;
#27134=ORIENTED_EDGE ( 'NONE', *, *, #57570, .T. ) ;
#27137=ORIENTED_EDGE ( 'NONE', *, *, #56982, .F. ) ;
#27138=CARTESIAN_POINT ( 'NONE',  ( 24.65820709255600818, -2.318610723833587794, -11.78042893945787384 ) ) ;
#27139=ORIENTED_EDGE ( 'NONE', *, *, #44829, .F. ) ;
#27142=CARTESIAN_POINT ( 'NONE',  ( -3.620643385775215162, 10.87206787913274830, 5.083569600177869852 ) ) ;
#27146=AXIS2_PLACEMENT_3D ( 'NONE', #24559, #59820, #64458 ) ;
#27153=CARTESIAN_POINT ( 'NONE',  ( 29.51976981715666781, -7.690765383426355406, 11.09513982864076276 ) ) ;
#27155=CARTESIAN_POINT ( 'NONE',  ( 10.67791943353093309, 1.166253086089546587, 13.45039264577783023 ) ) ;
#27157=CARTESIAN_POINT ( 'NONE',  ( 37.00000000000000711, -12.54989509947652415, -2.250029553613715372 ) ) ;
#27158=DIRECTION ( 'NONE',  ( 1.000000000000000000, -0.000000000000000000, -0.000000000000000000 ) ) ;
#27159=DIRECTION ( 'NONE',  ( -1.000000000000000000, 0.000000000000000000, 0.000000000000000000 ) ) ;
#27160=CARTESIAN_POINT ( 'NONE',  ( 35.00000000000000000, 7.238157050195628273, -10.49626516989273384 ) ) ;
#27162=EDGE_LOOP ( 'NONE', ( #9787, #47859, #47354, #11666 ) ) ;
#27163=DIRECTION ( 'NONE',  ( 1.000000000000000000, 0.000000000000000000, -0.000000000000000000 ) ) ;
#27164=ORIENTED_EDGE ( 'NONE', *, *, #22220, .T. ) ;
#27165=CARTESIAN_POINT ( 'NONE',  ( 35.00000000000000000, 10.80478261802181628, -5.636262487437359248 ) ) ;
#27167=CARTESIAN_POINT ( 'NONE',  ( -27.78468958554971380, 25.00000000000000000, 8.565911087387465983 ) ) ;
#27168=CARTESIAN_POINT ( 'NONE',  ( -35.00000000000000000, 1.030638227056741574, -12.14284015767849034 ) ) ;
#27171=VERTEX_POINT ( 'NONE', #31058 ) ;
#27172=EDGE_CURVE ( 'NONE', #35706, #53805, #37213, .T. ) ;
#27175=ORIENTED_EDGE ( 'NONE', *, *, #18767, .F. ) ;
#27176=CARTESIAN_POINT ( 'NONE',  ( -7.489022030332961322, 8.034049540753141372, -10.84914964302385521 ) ) ;
#27177=CARTESIAN_POINT ( 'NONE',  ( 26.08439714455133185, 12.97057518889166516, 3.743551691817328386 ) ) ;
#27178=DIRECTION ( 'NONE',  ( 1.000000000000000000, 0.000000000000000000, 0.000000000000000000 ) ) ;
#27179=CARTESIAN_POINT ( 'NONE',  ( -37.00000000000000711, -9.196955404009360180, 8.830544224262913744 ) ) ;
#27182=CARTESIAN_POINT ( 'NONE',  ( 26.34661844826604593, -13.08594712317289321, 3.317828791472332117 ) ) ;
#27186=CARTESIAN_POINT ( 'NONE',  ( -35.00000000000000000, 9.733281772932279807, -8.235637554476539890 ) ) ;
#27187=DIRECTION ( 'NONE',  ( 0.000000000000000000, 0.8696919319575200369, 0.4935949184179230786 ) ) ;
#27190=ORIENTED_EDGE ( 'NONE', *, *, #26062, .T. ) ;
#27191=LINE ( 'NONE', #27505, #13724 ) ;
#27192=EDGE_LOOP ( 'NONE', ( #46306, #35236, #17348, #54787 ) ) ;
#27193=CARTESIAN_POINT ( 'NONE',  ( -4.989057617119008192, -0.9162120371760335003, -13.46887357958837406 ) ) ;
#27194=DIRECTION ( 'NONE',  ( 0.000000000000000000, 0.3554799084908900619, 0.9346839223284566511 ) ) ;
#27195=DIRECTION ( 'NONE',  ( 0.000000000000000000, 0.01356324068817998073, -0.9999080150203990547 ) ) ;
#27197=CARTESIAN_POINT ( 'NONE',  ( 3.347841273039249721, -10.61118957148187825, 8.345816669330455184 ) ) ;
#27198=CIRCLE ( 'NONE', #16577, 5.000000000000001776 ) ;
#27199=VERTEX_POINT ( 'NONE', #65623 ) ;
#27200=VERTEX_POINT ( 'NONE', #46359 ) ;
#27201=DIRECTION ( 'NONE',  ( -1.000000000000000000, 0.000000000000000000, 0.000000000000000000 ) ) ;
#27202=ORIENTED_EDGE ( 'NONE', *, *, #14740, .F. ) ;
#27204=DIRECTION ( 'NONE',  ( 1.000000000000000000, 0.000000000000000000, -0.000000000000000000 ) ) ;
#27206=DIRECTION ( 'NONE',  ( 0.000000000000000000, 0.01356324068817998940, -0.9999080150203990547 ) ) ;
#27207=CARTESIAN_POINT ( 'NONE',  ( -37.00000000000000711, -5.644643009978993931, -10.30098186818255890 ) ) ;
#27209=DIRECTION ( 'NONE',  ( 1.000000000000000000, -0.000000000000000000, 0.000000000000000000 ) ) ;
#27210=ORIENTED_EDGE ( 'NONE', *, *, #50456, .F. ) ;
#27211=VERTEX_POINT ( 'NONE', #15100 ) ;
#27213=ORIENTED_EDGE ( 'NONE', *, *, #55883, .T. ) ;
#27216=CARTESIAN_POINT ( 'NONE',  ( 21.63322885546936192, -13.42214251193591679, -1.501346303079956090 ) ) ;
#27218=DIRECTION ( 'NONE',  ( 1.000000000000000000, -0.000000000000000000, 0.000000000000000000 ) ) ;
#27220=EDGE_LOOP ( 'NONE', ( #32016, #23769 ) ) ;
#27221=DIRECTION ( 'NONE',  ( 1.000000000000000000, -0.000000000000000000, 0.000000000000000000 ) ) ;
#27224=VERTEX_POINT ( 'NONE', #27697 ) ;
#27226=DIRECTION ( 'NONE',  ( -1.000000000000000000, -0.000000000000000000, 0.000000000000000000 ) ) ;
#27227=VERTEX_POINT ( 'NONE', #7410 ) ;
#27228=ORIENTED_EDGE ( 'NONE', *, *, #16047, .F. ) ;
#27234=CARTESIAN_POINT ( 'NONE',  ( -37.00000000000000711, 0.000000000000000000, 0.000000000000000000 ) ) ;
#27236=DIRECTION ( 'NONE',  ( 0.000000000000000000, -0.01356324068817998940, 0.9999080150203990547 ) ) ;
#27239=CIRCLE ( 'NONE', #38921, 12.18649999999999878 ) ;
#27240=EDGE_CURVE ( 'NONE', #58346, #30510, #5379, .T. ) ;
#27241=ORIENTED_EDGE ( 'NONE', *, *, #38128, .F. ) ;
#27242=CARTESIAN_POINT ( 'NONE',  ( -35.00000000000000000, 11.99999999999999289, 1.469576158976823158E-15 ) ) ;
#27243=EDGE_CURVE ( 'NONE', #36620, #9122, #47353, .T. ) ;
#27245=ADVANCED_FACE ( 'NONE', ( #7765 ), #48348, .T. ) ;
#27248=CYLINDRICAL_SURFACE ( 'NONE', #62049, 5.000000000000001776 ) ;
#27249=CARTESIAN_POINT ( 'NONE',  ( 37.00000000000000711, 10.01317267707886494, -6.946017217729976601 ) ) ;
#27250=ORIENTED_EDGE ( 'NONE', *, *, #49029, .T. ) ;
#27251=EDGE_CURVE ( 'NONE', #42435, #42706, #30668, .T. ) ;
#27252=CARTESIAN_POINT ( 'NONE',  ( 8.437200413559441614, 4.476360154859203355, 11.13383131558893346 ) ) ;
#27254=EDGE_CURVE ( 'NONE', #43456, #44869, #14460, .T. ) ;
#27256=CARTESIAN_POINT ( 'NONE',  ( -35.00000000000000000, -10.28547182238004076, -5.672855678558794246 ) ) ;
#27258=DIRECTION ( 'NONE',  ( 0.000000000000000000, 0.2006870767258890631, -0.9796553971857742127 ) ) ;
#27260=ORIENTED_EDGE ( 'NONE', *, *, #11308, .T. ) ;
#27261=DIRECTION ( 'NONE',  ( 0.000000000000000000, -0.2960891610144577024, -0.9551603052523457427 ) ) ;
#27263=CARTESIAN_POINT ( 'NONE',  ( 35.00000000000000000, 4.705694406421931860E-17, -3.469127814946512892E-15 ) ) ;
#27265=EDGE_CURVE ( 'NONE', #28690, #2019, #12724, .T. ) ;
#27272=AXIS2_PLACEMENT_3D ( 'NONE', #26325, #46608, #30342 ) ;
#27273=VERTEX_POINT ( 'NONE', #33008 ) ;
#27274=VERTEX_POINT ( 'NONE', #42645 ) ;
#27275=DIRECTION ( 'NONE',  ( 0.000000000000000000, 0.01356324068817998940, -0.9999080150203990547 ) ) ;
#27276=CARTESIAN_POINT ( 'NONE',  ( 37.00000000000000711, 4.705694406421931860E-17, -3.469127814946512892E-15 ) ) ;
#27277=CARTESIAN_POINT ( 'NONE',  ( 37.00000000000000711, 4.705694406421931860E-17, -3.469127814946512892E-15 ) ) ;
#27280=ORIENTED_EDGE ( 'NONE', *, *, #61867, .T. ) ;
#27283=EDGE_CURVE ( 'NONE', #29745, #33694, #17413, .T. ) ;
#27286=ORIENTED_EDGE ( 'NONE', *, *, #9929, .T. ) ;
#27287=CARTESIAN_POINT ( 'NONE',  ( -10.95212338237647920, -9.902220863987562183, 6.778349501228839280 ) ) ;
#27288=CARTESIAN_POINT ( 'NONE',  ( -36.00000000000000711, -9.390600770287932164, -8.624332853796161658 ) ) ;
#27289=ORIENTED_EDGE ( 'NONE', *, *, #14548, .T. ) ;
#27292=CARTESIAN_POINT ( 'NONE',  ( 23.96628737370385664, -3.705566309175509332, 11.41801794016889282 ) ) ;
#27293=ORIENTED_EDGE ( 'NONE', *, *, #21806, .T. ) ;
#27295=ORIENTED_EDGE ( 'NONE', *, *, #5404, .F. ) ;
#27297=CARTESIAN_POINT ( 'NONE',  ( -19.42938127781367896, -4.328328797226848934, 12.78801166805076583 ) ) ;
#27299=DIRECTION ( 'NONE',  ( -1.000000000000000000, 0.000000000000000000, -0.000000000000000000 ) ) ;
#27301=EDGE_CURVE ( 'NONE', #32993, #23007, #41473, .T. ) ;
#27303=CARTESIAN_POINT ( 'NONE',  ( -35.00000000000000000, 0.000000000000000000, 0.000000000000000000 ) ) ;
#27304=EDGE_LOOP ( 'NONE', ( #55202, #41540, #34484, #184 ) ) ;
#27308=EDGE_CURVE ( 'NONE', #35192, #42088, #37473, .T. ) ;
#27310=EDGE_CURVE ( 'NONE', #37124, #34795, #8156, .T. ) ;
#27311=ORIENTED_EDGE ( 'NONE', *, *, #15747, .F. ) ;
#27312=DIRECTION ( 'NONE',  ( 0.000000000000000000, -0.01356324068817992175, 0.9999080150203990547 ) ) ;
#27316=ORIENTED_EDGE ( 'NONE', *, *, #54291, .F. ) ;
#27317=ORIENTED_EDGE ( 'NONE', *, *, #18122, .T. ) ;
#27319=EDGE_CURVE ( 'NONE', #57915, #50989, #2200, .T. ) ;
#27320=CARTESIAN_POINT ( 'NONE',  ( 35.00000000000000000, -12.18632975068352664, -0.06441628369832411161 ) ) ;
#27322=EDGE_CURVE ( 'NONE', #51686, #15952, #12812, .T. ) ;
#27324=B_SPLINE_CURVE_WITH_KNOTS ( 'NONE', 3,
 ( #44270, #10245, #60460, #30523, #45835, #59255, #50828, #20571, #50510, #40851, #9930, #25216, #54272, #31201, #56124, #10566, #49303, #3751, #40169, #62747 ),
 .UNSPECIFIED., .F., .F.,
 ( 4, 2, 2, 2, 2, 2, 2, 2, 2, 4 ),
 ( 0.000000000000000000, 0.001056023233319194161, 0.001584034849978791133, 0.002112046466638388322, 0.003168069699957580532, 0.003696081316617175986, 0.004224092933276770573, 0.005280116166595961481, 0.006336139399915151522, 0.008448185866553530737 ),
 .UNSPECIFIED. ) ;
#27329=EDGE_LOOP ( 'NONE', ( #8409, #2683, #8625, #16030 ) ) ;
#27330=CARTESIAN_POINT ( 'NONE',  ( 37.00000000000000711, -11.68758509253247091, 1.171570255487570655 ) ) ;
#27333=DIRECTION ( 'NONE',  ( -1.000000000000000000, 0.000000000000000000, 0.000000000000000000 ) ) ;
#27334=CARTESIAN_POINT ( 'NONE',  ( -35.00000000000000000, 10.80478261802190154, -5.636262487437199376 ) ) ;
#27335=ADVANCED_FACE ( 'NONE', ( #23724 ), #23377, .T. ) ;
#27336=CARTESIAN_POINT ( 'NONE',  ( 3.291290029914074378, 8.250315036047103590, 10.68561190601527855 ) ) ;
#27338=DIRECTION ( 'NONE',  ( 0.000000000000000000, 0.01356324068817991828, -0.9999080150203990547 ) ) ;
#27339=DIRECTION ( 'NONE',  ( -1.000000000000000000, -0.000000000000000000, 0.000000000000000000 ) ) ;
#27341=AXIS2_PLACEMENT_3D ( 'NONE', #51936, #6378, #46939 ) ;
#27342=ORIENTED_EDGE ( 'NONE', *, *, #64378, .T. ) ;
#27344=DIRECTION ( 'NONE',  ( 0.000000000000000000, -0.01356324068817992175, 0.9999080150203990547 ) ) ;
#27345=CIRCLE ( 'NONE', #18871, 12.18649999999999878 ) ;
#27348=DIRECTION ( 'NONE',  ( 0.000000000000000000, 0.01356324068817998940, -0.9999080150203990547 ) ) ;
#27349=ORIENTED_EDGE ( 'NONE', *, *, #27240, .T. ) ;
#27350=CARTESIAN_POINT ( 'NONE',  ( 36.00000000000000711, -0.6593684648219547695, 12.73293890771483561 ) ) ;
#27352=DIRECTION ( 'NONE',  ( 0.2180658516479614395, -0.9759340573753174652, 0.000000000000000000 ) ) ;
#27354=VECTOR ( 'NONE', #57685, 1000.000000000000000 ) ;
#27356=DIRECTION ( 'NONE',  ( -1.000000000000000000, -1.836970198721029688E-16, 0.000000000000000000 ) ) ;
#27357=EDGE_CURVE ( 'NONE', #61328, #26747, #58509, .T. ) ;
#27360=CARTESIAN_POINT ( 'NONE',  ( -35.00000000000000000, 0.000000000000000000, 0.000000000000000000 ) ) ;
#27361=CYLINDRICAL_SURFACE ( 'NONE', #8121, 13.50000000000000178 ) ;
#27362=CARTESIAN_POINT ( 'NONE',  ( 37.00000000000000711, -3.614449339633571512, -11.17622378668005290 ) ) ;
#27363=CYLINDRICAL_SURFACE ( 'NONE', #56655, 4.785769192180104881 ) ;
#27364=VERTEX_POINT ( 'NONE', #49336 ) ;
#27369=CARTESIAN_POINT ( 'NONE',  ( -24.30804329714943535, 8.222810952426842235, 8.742709031936243491 ) ) ;
#27370=VERTEX_POINT ( 'NONE', #24347 ) ;
#27371=CARTESIAN_POINT ( 'NONE',  ( 35.00000000000000000, -7.215058775251181444, 9.821084925794645315 ) ) ;
#27373=DIRECTION ( 'NONE',  ( 0.000000000000000000, 0.6478160128811948359, -0.7617968321374878338 ) ) ;
#27374=EDGE_CURVE ( 'NONE', #35285, #57971, #8546, .T. ) ;
#27376=DIRECTION ( 'NONE',  ( 0.000000000000000000, 0.01356324068817992522, -0.9999080150203990547 ) ) ;
#27379=VERTEX_POINT ( 'NONE', #44300 ) ;
#27380=DIRECTION ( 'NONE',  ( 0.000000000000000000, 0.01356324068817991828, -0.9999080150203990547 ) ) ;
#27383=CARTESIAN_POINT ( 'NONE',  ( 12.96254931691228940, 11.37456213158350060, -7.274141147047163081 ) ) ;
#27388=ORIENTED_EDGE ( 'NONE', *, *, #13403, .T. ) ;
#27391=CARTESIAN_POINT ( 'NONE',  ( -37.00000000000000711, -9.063649021439015740, 8.146229107149364879 ) ) ;
#27392=CARTESIAN_POINT ( 'NONE',  ( -17.72422596690857688, -11.73861005525308343, 2.575547964227135278 ) ) ;
#27394=CYLINDRICAL_SURFACE ( 'NONE', #50113, 12.75000000000000178 ) ;
#27395=CARTESIAN_POINT ( 'NONE',  ( 47.00000000000000711, 4.705694406421931860E-17, -3.469127814946512892E-15 ) ) ;
#27396=AXIS2_PLACEMENT_3D ( 'NONE', #14296, #60504, #50554 ) ;
#27397=LINE ( 'NONE', #37717, #38416 ) ;
#27399=AXIS2_PLACEMENT_3D ( 'NONE', #27330, #12361, #32963 ) ;
#27400=ORIENTED_EDGE ( 'NONE', *, *, #33411, .T. ) ;
#27401=LINE ( 'NONE', #2143, #28177 ) ;
#27404=CIRCLE ( 'NONE', #41218, 12.75000000000000178 ) ;
#27405=EDGE_CURVE ( 'NONE', #39189, #12727, #39969, .T. ) ;
#27407=CARTESIAN_POINT ( 'NONE',  ( -27.19357181888462094, 12.48377454417557253, 5.138615876886901468 ) ) ;
#27409=FACE_OUTER_BOUND ( 'NONE', #1122, .T. ) ;
#27412=CARTESIAN_POINT ( 'NONE',  ( 9.373266352144048241, 2.643534358090585457, -11.70720285747480460 ) ) ;
#27413=ORIENTED_EDGE ( 'NONE', *, *, #12459, .T. ) ;
#27414=DIRECTION ( 'NONE',  ( 0.000000000000000000, 0.1387779952735747335, -0.9903235168508560671 ) ) ;
#27415=FACE_OUTER_BOUND ( 'NONE', #13541, .T. ) ;
#27416=DIRECTION ( 'NONE',  ( 0.000000000000000000, 0.01356324068817998940, -0.9999080150203990547 ) ) ;
#27418=CARTESIAN_POINT ( 'NONE',  ( 32.00000000000000000, 12.00000000000000000, 1.469576158976823553E-15 ) ) ;
#27419=FACE_OUTER_BOUND ( 'NONE', #27861, .T. ) ;
#27420=EDGE_LOOP ( 'NONE', ( #3088, #19304, #46431, #28055 ) ) ;
#27421=AXIS2_PLACEMENT_3D ( 'NONE', #23477, #44387, #3553 ) ;
#27422=CARTESIAN_POINT ( 'NONE',  ( -37.00000000000000711, 9.060822531526156354, -7.474872387600913548 ) ) ;
#27423=CARTESIAN_POINT ( 'NONE',  ( -27.01437459610461644, -10.69338818478079922, -8.240233560378637634 ) ) ;
#27428=CARTESIAN_POINT ( 'NONE',  ( -36.00000000000000711, 4.400442035671114027, -11.96656215839364457 ) ) ;
#27431=CARTESIAN_POINT ( 'NONE',  ( 36.00000000000000711, 3.033604067594577902, -12.38385022362083454 ) ) ;
#27432=EDGE_CURVE ( 'NONE', #49077, #10832, #9367, .T. ) ;
#27433=CARTESIAN_POINT ( 'NONE',  ( 35.00000000000000000, 9.348667969174517367, 7.817492529713752525 ) ) ;
#27437=CARTESIAN_POINT ( 'NONE',  ( 35.00000000000000000, -9.512294188640847636, 6.891188680298922620 ) ) ;
#27441=CARTESIAN_POINT ( 'NONE',  ( -9.829859729628957155, 10.62238046397816582, -5.599206581597568899 ) ) ;
#27444=VERTEX_POINT ( 'NONE', #31546 ) ;
#27449=VERTEX_POINT ( 'NONE', #22224 ) ;
#27451=CIRCLE ( 'NONE', #36987, 12.74999999999999822 ) ;
#27452=CARTESIAN_POINT ( 'NONE',  ( -35.00000000000000000, 11.37311665002359540, 2.936739658820077370 ) ) ;
#27454=DIRECTION ( 'NONE',  ( -1.000000000000000000, 0.000000000000000000, -0.000000000000000000 ) ) ;
#27455=CARTESIAN_POINT ( 'NONE',  ( 36.00000000000000711, 5.300372733891643762, -11.59605747147788790 ) ) ;
#27457=ORIENTED_EDGE ( 'NONE', *, *, #17642, .F. ) ;
#27458=CARTESIAN_POINT ( 'NONE',  ( -24.29708947709745104, -8.221392171298289142, 8.752766005952057782 ) ) ;
#27459=LINE ( 'NONE', #2883, #11724 ) ;
#27461=ORIENTED_EDGE ( 'NONE', *, *, #50558, .F. ) ;
#27466=CARTESIAN_POINT ( 'NONE',  ( -10.90165637463001680, -7.936842980705543837, 9.017060805754692154 ) ) ;
#27467=CARTESIAN_POINT ( 'NONE',  ( -35.00000000000000000, -7.376655759824951808, 9.700295462048636352 ) ) ;
#27472=AXIS2_PLACEMENT_3D ( 'NONE', #34603, #8052, #4037 ) ;
#27475=DIRECTION ( 'NONE',  ( -0.000000000000000000, -0.000000000000000000, -1.000000000000000000 ) ) ;
#27477=VERTEX_POINT ( 'NONE', #50304 ) ;
#27481=CYLINDRICAL_SURFACE ( 'NONE', #9634, 5.000000000000000888 ) ;
#27482=ADVANCED_FACE ( 'NONE', ( #11277 ), #46848, .T. ) ;
#27485=ORIENTED_EDGE ( 'NONE', *, *, #18034, .F. ) ;
#27487=EDGE_CURVE ( 'NONE', #56112, #19566, #20277, .T. ) ;
#27488=AXIS2_PLACEMENT_3D ( 'NONE', #1364, #10330, #61522 ) ;
#27489=VERTEX_POINT ( 'NONE', #1313 ) ;
#27490=DIRECTION ( 'NONE',  ( -1.000000000000000000, 0.000000000000000000, 0.000000000000000000 ) ) ;
#27491=CARTESIAN_POINT ( 'NONE',  ( 36.00000000000000711, -6.711949091238069265, 10.84030624090613237 ) ) ;
#27492=AXIS2_PLACEMENT_3D ( 'NONE', #598, #11528, #30814 ) ;
#27493=EDGE_CURVE ( 'NONE', #50042, #58893, #19239, .T. ) ;
#27496=ORIENTED_EDGE ( 'NONE', *, *, #63483, .F. ) ;
#27500=AXIS2_PLACEMENT_3D ( 'NONE', #25444, #30110, #9474 ) ;
#27502=DIRECTION ( 'NONE',  ( 1.000000000000000000, 0.000000000000000000, -0.000000000000000000 ) ) ;
#27505=CARTESIAN_POINT ( 'NONE',  ( 35.00000000000000000, 11.35427606708806003, -4.426194442447284771 ) ) ;
#27506=ORIENTED_EDGE ( 'NONE', *, *, #59935, .T. ) ;
#27507=CARTESIAN_POINT ( 'NONE',  ( -37.00000000000000711, -8.551552972817024312, -8.052525312709976291 ) ) ;
#27510=FACE_OUTER_BOUND ( 'NONE', #31379, .T. ) ;
#27512=VECTOR ( 'NONE', #60131, 1000.000000000000000 ) ;
#27513=EDGE_LOOP ( 'NONE', ( #32045, #30508, #42657, #60143 ) ) ;
#27514=EDGE_LOOP ( 'NONE', ( #58099, #32818, #2092, #54794, #61015, #30485 ) ) ;
#27516=ORIENTED_EDGE ( 'NONE', *, *, #56579, .F. ) ;
#27517=ADVANCED_FACE ( 'NONE', ( #31861 ), #6295, .T. ) ;
#27518=CARTESIAN_POINT ( 'NONE',  ( 3.460083169609886156, 6.940591624561522011, 9.798413085330784256 ) ) ;
#27519=DIRECTION ( 'NONE',  ( -1.000000000000000000, 0.000000000000000000, 0.000000000000000000 ) ) ;
#27520=DIRECTION ( 'NONE',  ( 1.000000000000000000, 0.000000000000000000, -0.000000000000000000 ) ) ;
#27522=AXIS2_PLACEMENT_3D ( 'NONE', #16687, #37292, #52290 ) ;
#27523=LINE ( 'NONE', #41499, #20499 ) ;
#27527=ORIENTED_EDGE ( 'NONE', *, *, #24522, .T. ) ;
#27528=VERTEX_POINT ( 'NONE', #11591 ) ;
#27532=LINE ( 'NONE', #21235, #50391 ) ;
#27533=AXIS2_PLACEMENT_3D ( 'NONE', #40780, #31758, #21132 ) ;
#27534=CARTESIAN_POINT ( 'NONE',  ( 17.00164331164202736, 11.45151090621293122, 7.188808658307459076 ) ) ;
#27536=DIRECTION ( 'NONE',  ( 1.000000000000000000, 0.000000000000000000, -0.000000000000000000 ) ) ;
#27538=VERTEX_POINT ( 'NONE', #21912 ) ;
#27539=CARTESIAN_POINT ( 'NONE',  ( 24.82652845881425208, 25.00000000000000000, -8.578654028722157321 ) ) ;
#27542=ORIENTED_EDGE ( 'NONE', *, *, #14689, .T. ) ;
#27544=DIRECTION ( 'NONE',  ( -0.000000000000000000, -0.000000000000000000, -1.000000000000000000 ) ) ;
#27545=ORIENTED_EDGE ( 'NONE', *, *, #35585, .T. ) ;
#27546=ADVANCED_FACE ( 'NONE', ( #62449 ), #42831, .T. ) ;
#27547=VERTEX_POINT ( 'NONE', #43823 ) ;
#27549=VERTEX_POINT ( 'NONE', #59135 ) ;
#27550=VECTOR ( 'NONE', #60837, 1000.000000000000000 ) ;
#27551=EDGE_LOOP ( 'NONE', ( #47513, #11864, #55351, #27995 ) ) ;
#27552=DIRECTION ( 'NONE',  ( 1.000000000000000000, 0.000000000000000000, 0.000000000000000000 ) ) ;
#27555=FACE_OUTER_BOUND ( 'NONE', #53671, .T. ) ;
#27557=LINE ( 'NONE', #63140, #30238 ) ;
#27558=VECTOR ( 'NONE', #25276, 1000.000000000000000 ) ;
#27562=CARTESIAN_POINT ( 'NONE',  ( -36.00000000000000711, 2.250029553613936528, -12.54989509947648685 ) ) ;
#27566=DIRECTION ( 'NONE',  ( 1.000000000000000000, 0.000000000000000000, 0.000000000000000000 ) ) ;
#27567=CARTESIAN_POINT ( 'NONE',  ( -37.00000000000000711, 11.59605747147786836, 5.300372733891681953 ) ) ;
#27568=EDGE_CURVE ( 'NONE', #56972, #31853, #33829, .T. ) ;
#27569=AXIS2_PLACEMENT_3D ( 'NONE', #15866, #41467, #51807 ) ;
#27573=ORIENTED_EDGE ( 'NONE', *, *, #45736, .T. ) ;
#27577=LINE ( 'NONE', #41895, #64877 ) ;
#27579=ORIENTED_EDGE ( 'NONE', *, *, #35490, .F. ) ;
#27580=DIRECTION ( 'NONE',  ( 1.000000000000000000, 0.000000000000000000, 0.000000000000000000 ) ) ;
#27583=CARTESIAN_POINT ( 'NONE',  ( -2.952869152607107139, 12.96714474214482138, 3.755417052241487585 ) ) ;
#27584=EDGE_CURVE ( 'NONE', #65451, #33526, #23215, .T. ) ;
#27585=AXIS2_PLACEMENT_3D ( 'NONE', #9945, #30227, #18945 ) ;
#27590=CIRCLE ( 'NONE', #18071, 12.75000000000000178 ) ;
#27591=ORIENTED_EDGE ( 'NONE', *, *, #7516, .F. ) ;
#27592=DIRECTION ( 'NONE',  ( 1.000000000000000000, 0.000000000000000000, 0.000000000000000000 ) ) ;
#27595=CARTESIAN_POINT ( 'NONE',  ( 26.34661844826604593, -13.08594712317289321, 3.317828791472332117 ) ) ;
#27596=CARTESIAN_POINT ( 'NONE',  ( -35.00000000000000000, -11.44858830469742017, 2.627174906296871448 ) ) ;
#27597=DIRECTION ( 'NONE',  ( 1.000000000000000000, 0.000000000000000000, 0.000000000000000000 ) ) ;
#27598=DIRECTION ( 'NONE',  ( -1.000000000000000000, 0.000000000000000000, 0.000000000000000000 ) ) ;
#27600=EDGE_CURVE ( 'NONE', #60515, #32661, #26686, .T. ) ;
#27602=ORIENTED_EDGE ( 'NONE', *, *, #16913, .F. ) ;
#27603=ORIENTED_EDGE ( 'NONE', *, *, #23547, .F. ) ;
#27607=CIRCLE ( 'NONE', #64764, 12.18650000000000055 ) ;
#27609=VERTEX_POINT ( 'NONE', #53148 ) ;
#27611=CARTESIAN_POINT ( 'NONE',  ( -37.00000000000000711, -10.75351884295731253, 4.725891942574718563 ) ) ;
#27612=VERTEX_POINT ( 'NONE', #7595 ) ;
#27613=CARTESIAN_POINT ( 'NONE',  ( -35.00000000000000000, 11.98254675519231682, -2.220215194441768514 ) ) ;
#27616=ORIENTED_EDGE ( 'NONE', *, *, #41255, .T. ) ;
#27619=VERTEX_POINT ( 'NONE', #43475 ) ;
#27621=CARTESIAN_POINT ( 'NONE',  ( -18.63153057747156893, 11.99999999999999822, -0.3572518721000119690 ) ) ;
#27622=VERTEX_POINT ( 'NONE', #22902 ) ;
#27624=AXIS2_PLACEMENT_3D ( 'NONE', #33174, #27209, #2280 ) ;
#27626=DIRECTION ( 'NONE',  ( 0.000000000000000000, -0.01356324068817998940, 0.9999080150203990547 ) ) ;
#27630=CARTESIAN_POINT ( 'NONE',  ( -35.00000000000000000, 0.000000000000000000, 0.000000000000000000 ) ) ;
#27631=VERTEX_POINT ( 'NONE', #3275 ) ;
#27632=VECTOR ( 'NONE', #27201, 1000.000000000000000 ) ;
#27634=ORIENTED_EDGE ( 'NONE', *, *, #52766, .T. ) ;
#27636=DIRECTION ( 'NONE',  ( 1.000000000000000000, 0.000000000000000000, 0.000000000000000000 ) ) ;
#27637=ORIENTED_EDGE ( 'NONE', *, *, #45519, .F. ) ;
#27638=CARTESIAN_POINT ( 'NONE',  ( -17.18936361399038404, 7.855595644171634362, 9.071939927147207428 ) ) ;
#27639=CARTESIAN_POINT ( 'NONE',  ( -35.00000000000000000, 10.39746860227890579, 7.379373053628905943 ) ) ;
#27641=LINE ( 'NONE', #43939, #38665 ) ;
#27642=VERTEX_POINT ( 'NONE', #43155 ) ;
#27644=DIRECTION ( 'NONE',  ( -0.000000000000000000, -1.000000000000000000, -0.000000000000000000 ) ) ;
#27645=AXIS2_PLACEMENT_3D ( 'NONE', #45446, #24515, #50779 ) ;
#27646=EDGE_LOOP ( 'NONE', ( #24712, #59411, #52954, #54730 ) ) ;
#27647=CARTESIAN_POINT ( 'NONE',  ( -37.00000000000000711, -0.1652884326465054177, 12.18537902504609072 ) ) ;
#27649=CARTESIAN_POINT ( 'NONE',  ( -3.496946155113953569, -10.55788327300660079, 8.446084379147929866 ) ) ;
#27650=AXIS2_PLACEMENT_3D ( 'NONE', #4824, #45041, #15737 ) ;
#27651=CARTESIAN_POINT ( 'NONE',  ( -37.00000000000000711, 11.61976888909158490, 3.827969819614504221 ) ) ;
#27654=EDGE_CURVE ( 'NONE', #63728, #29225, #63754, .T. ) ;
#27657=CARTESIAN_POINT ( 'NONE',  ( 35.00000000000000000, -2.346765782874354667, 11.95840593935203522 ) ) ;
#27658=DIRECTION ( 'NONE',  ( -0.000000000000000000, -0.000000000000000000, -1.000000000000000000 ) ) ;
#27660=DIRECTION ( 'NONE',  ( 0.000000000000000000, 0.01356324068817992175, -0.9999080150203990547 ) ) ;
#27662=CARTESIAN_POINT ( 'NONE',  ( -35.00000000000000000, 1.262958560998759472, 12.12087942037210198 ) ) ;
#27664=EDGE_CURVE ( 'NONE', #16920, #3974, #14938, .T. ) ;
#27665=ORIENTED_EDGE ( 'NONE', *, *, #36555, .T. ) ;
#27667=DIRECTION ( 'NONE',  ( 0.000000000000000000, -0.01356324068817998940, 0.9999080150203990547 ) ) ;
#27669=AXIS2_PLACEMENT_3D ( 'NONE', #4086, #25337, #10362 ) ;
#27674=ORIENTED_EDGE ( 'NONE', *, *, #9270, .T. ) ;
#27675=VECTOR ( 'NONE', #34820, 1000.000000000000000 ) ;
#27676=UNCERTAINTY_MEASURE_WITH_UNIT (LENGTH_MEASURE( 1.000000000000000082E-05 ), #5383, 'distance_accuracy_value', 'NONE');
#27677=CARTESIAN_POINT ( 'NONE',  ( -35.00000000000000000, -9.348667969174350389, -7.817492529713957694 ) ) ;
#27681=CARTESIAN_POINT ( 'NONE',  ( -35.00000000000000000, 5.636262487437317503, 10.80478261802183937 ) ) ;
#27682=ORIENTED_EDGE ( 'NONE', *, *, #36009, .F. ) ;
#27683=VERTEX_POINT ( 'NONE', #4585 ) ;
#27685=EDGE_CURVE ( 'NONE', #39732, #54691, #14926, .T. ) ;
#27686=VERTEX_POINT ( 'NONE', #39811 ) ;
#27687=CARTESIAN_POINT ( 'NONE',  ( -24.97754535057679348, -7.227978708121235663, 9.585722579478227701 ) ) ;
#27688=CARTESIAN_POINT ( 'NONE',  ( 145.1370849898475797, 3.309064568108273190E-14, 0.000000000000000000 ) ) ;
#27689=CARTESIAN_POINT ( 'NONE',  ( 35.00000000000000000, 4.705694406421931860E-17, -3.469127814946512892E-15 ) ) ;
#27690=CIRCLE ( 'NONE', #43640, 12.74999999999999822 ) ;
#27691=CYLINDRICAL_SURFACE ( 'NONE', #46014, 12.75000000000000178 ) ;
#27692=ORIENTED_EDGE ( 'NONE', *, *, #54524, .F. ) ;
#27694=ADVANCED_FACE ( 'NONE', ( #29493 ), #4910, .T. ) ;
#27696=CARTESIAN_POINT ( 'NONE',  ( 37.00000000000000711, 3.614449339633649227, 11.17622378668002092 ) ) ;
#27697=CARTESIAN_POINT ( 'NONE',  ( -37.00000000000000711, 12.49688848680888142, -2.527899948230500460 ) ) ;
#27698=ORIENTED_EDGE ( 'NONE', *, *, #46318, .F. ) ;
#27700=CIRCLE ( 'NONE', #36185, 5.000000000000000000 ) ;
#27701=ORIENTED_EDGE ( 'NONE', *, *, #14727, .T. ) ;
#27702=CARTESIAN_POINT ( 'NONE',  ( -35.00000000000000000, 0.000000000000000000, 0.000000000000000000 ) ) ;
#27703=VERTEX_POINT ( 'NONE', #59440 ) ;
#27705=CARTESIAN_POINT ( 'NONE',  ( -29.68541646480311869, -1.416020129149132334, -13.42553116244736877 ) ) ;
#27707=CARTESIAN_POINT ( 'NONE',  ( -35.00000000000000000, 1.457575200925722125, -12.66641127287624258 ) ) ;
#27708=VECTOR ( 'NONE', #37088, 1000.000000000000000 ) ;
#27710=DIRECTION ( 'NONE',  ( -1.000000000000000000, 0.000000000000000000, -0.000000000000000000 ) ) ;
#27712=ORIENTED_EDGE ( 'NONE', *, *, #31828, .T. ) ;
#27714=VECTOR ( 'NONE', #37040, 1000.000000000000000 ) ;
#27716=VERTEX_POINT ( 'NONE', #60098 ) ;
#27717=ADVANCED_FACE ( 'NONE', ( #45133 ), #15191, .T. ) ;
#27720=DIRECTION ( 'NONE',  ( -1.000000000000000000, 0.000000000000000000, 0.000000000000000000 ) ) ;
#27721=DIRECTION ( 'NONE',  ( 0.000000000000000000, -1.000000000000000000, 0.000000000000000000 ) ) ;
#27724=CARTESIAN_POINT ( 'NONE',  ( 36.00000000000000711, 7.379373053628869528, -10.39746860227893421 ) ) ;
#27725=CIRCLE ( 'NONE', #7548, 5.000000000000000000 ) ;
#27726=AXIS2_PLACEMENT_3D ( 'NONE', #54887, #4356, #24626 ) ;
#27728=CARTESIAN_POINT ( 'NONE',  ( 35.00000000000000000, -7.817492529713787164, 9.348667969174485393 ) ) ;
#27729=AXIS2_PLACEMENT_3D ( 'NONE', #12601, #46558, #31582 ) ;
#27731=ORIENTED_EDGE ( 'NONE', *, *, #34116, .F. ) ;
#27732=VECTOR ( 'NONE', #14283, 1000.000000000000000 ) ;
#27733=DIRECTION ( 'NONE',  ( 1.000000000000000000, -0.000000000000000000, -0.000000000000000000 ) ) ;
#27734=CARTESIAN_POINT ( 'NONE',  ( 37.00000000000000711, 3.213188559034240832, -11.29812557209478285 ) ) ;
#27735=AXIS2_PLACEMENT_3D ( 'NONE', #30178, #9227, #44470 ) ;
#27736=EDGE_CURVE ( 'NONE', #64793, #12206, #45759, .T. ) ;
#27739=LINE ( 'NONE', #1520, #13056 ) ;
#27740=AXIS2_PLACEMENT_3D ( 'NONE', #15525, #50144, #15840 ) ;
#27743=CIRCLE ( 'NONE', #1235, 5.000000000000000000 ) ;
#27744=ORIENTED_EDGE ( 'NONE', *, *, #25890, .F. ) ;
#27747=DIRECTION ( 'NONE',  ( -1.000000000000000000, 0.000000000000000000, 0.000000000000000000 ) ) ;
#27748=ADVANCED_FACE ( 'NONE', ( #14514 ), #13863, .T. ) ;
#27751=AXIS2_PLACEMENT_3D ( 'NONE', #20883, #43958, #46176 ) ;
#27752=ADVANCED_FACE ( 'NONE', ( #10201 ), #45444, .T. ) ;
#27754=CARTESIAN_POINT ( 'NONE',  ( -47.00000000000000711, 0.000000000000000000, 0.000000000000000000 ) ) ;
#27755=( BOUNDED_CURVE ( )  B_SPLINE_CURVE ( 3, ( #48223, #2672, #38537, #58508 ),
 .UNSPECIFIED., .F., .F. ) 
 B_SPLINE_CURVE_WITH_KNOTS ( ( 4, 4 ),
 ( 0.8924480861843639978, 0.9142464078881809009 ),
 .UNSPECIFIED. ) 
 CURVE ( )  GEOMETRIC_REPRESENTATION_ITEM ( )  RATIONAL_B_SPLINE_CURVE ( ( 1.000000000000000000, 0.9999604031562251416, 0.9999604031562251416, 1.000000000000000000 ) ) 
 REPRESENTATION_ITEM ( '' )  );
#27757=CARTESIAN_POINT ( 'NONE',  ( 17.92615217306980568, -8.262653472663041399, 8.714354160369650160 ) ) ;
#27758=CARTESIAN_POINT ( 'NONE',  ( -35.00000000000000000, -7.971186206369537786, 9.217970097227697224 ) ) ;
#27761=EDGE_LOOP ( 'NONE', ( #12254, #23666, #61887, #18238 ) ) ;
#27766=EDGE_LOOP ( 'NONE', ( #12788, #5662, #49155, #25593 ) ) ;
#27767=LINE ( 'NONE', #7155, #39472 ) ;
#27768=CIRCLE ( 'NONE', #19288, 5.000000000000000888 ) ;
#27771=AXIS2_PLACEMENT_3D ( 'NONE', #14796, #15475, #29451 ) ;
#27772=CARTESIAN_POINT ( 'NONE',  ( -35.00000000000000000, 0.000000000000000000, 0.000000000000000000 ) ) ;
#27773=DIRECTION ( 'NONE',  ( -1.000000000000000000, -0.000000000000000000, 0.000000000000000000 ) ) ;
#27774=DIRECTION ( 'NONE',  ( 0.000000000000000000, 0.9847383929261610547, -0.1740410799127649344 ) ) ;
#27775=DIRECTION ( 'NONE',  ( 0.000000000000000000, -0.01356324068817998940, 0.9999080150203990547 ) ) ;
#27776=CARTESIAN_POINT ( 'NONE',  ( -27.74986723846695114, 10.95058365257675881, -4.916369140193016740 ) ) ;
#27777=EDGE_CURVE ( 'NONE', #12206, #26019, #65392, .T. ) ;
#27778=DIRECTION ( 'NONE',  ( 0.000000000000000000, -0.01356324068817992175, 0.9999080150203990547 ) ) ;
#27780=EDGE_LOOP ( 'NONE', ( #13783, #36779, #5771, #61820 ) ) ;
#27784=CARTESIAN_POINT ( 'NONE',  ( 24.90230333882989200, -0.3472681461867982988, -12.00162445426803437 ) ) ;
#27785=AXIS2_PLACEMENT_3D ( 'NONE', #55041, #18826, #24447 ) ;
#27789=CARTESIAN_POINT ( 'NONE',  ( -25.20868475945270504, 11.50518608263469922, 7.064184148472541835 ) ) ;
#27790=ADVANCED_FACE ( 'NONE', ( #35124 ), #9873, .T. ) ;
#27791=PLANE ( 'NONE',  #34229 ) ;
#27797=AXIS2_PLACEMENT_3D ( 'NONE', #27083, #47378, #17097 ) ;
#27798=CARTESIAN_POINT ( 'NONE',  ( 35.00000000000000000, -4.339012074899872395, 10.91536515067652324 ) ) ;
#27799=FACE_OUTER_BOUND ( 'NONE', #5909, .T. ) ;
#27800=CYLINDRICAL_SURFACE ( 'NONE', #25263, 4.999999999999999112 ) ;
#27801=ORIENTED_EDGE ( 'NONE', *, *, #1815, .F. ) ;
#27802=ORIENTED_EDGE ( 'NONE', *, *, #21963, .T. ) ;
#27803=ADVANCED_FACE ( 'NONE', ( #40453 ), #30793, .T. ) ;
#27804=CARTESIAN_POINT ( 'NONE',  ( -35.00000000000000000, 8.235637554476644695, 9.733281772932190989 ) ) ;
#27806=ORIENTED_EDGE ( 'NONE', *, *, #42771, .F. ) ;
#27807=LINE ( 'NONE', #48108, #3017 ) ;
#27809=LINE ( 'NONE', #48110, #33106 ) ;
#27811=VECTOR ( 'NONE', #15679, 1000.000000000000000 ) ;
#27815=DIRECTION ( 'NONE',  ( 1.000000000000000000, 0.000000000000000000, 0.000000000000000000 ) ) ;
#27817=DIRECTION ( 'NONE',  ( -1.000000000000000000, 0.000000000000000000, 0.000000000000000000 ) ) ;
#27818=ORIENTED_EDGE ( 'NONE', *, *, #41872, .T. ) ;
#27819=CARTESIAN_POINT ( 'NONE',  ( -37.00000000000000711, 0.000000000000000000, 0.000000000000000000 ) ) ;
#27820=CARTESIAN_POINT ( 'NONE',  ( 35.00000000000000000, -2.497432891016756251, 11.47758908105696740 ) ) ;
#27821=LINE ( 'NONE', #33131, #18036 ) ;
#27822=AXIS2_PLACEMENT_3D ( 'NONE', #3680, #44509, #40514 ) ;
#27823=ORIENTED_EDGE ( 'NONE', *, *, #57858, .T. ) ;
#27824=VECTOR ( 'NONE', #62754, 1000.000000000000000 ) ;
#27825=EDGE_CURVE ( 'NONE', #23170, #12670, #27725, .T. ) ;
#27826=ORIENTED_EDGE ( 'NONE', *, *, #39102, .F. ) ;
#27827=CYLINDRICAL_SURFACE ( 'NONE', #43957, 12.74999999999999822 ) ;
#27832=CIRCLE ( 'NONE', #53340, 12.18649999999999878 ) ;
#27834=CYLINDRICAL_SURFACE ( 'NONE', #55198, 12.18649999999999878 ) ;
#27835=VERTEX_POINT ( 'NONE', #31150 ) ;
#27837=CARTESIAN_POINT ( 'NONE',  ( 37.00000000000000711, 6.036400161834703404, 10.07641281632170838 ) ) ;
#27838=AXIS2_PLACEMENT_3D ( 'NONE', #50491, #45158, #19886 ) ;
#27839=EDGE_CURVE ( 'NONE', #56608, #5051, #577, .T. ) ;
#27840=CARTESIAN_POINT ( 'NONE',  ( -29.54910026239419807, 0.3010961243626856243, -13.50337375539546336 ) ) ;
#27843=AXIS2_PLACEMENT_3D ( 'NONE', #25952, #20937, #24373 ) ;
#27844=FACE_OUTER_BOUND ( 'NONE', #35399, .T. ) ;
#27845=ORIENTED_EDGE ( 'NONE', *, *, #51797, .F. ) ;
#27849=ORIENTED_EDGE ( 'NONE', *, *, #49069, .T. ) ;
#27850=CARTESIAN_POINT ( 'NONE',  ( -11.19197262092341738, -9.208027763853694481, -7.717244145212098339 ) ) ;
#27851=DIRECTION ( 'NONE',  ( -0.000000000000000000, -1.000000000000000000, -0.000000000000000000 ) ) ;
#27852=CARTESIAN_POINT ( 'NONE',  ( -37.00000000000000711, 6.891188680298823144, 9.512294188640927572 ) ) ;
#27853=EDGE_CURVE ( 'NONE', #65184, #9921, #33038, .T. ) ;
#27855=CARTESIAN_POINT ( 'NONE',  ( -29.25940519196071321, 2.962255644788923892, -13.17777891311915894 ) ) ;
#27860=VERTEX_POINT ( 'NONE', #15828 ) ;
#27861=EDGE_LOOP ( 'NONE', ( #37379, #32579, #50184, #25164 ) ) ;
#27864=CARTESIAN_POINT ( 'NONE',  ( 16.94760237393643720, -10.49682181221981025, 5.815268149447256008 ) ) ;
#27866=DIRECTION ( 'NONE',  ( 0.000000000000000000, 0.01356324068817992175, -0.9999080150203990547 ) ) ;
#27867=CARTESIAN_POINT ( 'NONE',  ( -35.00000000000000000, 6.891188680298823144, 9.512294188640927572 ) ) ;
#27868=DIRECTION ( 'NONE',  ( 0.000000000000000000, -0.2618041379715496664, 0.9651210252299831094 ) ) ;
#27869=DIRECTION ( 'NONE',  ( -0.000000000000000000, -0.000000000000000000, -1.000000000000000000 ) ) ;
#27870=CYLINDRICAL_SURFACE ( 'NONE', #40334, 5.000000000000000888 ) ;
#27871=ORIENTED_EDGE ( 'NONE', *, *, #9491, .T. ) ;
#27872=ORIENTED_EDGE ( 'NONE', *, *, #5028, .F. ) ;
#27876=EDGE_CURVE ( 'NONE', #29225, #28103, #56446, .T. ) ;
#27878=DIRECTION ( 'NONE',  ( 0.000000000000000000, 0.01356324068817992175, -0.9999080150203990547 ) ) ;
#27879=EDGE_CURVE ( 'NONE', #61666, #8847, #8651, .T. ) ;
#27882=LINE ( 'NONE', #31863, #15251 ) ;
#27883=AXIS2_PLACEMENT_3D ( 'NONE', #61545, #46282, #30965 ) ;
#27885=CARTESIAN_POINT ( 'NONE',  ( 37.00000000000000711, 11.47561260193577048, -5.556331110570448928 ) ) ;
#27886=ORIENTED_EDGE ( 'NONE', *, *, #21202, .T. ) ;
#27887=AXIS2_PLACEMENT_3D ( 'NONE', #53504, #33195, #22577 ) ;
#27889=EDGE_CURVE ( 'NONE', #33067, #29231, #21840, .T. ) ;
#27890=DIRECTION ( 'NONE',  ( 0.000000000000000000, 0.01356324068817991828, -0.9999080150203990547 ) ) ;
#27891=ORIENTED_EDGE ( 'NONE', *, *, #6068, .T. ) ;
#27892=FACE_OUTER_BOUND ( 'NONE', #40310, .T. ) ;
#27893=ORIENTED_EDGE ( 'NONE', *, *, #39857, .T. ) ;
#27894=VERTEX_POINT ( 'NONE', #26476 ) ;
#27896=DIRECTION ( 'NONE',  ( 0.000000000000000000, -0.9987865678893281807, 0.04924826701373505311 ) ) ;
#27899=DIRECTION ( 'NONE',  ( -1.000000000000000000, 0.000000000000000000, 0.000000000000000000 ) ) ;
#27900=EDGE_CURVE ( 'NONE', #9878, #17695, #18251, .T. ) ;
#27902=VERTEX_POINT ( 'NONE', #1567 ) ;
#27906=CARTESIAN_POINT ( 'NONE',  ( 37.00000000000000711, -4.986700593229777212, -10.63508530065520219 ) ) ;
#27907=AXIS2_PLACEMENT_3D ( 'NONE', #2520, #58358, #12778 ) ;
#27908=CARTESIAN_POINT ( 'NONE',  ( 26.08439714455133185, -11.40113243194250359, 3.743551691817327942 ) ) ;
#27911=CARTESIAN_POINT ( 'NONE',  ( 37.00000000000000711, 4.705694406421931860E-17, -3.469127814946512892E-15 ) ) ;
#27914=AXIS2_PLACEMENT_3D ( 'NONE', #25457, #35082, #44749 ) ;
#27915=CIRCLE ( 'NONE', #28958, 5.000000000000001776 ) ;
#27916=ORIENTED_EDGE ( 'NONE', *, *, #62463, .T. ) ;
#27919=EDGE_LOOP ( 'NONE', ( #60743, #18749, #32004, #2885 ) ) ;
#27922=CARTESIAN_POINT ( 'NONE',  ( 12.90005361535634520, -12.56318921256607801, -4.945239668744613404 ) ) ;
#27925=ORIENTED_EDGE ( 'NONE', *, *, #13089, .T. ) ;
#27928=DIRECTION ( 'NONE',  ( -1.000000000000000000, 0.000000000000000000, 0.000000000000000000 ) ) ;
#27938=ADVANCED_FACE ( 'NONE', ( #6540 ), #51459, .T. ) ;
#27940=CIRCLE ( 'NONE', #58770, 12.75000000000000178 ) ;
#27942=CYLINDRICAL_SURFACE ( 'NONE', #5290, 4.445031439545090279 ) ;
#27943=EDGE_LOOP ( 'NONE', ( #53914, #1151, #20911, #857 ) ) ;
#27944=CARTESIAN_POINT ( 'NONE',  ( -35.00000000000000000, -11.74226168163341022, -0.3025107581132430723 ) ) ;
#27946=CARTESIAN_POINT ( 'NONE',  ( 35.00000000000000000, 2.772148766916280316, 11.86701198550353098 ) ) ;
#27950=VECTOR ( 'NONE', #31925, 1000.000000000000000 ) ;
#27952=EDGE_LOOP ( 'NONE', ( #20983, #27134, #62778, #59435 ) ) ;
#27953=VERTEX_POINT ( 'NONE', #56774 ) ;
#27957=DIRECTION ( 'NONE',  ( -1.000000000000000000, 0.000000000000000000, 0.000000000000000000 ) ) ;
#27958=AXIS2_PLACEMENT_3D ( 'NONE', #6689, #31926, #1703 ) ;
#27960=CYLINDRICAL_SURFACE ( 'NONE', #54906, 13.50000000000000178 ) ;
#27963=( BOUNDED_CURVE ( )  B_SPLINE_CURVE ( 3, ( #27153, #12831, #48439, #17175 ),
 .UNSPECIFIED., .F., .F. ) 
 B_SPLINE_CURVE_WITH_KNOTS ( ( 4, 4 ),
 ( 3.747716794192935019, 3.763247559512395757 ),
 .UNSPECIFIED. ) 
 CURVE ( )  GEOMETRIC_REPRESENTATION_ITEM ( )  RATIONAL_B_SPLINE_CURVE ( ( 1.000000000000000000, 0.9999798997117221866, 0.9999798997117221866, 1.000000000000000000 ) ) 
 REPRESENTATION_ITEM ( '' )  );
#27966=LINE ( 'NONE', #13321, #23944 ) ;
#27967=ORIENTED_EDGE ( 'NONE', *, *, #26763, .F. ) ;
#27969=ORIENTED_EDGE ( 'NONE', *, *, #695, .T. ) ;
#27971=VERTEX_POINT ( 'NONE', #51771 ) ;
#27972=CARTESIAN_POINT ( 'NONE',  ( 8.817269919411085510, 2.645982468348137662, -13.24072998050336203 ) ) ;
#27973=ORIENTED_EDGE ( 'NONE', *, *, #42072, .F. ) ;
#27976=ADVANCED_FACE ( 'NONE', ( #46764 ), #36789, .T. ) ;
#27978=CARTESIAN_POINT ( 'NONE',  ( 35.00000000000000000, -11.38112321385048631, 2.905556151562744382 ) ) ;
#27979=LINE ( 'NONE', #43924, #19750 ) ;
#27980=CYLINDRICAL_SURFACE ( 'NONE', #30855, 12.75000000000000178 ) ;
#27982=CARTESIAN_POINT ( 'NONE',  ( -27.63886315033333574, -10.11438670753379299, -6.464158504329111210 ) ) ;
#27983=VERTEX_POINT ( 'NONE', #32756 ) ;
#27984=CARTESIAN_POINT ( 'NONE',  ( 35.00000000000000000, 6.475373545682446164, 10.32377448871660519 ) ) ;
#27985=CIRCLE ( 'NONE', #19487, 12.74999999999999822 ) ;
#27987=( BOUNDED_CURVE ( )  B_SPLINE_CURVE ( 3, ( #40258, #55236, #35607, #60545 ),
 .UNSPECIFIED., .F., .F. ) 
 B_SPLINE_CURVE_WITH_KNOTS ( ( 4, 4 ),
 ( 5.770121532352542104, 5.841648021086276898 ),
 .UNSPECIFIED. ) 
 CURVE ( )  GEOMETRIC_REPRESENTATION_ITEM ( )  RATIONAL_B_SPLINE_CURVE ( ( 1.000000000000000000, 0.9995737088895613187, 0.9995737088895613187, 1.000000000000000000 ) ) 
 REPRESENTATION_ITEM ( '' )  );
#27988=DIRECTION ( 'NONE',  ( -1.000000000000000000, 0.000000000000000000, 0.000000000000000000 ) ) ;
#27989=AXIS2_PLACEMENT_3D ( 'NONE', #43929, #63531, #33622 ) ;
#27990=DIRECTION ( 'NONE',  ( -1.000000000000000000, 0.000000000000000000, 0.000000000000000000 ) ) ;
#27991=ORIENTED_EDGE ( 'NONE', *, *, #22013, .F. ) ;
#27992=DIRECTION ( 'NONE',  ( -1.000000000000000000, 0.000000000000000000, 0.000000000000000000 ) ) ;
#27995=ORIENTED_EDGE ( 'NONE', *, *, #14697, .T. ) ;
#27996=AXIS2_PLACEMENT_3D ( 'NONE', #6630, #27221, #32840 ) ;
#27997=ORIENTED_EDGE ( 'NONE', *, *, #37919, .F. ) ;
#27999=EDGE_CURVE ( 'NONE', #665, #46663, #63678, .T. ) ;
#28000=ORIENTED_EDGE ( 'NONE', *, *, #37043, .T. ) ;
#28001=CARTESIAN_POINT ( 'NONE',  ( -35.00000000000000000, -3.614449339633411196, -11.17622378668010441 ) ) ;
#28003=EDGE_CURVE ( 'NONE', #47877, #33694, #36259, .T. ) ;
#28004=DIRECTION ( 'NONE',  ( -1.000000000000000000, -0.000000000000000000, 0.000000000000000000 ) ) ;
#28005=CARTESIAN_POINT ( 'NONE',  ( -18.81994070919206763, -4.785352002469239530, 11.00505384451766666 ) ) ;
#28008=AXIS2_PLACEMENT_3D ( 'NONE', #13084, #38688, #12735 ) ;
#28011=EDGE_CURVE ( 'NONE', #19607, #56863, #3200, .T. ) ;
#28014=CIRCLE ( 'NONE', #58849, 12.75000000000000178 ) ;
#28015=CARTESIAN_POINT ( 'NONE',  ( 22.11764649685935069, 13.40615838776775171, -1.629994490815044772 ) ) ;
#28016=CARTESIAN_POINT ( 'NONE',  ( -37.00000000000000711, -0.7008968033237865658, -12.16632754454237819 ) ) ;
#28018=EDGE_CURVE ( 'NONE', #40199, #29886, #23136, .T. ) ;
#28019=CARTESIAN_POINT ( 'NONE',  ( -37.00000000000000711, 0.000000000000000000, 0.000000000000000000 ) ) ;
#28021=CIRCLE ( 'NONE', #21664, 12.74999999999999822 ) ;
#28022=CIRCLE ( 'NONE', #7855, 14.99999999999998757 ) ;
#28026=DIRECTION ( 'NONE',  ( 1.000000000000000000, 0.000000000000000000, -0.000000000000000000 ) ) ;
#28029=AXIS2_PLACEMENT_3D ( 'NONE', #62387, #26830, #16845 ) ;
#28033=CARTESIAN_POINT ( 'NONE',  ( 35.00000000000000000, 2.968224442958566911, 11.81949347079743440 ) ) ;
#28034=VERTEX_POINT ( 'NONE', #2880 ) ;
#28035=EDGE_LOOP ( 'NONE', ( #47445, #40619, #40270, #21309 ) ) ;
#28036=CARTESIAN_POINT ( 'NONE',  ( -36.00000000000000711, 12.16893194857550142, 3.805206332242516254 ) ) ;
#28041=LINE ( 'NONE', #23371, #51439 ) ;
#28042=CARTESIAN_POINT ( 'NONE',  ( 18.82686498295705135, 4.840479739905770629, 10.99031994906281540 ) ) ;
#28043=ORIENTED_EDGE ( 'NONE', *, *, #26864, .F. ) ;
#28044=DIRECTION ( 'NONE',  ( -1.000000000000000000, 0.000000000000000000, -0.000000000000000000 ) ) ;
#28047=CARTESIAN_POINT ( 'NONE',  ( -24.61176285888814519, 9.685806582847478197, 7.097305586750869644 ) ) ;
#28050=ORIENTED_EDGE ( 'NONE', *, *, #13151, .F. ) ;
#28052=DIRECTION ( 'NONE',  ( -1.000000000000000000, 0.000000000000000000, 0.000000000000000000 ) ) ;
#28053=EDGE_CURVE ( 'NONE', #29988, #13694, #64930, .T. ) ;
#28054=AXIS2_PLACEMENT_3D ( 'NONE', #27507, #61778, #56472 ) ;
#28055=ORIENTED_EDGE ( 'NONE', *, *, #26424, .T. ) ;
#28057=FACE_OUTER_BOUND ( 'NONE', #28203, .T. ) ;
#28058=CARTESIAN_POINT ( 'NONE',  ( -35.00000000000000000, 0.000000000000000000, 0.000000000000000000 ) ) ;
#28059=AXIS2_PLACEMENT_3D ( 'NONE', #54918, #44281, #9345 ) ;
#28061=EDGE_CURVE ( 'NONE', #14288, #41167, #58068, .T. ) ;
#28063=CARTESIAN_POINT ( 'NONE',  ( -17.54726996257253191, 11.36053454945672847, 3.865003848717349033 ) ) ;
#28064=CARTESIAN_POINT ( 'NONE',  ( 36.00000000000000711, -9.390600770288051180, -8.624332853796024878 ) ) ;
#28071=LINE ( 'NONE', #7432, #44297 ) ;
#28072=DIRECTION ( 'NONE',  ( 1.000000000000000000, 0.000000000000000000, 0.000000000000000000 ) ) ;
#28074=DIRECTION ( 'NONE',  ( 0.000000000000000000, 0.01356324068817998940, -0.9999080150203990547 ) ) ;
#28075=CIRCLE ( 'NONE', #43963, 5.000000000000000888 ) ;
#28080=EDGE_CURVE ( 'NONE', #12197, #42153, #38764, .T. ) ;
#28081=ORIENTED_EDGE ( 'NONE', *, *, #14318, .T. ) ;
#28082=CIRCLE ( 'NONE', #55707, 4.999999999999998224 ) ;
#28085=EDGE_CURVE ( 'NONE', #1795, #56510, #35331, .T. ) ;
#28086=CARTESIAN_POINT ( 'NONE',  ( -17.18002655544815838, -8.043634770698369962, 10.84711994095657950 ) ) ;
#28088=EDGE_CURVE ( 'NONE', #46364, #7895, #52194, .T. ) ;
#28090=CARTESIAN_POINT ( 'NONE',  ( -34.00000000000000000, 15.00000000000000000, 1.836970198721029589E-15 ) ) ;
#28091=EDGE_CURVE ( 'NONE', #52020, #31676, #63893, .T. ) ;
#28092=CARTESIAN_POINT ( 'NONE',  ( -35.00000000000000000, 11.35427606708812753, -4.426194442447117794 ) ) ;
#28094=CARTESIAN_POINT ( 'NONE',  ( 37.00000000000000711, -5.273331777780263074, 10.49591321039685887 ) ) ;
#28095=CIRCLE ( 'NONE', #62078, 12.75000000000000178 ) ;
#28096=CARTESIAN_POINT ( 'NONE',  ( -35.00000000000000000, 0.3137578094509240190, 12.74613886779085092 ) ) ;
#28097=CYLINDRICAL_SURFACE ( 'NONE', #52409, 4.999999999999999112 ) ;
#28098=VECTOR ( 'NONE', #22876, 1000.000000000000000 ) ;
#28099=B_SPLINE_CURVE_WITH_KNOTS ( 'NONE', 3,
 ( #56743, #57053, #52720, #7147, #26133, #22113, #62342, #62660, #41079, #62037, #56383, #27423 ),
 .UNSPECIFIED., .F., .F.,
 ( 4, 2, 2, 2, 2, 4 ),
 ( 0.000000000000000000, 0.001701700952312556721, 0.002552551428468834756, 0.003403401904625113442, 0.005105102856937667778, 0.006806803809250222548 ),
 .UNSPECIFIED. ) ;
#28102=CARTESIAN_POINT ( 'NONE',  ( -25.21604033134154577, -8.971440100409701301, 10.09254481884992316 ) ) ;
#28103=VERTEX_POINT ( 'NONE', #52751 ) ;
#28104=CARTESIAN_POINT ( 'NONE',  ( 18.99404383257591533, 0.5703370437478672006, 12.04059188870767194 ) ) ;
#28105=DIRECTION ( 'NONE',  ( 0.000000000000000000, 0.07632122047555797706, -0.9970832820307042876 ) ) ;
#28106=FACE_OUTER_BOUND ( 'NONE', #24916, .T. ) ;
#28107=EDGE_LOOP ( 'NONE', ( #37809, #26004, #18396, #2238 ) ) ;
#28110=ORIENTED_EDGE ( 'NONE', *, *, #54731, .F. ) ;
#28112=DIRECTION ( 'NONE',  ( 0.000000000000000000, -0.01356324068817998940, 0.9999080150203990547 ) ) ;
#28113=VERTEX_POINT ( 'NONE', #33104 ) ;
#28115=CARTESIAN_POINT ( 'NONE',  ( -35.00000000000000000, 1.463443770872774774, 12.09831040184924866 ) ) ;
#28117=DIRECTION ( 'NONE',  ( -1.000000000000000000, 0.000000000000000000, 0.000000000000000000 ) ) ;
#28123=EDGE_LOOP ( 'NONE', ( #28864, #40786, #44049, #15363 ) ) ;
#28125=EDGE_LOOP ( 'NONE', ( #25057, #61173, #59357, #58731 ) ) ;
#28126=ORIENTED_EDGE ( 'NONE', *, *, #30555, .F. ) ;
#28127=CARTESIAN_POINT ( 'NONE',  ( -25.21790179505041962, 8.968132426929548373, 10.09542157472211166 ) ) ;
#28129=FACE_OUTER_BOUND ( 'NONE', #23061, .T. ) ;
#28131=AXIS2_PLACEMENT_3D ( 'NONE', #41886, #21943, #15621 ) ;
#28133=CARTESIAN_POINT ( 'NONE',  ( -35.00000000000000000, 5.814360711498290257, 10.70999494708494559 ) ) ;
#28135=DIRECTION ( 'NONE',  ( -1.000000000000000000, 0.000000000000000000, 0.000000000000000000 ) ) ;
#28136=VERTEX_POINT ( 'NONE', #65332 ) ;
#28138=CARTESIAN_POINT ( 'NONE',  ( 3.899857516006353553, 5.327130952939131525, -12.43655783340662779 ) ) ;
#28140=EDGE_LOOP ( 'NONE', ( #59068, #63361, #22285, #37669 ) ) ;
#28142=MECHANICAL_DESIGN_GEOMETRIC_PRESENTATION_REPRESENTATION('',(#31316),#33455);
#28144=DIRECTION ( 'NONE',  ( 0.000000000000000000, -0.01356324068817998940, 0.9999080150203990547 ) ) ;
#28145=CARTESIAN_POINT ( 'NONE',  ( -10.85732715899702328, -8.333102996281885666, 8.651287110141016257 ) ) ;
#28147=DIRECTION ( 'NONE',  ( 0.000000000000000000, 0.01356324068817992175, -0.9999080150203990547 ) ) ;
#28149=CARTESIAN_POINT ( 'NONE',  ( 35.00000000000000000, 7.251710744571704836, 9.240395740215555875 ) ) ;
#28150=EDGE_CURVE ( 'NONE', #24439, #22257, #15112, .T. ) ;
#28153=CARTESIAN_POINT ( 'NONE',  ( -18.04458733766117362, 12.91933584589294703, 3.916728392552376370 ) ) ;
#28154=EDGE_CURVE ( 'NONE', #24332, #35410, #8831, .T. ) ;
#28155=VERTEX_POINT ( 'NONE', #24122 ) ;
#28156=EDGE_CURVE ( 'NONE', #13458, #57555, #39402, .T. ) ;
#28158=CYLINDRICAL_SURFACE ( 'NONE', #7439, 5.000000000000000888 ) ;
#28159=CARTESIAN_POINT ( 'NONE',  ( 29.36289517528272697, 4.666195979332582233, 11.05608984446922349 ) ) ;
#28160=AXIS2_PLACEMENT_3D ( 'NONE', #50621, #40626, #10047 ) ;
#28161=CYLINDRICAL_SURFACE ( 'NONE', #38726, 12.74999999999999822 ) ;
#28162=FACE_OUTER_BOUND ( 'NONE', #52875, .T. ) ;
#28165=DIRECTION ( 'NONE',  ( -1.000000000000000000, -0.000000000000000000, 0.000000000000000000 ) ) ;
#28166=ADVANCED_FACE ( 'NONE', ( #18813 ), #60678, .T. ) ;
#28169=FACE_OUTER_BOUND ( 'NONE', #60371, .T. ) ;
#28170=EDGE_CURVE ( 'NONE', #47999, #52971, #35393, .T. ) ;
#28173=CARTESIAN_POINT ( 'NONE',  ( 17.78300047788348337, 10.70435634735966168, 8.233749023714018733 ) ) ;
#28176=ADVANCED_FACE ( 'NONE', ( #29120 ), #19798, .T. ) ;
#28177=VECTOR ( 'NONE', #22416, 1000.000000000000000 ) ;
#28181=VERTEX_POINT ( 'NONE', #39073 ) ;
#28182=FACE_OUTER_BOUND ( 'NONE', #7834, .T. ) ;
#28184=CARTESIAN_POINT ( 'NONE',  ( 37.00000000000000711, 2.250029553613756228, -12.54989509947652060 ) ) ;
#28185=EDGE_CURVE ( 'NONE', #35317, #16693, #2306, .T. ) ;
#28187=CARTESIAN_POINT ( 'NONE',  ( -8.866348673818475135, -2.306797143118023641, -13.30210064843870654 ) ) ;
#28192=ORIENTED_EDGE ( 'NONE', *, *, #42329, .T. ) ;
#28195=LINE ( 'NONE', #17886, #46795 ) ;
#28196=DIRECTION ( 'NONE',  ( 0.000000000000000000, -0.2618041379715703165, 0.9651210252299775583 ) ) ;
#28197=LINE ( 'NONE', #13533, #17070 ) ;
#28198=DIRECTION ( 'NONE',  ( 0.6088860180392798860, 0.7932577242209933877, 0.000000000000000000 ) ) ;
#28202=ORIENTED_EDGE ( 'NONE', *, *, #32685, .T. ) ;
#28203=EDGE_LOOP ( 'NONE', ( #40988, #7294, #31363, #32592 ) ) ;
#28204=CARTESIAN_POINT ( 'NONE',  ( -18.69968187819808136, -4.886710041940224514, -10.96191920124609176 ) ) ;
#28205=ORIENTED_EDGE ( 'NONE', *, *, #58899, .T. ) ;
#28206=AXIS2_PLACEMENT_3D ( 'NONE', #24120, #64997, #49423 ) ;
#28210=VERTEX_POINT ( 'NONE', #55025 ) ;
#28214=VERTEX_POINT ( 'NONE', #9457 ) ;
#28215=ORIENTED_EDGE ( 'NONE', *, *, #14598, .F. ) ;
#28216=DIRECTION ( 'NONE',  ( 0.000000000000000000, -0.5243256840888443904, -0.8515178078024941977 ) ) ;
#28217=EDGE_LOOP ( 'NONE', ( #57017, #63008, #2367, #9521 ) ) ;
#28219=EDGE_CURVE ( 'NONE', #43734, #23613, #20111, .T. ) ;
#28220=VERTEX_POINT ( 'NONE', #50052 ) ;
#28221=ORIENTED_EDGE ( 'NONE', *, *, #58271, .T. ) ;
#28222=DIRECTION ( 'NONE',  ( 0.000000000000000000, -0.01356324068817999114, 0.9999080150203989437 ) ) ;
#28225=CARTESIAN_POINT ( 'NONE',  ( -19.02967556479664069, -11.99999999999998934, 9.262893081595934602E-16 ) ) ;
#28228=EDGE_CURVE ( 'NONE', #33360, #12400, #65637, .T. ) ;
#28232=CYLINDRICAL_SURFACE ( 'NONE', #17019, 12.74999999999999822 ) ;
#28233=CARTESIAN_POINT ( 'NONE',  ( -2.532614230583022152, 11.30437021680556242, 4.026315189028233377 ) ) ;
#28234=EDGE_CURVE ( 'NONE', #11746, #52407, #45815, .T. ) ;
#28237=DIRECTION ( 'NONE',  ( 0.000000000000000000, -0.01356324068817992001, 0.9999080150203990547 ) ) ;
#28239=CYLINDRICAL_SURFACE ( 'NONE', #30213, 5.000000000000000888 ) ;
#28243=AXIS2_PLACEMENT_3D ( 'NONE', #31955, #22306, #42247 ) ;
#28244=EDGE_LOOP ( 'NONE', ( #46863, #35039, #61974, #22974 ) ) ;
#28245=DIRECTION ( 'NONE',  ( 0.000000000000000000, -0.01356324068817992175, 0.9999080150203990547 ) ) ;
#28247=DIRECTION ( 'NONE',  ( 0.000000000000000000, -0.1740410799127685149, -0.9847383929261604996 ) ) ;
#28250=VERTEX_POINT ( 'NONE', #15759 ) ;
#28256=AXIS2_PLACEMENT_3D ( 'NONE', #56339, #65636, #20110 ) ;
#28258=CARTESIAN_POINT ( 'NONE',  ( -4.979815405451806676, -1.249695498034863128, -13.44307378499100913 ) ) ;
#28260=LINE ( 'NONE', #53203, #9436 ) ;
#28261=EDGE_CURVE ( 'NONE', #19382, #63181, #57015, .T. ) ;
#28268=ORIENTED_EDGE ( 'NONE', *, *, #28591, .F. ) ;
#28272=DIRECTION ( 'NONE',  ( 1.000000000000000000, 0.000000000000000000, 0.000000000000000000 ) ) ;
#28273=CARTESIAN_POINT ( 'NONE',  ( -37.00000000000000711, -11.38112321385052716, 2.905556151562584954 ) ) ;
#28274=ORIENTED_EDGE ( 'NONE', *, *, #46205, .T. ) ;
#28275=ORIENTED_EDGE ( 'NONE', *, *, #47128, .T. ) ;
#28276=VERTEX_POINT ( 'NONE', #5158 ) ;
#28277=CARTESIAN_POINT ( 'NONE',  ( 22.36482863261543486, 11.96441317219527889, -0.9234811557364158707 ) ) ;
#28279=ORIENTED_EDGE ( 'NONE', *, *, #35527, .T. ) ;
#28281=FACE_OUTER_BOUND ( 'NONE', #48719, .T. ) ;
#28283=EDGE_CURVE ( 'NONE', #3518, #42938, #15447, .T. ) ;
#28284=EDGE_LOOP ( 'NONE', ( #4404, #49173, #4459, #54183 ) ) ;
#28294=( NAMED_UNIT ( * ) SI_UNIT ( $, .STERADIAN. ) SOLID_ANGLE_UNIT ( ) );
#28295=ORIENTED_EDGE ( 'NONE', *, *, #37964, .F. ) ;
#28296=EDGE_CURVE ( 'NONE', #58711, #16620, #54336, .T. ) ;
#28300=CARTESIAN_POINT ( 'NONE',  ( -36.00000000000000711, -5.143145423404365424, 11.66664283989678275 ) ) ;
#28301=DIRECTION ( 'NONE',  ( 0.000000000000000000, -0.9796553971857721033, -0.2006870767258996657 ) ) ;
#28302=CARTESIAN_POINT ( 'NONE',  ( -35.00000000000000000, -9.493370459201647904, -6.917234959366931335 ) ) ;
#28305=ORIENTED_EDGE ( 'NONE', *, *, #36763, .T. ) ;
#28307=DIRECTION ( 'NONE',  ( 0.000000000000000000, 0.01356324068817998940, -0.9999080150203990547 ) ) ;
#28309=EDGE_CURVE ( 'NONE', #28210, #27619, #34925, .T. ) ;
#28310=ORIENTED_EDGE ( 'NONE', *, *, #44826, .T. ) ;
#28314=EDGE_CURVE ( 'NONE', #31078, #31872, #814, .T. ) ;
#28315=ORIENTED_EDGE ( 'NONE', *, *, #61286, .F. ) ;
#28316=EDGE_LOOP ( 'NONE', ( #23073, #5233, #49827, #9388 ) ) ;
#28317=CARTESIAN_POINT ( 'NONE',  ( 35.00000000000000000, -11.10408318471055011, 6.265926637539605437 ) ) ;
#28318=ORIENTED_EDGE ( 'NONE', *, *, #11229, .T. ) ;
#28319=LINE ( 'NONE', #19334, #56135 ) ;
#28320=CARTESIAN_POINT ( 'NONE',  ( -35.00000000000000000, -0.4993900848166508144, -12.17626345777664554 ) ) ;
#28323=CARTESIAN_POINT ( 'NONE',  ( -37.00000000000000711, -12.73293890771483028, -0.6593684648221820321 ) ) ;
#28324=ORIENTED_EDGE ( 'NONE', *, *, #3316, .F. ) ;
#28325=AXIS2_PLACEMENT_3D ( 'NONE', #10520, #50468, #4913 ) ;
#28326=CARTESIAN_POINT ( 'NONE',  ( 35.00000000000000000, -10.07641281632173325, 6.036400161834665212 ) ) ;
#28328=CIRCLE ( 'NONE', #45321, 5.000000000000000000 ) ;
#28329=EDGE_CURVE ( 'NONE', #48483, #55391, #12094, .T. ) ;
#28331=CARTESIAN_POINT ( 'NONE',  ( 35.00000000000000000, 3.307597835713413037, 12.31350058095519096 ) ) ;
#28332=CYLINDRICAL_SURFACE ( 'NONE', #46578, 12.18649999999999878 ) ;
#28337=VERTEX_POINT ( 'NONE', #43329 ) ;
#28338=CARTESIAN_POINT ( 'NONE',  ( 12.84033272753670474, -11.13604314287161401, -4.475189157715393939 ) ) ;
#28339=( BOUNDED_CURVE ( )  B_SPLINE_CURVE ( 3, ( #48945, #48615, #23675, #53611 ),
 .UNSPECIFIED., .F., .F. ) 
 B_SPLINE_CURVE_WITH_KNOTS ( ( 4, 4 ),
 ( 4.975352684836342299, 4.993910677237379581 ),
 .UNSPECIFIED. ) 
 CURVE ( )  GEOMETRIC_REPRESENTATION_ITEM ( )  RATIONAL_B_SPLINE_CURVE ( ( 1.000000000000000000, 0.9999713002824244246, 0.9999713002824244246, 1.000000000000000000 ) ) 
 REPRESENTATION_ITEM ( '' )  );
#28341=CARTESIAN_POINT ( 'NONE',  ( 35.00000000000000000, -3.287724142101329683, 11.73463472867578972 ) ) ;
#28342=DIRECTION ( 'NONE',  ( 0.000000000000000000, 0.01356324068817998940, -0.9999080150203989437 ) ) ;
#28345=CARTESIAN_POINT ( 'NONE',  ( 21.90174657591892071, -13.47998113580522528, -0.7349207973210680755 ) ) ;
#28346=FACE_OUTER_BOUND ( 'NONE', #15420, .T. ) ;
#28349=ORIENTED_EDGE ( 'NONE', *, *, #2832, .T. ) ;
#28350=CARTESIAN_POINT ( 'NONE',  ( -35.00000000000000000, 0.000000000000000000, 0.000000000000000000 ) ) ;
#28354=CARTESIAN_POINT ( 'NONE',  ( 3.934515826361683288, 5.928730106699989122, 12.13052178345963128 ) ) ;
#28356=CARTESIAN_POINT ( 'NONE',  ( 18.73357960737152794, 5.263351130133424149, 10.79392331976826291 ) ) ;
#28357=EDGE_CURVE ( 'NONE', #52828, #40351, #19287, .T. ) ;
#28358=EDGE_LOOP ( 'NONE', ( #60426, #17655, #29735, #40906 ) ) ;
#28360=AXIS2_PLACEMENT_3D ( 'NONE', #2133, #42670, #48369 ) ;
#28362=CARTESIAN_POINT ( 'NONE',  ( -35.00000000000000000, -2.627174906296831480, -11.44858830469743083 ) ) ;
#28364=VERTEX_POINT ( 'NONE', #32372 ) ;
#28366=ORIENTED_EDGE ( 'NONE', *, *, #11066, .T. ) ;
#28367=CARTESIAN_POINT ( 'NONE',  ( -18.87309976548205626, 13.48469254801326755, -0.9257068828140080363 ) ) ;
#28368=ORIENTED_EDGE ( 'NONE', *, *, #13241, .T. ) ;
#28369=AXIS2_PLACEMENT_3D ( 'NONE', #29589, #18676, #33927 ) ;
#28371=DIRECTION ( 'NONE',  ( 0.000000000000000000, 0.01356324068817992175, -0.9999080150203990547 ) ) ;
#28372=DIRECTION ( 'NONE',  ( 1.000000000000000000, -0.000000000000000000, 0.000000000000000000 ) ) ;
#28375=DIRECTION ( 'NONE',  ( 1.000000000000000000, 0.000000000000000000, 0.000000000000000000 ) ) ;
#28377=CARTESIAN_POINT ( 'NONE',  ( -6.973115560797586099, -1.808105581326604705, -13.37853677315561285 ) ) ;
#28378=DIRECTION ( 'NONE',  ( -1.000000000000000000, -0.000000000000000000, -0.000000000000000000 ) ) ;
#28380=CARTESIAN_POINT ( 'NONE',  ( 35.00000000000000000, -5.273331777780263074, 10.49591321039685887 ) ) ;
#28381=ORIENTED_EDGE ( 'NONE', *, *, #49618, .T. ) ;
#28383=ORIENTED_EDGE ( 'NONE', *, *, #58285, .T. ) ;
#28388=CARTESIAN_POINT ( 'NONE',  ( 36.00000000000000711, 11.90598845858539967, 4.561791185930283099 ) ) ;
#28389=EDGE_CURVE ( 'NONE', #52228, #19449, #51146, .T. ) ;
#28393=CARTESIAN_POINT ( 'NONE',  ( 37.00000000000000711, 4.705694406421931860E-17, -3.469127814946512892E-15 ) ) ;
#28395=CARTESIAN_POINT ( 'NONE',  ( 6.511148368283224741, -4.283242813471564325, -11.20980722696366882 ) ) ;
#28396=EDGE_CURVE ( 'NONE', #6864, #59141, #42328, .T. ) ;
#28402=ORIENTED_EDGE ( 'NONE', *, *, #7177, .T. ) ;
#28406=EDGE_CURVE ( 'NONE', #1560, #64905, #45330, .T. ) ;
#28407=AXIS2_PLACEMENT_3D ( 'NONE', #27452, #26472, #11828 ) ;
#28409=CARTESIAN_POINT ( 'NONE',  ( 35.00000000000000000, 11.13736569743274174, -4.946702696913213515 ) ) ;
#28410=ORIENTED_EDGE ( 'NONE', *, *, #58000, .F. ) ;
#28411=CARTESIAN_POINT ( 'NONE',  ( -18.06472325377715649, 4.740409429902864069, 12.64225488003265774 ) ) ;
#28413=CARTESIAN_POINT ( 'NONE',  ( 36.00000000000000711, 10.39746860227901060, 7.379373053628751400 ) ) ;
#28414=ORIENTED_EDGE ( 'NONE', *, *, #58874, .F. ) ;
#28415=DIRECTION ( 'NONE',  ( 0.000000000000000000, -0.9651210252299821102, -0.2618041379715529970 ) ) ;
#28417=ORIENTED_EDGE ( 'NONE', *, *, #36258, .F. ) ;
#28420=FACE_OUTER_BOUND ( 'NONE', #37977, .T. ) ;
#28422=CARTESIAN_POINT ( 'NONE',  ( 35.00000000000000000, 7.379373053628867751, -10.39746860227893244 ) ) ;
#28423=CYLINDRICAL_SURFACE ( 'NONE', #3895, 4.999999999999999112 ) ;
#28424=CARTESIAN_POINT ( 'NONE',  ( 35.00000000000000000, 12.26766708251991389, -3.473736367725300589 ) ) ;
#28425=FACE_OUTER_BOUND ( 'NONE', #12915, .T. ) ;
#28426=EDGE_CURVE ( 'NONE', #37783, #27549, #35265, .T. ) ;
#28429=LINE ( 'NONE', #22135, #7497 ) ;
#28430=ORIENTED_EDGE ( 'NONE', *, *, #56271, .T. ) ;
#28432=DIRECTION ( 'NONE',  ( -1.000000000000000000, 0.000000000000000000, 0.000000000000000000 ) ) ;
#28433=ORIENTED_EDGE ( 'NONE', *, *, #5712, .F. ) ;
#28436=EDGE_LOOP ( 'NONE', ( #28110, #48328, #35380, #20175 ) ) ;
#28437=CARTESIAN_POINT ( 'NONE',  ( -26.62724309483121488, 12.18261572180475127, 5.817022916452319059 ) ) ;
#28440=CARTESIAN_POINT ( 'NONE',  ( -24.31937550808052251, 10.15575759614895190, 8.896613522854025291 ) ) ;
#28446=AXIS2_PLACEMENT_3D ( 'NONE', #6438, #42301, #1783 ) ;
#28447=DIRECTION ( 'NONE',  ( 0.000000000000000000, 0.8009703041134145218, 0.5987040770935704304 ) ) ;
#28449=DIRECTION ( 'NONE',  ( 0.000000000000000000, 0.01356324068817998940, -0.9999080150203989437 ) ) ;
#28453=ORIENTED_EDGE ( 'NONE', *, *, #59076, .T. ) ;
#28457=CARTESIAN_POINT ( 'NONE',  ( 29.35982233226165405, 7.748204631658820674, 11.05532493772648195 ) ) ;
#28458=FACE_OUTER_BOUND ( 'NONE', #56779, .T. ) ;
#28463=CARTESIAN_POINT ( 'NONE',  ( -17.54726996257253191, 12.93490414535030020, 3.865003848717349033 ) ) ;
#28464=ORIENTED_EDGE ( 'NONE', *, *, #63377, .F. ) ;
#28465=LINE ( 'NONE', #13491, #29585 ) ;
#28467=CARTESIAN_POINT ( 'NONE',  ( -35.00000000000000000, 0.000000000000000000, 0.000000000000000000 ) ) ;
#28468=FACE_OUTER_BOUND ( 'NONE', #21678, .T. ) ;
#28469=CARTESIAN_POINT ( 'NONE',  ( 37.00000000000000711, -8.766823244861932096, 7.817610399097601359 ) ) ;
#28471=AXIS2_PLACEMENT_3D ( 'NONE', #14136, #18820, #3869 ) ;
#28472=CARTESIAN_POINT ( 'NONE',  ( 5.195242505075158057, -10.34130555456374445, -8.684426116891836855 ) ) ;
#28473=CARTESIAN_POINT ( 'NONE',  ( -35.00000000000000000, -11.30684963584386082, -4.545979934229532837 ) ) ;
#28475=PLANE ( 'NONE',  #3152 ) ;
#28478=LINE ( 'NONE', #38124, #55537 ) ;
#28482=EDGE_CURVE ( 'NONE', #54635, #24055, #15046, .T. ) ;
#28485=CIRCLE ( 'NONE', #11493, 4.999999999999999112 ) ;
#28486=CIRCLE ( 'NONE', #55067, 12.18650000000000055 ) ;
#28489=CYLINDRICAL_SURFACE ( 'NONE', #13137, 5.683183579532407492 ) ;
#28492=CIRCLE ( 'NONE', #45481, 5.000000000000000888 ) ;
#28495=DIRECTION ( 'NONE',  ( 0.000000000000000000, 0.000000000000000000, -1.000000000000000000 ) ) ;
#28496=CIRCLE ( 'NONE', #55078, 4.999999999999999112 ) ;
#28497=DIRECTION ( 'NONE',  ( 0.000000000000000000, -0.6269146997508042718, -0.7790879021242460567 ) ) ;
#28498=FACE_OUTER_BOUND ( 'NONE', #586, .T. ) ;
#28499=EDGE_CURVE ( 'NONE', #62589, #7316, #49014, .T. ) ;
#28500=CARTESIAN_POINT ( 'NONE',  ( 35.00000000000000000, -12.60630747491661552, 1.908798535168510169 ) ) ;
#28501=ORIENTED_EDGE ( 'NONE', *, *, #47031, .F. ) ;
#28503=DIRECTION ( 'NONE',  ( 0.000000000000000000, -1.000000000000000000, 0.000000000000000000 ) ) ;
#28506=DIRECTION ( 'NONE',  ( 1.000000000000000000, 0.000000000000000000, 0.000000000000000000 ) ) ;
#28507=DIRECTION ( 'NONE',  ( 0.000000000000000000, 0.01356324068817998940, -0.9999080150203990547 ) ) ;
#28508=EDGE_CURVE ( 'NONE', #36243, #5675, #59963, .T. ) ;
#28510=CARTESIAN_POINT ( 'NONE',  ( -35.00000000000000000, -2.905556151562544986, -11.38112321385053960 ) ) ;
#28511=ORIENTED_EDGE ( 'NONE', *, *, #43176, .T. ) ;
#28512=EDGE_CURVE ( 'NONE', #42779, #22257, #34172, .T. ) ;
#28513=EDGE_LOOP ( 'NONE', ( #16232, #43892, #49311, #15383 ) ) ;
#28518=VECTOR ( 'NONE', #53536, 1000.000000000000000 ) ;
#28520=DIRECTION ( 'NONE',  ( 0.000000000000000000, 0.01356324068817998940, -0.9999080150203990547 ) ) ;
#28522=DIRECTION ( 'NONE',  ( 0.000000000000000000, 0.01356324068817998940, -0.9999080150203990547 ) ) ;
#28526=EDGE_CURVE ( 'NONE', #55514, #62548, #52239, .T. ) ;
#28528=ORIENTED_EDGE ( 'NONE', *, *, #51808, .T. ) ;
#28529=DIRECTION ( 'NONE',  ( 1.000000000000000000, -0.000000000000000000, 0.000000000000000000 ) ) ;
#28530=ORIENTED_EDGE ( 'NONE', *, *, #23587, .F. ) ;
#28532=ORIENTED_EDGE ( 'NONE', *, *, #18157, .T. ) ;
#28533=ORIENTED_EDGE ( 'NONE', *, *, #27664, .F. ) ;
#28534=EDGE_CURVE ( 'NONE', #18362, #4143, #31004, .T. ) ;
#28536=CARTESIAN_POINT ( 'NONE',  ( 35.00000000000000000, 11.24036214326529048, 6.018036132182036368 ) ) ;
#28537=VECTOR ( 'NONE', #32009, 1000.000000000000000 ) ;
#28539=DIRECTION ( 'NONE',  ( 1.000000000000000000, 0.000000000000000000, -0.000000000000000000 ) ) ;
#28541=EDGE_CURVE ( 'NONE', #25112, #16758, #8760, .T. ) ;
#28542=DIRECTION ( 'NONE',  ( 1.000000000000000000, 0.000000000000000000, 0.000000000000000000 ) ) ;
#28543=CIRCLE ( 'NONE', #7172, 4.999999999999999112 ) ;
#28544=ORIENTED_EDGE ( 'NONE', *, *, #47616, .T. ) ;
#28546=CARTESIAN_POINT ( 'NONE',  ( 35.00000000000000000, 4.705694406421931860E-17, -3.469127814946512892E-15 ) ) ;
#28548=EDGE_CURVE ( 'NONE', #52495, #15087, #3411, .T. ) ;
#28549=CARTESIAN_POINT ( 'NONE',  ( -19.62940142185039250, -13.44226311714747624, -1.286935523930725855 ) ) ;
#28551=CARTESIAN_POINT ( 'NONE',  ( -18.48287316985193485, 13.41107218970293147, 1.582951252990374202 ) ) ;
#28554=DIRECTION ( 'NONE',  ( -1.000000000000000000, 0.000000000000000000, 0.000000000000000000 ) ) ;
#28556=FACE_OUTER_BOUND ( 'NONE', #9511, .T. ) ;
#28557=ORIENTED_EDGE ( 'NONE', *, *, #65090, .T. ) ;
#28558=DIRECTION ( 'NONE',  ( -1.000000000000000000, -1.836970198721029688E-16, -0.000000000000000000 ) ) ;
#28562=CARTESIAN_POINT ( 'NONE',  ( -37.00000000000000711, 0.000000000000000000, 0.000000000000000000 ) ) ;
#28564=CARTESIAN_POINT ( 'NONE',  ( 35.00000000000000000, 4.705694406421931860E-17, -3.469127814946512892E-15 ) ) ;
#28568=DIRECTION ( 'NONE',  ( 1.000000000000000000, -0.000000000000000000, 0.000000000000000000 ) ) ;
#28570=EDGE_CURVE ( 'NONE', #27227, #31240, #54953, .T. ) ;
#28573=DIRECTION ( 'NONE',  ( -1.000000000000000000, 0.000000000000000000, 0.000000000000000000 ) ) ;
#28574=ORIENTED_EDGE ( 'NONE', *, *, #55147, .F. ) ;
#28575=AXIS2_PLACEMENT_3D ( 'NONE', #55636, #20707, #30018 ) ;
#28576=CARTESIAN_POINT ( 'NONE',  ( 37.00000000000000711, -11.53507381115584529, -2.216820770815045805 ) ) ;
#28578=CARTESIAN_POINT ( 'NONE',  ( -35.00000000000000000, 0.000000000000000000, 0.000000000000000000 ) ) ;
#28579=EDGE_CURVE ( 'NONE', #21209, #37865, #5533, .T. ) ;
#28580=ADVANCED_FACE ( 'NONE', ( #15680 ), #26331, .T. ) ;
#28583=LINE ( 'NONE', #18304, #58412 ) ;
#28588=DIRECTION ( 'NONE',  ( 1.000000000000000000, -0.000000000000000000, 0.000000000000000000 ) ) ;
#28591=EDGE_CURVE ( 'NONE', #37175, #27686, #36303, .T. ) ;
#28593=ORIENTED_EDGE ( 'NONE', *, *, #442, .T. ) ;
#28598=CARTESIAN_POINT ( 'NONE',  ( -35.00000000000000000, 0.000000000000000000, 0.000000000000000000 ) ) ;
#28600=ORIENTED_EDGE ( 'NONE', *, *, #30086, .F. ) ;
#28602=CARTESIAN_POINT ( 'NONE',  ( 35.00000000000000000, -5.015831474386232891, 10.62137734850272786 ) ) ;
#28603=EDGE_CURVE ( 'NONE', #39315, #15531, #25417, .T. ) ;
#28605=VERTEX_POINT ( 'NONE', #35316 ) ;
#28606=ORIENTED_EDGE ( 'NONE', *, *, #19104, .T. ) ;
#28608=EDGE_CURVE ( 'NONE', #13628, #42786, #15088, .T. ) ;
#28610=FACE_OUTER_BOUND ( 'NONE', #10292, .T. ) ;
#28615=EDGE_CURVE ( 'NONE', #60283, #37661, #30947, .T. ) ;
#28616=LINE ( 'NONE', #49578, #59560 ) ;
#28617=DIRECTION ( 'NONE',  ( 0.000000000000000000, 0.2355298848897447450, 0.9718671068226475418 ) ) ;
#28618=VECTOR ( 'NONE', #63081, 1000.000000000000000 ) ;
#28619=CARTESIAN_POINT ( 'NONE',  ( -47.00000000000000711, 0.000000000000000000, 0.000000000000000000 ) ) ;
#28623=EDGE_CURVE ( 'NONE', #12171, #32174, #50960, .T. ) ;
#28625=VERTEX_POINT ( 'NONE', #428 ) ;
#28626=CIRCLE ( 'NONE', #24388, 12.18650000000000233 ) ;
#28627=CARTESIAN_POINT ( 'NONE',  ( -47.00000000000000711, 0.000000000000000000, 0.000000000000000000 ) ) ;
#28630=ORIENTED_EDGE ( 'NONE', *, *, #20140, .F. ) ;
#28631=CARTESIAN_POINT ( 'NONE',  ( 37.00000000000000711, 5.428340790341704469, -10.91072401419412863 ) ) ;
#28634=AXIS2_PLACEMENT_3D ( 'NONE', #52064, #49318, #38975 ) ;
#28635=ORIENTED_EDGE ( 'NONE', *, *, #62031, .F. ) ;
#28636=ORIENTED_EDGE ( 'NONE', *, *, #29089, .T. ) ;
#28640=CARTESIAN_POINT ( 'NONE',  ( -25.45090860874581296, -12.10390572719422586, 5.980235094230700987 ) ) ;
#28641=DIRECTION ( 'NONE',  ( 0.000000000000000000, 0.01356324068817992175, -0.9999080150203990547 ) ) ;
#28643=CARTESIAN_POINT ( 'NONE',  ( -3.138774296833683586, 10.80513712183324238, 5.223565235433476950 ) ) ;
#28644=CARTESIAN_POINT ( 'NONE',  ( 12.58250891015083539, 8.987906597619184978, -7.961848984263494522 ) ) ;
#28645=ORIENTED_EDGE ( 'NONE', *, *, #3335, .F. ) ;
#28648=ADVANCED_FACE ( 'NONE', ( #14895 ), #19268, .T. ) ;
#28651=CARTESIAN_POINT ( 'NONE',  ( 25.05309951391468459, 10.77522019223767558, -8.132934882857098202 ) ) ;
#28653=CARTESIAN_POINT ( 'NONE',  ( -37.00000000000000711, 10.07641281632186114, -6.036400161834460043 ) ) ;
#28654=CARTESIAN_POINT ( 'NONE',  ( 6.848819816998693355, -8.369264212050962826, -8.610838094864671888 ) ) ;
#28655=CARTESIAN_POINT ( 'NONE',  ( -37.00000000000000711, -3.511814412392038953, -11.66953048682403171 ) ) ;
#28656=EDGE_CURVE ( 'NONE', #3635, #10611, #35187, .T. ) ;
#28663=CARTESIAN_POINT ( 'NONE',  ( 37.00000000000000711, -8.927548052240835474, 8.295159312811946961 ) ) ;
#28664=DIRECTION ( 'NONE',  ( -0.000000000000000000, -0.000000000000000000, -1.000000000000000000 ) ) ;
#28665=CARTESIAN_POINT ( 'NONE',  ( -27.16190680910943200, 11.80725687591872841, -2.143550592226123985 ) ) ;
#28669=ORIENTED_EDGE ( 'NONE', *, *, #39843, .F. ) ;
#28671=EDGE_CURVE ( 'NONE', #22363, #4226, #20375, .T. ) ;
#28672=VECTOR ( 'NONE', #5561, 1000.000000000000000 ) ;
#28688=CARTESIAN_POINT ( 'NONE',  ( -19.94256134539602243, 13.21349453248879868, -2.782655092070258629 ) ) ;
#28689=AXIS2_PLACEMENT_3D ( 'NONE', #61084, #16185, #10522 ) ;
#28690=VERTEX_POINT ( 'NONE', #3980 ) ;
#28691=CARTESIAN_POINT ( 'NONE',  ( -35.00000000000000000, 0.000000000000000000, 0.000000000000000000 ) ) ;
#28692=CARTESIAN_POINT ( 'NONE',  ( -35.00000000000000000, 3.287724142101577485, -11.73463472867572932 ) ) ;
#28695=DIRECTION ( 'NONE',  ( 1.000000000000000000, 0.000000000000000000, 0.000000000000000000 ) ) ;
#28697=CARTESIAN_POINT ( 'NONE',  ( -9.026820310266758796, -3.106532851708875942, -13.13844627572322921 ) ) ;
#28698=CARTESIAN_POINT ( 'NONE',  ( 11.13635633779574974, 13.44934996100431235, -1.173364222693725756 ) ) ;
#28700=AXIS2_PLACEMENT_3D ( 'NONE', #63932, #23374, #29989 ) ;
#28701=VERTEX_POINT ( 'NONE', #4646 ) ;
#28704=EDGE_CURVE ( 'NONE', #11282, #65463, #204, .T. ) ;
#28708=DIRECTION ( 'NONE',  ( 1.000000000000000000, -0.000000000000000000, 0.000000000000000000 ) ) ;
#28710=B_SPLINE_CURVE_WITH_KNOTS ( 'NONE', 3,
 ( #65686, #20491, #46105, #36081, #36761, #37978, #56387, #36435, #22712, #61059, #62042, #51746, #15488, #35754, #56747, #11171, #21129, #31756 ),
 .UNSPECIFIED., .F., .F.,
 ( 4, 2, 2, 2, 2, 2, 2, 2, 4 ),
 ( 0.000000000000000000, 0.0007305591798604922594, 0.001461118359720984519, 0.002191677539581471466, 0.002922236719441957328, 0.003652795899302445359, 0.004383355079162932523, 0.005113914259023420554, 0.005844473438883908585 ),
 .UNSPECIFIED. ) ;
#28712=FACE_OUTER_BOUND ( 'NONE', #14810, .T. ) ;
#28713=AXIS2_PLACEMENT_3D ( 'NONE', #14149, #8850, #29143 ) ;
#28714=VECTOR ( 'NONE', #50021, 1000.000000000000000 ) ;
#28715=ADVANCED_FACE ( 'NONE', ( #55156 ), #23942, .T. ) ;
#28716=CARTESIAN_POINT ( 'NONE',  ( 35.00000000000000000, -7.110831038798346881, -9.896810808925367908 ) ) ;
#28717=ORIENTED_EDGE ( 'NONE', *, *, #38351, .T. ) ;
#28720=CARTESIAN_POINT ( 'NONE',  ( 37.00000000000000711, 4.705694406421931860E-17, -3.469127814946512892E-15 ) ) ;
#28721=VECTOR ( 'NONE', #34408, 1000.000000000000000 ) ;
#28722=DIRECTION ( 'NONE',  ( 1.000000000000000000, 0.000000000000000000, -0.000000000000000000 ) ) ;
#28723=CARTESIAN_POINT ( 'NONE',  ( 37.00000000000000711, -6.036400161834636791, -10.07641281632175634 ) ) ;
#28725=CIRCLE ( 'NONE', #32979, 12.18649999999999878 ) ;
#28726=EDGE_CURVE ( 'NONE', #58057, #48505, #34847, .T. ) ;
#28728=CARTESIAN_POINT ( 'NONE',  ( -10.21802740604751669, -3.732897637691882320, 12.97489559727909025 ) ) ;
#28732=DIRECTION ( 'NONE',  ( 1.000000000000000000, -0.000000000000000000, 0.000000000000000000 ) ) ;
#28733=DIRECTION ( 'NONE',  ( -1.000000000000000000, 0.000000000000000000, 0.000000000000000000 ) ) ;
#28734=CARTESIAN_POINT ( 'NONE',  ( -37.00000000000000711, 0.000000000000000000, 0.000000000000000000 ) ) ;
#28735=AXIS2_PLACEMENT_3D ( 'NONE', #10618, #56179, #6646 ) ;
#28736=FACE_OUTER_BOUND ( 'NONE', #60316, .T. ) ;
#28738=VECTOR ( 'NONE', #40295, 1000.000000000000000 ) ;
#28739=ORIENTED_EDGE ( 'NONE', *, *, #41878, .F. ) ;
#28743=VERTEX_POINT ( 'NONE', #8630 ) ;
#28744=CARTESIAN_POINT ( 'NONE',  ( 24.16725417678432564, 10.72501634808748605, -8.203748878436343261 ) ) ;
#28746=CARTESIAN_POINT ( 'NONE',  ( 35.00000000000000000, -10.80478261802177897, 5.636262487437428526 ) ) ;
#28747=EDGE_LOOP ( 'NONE', ( #40121, #46681, #47207, #34236 ) ) ;
#28750=DIRECTION ( 'NONE',  ( -1.000000000000000000, -0.000000000000000000, 0.000000000000000000 ) ) ;
#28751=EDGE_CURVE ( 'NONE', #3064, #62086, #64473, .T. ) ;
#28752=AXIS2_PLACEMENT_3D ( 'NONE', #36074, #56379, #31111 ) ;
#28753=AXIS2_PLACEMENT_3D ( 'NONE', #3661, #60132, #55137 ) ;
#28754=AXIS2_PLACEMENT_3D ( 'NONE', #42723, #36093, #16163 ) ;
#28755=ORIENTED_EDGE ( 'NONE', *, *, #14467, .F. ) ;
#28757=DIRECTION ( 'NONE',  ( 0.000000000000000000, -0.4134677391718385997, -0.9105187689796011563 ) ) ;
#28758=CARTESIAN_POINT ( 'NONE',  ( 35.00000000000000000, 4.705694406421931860E-17, -3.469127814946512892E-15 ) ) ;
#28764=EDGE_LOOP ( 'NONE', ( #19785, #35681, #15021, #64773 ) ) ;
#28765=DIRECTION ( 'NONE',  ( -1.000000000000000000, 0.000000000000000000, -0.000000000000000000 ) ) ;
#28768=CARTESIAN_POINT ( 'NONE',  ( -25.10024331987605706, 9.207671482944922658, 9.878016613807114155 ) ) ;
#28770=EDGE_CURVE ( 'NONE', #41816, #32188, #42119, .T. ) ;
#28771=CARTESIAN_POINT ( 'NONE',  ( -3.966091003153757288, 8.436959275399312119, 8.545114390545426986 ) ) ;
#28775=AXIS2_PLACEMENT_3D ( 'NONE', #65508, #10992, #31274 ) ;
#28777=CIRCLE ( 'NONE', #37262, 5.000000000000001776 ) ;
#28779=VERTEX_POINT ( 'NONE', #65133 ) ;
#28781=CARTESIAN_POINT ( 'NONE',  ( 37.00000000000000711, -5.143145423404195782, 11.66664283989685025 ) ) ;
#28782=AXIS2_PLACEMENT_3D ( 'NONE', #36188, #38077, #56494 ) ;
#28784=VERTEX_POINT ( 'NONE', #24911 ) ;
#28785=AXIS2_PLACEMENT_3D ( 'NONE', #55866, #10297, #50880 ) ;
#28789=CARTESIAN_POINT ( 'NONE',  ( 37.00000000000000711, -11.91791701451268004, -2.544412758415803388 ) ) ;
#28790=EDGE_CURVE ( 'NONE', #25468, #65390, #64289, .T. ) ;
#28793=CARTESIAN_POINT ( 'NONE',  ( 35.00000000000000000, 10.70999494708492250, -5.814360711498331113 ) ) ;
#28795=ORIENTED_EDGE ( 'NONE', *, *, #28154, .T. ) ;
#28796=ORIENTED_EDGE ( 'NONE', *, *, #22945, .T. ) ;
#28797=AXIS2_PLACEMENT_3D ( 'NONE', #45348, #44676, #55983 ) ;
#28799=DIRECTION ( 'NONE',  ( 0.000000000000000000, -0.7617968321374946061, -0.6478160128811867313 ) ) ;
#28803=CARTESIAN_POINT ( 'NONE',  ( 35.00000000000000000, 1.463443770872944194, 12.09831040184922024 ) ) ;
#28804=VECTOR ( 'NONE', #11882, 1000.000000000000000 ) ;
#28805=CARTESIAN_POINT ( 'NONE',  ( 37.00000000000000711, 12.42372387097886488, 2.865935305911484932 ) ) ;
#28806=EDGE_CURVE ( 'NONE', #16743, #25074, #12963, .T. ) ;
#28808=CARTESIAN_POINT ( 'NONE',  ( 35.00000000000000000, -10.42955799785315563, 6.303578524887051948 ) ) ;
#28811=DIRECTION ( 'NONE',  ( -0.8214942970785323872, -0.5702167306099040767, 0.000000000000000000 ) ) ;
#28812=ORIENTED_EDGE ( 'NONE', *, *, #59371, .T. ) ;
#28817=AXIS2_PLACEMENT_3D ( 'NONE', #1445, #56968, #11392 ) ;
#28820=AXIS2_PLACEMENT_3D ( 'NONE', #57444, #32148, #52472 ) ;
#28828=CARTESIAN_POINT ( 'NONE',  ( -17.90080902915205741, 4.123225404297082619, -12.85650399841923708 ) ) ;
#28832=CIRCLE ( 'NONE', #21380, 12.18649999999999700 ) ;
#28833=FACE_OUTER_BOUND ( 'NONE', #40217, .T. ) ;
#28834=CARTESIAN_POINT ( 'NONE',  ( -9.824294270242463156, -12.26381755720376709, -5.646954415730274235 ) ) ;
#28835=DIRECTION ( 'NONE',  ( 1.000000000000000000, 0.000000000000000000, -0.000000000000000000 ) ) ;
#28837=CYLINDRICAL_SURFACE ( 'NONE', #13187, 5.000000000000000888 ) ;
#28838=CIRCLE ( 'NONE', #182, 12.18650000000000055 ) ;
#28839=CARTESIAN_POINT ( 'NONE',  ( 35.00000000000000000, 4.705694406421931860E-17, -3.469127814946512892E-15 ) ) ;
#28842=CARTESIAN_POINT ( 'NONE',  ( 37.00000000000000711, 4.705694406421931860E-17, -3.469127814946512892E-15 ) ) ;
#28843=LINE ( 'NONE', #33514, #39523 ) ;
#28845=DIRECTION ( 'NONE',  ( -0.000000000000000000, -1.000000000000000000, -0.000000000000000000 ) ) ;
#28850=ORIENTED_EDGE ( 'NONE', *, *, #35958, .F. ) ;
#28851=DIRECTION ( 'NONE',  ( -1.000000000000000000, 0.000000000000000000, 0.000000000000000000 ) ) ;
#28853=AXIS2_PLACEMENT_3D ( 'NONE', #7347, #19216, #54804 ) ;
#28857=DIRECTION ( 'NONE',  ( 0.000000000000000000, 0.9970832820307037325, 0.07632122047556839928 ) ) ;
#28861=VERTEX_POINT ( 'NONE', #963 ) ;
#28863=DIRECTION ( 'NONE',  ( 0.000000000000000000, 0.01356324068817998940, -0.9999080150203990547 ) ) ;
#28864=ORIENTED_EDGE ( 'NONE', *, *, #42434, .F. ) ;
#28865=ORIENTED_EDGE ( 'NONE', *, *, #20552, .T. ) ;
#28866=AXIS2_PLACEMENT_3D ( 'NONE', #34219, #9940, #30222 ) ;
#28867=DIRECTION ( 'NONE',  ( -1.000000000000000000, 0.000000000000000000, 0.000000000000000000 ) ) ;
#28869=EDGE_CURVE ( 'NONE', #19813, #21025, #51195, .T. ) ;
#28870=AXIS2_PLACEMENT_3D ( 'NONE', #5281, #54529, #24908 ) ;
#28874=CIRCLE ( 'NONE', #51201, 4.999999999999998224 ) ;
#28878=CARTESIAN_POINT ( 'NONE',  ( -18.08686583997218378, 5.371948137514286792, 10.73321488716334215 ) ) ;
#28879=CIRCLE ( 'NONE', #3416, 12.75000000000000178 ) ;
#28881=CARTESIAN_POINT ( 'NONE',  ( -47.00000000000000711, 0.000000000000000000, 0.000000000000000000 ) ) ;
#28886=CYLINDRICAL_SURFACE ( 'NONE', #53590, 12.18650000000000055 ) ;
#28889=ORIENTED_EDGE ( 'NONE', *, *, #65648, .T. ) ;
#28890=DIRECTION ( 'NONE',  ( 1.000000000000000000, -0.000000000000000000, 0.000000000000000000 ) ) ;
#28892=ORIENTED_EDGE ( 'NONE', *, *, #21629, .T. ) ;
#28894=CARTESIAN_POINT ( 'NONE',  ( 37.00000000000000711, 4.603882218679549609, -10.80631716521668828 ) ) ;
#28895=CYLINDRICAL_SURFACE ( 'NONE', #9609, 4.999999999999999112 ) ;
#28896=DIRECTION ( 'NONE',  ( 1.000000000000000000, 0.000000000000000000, -0.000000000000000000 ) ) ;
#28898=EDGE_CURVE ( 'NONE', #28136, #63071, #11910, .T. ) ;
#28900=ORIENTED_EDGE ( 'NONE', *, *, #43117, .T. ) ;
#28901=DIRECTION ( 'NONE',  ( 1.000000000000000000, 0.000000000000000000, 0.000000000000000000 ) ) ;
#28902=CARTESIAN_POINT ( 'NONE',  ( 37.00000000000000711, 0.7536123767498499326, -11.72195762423410414 ) ) ;
#28904=CARTESIAN_POINT ( 'NONE',  ( 10.67301420047229676, 1.169570914859076716, 11.94385026977490405 ) ) ;
#28907=AXIS2_PLACEMENT_3D ( 'NONE', #15839, #50476, #5237 ) ;
#28908=AXIS2_PLACEMENT_3D ( 'NONE', #43506, #58171, #64444 ) ;
#28909=EDGE_CURVE ( 'NONE', #50699, #20343, #21464, .T. ) ;
#28910=CARTESIAN_POINT ( 'NONE',  ( -37.00000000000000711, -9.512294188640947112, 6.891188680298791169 ) ) ;
#28912=ADVANCED_FACE ( 'NONE', ( #62137 ), #57485, .T. ) ;
#28913=ORIENTED_EDGE ( 'NONE', *, *, #54277, .T. ) ;
#28914=DIRECTION ( 'NONE',  ( -1.000000000000000000, 0.000000000000000000, 0.000000000000000000 ) ) ;
#28918=CARTESIAN_POINT ( 'NONE',  ( 35.00000000000000000, -2.021542716731485001, -12.01765980939841327 ) ) ;
#28921=EDGE_LOOP ( 'NONE', ( #49471, #36101, #58127, #39649 ) ) ;
#28922=DIRECTION ( 'NONE',  ( 0.000000000000000000, -0.01356324068817991828, 0.9999080150203990547 ) ) ;
#28923=ADVANCED_FACE ( 'NONE', ( #33179 ), #48182, .T. ) ;
#28928=AXIS2_PLACEMENT_3D ( 'NONE', #64423, #7948, #28216 ) ;
#28930=ORIENTED_EDGE ( 'NONE', *, *, #6392, .T. ) ;
#28933=LINE ( 'NONE', #50855, #27732 ) ;
#28934=CARTESIAN_POINT ( 'NONE',  ( 35.00000000000000000, 11.65150730582934635, 1.488153103997001514 ) ) ;
#28935=ORIENTED_EDGE ( 'NONE', *, *, #34976, .T. ) ;
#28936=CYLINDRICAL_SURFACE ( 'NONE', #60220, 4.999999999999999112 ) ;
#28937=AXIS2_PLACEMENT_3D ( 'NONE', #26500, #270, #25191 ) ;
#28943=DIRECTION ( 'NONE',  ( 1.000000000000000000, 0.000000000000000000, -0.000000000000000000 ) ) ;
#28944=EDGE_LOOP ( 'NONE', ( #11331, #57114, #62310, #47839 ) ) ;
#28948=SURFACE_STYLE_FILL_AREA ( #54225 ) ;
#28949=ORIENTED_EDGE ( 'NONE', *, *, #12755, .T. ) ;
#28950=AXIS2_PLACEMENT_3D ( 'NONE', #54550, #24597, #58901 ) ;
#28951=ORIENTED_EDGE ( 'NONE', *, *, #57021, .F. ) ;
#28952=EDGE_LOOP ( 'NONE', ( #50197, #5564, #19652, #28381 ) ) ;
#28953=DIRECTION ( 'NONE',  ( 0.000000000000000000, 0.01356324068817998940, -0.9999080150203990547 ) ) ;
#28955=AXIS2_PLACEMENT_3D ( 'NONE', #17122, #21462, #16481 ) ;
#28958=AXIS2_PLACEMENT_3D ( 'NONE', #44671, #39367, #23778 ) ;
#28959=CARTESIAN_POINT ( 'NONE',  ( -35.00000000000000000, 11.90598845858533572, 4.561791185930457182 ) ) ;
#28963=VERTEX_POINT ( 'NONE', #47505 ) ;
#28964=FACE_OUTER_BOUND ( 'NONE', #37886, .T. ) ;
#28965=DIRECTION ( 'NONE',  ( 0.000000000000000000, -0.01356324068817999114, 0.9999080150203989437 ) ) ;
#28966=ORIENTED_EDGE ( 'NONE', *, *, #34677, .T. ) ;
#28969=AXIS2_PLACEMENT_3D ( 'NONE', #49295, #41726, #21797 ) ;
#28972=ORIENTED_EDGE ( 'NONE', *, *, #34289, .T. ) ;
#28973=VECTOR ( 'NONE', #25643, 1000.000000000000000 ) ;
#28974=EDGE_CURVE ( 'NONE', #1959, #64903, #61857, .T. ) ;
#28975=ORIENTED_EDGE ( 'NONE', *, *, #16909, .T. ) ;
#28977=ORIENTED_EDGE ( 'NONE', *, *, #376, .T. ) ;
#28978=EDGE_CURVE ( 'NONE', #167, #57337, #57606, .T. ) ;
#28979=DIRECTION ( 'NONE',  ( 0.000000000000000000, 0.000000000000000000, -1.000000000000000000 ) ) ;
#28980=CARTESIAN_POINT ( 'NONE',  ( -19.30612897158720997, -13.39145038892620398, -1.740264294593142358 ) ) ;
#28981=CIRCLE ( 'NONE', #33242, 5.000000000000000888 ) ;
#28982=CARTESIAN_POINT ( 'NONE',  ( 36.00000000000000711, 12.31350058095523003, -3.307597835713290912 ) ) ;
#28983=DIRECTION ( 'NONE',  ( -1.000000000000000000, 0.000000000000000000, 0.000000000000000000 ) ) ;
#28986=ORIENTED_EDGE ( 'NONE', *, *, #34718, .T. ) ;
#28988=CARTESIAN_POINT ( 'NONE',  ( 35.00000000000000000, 4.705694406421931860E-17, -3.469127814946512892E-15 ) ) ;
#28993=EDGE_CURVE ( 'NONE', #20288, #31780, #34113, .T. ) ;
#28995=CARTESIAN_POINT ( 'NONE',  ( 37.00000000000000711, 4.705694406421931860E-17, -3.469127814946512892E-15 ) ) ;
#28997=AXIS2_PLACEMENT_3D ( 'NONE', #20969, #11012, #40942 ) ;
#28999=EDGE_CURVE ( 'NONE', #13921, #1587, #3923, .T. ) ;
#29000=VECTOR ( 'NONE', #24993, 1000.000000000000000 ) ;
#29001=AXIS2_PLACEMENT_3D ( 'NONE', #17968, #49233, #64483 ) ;
#29002=ORIENTED_EDGE ( 'NONE', *, *, #15182, .T. ) ;
#29003=EDGE_CURVE ( 'NONE', #6117, #53424, #24695, .T. ) ;
#29006=EDGE_LOOP ( 'NONE', ( #3920, #58728, #17638, #38661 ) ) ;
#29007=FACE_OUTER_BOUND ( 'NONE', #14924, .T. ) ;
#29011=CYLINDRICAL_SURFACE ( 'NONE', #28634, 4.999999999999999112 ) ;
#29013=AXIS2_PLACEMENT_3D ( 'NONE', #42880, #38554, #52563 ) ;
#29014=VERTEX_POINT ( 'NONE', #48821 ) ;
#29016=CARTESIAN_POINT ( 'NONE',  ( 29.13270927395454990, -11.82606251486632587, 6.514588969236678295 ) ) ;
#29018=ORIENTED_EDGE ( 'NONE', *, *, #51948, .T. ) ;
#29020=DIRECTION ( 'NONE',  ( -1.000000000000000000, 0.000000000000000000, -0.000000000000000000 ) ) ;
#29022=CARTESIAN_POINT ( 'NONE',  ( 18.43752717680369457, 6.464745515762281514, 10.12011330815638921 ) ) ;
#29023=ORIENTED_EDGE ( 'NONE', *, *, #26975, .T. ) ;
#29024=CARTESIAN_POINT ( 'NONE',  ( 35.00000000000000000, 4.705694406421931860E-17, -3.469127814946512892E-15 ) ) ;
#29025=VECTOR ( 'NONE', #52841, 1000.000000000000000 ) ;
#29031=ORIENTED_EDGE ( 'NONE', *, *, #44432, .T. ) ;
#29032=DIRECTION ( 'NONE',  ( 0.000000000000000000, -0.01356324068817992175, 0.9999080150203990547 ) ) ;
#29033=EDGE_LOOP ( 'NONE', ( #58763, #36809, #37491, #55981 ) ) ;
#29034=CARTESIAN_POINT ( 'NONE',  ( 35.00000000000000000, -0.1414404973753014549, -12.74921544981111055 ) ) ;
#29037=CARTESIAN_POINT ( 'NONE',  ( -35.00000000000000000, 0.000000000000000000, 0.000000000000000000 ) ) ;
#29039=EDGE_CURVE ( 'NONE', #9298, #7202, #24181, .T. ) ;
#29040=AXIS2_PLACEMENT_3D ( 'NONE', #42916, #6704, #38241 ) ;
#29042=CARTESIAN_POINT ( 'NONE',  ( -35.00000000000000000, 7.817610399097512541, 8.766823244862019138 ) ) ;
#29043=CARTESIAN_POINT ( 'NONE',  ( -36.00000000000000711, -12.63095688309030429, 1.738225594539952956 ) ) ;
#29045=ORIENTED_EDGE ( 'NONE', *, *, #31657, .F. ) ;
#29048=CIRCLE ( 'NONE', #3579, 5.000000000000000888 ) ;
#29052=AXIS2_PLACEMENT_3D ( 'NONE', #4167, #60028, #65328 ) ;
#29057=AXIS2_PLACEMENT_3D ( 'NONE', #32808, #53117, #64073 ) ;
#29060=VECTOR ( 'NONE', #39801, 1000.000000000000000 ) ;
#29061=CARTESIAN_POINT ( 'NONE',  ( 37.00000000000000711, 6.950793414699941053, 10.68873102412834797 ) ) ;
#29063=DIRECTION ( 'NONE',  ( 0.000000000000000000, 0.04924826701373895277, 0.9987865678893280696 ) ) ;
#29066=CARTESIAN_POINT ( 'NONE',  ( -17.16708216679437271, -6.932898597583876388, 11.58855638538233990 ) ) ;
#29067=EDGE_CURVE ( 'NONE', #21416, #51437, #23611, .T. ) ;
#29069=AXIS2_PLACEMENT_3D ( 'NONE', #50375, #40036, #14750 ) ;
#29071=LINE ( 'NONE', #24733, #30939 ) ;
#29074=CARTESIAN_POINT ( 'NONE',  ( -10.48620311856347875, -9.720786832536937538, -9.367833439828894271 ) ) ;
#29075=VERTEX_POINT ( 'NONE', #61714 ) ;
#29076=CARTESIAN_POINT ( 'NONE',  ( -35.00000000000000000, -2.216820770815165265, 11.53507381115582575 ) ) ;
#29077=CARTESIAN_POINT ( 'NONE',  ( -35.00000000000000000, -11.73808581813438323, 0.4353888892047964587 ) ) ;
#29079=EDGE_CURVE ( 'NONE', #60763, #59719, #65018, .T. ) ;
#29080=AXIS2_PLACEMENT_3D ( 'NONE', #35858, #10278, #55521 ) ;
#29081=EDGE_CURVE ( 'NONE', #18385, #17578, #36361, .T. ) ;
#29082=DIRECTION ( 'NONE',  ( -1.000000000000000000, -1.836970198721029688E-16, -0.000000000000000000 ) ) ;
#29087=CARTESIAN_POINT ( 'NONE',  ( 6.812204945636112896, -4.138731716409435712, 11.26369831714195335 ) ) ;
#29088=ORIENTED_EDGE ( 'NONE', *, *, #6516, .F. ) ;
#29089=EDGE_CURVE ( 'NONE', #42172, #5900, #7708, .T. ) ;
#29090=DIRECTION ( 'NONE',  ( -1.000000000000000000, 0.000000000000000000, 0.000000000000000000 ) ) ;
#29091=DIRECTION ( 'NONE',  ( 1.000000000000000000, 0.000000000000000000, -0.000000000000000000 ) ) ;
#29092=ORIENTED_EDGE ( 'NONE', *, *, #62425, .F. ) ;
#29096=FACE_OUTER_BOUND ( 'NONE', #23157, .T. ) ;
#29097=AXIS2_PLACEMENT_3D ( 'NONE', #6037, #56215, #61525 ) ;
#29099=DIRECTION ( 'NONE',  ( 0.000000000000000000, 0.01356324068817998940, -0.9999080150203989437 ) ) ;
#29100=DIRECTION ( 'NONE',  ( 0.000000000000000000, 0.01356324068817996685, -0.9999080150203990547 ) ) ;
#29103=VECTOR ( 'NONE', #2164, 1000.000000000000000 ) ;
#29104=AXIS2_PLACEMENT_3D ( 'NONE', #54425, #49117, #43775 ) ;
#29107=VERTEX_POINT ( 'NONE', #41423 ) ;
#29108=FACE_OUTER_BOUND ( 'NONE', #65615, .T. ) ;
#29109=ORIENTED_EDGE ( 'NONE', *, *, #54054, .F. ) ;
#29111=AXIS2_PLACEMENT_3D ( 'NONE', #48052, #27107, #22106 ) ;
#29114=CARTESIAN_POINT ( 'NONE',  ( -18.58686583997218378, 5.151216734910788908, 12.47858029384653555 ) ) ;
#29116=DIRECTION ( 'NONE',  ( -1.000000000000000000, -0.000000000000000000, 0.000000000000000000 ) ) ;
#29117=EDGE_CURVE ( 'NONE', #35757, #25311, #29814, .T. ) ;
#29118=CARTESIAN_POINT ( 'NONE',  ( 24.38667543136798344, -1.087042411491959459, 11.95203068355522369 ) ) ;
#29119=DIRECTION ( 'NONE',  ( 0.000000000000000000, 0.01356324068817998940, -0.9999080150203990547 ) ) ;
#29120=FACE_OUTER_BOUND ( 'NONE', #8977, .T. ) ;
#29121=ORIENTED_EDGE ( 'NONE', *, *, #34122, .F. ) ;
#29122=ADVANCED_FACE ( 'NONE', ( #10195 ), #55763, .T. ) ;
#29123=VERTEX_POINT ( 'NONE', #9522 ) ;
#29125=CIRCLE ( 'NONE', #459, 5.000000000000000888 ) ;
#29126=B_SPLINE_CURVE_WITH_KNOTS ( 'NONE', 3,
 ( #8105, #9379, #33369, #38345, #54657, #28377, #18425, #24360, #19396, #8424, #44005, #28697, #54322, #44624, #53669, #59296, #58993, #3128, #49971, #23391, #38690, #33689 ),
 .UNSPECIFIED., .F., .F.,
 ( 4, 2, 2, 2, 2, 2, 2, 2, 2, 2, 4 ),
 ( 0.000000000000000000, 0.001221936687227891637, 0.001832905030841836154, 0.002443873374455780671, 0.003665810061683667537, 0.004276778405297610754, 0.004887746748911554404, 0.006109683436139443438, 0.007331620123367331605, 0.008553556810595219773, 0.009775493497823107072 ),
 .UNSPECIFIED. ) ;
#29129=LINE ( 'NONE', #34086, #56097 ) ;
#29132=DIRECTION ( 'NONE',  ( 1.000000000000000000, 0.000000000000000000, 0.000000000000000000 ) ) ;
#29134=VECTOR ( 'NONE', #24970, 1000.000000000000000 ) ;
#29136=ORIENTED_EDGE ( 'NONE', *, *, #61613, .F. ) ;
#29139=ADVANCED_FACE ( 'NONE', ( #9867 ), #30157, .T. ) ;
#29141=ADVANCED_FACE ( 'NONE', ( #4904 ), #25165, .T. ) ;
#29143=DIRECTION ( 'NONE',  ( 0.000000000000000000, 0.01356324068817992175, -0.9999080150203990547 ) ) ;
#29144=CIRCLE ( 'NONE', #481, 12.75000000000000178 ) ;
#29146=EDGE_CURVE ( 'NONE', #64071, #63385, #37398, .T. ) ;
#29147=DIRECTION ( 'NONE',  ( -1.000000000000000000, 0.000000000000000000, 0.000000000000000000 ) ) ;
#29149=CARTESIAN_POINT ( 'NONE',  ( -10.25715257150912940, -4.753195267362797516, -11.02444816437827591 ) ) ;
#29153=ORIENTED_EDGE ( 'NONE', *, *, #4064, .T. ) ;
#29154=AXIS2_PLACEMENT_3D ( 'NONE', #62319, #57348, #11452 ) ;
#29156=CARTESIAN_POINT ( 'NONE',  ( 22.68177428654798433, -4.560196341733014691, -11.10067150598529473 ) ) ;
#29157=CARTESIAN_POINT ( 'NONE',  ( 35.00000000000000000, 4.705694406421931860E-17, -3.469127814946512892E-15 ) ) ;
#29158=EDGE_CURVE ( 'NONE', #48986, #11917, #5563, .T. ) ;
#29159=AXIS2_PLACEMENT_3D ( 'NONE', #6862, #11820, #27778 ) ;
#29161=EDGE_CURVE ( 'NONE', #19944, #28113, #25737, .T. ) ;
#29168=VERTEX_POINT ( 'NONE', #46758 ) ;
#29169=CARTESIAN_POINT ( 'NONE',  ( -7.353169898081519662, -1.421260117484592689, -13.42529598466177276 ) ) ;
#29170=LINE ( 'NONE', #55746, #25738 ) ;
#29171=CARTESIAN_POINT ( 'NONE',  ( 37.00000000000000711, 12.05416472667167760, 1.791059740004291578 ) ) ;
#29172=DIRECTION ( 'NONE',  ( 0.000000000000000000, 0.6943713148249639477, -0.7196168960969793194 ) ) ;
#29174=CIRCLE ( 'NONE', #37660, 5.000000000000000000 ) ;
#29175=DIRECTION ( 'NONE',  ( -1.000000000000000000, -0.000000000000000000, 0.000000000000000000 ) ) ;
#29176=ORIENTED_EDGE ( 'NONE', *, *, #49188, .F. ) ;
#29179=CARTESIAN_POINT ( 'NONE',  ( -18.55537666206150504, 5.673200735153683283, -12.25320171535231495 ) ) ;
#29182=CARTESIAN_POINT ( 'NONE',  ( 47.00000000000000711, 4.705694406421931860E-17, -3.469127814946512892E-15 ) ) ;
#29184=DIRECTION ( 'NONE',  ( 0.000000000000000000, -0.01356324068817999114, 0.9999080150203989437 ) ) ;
#29185=ORIENTED_EDGE ( 'NONE', *, *, #52660, .T. ) ;
#29186=AXIS2_PLACEMENT_3D ( 'NONE', #18056, #58972, #12715 ) ;
#29190=DIRECTION ( 'NONE',  ( 0.000000000000000000, 0.000000000000000000, -1.000000000000000000 ) ) ;
#29191=ORIENTED_EDGE ( 'NONE', *, *, #64392, .T. ) ;
#29192=DIRECTION ( 'NONE',  ( 0.000000000000000000, 0.3807014730195220631, -0.9246979985058721985 ) ) ;
#29193=EDGE_CURVE ( 'NONE', #64221, #28784, #37766, .T. ) ;
#29199=CIRCLE ( 'NONE', #37694, 5.000000000000000888 ) ;
#29200=CARTESIAN_POINT ( 'NONE',  ( 35.00000000000000000, 4.705694406421931860E-17, -3.469127814946512892E-15 ) ) ;
#29202=DIRECTION ( 'NONE',  ( 0.000000000000000000, -0.01356324068817999114, 0.9999080150203989437 ) ) ;
#29206=DIRECTION ( 'NONE',  ( 1.000000000000000000, 0.000000000000000000, 0.000000000000000000 ) ) ;
#29207=CARTESIAN_POINT ( 'NONE',  ( 9.687175622948609899, -11.98570860552670325, -0.5854820436212360146 ) ) ;
#29208=EDGE_CURVE ( 'NONE', #63500, #43482, #63444, .T. ) ;
#29209=DIRECTION ( 'NONE',  ( -1.000000000000000000, 0.000000000000000000, 0.000000000000000000 ) ) ;
#29210=CARTESIAN_POINT ( 'NONE',  ( -9.351388602708162523, -11.42638970207761950, -3.665735721005252135 ) ) ;
#29216=DIRECTION ( 'NONE',  ( 0.000000000000000000, -0.01356324068817992175, 0.9999080150203990547 ) ) ;
#29220=DIRECTION ( 'NONE',  ( -1.000000000000000000, 0.000000000000000000, -0.000000000000000000 ) ) ;
#29222=AXIS2_PLACEMENT_3D ( 'NONE', #30505, #45813, #51143 ) ;
#29223=ORIENTED_EDGE ( 'NONE', *, *, #61329, .F. ) ;
#29225=VERTEX_POINT ( 'NONE', #2545 ) ;
#29227=CYLINDRICAL_SURFACE ( 'NONE', #28753, 4.999999999999999112 ) ;
#29231=VERTEX_POINT ( 'NONE', #47746 ) ;
#29234=DIRECTION ( 'NONE',  ( 0.000000000000000000, 0.9346839223284527653, -0.3554799084909000539 ) ) ;
#29235=CARTESIAN_POINT ( 'NONE',  ( 10.88148533521881944, 1.035935135079044001, 11.95575279693729520 ) ) ;
#29239=AXIS2_PLACEMENT_3D ( 'NONE', #61204, #371, #1019 ) ;
#29242=ORIENTED_EDGE ( 'NONE', *, *, #56311, .F. ) ;
#29248=ORIENTED_EDGE ( 'NONE', *, *, #22756, .F. ) ;
#29253=CYLINDRICAL_SURFACE ( 'NONE', #42787, 4.999999999999999112 ) ;
#29255=CARTESIAN_POINT ( 'NONE',  ( -37.00000000000000711, 4.725891942574755866, 10.75351884295729477 ) ) ;
#29256=DIRECTION ( 'NONE',  ( -0.2034311943119418153, 0.9790892447477997917, 0.000000000000000000 ) ) ;
#29259=EDGE_LOOP ( 'NONE', ( #15921, #61530, #36045, #39561 ) ) ;
#29263=ORIENTED_EDGE ( 'NONE', *, *, #50664, .T. ) ;
#29264=DIRECTION ( 'NONE',  ( 1.000000000000000000, -0.000000000000000000, 0.000000000000000000 ) ) ;
#29265=DIRECTION ( 'NONE',  ( 1.000000000000000000, 0.000000000000000000, 0.000000000000000000 ) ) ;
#29266=VERTEX_POINT ( 'NONE', #32747 ) ;
#29268=EDGE_CURVE ( 'NONE', #59070, #44987, #9895, .T. ) ;
#29269=EDGE_CURVE ( 'NONE', #5474, #2944, #51252, .T. ) ;
#29270=CARTESIAN_POINT ( 'NONE',  ( 37.00000000000000711, 4.725891942574903304, 10.75351884295722193 ) ) ;
#29274=CYLINDRICAL_SURFACE ( 'NONE', #56509, 12.18650000000000055 ) ;
#29275=EDGE_CURVE ( 'NONE', #43237, #395, #31043, .T. ) ;
#29276=ORIENTED_EDGE ( 'NONE', *, *, #61996, .F. ) ;
#29277=DIRECTION ( 'NONE',  ( 0.000000000000000000, -0.01356324068817998940, 0.9999080150203990547 ) ) ;
#29278=VERTEX_POINT ( 'NONE', #62689 ) ;
#29279=ORIENTED_EDGE ( 'NONE', *, *, #49350, .T. ) ;
#29282=CARTESIAN_POINT ( 'NONE',  ( -20.79170840334646542, 25.00000000000000000, -3.921648409140116698 ) ) ;
#29283=CARTESIAN_POINT ( 'NONE',  ( 35.00000000000000000, 7.251710744571704836, 9.240395740215555875 ) ) ;
#29284=EDGE_CURVE ( 'NONE', #2547, #35661, #40154, .T. ) ;
#29288=ORIENTED_EDGE ( 'NONE', *, *, #18100, .F. ) ;
#29289=CARTESIAN_POINT ( 'NONE',  ( -15.27729454824424948, 5.151216734910788908, 25.00000000000000000 ) ) ;
#29291=CARTESIAN_POINT ( 'NONE',  ( -17.67250291340853607, -7.948201322890581011, -10.91603686538583418 ) ) ;
#29293=CARTESIAN_POINT ( 'NONE',  ( -15.94818086038523752, 8.395239208160713673, 8.574438310199999691 ) ) ;
#29294=DIRECTION ( 'NONE',  ( -1.000000000000000000, -0.000000000000000000, 0.000000000000000000 ) ) ;
#29295=DIRECTION ( 'NONE',  ( -1.000000000000000000, 0.000000000000000000, -0.000000000000000000 ) ) ;
#29300=EDGE_CURVE ( 'NONE', #9098, #15712, #38079, .T. ) ;
#29303=DIRECTION ( 'NONE',  ( -1.000000000000000000, 0.000000000000000000, -0.000000000000000000 ) ) ;
#29306=CARTESIAN_POINT ( 'NONE',  ( 11.34628703507253178, 11.92903996101671460, -1.310401472515283716 ) ) ;
#29307=EDGE_LOOP ( 'NONE', ( #15, #45129, #64623, #61979 ) ) ;
#29313=CARTESIAN_POINT ( 'NONE',  ( 6.812204945636112896, -4.138731716409435712, -11.26369831714194092 ) ) ;
#29314=CYLINDRICAL_SURFACE ( 'NONE', #59805, 4.999999999999999112 ) ;
#29316=ADVANCED_FACE ( 'NONE', ( #4161 ), #14118, .T. ) ;
#29317=CIRCLE ( 'NONE', #51651, 12.18649999999999700 ) ;
#29319=DIRECTION ( 'NONE',  ( -1.000000000000000000, 0.000000000000000000, 0.000000000000000000 ) ) ;
#29322=FACE_OUTER_BOUND ( 'NONE', #47447, .T. ) ;
#29325=FACE_OUTER_BOUND ( 'NONE', #28284, .T. ) ;
#29326=DIRECTION ( 'NONE',  ( -1.000000000000000000, 0.000000000000000000, 0.000000000000000000 ) ) ;
#29329=ORIENTED_EDGE ( 'NONE', *, *, #27568, .F. ) ;
#29330=LINE ( 'NONE', #38979, #39746 ) ;
#29331=ADVANCED_FACE ( 'NONE', ( #34413 ), #18804, .T. ) ;
#29332=VERTEX_POINT ( 'NONE', #63349 ) ;
#29334=DIRECTION ( 'NONE',  ( 0.000000000000000000, -0.01356324068817998940, 0.9999080150203990547 ) ) ;
#29336=DIRECTION ( 'NONE',  ( 0.000000000000000000, 0.9987865678893275145, -0.04924826701374940968 ) ) ;
#29338=CARTESIAN_POINT ( 'NONE',  ( -27.19357181888462094, -10.84410562793472543, 5.138615876886901468 ) ) ;
#29339=EDGE_CURVE ( 'NONE', #53140, #31809, #36976, .T. ) ;
#29341=DIRECTION ( 'NONE',  ( 0.000000000000000000, 0.000000000000000000, -1.000000000000000000 ) ) ;
#29343=ORIENTED_EDGE ( 'NONE', *, *, #7835, .T. ) ;
#29345=EDGE_CURVE ( 'NONE', #2755, #25848, #63667, .T. ) ;
#29346=ORIENTED_EDGE ( 'NONE', *, *, #2640, .T. ) ;
#29349=CARTESIAN_POINT ( 'NONE',  ( -29.46118758560114514, 0.7225184543564773243, -11.98011844538937787 ) ) ;
#29352=CARTESIAN_POINT ( 'NONE',  ( -35.00000000000000000, -2.250029553613845934, 12.54989509947650284 ) ) ;
#29354=ADVANCED_FACE ( 'NONE', ( #38753 ), #64012, .T. ) ;
#29356=DIRECTION ( 'NONE',  ( 0.000000000000000000, 0.01356324068817998940, -0.9999080150203990547 ) ) ;
#29357=DIRECTION ( 'NONE',  ( 0.000000000000000000, -1.000000000000000000, 0.000000000000000000 ) ) ;
#29363=EDGE_CURVE ( 'NONE', #64644, #13346, #22130, .T. ) ;
#29364=ORIENTED_EDGE ( 'NONE', *, *, #53768, .T. ) ;
#29366=CARTESIAN_POINT ( 'NONE',  ( -35.00000000000000000, -11.24036214326516436, -6.018036132182280618 ) ) ;
#29369=CARTESIAN_POINT ( 'NONE',  ( 35.00000000000000000, -10.54834585426224258, -6.102719229070642903 ) ) ;
#29370=EDGE_CURVE ( 'NONE', #50038, #58596, #14652, .T. ) ;
#29372=CYLINDRICAL_SURFACE ( 'NONE', #45724, 12.18650000000000055 ) ;
#29373=VECTOR ( 'NONE', #63264, 1000.000000000000000 ) ;
#29376=ORIENTED_EDGE ( 'NONE', *, *, #30675, .F. ) ;
#29377=DIRECTION ( 'NONE',  ( -0.7886918350401376232, 0.6147887355352408267, 0.000000000000000000 ) ) ;
#29380=CARTESIAN_POINT ( 'NONE',  ( -17.62939896453930544, -5.509730556738257512, 12.32537139461556386 ) ) ;
#29384=VERTEX_POINT ( 'NONE', #2870 ) ;
#29386=CARTESIAN_POINT ( 'NONE',  ( -35.00000000000000000, -6.711949091238219367, 10.84030624090604178 ) ) ;
#29387=CARTESIAN_POINT ( 'NONE',  ( 1.009264106688026130, 0.1360895039168394938, 12.00328975538737630 ) ) ;
#29388=EDGE_CURVE ( 'NONE', #63989, #24479, #28486, .T. ) ;
#29389=EDGE_CURVE ( 'NONE', #40279, #50140, #23126, .T. ) ;
#29390=CARTESIAN_POINT ( 'NONE',  ( 35.00000000000000000, -11.72195762423410414, -0.7536123767498126291 ) ) ;
#29392=ORIENTED_EDGE ( 'NONE', *, *, #23485, .F. ) ;
#29393=LINE ( 'NONE', #24402, #24728 ) ;
#29394=DIRECTION ( 'NONE',  ( 0.000000000000000000, 0.01356324068817992175, -0.9999080150203990547 ) ) ;
#29395=CARTESIAN_POINT ( 'NONE',  ( -18.44728739097037007, 4.191944866150937976, -11.24471234151735999 ) ) ;
#29397=CYLINDRICAL_SURFACE ( 'NONE', #8528, 5.000000000000000888 ) ;
#29398=CARTESIAN_POINT ( 'NONE',  ( -2.532614230583023041, -12.88560382747352584, 4.026315189028235153 ) ) ;
#29399=ORIENTED_EDGE ( 'NONE', *, *, #40123, .F. ) ;
#29402=CIRCLE ( 'NONE', #64426, 5.000000000000001776 ) ;
#29403=ORIENTED_EDGE ( 'NONE', *, *, #46528, .T. ) ;
#29404=CYLINDRICAL_SURFACE ( 'NONE', #3491, 12.18649999999999878 ) ;
#29406=ADVANCED_FACE ( 'NONE', ( #39730 ), #46043, .T. ) ;
#29407=VECTOR ( 'NONE', #1713, 1000.000000000000000 ) ;
#29408=VERTEX_POINT ( 'NONE', #40712 ) ;
#29410=DIRECTION ( 'NONE',  ( -0.000000000000000000, -1.000000000000000000, -0.000000000000000000 ) ) ;
#29415=ORIENTED_EDGE ( 'NONE', *, *, #30754, .F. ) ;
#29416=LINE ( 'NONE', #54386, #7622 ) ;
#29424=CARTESIAN_POINT ( 'NONE',  ( -24.30799348672965010, 10.28595639659987881, 8.745824847788130185 ) ) ;
#29425=CARTESIAN_POINT ( 'NONE',  ( 24.39805594623851093, -0.9048399250569106878, 11.96720254132417338 ) ) ;
#29428=ORIENTED_EDGE ( 'NONE', *, *, #47247, .F. ) ;
#29430=CARTESIAN_POINT ( 'NONE',  ( 37.00000000000000711, -5.710938531231790627, -11.39945968423469580 ) ) ;
#29433=DIRECTION ( 'NONE',  ( 1.000000000000000000, -0.000000000000000000, -0.000000000000000000 ) ) ;
#29434=CARTESIAN_POINT ( 'NONE',  ( 35.00000000000000000, 11.26103545359850955, -3.340853584269734000 ) ) ;
#29435=EDGE_CURVE ( 'NONE', #16609, #14915, #16812, .T. ) ;
#29436=DIRECTION ( 'NONE',  ( -1.000000000000000000, 0.000000000000000000, 0.000000000000000000 ) ) ;
#29437=CARTESIAN_POINT ( 'NONE',  ( 35.00000000000000000, 12.18632975068352664, 0.06441628369840225743 ) ) ;
#29438=EDGE_CURVE ( 'NONE', #65388, #9878, #5825, .T. ) ;
#29441=VERTEX_POINT ( 'NONE', #34716 ) ;
#29442=EDGE_CURVE ( 'NONE', #32242, #18051, #34875, .T. ) ;
#29443=CARTESIAN_POINT ( 'NONE',  ( -35.00000000000000000, 0.000000000000000000, 0.000000000000000000 ) ) ;
#29444=DIRECTION ( 'NONE',  ( -1.000000000000000000, 0.000000000000000000, 0.000000000000000000 ) ) ;
#29445=CARTESIAN_POINT ( 'NONE',  ( -37.00000000000000711, 11.66953048682404415, -3.511814412391998541 ) ) ;
#29447=CARTESIAN_POINT ( 'NONE',  ( -28.24722641916570254, 12.60412408455661115, -4.845634205101751135 ) ) ;
#29448=AXIS2_PLACEMENT_3D ( 'NONE', #17159, #37100, #6211 ) ;
#29449=DIRECTION ( 'NONE',  ( -1.000000000000000000, 0.000000000000000000, -0.000000000000000000 ) ) ;
#29450=DIRECTION ( 'NONE',  ( 1.000000000000000000, -0.000000000000000000, -0.000000000000000000 ) ) ;
#29451=DIRECTION ( 'NONE',  ( 0.000000000000000000, -0.2618041379715703165, 0.9651210252299775583 ) ) ;
#29452=DIRECTION ( 'NONE',  ( 0.000000000000000000, 0.8827602140260299990, -0.4698238015817395308 ) ) ;
#29453=ORIENTED_EDGE ( 'NONE', *, *, #59029, .T. ) ;
#29454=DIRECTION ( 'NONE',  ( 0.2235469969004301449, -0.9746931518056330956, 0.000000000000000000 ) ) ;
#29463=CYLINDRICAL_SURFACE ( 'NONE', #9959, 12.74999999999999822 ) ;
#29466=DIRECTION ( 'NONE',  ( 0.000000000000000000, -0.4134677391718576955, -0.9105187689795926076 ) ) ;
#29467=CARTESIAN_POINT ( 'NONE',  ( 37.00000000000000711, -9.733281772932102172, 8.235637554476744171 ) ) ;
#29469=ADVANCED_FACE ( 'NONE', ( #25414 ), #24771, .T. ) ;
#29470=CYLINDRICAL_SURFACE ( 'NONE', #44512, 4.999999999999999112 ) ;
#29471=CARTESIAN_POINT ( 'NONE',  ( -9.089039412240934368, -10.06143729587027735, -9.029120393835746938 ) ) ;
#29472=AXIS2_PLACEMENT_3D ( 'NONE', #50871, #49574, #39898 ) ;
#29473=CARTESIAN_POINT ( 'NONE',  ( 35.00000000000000000, 5.644643009979216863, 10.30098186818242922 ) ) ;
#29474=ORIENTED_EDGE ( 'NONE', *, *, #18866, .F. ) ;
#29475=DIRECTION ( 'NONE',  ( 0.000000000000000000, -0.01356324068817998940, 0.9999080150203990547 ) ) ;
#29476=LINE ( 'NONE', #9197, #29836 ) ;
#29477=AXIS2_PLACEMENT_3D ( 'NONE', #60162, #23709, #3442 ) ;
#29482=CARTESIAN_POINT ( 'NONE',  ( -35.00000000000000000, 0.000000000000000000, 0.000000000000000000 ) ) ;
#29483=CARTESIAN_POINT ( 'NONE',  ( -37.00000000000000711, 0.3025107581132838175, -11.74226168163341377 ) ) ;
#29484=ORIENTED_EDGE ( 'NONE', *, *, #57818, .T. ) ;
#29485=EDGE_CURVE ( 'NONE', #26426, #27538, #15749, .T. ) ;
#29486=VERTEX_POINT ( 'NONE', #36028 ) ;
#29487=CARTESIAN_POINT ( 'NONE',  ( -17.81785227179914699, -6.314196589589617936, -10.20856936847407503 ) ) ;
#29488=ORIENTED_EDGE ( 'NONE', *, *, #40656, .F. ) ;
#29490=EDGE_CURVE ( 'NONE', #32582, #62051, #51872, .T. ) ;
#29491=CARTESIAN_POINT ( 'NONE',  ( -15.27729454824424948, 5.151216734910788908, 25.00000000000000000 ) ) ;
#29492=AXIS2_PLACEMENT_3D ( 'NONE', #28691, #38336, #53974 ) ;
#29493=FACE_OUTER_BOUND ( 'NONE', #44303, .T. ) ;
#29496=( BOUNDED_CURVE ( )  B_SPLINE_CURVE ( 3, ( #28153, #33468, #12841, #28463 ),
 .UNSPECIFIED., .F., .F. ) 
 B_SPLINE_CURVE_WITH_KNOTS ( ( 4, 4 ),
 ( 1.276435708367962052, 1.280436945677107419 ),
 .UNSPECIFIED. ) 
 CURVE ( )  GEOMETRIC_REPRESENTATION_ITEM ( )  RATIONAL_B_SPLINE_CURVE ( ( 1.000000000000000000, 0.9999986658421111674, 0.9999986658421111674, 1.000000000000000000 ) ) 
 REPRESENTATION_ITEM ( '' )  );
#29497=CARTESIAN_POINT ( 'NONE',  ( 12.86876090758356561, 11.06400415918094993, -4.650693114441405207 ) ) ;
#29499=ORIENTED_EDGE ( 'NONE', *, *, #64000, .T. ) ;
#29502=DIRECTION ( 'NONE',  ( 0.000000000000000000, 0.01356324068817998940, -0.9999080150203989437 ) ) ;
#29503=ORIENTED_EDGE ( 'NONE', *, *, #39144, .T. ) ;
#29504=CARTESIAN_POINT ( 'NONE',  ( 6.778363379174657588, -6.828539355312321923, -9.876072021181311555 ) ) ;
#29505=ORIENTED_EDGE ( 'NONE', *, *, #40536, .F. ) ;
#29506=DIRECTION ( 'NONE',  ( 0.000000000000000000, -0.7790879021242574920, 0.6269146997507901720 ) ) ;
#29508=CARTESIAN_POINT ( 'NONE',  ( -37.00000000000000711, 0.000000000000000000, 0.000000000000000000 ) ) ;
#29509=DIRECTION ( 'NONE',  ( 0.000000000000000000, -0.5472293298355157543, 0.8369827122275419473 ) ) ;
#29511=DIRECTION ( 'NONE',  ( 1.000000000000000000, 0.000000000000000000, 0.000000000000000000 ) ) ;
#29512=EDGE_LOOP ( 'NONE', ( #7035, #31368, #58944, #42551 ) ) ;
#29513=DIRECTION ( 'NONE',  ( -1.000000000000000000, 0.000000000000000000, 0.000000000000000000 ) ) ;
#29514=CARTESIAN_POINT ( 'NONE',  ( -14.74468430517067219, 7.920754711258918057, 9.014586841720371169 ) ) ;
#29515=EDGE_CURVE ( 'NONE', #8204, #45350, #4832, .T. ) ;
#29516=DIRECTION ( 'NONE',  ( 1.000000000000000000, 0.000000000000000000, -0.000000000000000000 ) ) ;
#29517=DIRECTION ( 'NONE',  ( -1.000000000000000000, -0.000000000000000000, 0.000000000000000000 ) ) ;
#29518=CARTESIAN_POINT ( 'NONE',  ( -37.00000000000000711, -9.060822531526103063, 7.474872387600973944 ) ) ;
#29520=LINE ( 'NONE', #45468, #9640 ) ;
#29521=DIRECTION ( 'NONE',  ( 0.000000000000000000, 0.01356324068817998940, -0.9999080150203989437 ) ) ;
#29522=DIRECTION ( 'NONE',  ( -0.000000000000000000, -0.000000000000000000, -1.000000000000000000 ) ) ;
#29523=CIRCLE ( 'NONE', #42274, 12.18650000000000233 ) ;
#29524=VERTEX_POINT ( 'NONE', #10127 ) ;
#29525=DIRECTION ( 'NONE',  ( -1.000000000000000000, 0.000000000000000000, 0.000000000000000000 ) ) ;
#29527=ORIENTED_EDGE ( 'NONE', *, *, #15569, .T. ) ;
#29529=FACE_OUTER_BOUND ( 'NONE', #48138, .T. ) ;
#29530=DIRECTION ( 'NONE',  ( -1.000000000000000000, 0.000000000000000000, -0.000000000000000000 ) ) ;
#29533=CARTESIAN_POINT ( 'NONE',  ( 12.52750123246316072, 0.4973700281276248192, 11.98968819674307618 ) ) ;
#29534=CARTESIAN_POINT ( 'NONE',  ( 35.00000000000000000, -11.91791701451267826, -2.544412758415803388 ) ) ;
#29535=CYLINDRICAL_SURFACE ( 'NONE', #47107, 4.999999999999999112 ) ;
#29539=ADVANCED_FACE ( 'NONE', ( #10438 ), #57989, .T. ) ;
#29542=CARTESIAN_POINT ( 'NONE',  ( 8.621148270653568702, 25.00000000000000000, -5.251012286260225537 ) ) ;
#29544=CARTESIAN_POINT ( 'NONE',  ( -35.00000000000000000, 11.73808581813437968, -0.4353888892048790038 ) ) ;
#29545=FACE_OUTER_BOUND ( 'NONE', #40012, .T. ) ;
#29547=EDGE_CURVE ( 'NONE', #16066, #21159, #52009, .T. ) ;
#29551=CARTESIAN_POINT ( 'NONE',  ( 47.00000000000000711, 4.705694406421931860E-17, -3.469127814946512892E-15 ) ) ;
#29552=ORIENTED_EDGE ( 'NONE', *, *, #60332, .T. ) ;
#29554=DIRECTION ( 'NONE',  ( -0.000000000000000000, -1.000000000000000000, -0.000000000000000000 ) ) ;
#29555=DIRECTION ( 'NONE',  ( 0.000000000000000000, -0.7381862504172023165, 0.6745969609292585822 ) ) ;
#29557=AXIS2_PLACEMENT_3D ( 'NONE', #46776, #16530, #45796 ) ;
#29560=CARTESIAN_POINT ( 'NONE',  ( -35.00000000000000000, -0.3025107581132014389, 11.74226168163341200 ) ) ;
#29561=EDGE_LOOP ( 'NONE', ( #48448, #26320, #47077, #5177 ) ) ;
#29562=EDGE_CURVE ( 'NONE', #49868, #39894, #57188, .T. ) ;
#29563=ORIENTED_EDGE ( 'NONE', *, *, #24901, .T. ) ;
#29564=ORIENTED_EDGE ( 'NONE', *, *, #29791, .T. ) ;
#29566=EDGE_CURVE ( 'NONE', #62732, #8336, #13629, .T. ) ;
#29569=VERTEX_POINT ( 'NONE', #12399 ) ;
#29571=VECTOR ( 'NONE', #55656, 1000.000000000000000 ) ;
#29572=ORIENTED_EDGE ( 'NONE', *, *, #46490, .T. ) ;
#29573=AXIS2_PLACEMENT_3D ( 'NONE', #154, #61003, #20435 ) ;
#29574=CARTESIAN_POINT ( 'NONE',  ( -35.00000000000000000, -0.01609748574453131326, 11.74614673114904129 ) ) ;
#29576=CARTESIAN_POINT ( 'NONE',  ( 5.121690992581745761, -10.38023541319821241, 6.023682858569486598 ) ) ;
#29577=ORIENTED_EDGE ( 'NONE', *, *, #8715, .F. ) ;
#29578=EDGE_LOOP ( 'NONE', ( #44903, #7181, #46161, #62089, #30131, #49655 ) ) ;
#29579=CIRCLE ( 'NONE', #51917, 5.000000000000000000 ) ;
#29580=FACE_OUTER_BOUND ( 'NONE', #58568, .T. ) ;
#29581=ORIENTED_EDGE ( 'NONE', *, *, #8980, .F. ) ;
#29582=CARTESIAN_POINT ( 'NONE',  ( 10.48620311856346454, 8.250315036047107142, 10.68561190601526611 ) ) ;
#29583=VERTEX_POINT ( 'NONE', #42011 ) ;
#29584=ORIENTED_EDGE ( 'NONE', *, *, #7230, .T. ) ;
#29585=VECTOR ( 'NONE', #53761, 1000.000000000000000 ) ;
#29587=DIRECTION ( 'NONE',  ( 0.000000000000000000, 0.01356324068817991828, -0.9999080150203990547 ) ) ;
#29589=CARTESIAN_POINT ( 'NONE',  ( -37.00000000000000711, 0.000000000000000000, 0.000000000000000000 ) ) ;
#29592=VERTEX_POINT ( 'NONE', #62955 ) ;
#29593=CARTESIAN_POINT ( 'NONE',  ( -36.00000000000000711, -9.196955404009360180, 8.830544224262913744 ) ) ;
#29595=DIRECTION ( 'NONE',  ( -1.000000000000000000, 0.000000000000000000, 0.000000000000000000 ) ) ;
#29596=DIRECTION ( 'NONE',  ( -1.000000000000000000, 0.000000000000000000, 0.000000000000000000 ) ) ;
#29597=EDGE_LOOP ( 'NONE', ( #63586, #60879, #26759, #2526 ) ) ;
#29600=CARTESIAN_POINT ( 'NONE',  ( -37.00000000000000711, 0.000000000000000000, 0.000000000000000000 ) ) ;
#29601=EDGE_LOOP ( 'NONE', ( #37832, #11805, #14960, #47645 ) ) ;
#29602=EDGE_CURVE ( 'NONE', #64793, #27273, #47626, .T. ) ;
#29603=ORIENTED_EDGE ( 'NONE', *, *, #34524, .F. ) ;
#29606=ORIENTED_EDGE ( 'NONE', *, *, #3241, .T. ) ;
#29607=CARTESIAN_POINT ( 'NONE',  ( -17.54726996257253191, -12.93490414535027710, 3.865003848717349033 ) ) ;
#29610=CARTESIAN_POINT ( 'NONE',  ( -3.201686629783078608, 10.71899063123891516, 5.398388898813950121 ) ) ;
#29611=CARTESIAN_POINT ( 'NONE',  ( 12.72541067165903073, 11.67533756787475241, -2.779695538651842046 ) ) ;
#29612=ORIENTED_EDGE ( 'NONE', *, *, #41651, .T. ) ;
#29613=CARTESIAN_POINT ( 'NONE',  ( -35.00000000000000000, 12.05416472667165806, 1.791059740004466994 ) ) ;
#29615=AXIS2_PLACEMENT_3D ( 'NONE', #34861, #9598, #29897 ) ;
#29616=AXIS2_PLACEMENT_3D ( 'NONE', #38640, #22701, #7376 ) ;
#29617=EDGE_CURVE ( 'NONE', #21666, #55845, #56110, .T. ) ;
#29619=CARTESIAN_POINT ( 'NONE',  ( 37.00000000000000711, 4.705694406421931860E-17, -3.469127814946512892E-15 ) ) ;
#29620=EDGE_CURVE ( 'NONE', #14030, #35611, #35919, .T. ) ;
#29623=DIRECTION ( 'NONE',  ( 1.000000000000000000, 0.000000000000000000, 0.000000000000000000 ) ) ;
#29624=CIRCLE ( 'NONE', #44485, 4.999999999999999112 ) ;
#29625=B_SPLINE_CURVE_WITH_KNOTS ( 'NONE', 3,
 ( #20423, #35695, #51017, #25744, #20754, #36695, #57654, #11109, #61626, #796 ),
 .UNSPECIFIED., .F., .F.,
 ( 4, 2, 2, 2, 4 ),
 ( 0.005947140490722368188, 0.007059672066379172467, 0.008172203642035975879, 0.009284735217692779291, 0.01039726679334958444 ),
 .UNSPECIFIED. ) ;
#29627=ORIENTED_EDGE ( 'NONE', *, *, #24929, .F. ) ;
#29629=ORIENTED_EDGE ( 'NONE', *, *, #57360, .T. ) ;
#29631=FACE_OUTER_BOUND ( 'NONE', #38884, .T. ) ;
#29632=CARTESIAN_POINT ( 'NONE',  ( 36.00000000000000711, -3.805206332242390133, 12.16893194857553340 ) ) ;
#29635=ORIENTED_EDGE ( 'NONE', *, *, #22426, .F. ) ;
#29636=EDGE_CURVE ( 'NONE', #6845, #34249, #26397, .T. ) ;
#29637=ORIENTED_EDGE ( 'NONE', *, *, #22969, .T. ) ;
#29641=VECTOR ( 'NONE', #57206, 1000.000000000000000 ) ;
#29642=CARTESIAN_POINT ( 'NONE',  ( -27.58653843872338385, 9.954257377628556114, -6.707763964583499217 ) ) ;
#29644=CYLINDRICAL_SURFACE ( 'NONE', #14484, 5.000000000000000888 ) ;
#29647=ORIENTED_EDGE ( 'NONE', *, *, #21015, .F. ) ;
#29648=DIRECTION ( 'NONE',  ( 0.000000000000000000, -0.5243256840888443904, -0.8515178078024941977 ) ) ;
#29651=CARTESIAN_POINT ( 'NONE',  ( 37.00000000000000711, -11.73808581813437613, 0.4353888892049613824 ) ) ;
#29652=DIRECTION ( 'NONE',  ( 0.000000000000000000, 0.01356324068817998940, -0.9999080150203990547 ) ) ;
#29654=DIRECTION ( 'NONE',  ( -1.000000000000000000, -1.836970198721029688E-16, 0.000000000000000000 ) ) ;
#29655=EDGE_LOOP ( 'NONE', ( #58997, #7180, #50833, #60163 ) ) ;
#29656=CARTESIAN_POINT ( 'NONE',  ( -29.60271627082686052, -3.677907232733526488, -11.42254165076253258 ) ) ;
#29658=CARTESIAN_POINT ( 'NONE',  ( -37.00000000000000711, 0.000000000000000000, 0.000000000000000000 ) ) ;
#29659=CARTESIAN_POINT ( 'NONE',  ( 11.36196501432236872, -11.93139467803644393, -1.301023099206525035 ) ) ;
#29660=AXIS2_PLACEMENT_3D ( 'NONE', #2927, #37157, #47488 ) ;
#29661=DIRECTION ( 'NONE',  ( 0.000000000000000000, 0.01356324068817991828, -0.9999080150203990547 ) ) ;
#29663=DIRECTION ( 'NONE',  ( 0.000000000000000000, 0.01356324068817992175, -0.9999080150203990547 ) ) ;
#29666=CARTESIAN_POINT ( 'NONE',  ( 11.32271610705270426, 13.43847017729220106, -1.294440836893753444 ) ) ;
#29667=ORIENTED_EDGE ( 'NONE', *, *, #37664, .T. ) ;
#29669=ORIENTED_EDGE ( 'NONE', *, *, #15882, .F. ) ;
#29670=CARTESIAN_POINT ( 'NONE',  ( 12.99163133893966915, -13.09490509379091527, -3.288953137075154132 ) ) ;
#29673=VERTEX_POINT ( 'NONE', #57322 ) ;
#29674=LINE ( 'NONE', #61261, #15784 ) ;
#29675=CARTESIAN_POINT ( 'NONE',  ( -37.00000000000000711, -6.307491713049102167, 9.908974237959624176 ) ) ;
#29676=AXIS2_PLACEMENT_3D ( 'NONE', #36870, #31864, #57167 ) ;
#29677=CARTESIAN_POINT ( 'NONE',  ( 35.00000000000000000, 11.74614673114903773, 0.01609748574448878478 ) ) ;
#29678=FACE_OUTER_BOUND ( 'NONE', #59155, .T. ) ;
#29679=CARTESIAN_POINT ( 'NONE',  ( 17.27839441901508621, 25.00000000000000000, 5.771933972472480967 ) ) ;
#29680=EDGE_CURVE ( 'NONE', #29997, #44077, #24269, .T. ) ;
#29682=DIRECTION ( 'NONE',  ( 1.000000000000000000, 0.000000000000000000, -0.000000000000000000 ) ) ;
#29684=ORIENTED_EDGE ( 'NONE', *, *, #53017, .T. ) ;
#29685=DIRECTION ( 'NONE',  ( -1.000000000000000000, 0.000000000000000000, -0.000000000000000000 ) ) ;
#29686=DIRECTION ( 'NONE',  ( -1.000000000000000000, -0.000000000000000000, 0.000000000000000000 ) ) ;
#29688=ORIENTED_EDGE ( 'NONE', *, *, #48885, .F. ) ;
#29689=AXIS2_PLACEMENT_3D ( 'NONE', #59093, #23847, #13197 ) ;
#29691=CIRCLE ( 'NONE', #47799, 5.000000000000000888 ) ;
#29692=( BOUNDED_CURVE ( )  B_SPLINE_CURVE ( 3, ( #14701, #54963, #5422, #35657 ),
 .UNSPECIFIED., .F., .F. ) 
 B_SPLINE_CURVE_WITH_KNOTS ( ( 4, 4 ),
 ( 4.298859771126309681, 4.334476141310460662 ),
 .UNSPECIFIED. ) 
 CURVE ( )  GEOMETRIC_REPRESENTATION_ITEM ( )  RATIONAL_B_SPLINE_CURVE ( ( 1.000000000000000000, 0.9998942923082225764, 0.9998942923082225764, 1.000000000000000000 ) ) 
 REPRESENTATION_ITEM ( '' )  );
#29693=CIRCLE ( 'NONE', #19085, 5.000000000000000888 ) ;
#29694=CARTESIAN_POINT ( 'NONE',  ( -37.00000000000000711, -5.300372733891723698, 11.59605747147784882 ) ) ;
#29695=EDGE_CURVE ( 'NONE', #20972, #26426, #41180, .T. ) ;
#29698=EDGE_CURVE ( 'NONE', #40241, #6864, #44417, .T. ) ;
#29699=VERTEX_POINT ( 'NONE', #64268 ) ;
#29702=CARTESIAN_POINT ( 'NONE',  ( 3.732195538077428321, 4.611300756578111226, 11.08753034506807822 ) ) ;
#29703=AXIS2_PLACEMENT_3D ( 'NONE', #64554, #59592, #27120 ) ;
#29704=EDGE_CURVE ( 'NONE', #26398, #41890, #4110, .T. ) ;
#29705=DIRECTION ( 'NONE',  ( 0.000000000000000000, -0.01356324068817992175, 0.9999080150203990547 ) ) ;
#29706=DIRECTION ( 'NONE',  ( 1.000000000000000000, 0.000000000000000000, 0.000000000000000000 ) ) ;
#29707=AXIS2_PLACEMENT_3D ( 'NONE', #61959, #12620, #32568 ) ;
#29710=EDGE_CURVE ( 'NONE', #47218, #25348, #58264, .T. ) ;
#29714=CARTESIAN_POINT ( 'NONE',  ( 35.00000000000000000, 12.17626345777663488, -0.4993900848167889817 ) ) ;
#29716=EDGE_LOOP ( 'NONE', ( #20921, #55058, #16137, #9338, #55520, #47233 ) ) ;
#29717=AXIS2_PLACEMENT_3D ( 'NONE', #12253, #32843, #7599 ) ;
#29719=ORIENTED_EDGE ( 'NONE', *, *, #35267, .T. ) ;
#29720=ORIENTED_EDGE ( 'NONE', *, *, #24289, .F. ) ;
#29721=EDGE_CURVE ( 'NONE', #52971, #30121, #10346, .T. ) ;
#29722=DIRECTION ( 'NONE',  ( -1.000000000000000000, 0.000000000000000000, 0.000000000000000000 ) ) ;
#29724=DIRECTION ( 'NONE',  ( 1.000000000000000000, 0.000000000000000000, 0.000000000000000000 ) ) ;
#29725=DIRECTION ( 'NONE',  ( 0.000000000000000000, -0.01356324068817999114, 0.9999080150203989437 ) ) ;
#29731=DIRECTION ( 'NONE',  ( 1.000000000000000000, -0.000000000000000000, 0.000000000000000000 ) ) ;
#29734=ORIENTED_EDGE ( 'NONE', *, *, #13744, .F. ) ;
#29735=ORIENTED_EDGE ( 'NONE', *, *, #61158, .T. ) ;
#29740=CIRCLE ( 'NONE', #13825, 12.18650000000000055 ) ;
#29741=FACE_OUTER_BOUND ( 'NONE', #51304, .T. ) ;
#29742=DIRECTION ( 'NONE',  ( 1.000000000000000000, 0.000000000000000000, -0.000000000000000000 ) ) ;
#29743=DIRECTION ( 'NONE',  ( 0.000000000000000000, -0.01356324068817998940, 0.9999080150203990547 ) ) ;
#29744=ORIENTED_EDGE ( 'NONE', *, *, #50810, .T. ) ;
#29745=VERTEX_POINT ( 'NONE', #43002 ) ;
#29746=LINE ( 'NONE', #40379, #10395 ) ;
#29747=ORIENTED_EDGE ( 'NONE', *, *, #56208, .T. ) ;
#29748=VERTEX_POINT ( 'NONE', #2462 ) ;
#29750=CARTESIAN_POINT ( 'NONE',  ( 3.780834652287974773, 8.352030633203080257, 10.60629927458383115 ) ) ;
#29751=CARTESIAN_POINT ( 'NONE',  ( 16.78263030916553333, 10.48479066935627202, 5.836879698929882565 ) ) ;
#29753=EDGE_CURVE ( 'NONE', #53931, #9134, #40203, .T. ) ;
#29754=CARTESIAN_POINT ( 'NONE',  ( 37.00000000000000711, -1.463443770872862482, -12.09831040184923978 ) ) ;
#29755=DIRECTION ( 'NONE',  ( 1.000000000000000000, -0.000000000000000000, -0.000000000000000000 ) ) ;
#29757=ORIENTED_EDGE ( 'NONE', *, *, #54655, .F. ) ;
#29758=EDGE_LOOP ( 'NONE', ( #39794, #52008, #15824, #44699, #54803, #57576 ) ) ;
#29760=DIRECTION ( 'NONE',  ( -1.000000000000000000, 0.000000000000000000, 0.000000000000000000 ) ) ;
#29761=EDGE_CURVE ( 'NONE', #65109, #54100, #48728, .T. ) ;
#29762=AXIS2_PLACEMENT_3D ( 'NONE', #38090, #53069, #7506 ) ;
#29764=CARTESIAN_POINT ( 'NONE',  ( 37.00000000000000711, 4.732539170486261604, -11.23004253107766282 ) ) ;
#29767=AXIS2_PLACEMENT_3D ( 'NONE', #34796, #15193, #65074 ) ;
#29768=CARTESIAN_POINT ( 'NONE',  ( -4.975205859172452172, -1.416020129149132778, -11.91616074890918675 ) ) ;
#29769=DIRECTION ( 'NONE',  ( 1.000000000000000000, 0.000000000000000000, 0.000000000000000000 ) ) ;
#29770=CARTESIAN_POINT ( 'NONE',  ( 28.12931769988050590, 12.24233004620663579, 5.700308019928762349 ) ) ;
#29771=EDGE_CURVE ( 'NONE', #43286, #52549, #50861, .T. ) ;
#29772=VERTEX_POINT ( 'NONE', #59289 ) ;
#29778=AXIS2_PLACEMENT_3D ( 'NONE', #63824, #53874, #8311 ) ;
#29784=EDGE_CURVE ( 'NONE', #64240, #1294, #50723, .T. ) ;
#29786=ORIENTED_EDGE ( 'NONE', *, *, #18915, .T. ) ;
#29789=FACE_OUTER_BOUND ( 'NONE', #57831, .T. ) ;
#29791=EDGE_CURVE ( 'NONE', #41767, #31515, #44304, .T. ) ;
#29792=CYLINDRICAL_SURFACE ( 'NONE', #19052, 3.594603870727467676 ) ;
#29795=AXIS2_PLACEMENT_3D ( 'NONE', #59610, #9062, #13392 ) ;
#29796=AXIS2_PLACEMENT_3D ( 'NONE', #57599, #47608, #53599 ) ;
#29799=VERTEX_POINT ( 'NONE', #29996 ) ;
#29800=VECTOR ( 'NONE', #42719, 1000.000000000000000 ) ;
#29801=EDGE_CURVE ( 'NONE', #38611, #62115, #32407, .T. ) ;
#29802=CYLINDRICAL_SURFACE ( 'NONE', #56733, 5.000000000000000888 ) ;
#29804=CARTESIAN_POINT ( 'NONE',  ( -2.822269947909832766, -4.599275498345574142, 11.08601571419041676 ) ) ;
#29806=CARTESIAN_POINT ( 'NONE',  ( 10.48620311856346454, 8.250315036047107142, -10.68561190601526789 ) ) ;
#29808=CIRCLE ( 'NONE', #7669, 5.000000000000001776 ) ;
#29809=ADVANCED_FACE ( 'NONE', ( #30638 ), #19386, .T. ) ;
#29810=CARTESIAN_POINT ( 'NONE',  ( -37.00000000000000711, 5.921969905510501064, -10.14408668126206869 ) ) ;
#29811=CARTESIAN_POINT ( 'NONE',  ( 35.00000000000000000, 1.456211999474505969, 11.65554240571055011 ) ) ;
#29812=ORIENTED_EDGE ( 'NONE', *, *, #39993, .T. ) ;
#29813=VERTEX_POINT ( 'NONE', #50948 ) ;
#29814=LINE ( 'NONE', #30474, #3462 ) ;
#29818=DIRECTION ( 'NONE',  ( 0.000000000000000000, 0.01356324068817998940, -0.9999080150203990547 ) ) ;
#29820=AXIS2_PLACEMENT_3D ( 'NONE', #30000, #50312, #26323 ) ;
#29821=DIRECTION ( 'NONE',  ( 0.000000000000000000, 0.000000000000000000, -1.000000000000000000 ) ) ;
#29822=CARTESIAN_POINT ( 'NONE',  ( -27.25047371082987269, -12.34411773464382200, 5.468532507261036457 ) ) ;
#29823=DIRECTION ( 'NONE',  ( 1.000000000000000000, -0.000000000000000000, 0.000000000000000000 ) ) ;
#29824=ORIENTED_EDGE ( 'NONE', *, *, #9083, .F. ) ;
#29827=VERTEX_POINT ( 'NONE', #34645 ) ;
#29828=ORIENTED_EDGE ( 'NONE', *, *, #10334, .F. ) ;
#29832=ADVANCED_FACE ( 'NONE', ( #35303 ), #50308, .T. ) ;
#29833=CIRCLE ( 'NONE', #23493, 12.18649999999999878 ) ;
#29835=CARTESIAN_POINT ( 'NONE',  ( 35.00000000000000000, -2.346765782874354667, 11.95840593935203522 ) ) ;
#29836=VECTOR ( 'NONE', #60398, 1000.000000000000000 ) ;
#29840=AXIS2_PLACEMENT_3D ( 'NONE', #8115, #28708, #33699 ) ;
#29841=DIRECTION ( 'NONE',  ( 0.000000000000000000, -0.01356324068817991828, 0.9999080150203990547 ) ) ;
#29842=CARTESIAN_POINT ( 'NONE',  ( 36.00000000000000711, -12.74068829017554094, -0.4871980014161073624 ) ) ;
#29846=CYLINDRICAL_SURFACE ( 'NONE', #18162, 4.945031439545089391 ) ;
#29849=DIRECTION ( 'NONE',  ( 1.000000000000000000, 0.000000000000000000, 0.000000000000000000 ) ) ;
#29851=AXIS2_PLACEMENT_3D ( 'NONE', #1100, #37657, #51976 ) ;
#29852=ORIENTED_EDGE ( 'NONE', *, *, #46864, .T. ) ;
#29853=CARTESIAN_POINT ( 'NONE',  ( -16.48910027788405586, 8.233971230660170448, -8.729683764212291308 ) ) ;
#29855=AXIS2_PLACEMENT_3D ( 'NONE', #37022, #37356, #57667 ) ;
#29856=ORIENTED_EDGE ( 'NONE', *, *, #28570, .T. ) ;
#29857=CARTESIAN_POINT ( 'NONE',  ( -3.215522858303206721, -10.71731889880403976, 5.411963614777410392 ) ) ;
#29859=LINE ( 'NONE', #55472, #26093 ) ;
#29861=CARTESIAN_POINT ( 'NONE',  ( -35.00000000000000000, -9.677500615117949678, 6.657191900728284928 ) ) ;
#29862=EDGE_CURVE ( 'NONE', #5232, #50756, #19904, .T. ) ;
#29863=ORIENTED_EDGE ( 'NONE', *, *, #4611, .T. ) ;
#29864=CARTESIAN_POINT ( 'NONE',  ( -11.40165637462999904, -7.731494526685026791, -11.07003512086042463 ) ) ;
#29866=VECTOR ( 'NONE', #27158, 1000.000000000000000 ) ;
#29867=CARTESIAN_POINT ( 'NONE',  ( 12.03384061974589514, 0.5718066298479855813, 11.98657780702208342 ) ) ;
#29872=ORIENTED_EDGE ( 'NONE', *, *, #37043, .F. ) ;
#29873=CARTESIAN_POINT ( 'NONE',  ( -10.48620311856347875, -9.720786832536937538, 7.036071585506805448 ) ) ;
#29874=VECTOR ( 'NONE', #33990, 1000.000000000000000 ) ;
#29876=CIRCLE ( 'NONE', #63868, 5.000000000000000888 ) ;
#29879=CARTESIAN_POINT ( 'NONE',  ( -2.952869152607111136, -7.581333670610126418, 11.17020052527586138 ) ) ;
#29880=FACE_OUTER_BOUND ( 'NONE', #37291, .T. ) ;
#29882=CIRCLE ( 'NONE', #45801, 12.74999999999999822 ) ;
#29883=AXIS2_PLACEMENT_3D ( 'NONE', #62466, #47215, #17603 ) ;
#29884=VECTOR ( 'NONE', #24007, 1000.000000000000000 ) ;
#29885=ORIENTED_EDGE ( 'NONE', *, *, #17879, .T. ) ;
#29886=VERTEX_POINT ( 'NONE', #15362 ) ;
#29888=EDGE_CURVE ( 'NONE', #36819, #24391, #28543, .T. ) ;
#29889=EDGE_LOOP ( 'NONE', ( #13220, #8668, #58970, #21252 ) ) ;
#29892=CARTESIAN_POINT ( 'NONE',  ( 6.361445718264521432, -4.355102044641763648, -11.18181944858513077 ) ) ;
#29894=DIRECTION ( 'NONE',  ( 0.000000000000000000, 0.01356324068817992175, -0.9999080150203990547 ) ) ;
#29896=EDGE_CURVE ( 'NONE', #1348, #62894, #8228, .T. ) ;
#29897=DIRECTION ( 'NONE',  ( 0.000000000000000000, -0.5767582926625032247, -0.8169148498130232028 ) ) ;
#29898=CARTESIAN_POINT ( 'NONE',  ( -4.989057617119011745, -0.9162120371760335003, 25.00000000000000000 ) ) ;
#29901=VERTEX_POINT ( 'NONE', #26988 ) ;
#29903=DIRECTION ( 'NONE',  ( -1.000000000000000000, -0.000000000000000000, 0.000000000000000000 ) ) ;
#29904=AXIS2_PLACEMENT_3D ( 'NONE', #21158, #21507, #15511 ) ;
#29905=AXIS2_PLACEMENT_3D ( 'NONE', #31208, #56826, #5959 ) ;
#29907=ORIENTED_EDGE ( 'NONE', *, *, #12297, .T. ) ;
#29908=ADVANCED_FACE ( 'NONE', ( #36631 ), #46603, .T. ) ;
#29909=AXIS2_PLACEMENT_3D ( 'NONE', #6830, #21800, #46719 ) ;
#29910=CARTESIAN_POINT ( 'NONE',  ( -21.17861794710831091, 25.00000000000000000, -3.604945070120774808 ) ) ;
#29911=ORIENTED_EDGE ( 'NONE', *, *, #65740, .T. ) ;
#29913=CARTESIAN_POINT ( 'NONE',  ( 4.044423495238602229, -10.40360026321140907, -8.606342947645041264 ) ) ;
#29914=DIRECTION ( 'NONE',  ( 0.000000000000000000, 0.01356324068817991828, -0.9999080150203990547 ) ) ;
#29915=CARTESIAN_POINT ( 'NONE',  ( 6.987255982139510380, -8.045048366716516242, 8.915354129207686995 ) ) ;
#29917=CIRCLE ( 'NONE', #13959, 12.18650000000000055 ) ;
#29918=ORIENTED_EDGE ( 'NONE', *, *, #3796, .T. ) ;
#29920=VERTEX_POINT ( 'NONE', #56246 ) ;
#29921=CARTESIAN_POINT ( 'NONE',  ( 10.48620311856346454, 8.250315036047107142, 25.00000000000000000 ) ) ;
#29923=AXIS2_PLACEMENT_3D ( 'NONE', #38360, #33040, #32384 ) ;
#29924=VERTEX_POINT ( 'NONE', #62533 ) ;
#29929=DIRECTION ( 'NONE',  ( 0.000000000000000000, 0.9651210252299785575, 0.2618041379715665973 ) ) ;
#29930=ORIENTED_EDGE ( 'NONE', *, *, #5380, .T. ) ;
#29931=DIRECTION ( 'NONE',  ( 1.000000000000000000, 0.000000000000000000, 0.000000000000000000 ) ) ;
#29932=AXIS2_PLACEMENT_3D ( 'NONE', #56877, #51232, #46881 ) ;
#29935=LINE ( 'NONE', #5011, #44424 ) ;
#29937=EDGE_LOOP ( 'NONE', ( #62686, #58836, #30958, #28414 ) ) ;
#29943=VERTEX_POINT ( 'NONE', #5741 ) ;
#29945=ORIENTED_EDGE ( 'NONE', *, *, #43117, .F. ) ;
#29947=DIRECTION ( 'NONE',  ( 0.000000000000000000, -0.01356324068817998940, 0.9999080150203989437 ) ) ;
#29948=CYLINDRICAL_SURFACE ( 'NONE', #4839, 12.75000000000000178 ) ;
#29949=LINE ( 'NONE', #5351, #22413 ) ;
#29952=ORIENTED_EDGE ( 'NONE', *, *, #49376, .T. ) ;
#29953=DIRECTION ( 'NONE',  ( 1.000000000000000000, 0.000000000000000000, 0.000000000000000000 ) ) ;
#29955=CARTESIAN_POINT ( 'NONE',  ( 35.00000000000000000, 4.705694406421931860E-17, -3.469127814946512892E-15 ) ) ;
#29956=CARTESIAN_POINT ( 'NONE',  ( -30.16311648624135344, -2.210271246884226937, 13.32375839521249361 ) ) ;
#29957=AXIS2_PLACEMENT_3D ( 'NONE', #12899, #7588, #22896 ) ;
#29958=EDGE_CURVE ( 'NONE', #8982, #17169, #732, .T. ) ;
#29960=AXIS2_PLACEMENT_3D ( 'NONE', #51974, #31991, #6751 ) ;
#29965=CARTESIAN_POINT ( 'NONE',  ( 37.00000000000000711, -8.352657516904727686, -8.258652103341406203 ) ) ;
#29966=CYLINDRICAL_SURFACE ( 'NONE', #8867, 5.000000000000000888 ) ;
#29968=VERTEX_POINT ( 'NONE', #35943 ) ;
#29969=CARTESIAN_POINT ( 'NONE',  ( 11.39226460963361376, -11.84307025323660234, -1.956600849590324875 ) ) ;
#29970=VECTOR ( 'NONE', #11531, 1000.000000000000000 ) ;
#29972=DIRECTION ( 'NONE',  ( 1.000000000000000000, 0.000000000000000000, -0.000000000000000000 ) ) ;
#29975=DIRECTION ( 'NONE',  ( 0.000000000000000000, 0.5472293298355273006, -0.8369827122275342868 ) ) ;
#29976=EDGE_LOOP ( 'NONE', ( #36042, #61507, #16069, #5942 ) ) ;
#29977=AXIS2_PLACEMENT_3D ( 'NONE', #42909, #57904, #33265 ) ;
#29978=ORIENTED_EDGE ( 'NONE', *, *, #63955, .T. ) ;
#29979=ORIENTED_EDGE ( 'NONE', *, *, #61519, .T. ) ;
#29980=CARTESIAN_POINT ( 'NONE',  ( 29.00864072608240463, -10.24877626319949186, 6.246278040546365595 ) ) ;
#29981=CIRCLE ( 'NONE', #56540, 12.75000000000000178 ) ;
#29983=AXIS2_PLACEMENT_3D ( 'NONE', #49935, #4394, #55243 ) ;
#29984=ORIENTED_EDGE ( 'NONE', *, *, #44910, .T. ) ;
#29985=CARTESIAN_POINT ( 'NONE',  ( 37.00000000000000711, -3.805206332242389244, 12.16893194857553340 ) ) ;
#29986=CARTESIAN_POINT ( 'NONE',  ( 36.00000000000000711, -0.9416912585475287756, -12.71517666308947625 ) ) ;
#29987=CARTESIAN_POINT ( 'NONE',  ( -37.00000000000000711, -2.627174906296831480, -11.44858830469743083 ) ) ;
#29988=VERTEX_POINT ( 'NONE', #51617 ) ;
#29989=DIRECTION ( 'NONE',  ( 0.000000000000000000, 0.000000000000000000, -1.000000000000000000 ) ) ;
#29992=CARTESIAN_POINT ( 'NONE',  ( 36.00000000000000711, 1.738225594540170782, 12.63095688309027054 ) ) ;
#29994=DIRECTION ( 'NONE',  ( 1.000000000000000000, -0.000000000000000000, -0.000000000000000000 ) ) ;
#29996=CARTESIAN_POINT ( 'NONE',  ( -35.00000000000000000, 12.68495603654571902, 1.286231064351356368 ) ) ;
#29997=VERTEX_POINT ( 'NONE', #6063 ) ;
#29998=CARTESIAN_POINT ( 'NONE',  ( -29.68541646480313645, -1.416020129149148543, -11.91616074890925780 ) ) ;
#29999=CARTESIAN_POINT ( 'NONE',  ( 13.31887391767931206, -10.25789760254341765, -6.242720968652719193 ) ) ;
#30000=CARTESIAN_POINT ( 'NONE',  ( 35.00000000000000000, 4.705694406421931860E-17, -3.469127814946512892E-15 ) ) ;
#30002=CIRCLE ( 'NONE', #34277, 5.000000000000001776 ) ;
#30006=CARTESIAN_POINT ( 'NONE',  ( 37.00000000000000711, -3.033604067594489528, 12.38385022362084698 ) ) ;
#30008=CARTESIAN_POINT ( 'NONE',  ( 9.906964480792026961, 13.48511810156870006, -0.6357016161040081048 ) ) ;
#30009=VERTEX_POINT ( 'NONE', #16002 ) ;
#30012=VECTOR ( 'NONE', #20260, 1000.000000000000000 ) ;
#30013=ORIENTED_EDGE ( 'NONE', *, *, #13744, .T. ) ;
#30014=CARTESIAN_POINT ( 'NONE',  ( 12.97755741834660981, -11.38317177042858042, -7.268834546894593629 ) ) ;
#30016=CIRCLE ( 'NONE', #9828, 12.75000000000000178 ) ;
#30017=EDGE_LOOP ( 'NONE', ( #22576, #40460, #21112, #34993 ) ) ;
#30018=DIRECTION ( 'NONE',  ( 0.000000000000000000, -0.01356324068818000328, 0.9999080150203990547 ) ) ;
#30019=DIRECTION ( 'NONE',  ( 1.000000000000000000, 0.000000000000000000, 0.000000000000000000 ) ) ;
#30020=DIRECTION ( 'NONE',  ( 1.000000000000000000, 0.000000000000000000, 0.000000000000000000 ) ) ;
#30021=DIRECTION ( 'NONE',  ( 0.000000000000000000, 0.01356324068817998940, -0.9999080150203990547 ) ) ;
#30022=CARTESIAN_POINT ( 'NONE',  ( 37.00000000000000711, -8.389074212634222150, 8.839356091080130540 ) ) ;
#30023=ADVANCED_FACE ( 'NONE', ( #61554 ), #36289, .T. ) ;
#30025=AXIS2_PLACEMENT_3D ( 'NONE', #11111, #46674, #20425 ) ;
#30026=ORIENTED_EDGE ( 'NONE', *, *, #61923, .T. ) ;
#30028=DIRECTION ( 'NONE',  ( 0.000000000000000000, -0.01356324068817999114, 0.9999080150203989437 ) ) ;
#30031=ORIENTED_EDGE ( 'NONE', *, *, #59381, .T. ) ;
#30032=CIRCLE ( 'NONE', #10904, 12.75000000000000178 ) ;
#30033=VECTOR ( 'NONE', #3926, 1000.000000000000000 ) ;
#30034=CIRCLE ( 'NONE', #21554, 5.000000000000000000 ) ;
#30035=VECTOR ( 'NONE', #12375, 1000.000000000000000 ) ;
#30037=FACE_OUTER_BOUND ( 'NONE', #64999, .T. ) ;
#30038=DIRECTION ( 'NONE',  ( 0.000000000000000000, 0.9718671068226468757, -0.2355298848897482422 ) ) ;
#30040=DIRECTION ( 'NONE',  ( -1.000000000000000000, 0.000000000000000000, -0.000000000000000000 ) ) ;
#30042=CARTESIAN_POINT ( 'NONE',  ( 3.924844264204268018, 5.816699323270774435, 10.49842868086190073 ) ) ;
#30043=AXIS2_PLACEMENT_3D ( 'NONE', #52043, #38959, #13672 ) ;
#30044=AXIS2_PLACEMENT_3D ( 'NONE', #22129, #36094, #30780 ) ;
#30045=DIRECTION ( 'NONE',  ( 0.000000000000000000, -0.3554799084909035511, -0.9346839223284514331 ) ) ;
#30046=CARTESIAN_POINT ( 'NONE',  ( 145.1370849898475797, 3.309064568108273190E-14, 0.000000000000000000 ) ) ;
#30048=CARTESIAN_POINT ( 'NONE',  ( 3.347841273039249721, -10.61118957148187825, 5.603807266321171987 ) ) ;
#30049=DIRECTION ( 'NONE',  ( 1.000000000000000000, 0.000000000000000000, 0.000000000000000000 ) ) ;
#30050=CIRCLE ( 'NONE', #31103, 12.18649999999999700 ) ;
#30052=VERTEX_POINT ( 'NONE', #52271 ) ;
#30053=CARTESIAN_POINT ( 'NONE',  ( 21.74230132213768485, 12.54654960210808134, -4.998279610834257092 ) ) ;
#30054=CARTESIAN_POINT ( 'NONE',  ( 37.00000000000000711, -2.772148766916200380, -11.86701198550355585 ) ) ;
#30056=EDGE_CURVE ( 'NONE', #42706, #39575, #17296, .T. ) ;
#30058=ORIENTED_EDGE ( 'NONE', *, *, #64865, .T. ) ;
#30059=ADVANCED_FACE ( 'NONE', ( #48920 ), #3041, .T. ) ;
#30060=AXIS2_PLACEMENT_3D ( 'NONE', #55278, #30647, #45624 ) ;
#30061=ORIENTED_EDGE ( 'NONE', *, *, #1162, .F. ) ;
#30065=CARTESIAN_POINT ( 'NONE',  ( -35.00000000000000000, -11.50504120060940316, -4.018060380616521599 ) ) ;
#30067=CARTESIAN_POINT ( 'NONE',  ( -18.49080574448724690, 11.99999999999999645, 2.510045011421233839E-15 ) ) ;
#30068=CARTESIAN_POINT ( 'NONE',  ( -35.00000000000000000, 6.280308599560139093, 9.926225166347048656 ) ) ;
#30069=ORIENTED_EDGE ( 'NONE', *, *, #22429, .T. ) ;
#30070=DIRECTION ( 'NONE',  ( 0.000000000000000000, 0.7790879021242487212, -0.6269146997508011632 ) ) ;
#30071=ORIENTED_EDGE ( 'NONE', *, *, #23444, .T. ) ;
#30074=AXIS2_PLACEMENT_3D ( 'NONE', #42324, #61642, #46687 ) ;
#30075=ORIENTED_EDGE ( 'NONE', *, *, #21332, .T. ) ;
#30078=PLANE ( 'NONE',  #1435 ) ;
#30079=AXIS2_PLACEMENT_3D ( 'NONE', #27277, #11334, #51916 ) ;
#30080=EDGE_CURVE ( 'NONE', #27538, #20683, #10097, .T. ) ;
#30081=DIRECTION ( 'NONE',  ( 0.000000000000000000, -0.9903235168508566222, -0.1387779952735712363 ) ) ;
#30084=ORIENTED_EDGE ( 'NONE', *, *, #20555, .F. ) ;
#30086=EDGE_CURVE ( 'NONE', #57900, #9681, #8374, .T. ) ;
#30087=ORIENTED_EDGE ( 'NONE', *, *, #59482, .F. ) ;
#30088=ADVANCED_FACE ( 'NONE', ( #28610 ), #3373, .T. ) ;
#30090=ORIENTED_EDGE ( 'NONE', *, *, #12976, .F. ) ;
#30091=AXIS2_PLACEMENT_3D ( 'NONE', #13662, #60527, #4711 ) ;
#30092=ADVANCED_FACE ( 'NONE', ( #12996 ), #8667, .T. ) ;
#30093=VERTEX_POINT ( 'NONE', #63520 ) ;
#30094=CIRCLE ( 'NONE', #20512, 12.18650000000000055 ) ;
#30097=LINE ( 'NONE', #31085, #48959 ) ;
#30098=CARTESIAN_POINT ( 'NONE',  ( 18.09544918135259906, 5.659161111724000826, 10.59477254556587233 ) ) ;
#30100=VECTOR ( 'NONE', #13142, 1000.000000000000000 ) ;
#30101=DIRECTION ( 'NONE',  ( -1.000000000000000000, 0.000000000000000000, 0.000000000000000000 ) ) ;
#30102=EDGE_CURVE ( 'NONE', #33400, #16971, #12331, .T. ) ;
#30103=CARTESIAN_POINT ( 'NONE',  ( 28.15950597331847405, -12.57621330935229231, 4.911510989912037495 ) ) ;
#30104=EDGE_LOOP ( 'NONE', ( #4978, #37630, #27342, #9205 ) ) ;
#30105=VECTOR ( 'NONE', #25091, 1000.000000000000000 ) ;
#30106=( BOUNDED_CURVE ( )  B_SPLINE_CURVE ( 3, ( #32177, #26882, #43139, #42148 ),
 .UNSPECIFIED., .F., .F. ) 
 B_SPLINE_CURVE_WITH_KNOTS ( ( 4, 4 ),
 ( 4.643929506547320507, 4.657923478229592185 ),
 .UNSPECIFIED. ) 
 CURVE ( )  GEOMETRIC_REPRESENTATION_ITEM ( )  RATIONAL_B_SPLINE_CURVE ( ( 1.000000000000000000, 0.9999836807962925178, 0.9999836807962925178, 1.000000000000000000 ) ) 
 REPRESENTATION_ITEM ( '' )  );
#30108=ORIENTED_EDGE ( 'NONE', *, *, #13676, .F. ) ;
#30109=AXIS2_PLACEMENT_3D ( 'NONE', #7961, #13264, #2972 ) ;
#30110=DIRECTION ( 'NONE',  ( 1.000000000000000000, 0.000000000000000000, 0.000000000000000000 ) ) ;
#30113=MANIFOLD_SOLID_BREP ( 'Cut-Extrude2', #44007 ) ;
#30114=CARTESIAN_POINT ( 'NONE',  ( 24.82652845881425208, 25.00000000000000000, -8.578654028722157321 ) ) ;
#30115=AXIS2_PLACEMENT_3D ( 'NONE', #33604, #44226, #18967 ) ;
#30116=CARTESIAN_POINT ( 'NONE',  ( -35.00000000000000000, 12.71517666308949401, -0.9416912585473022901 ) ) ;
#30117=EDGE_CURVE ( 'NONE', #46746, #40556, #25214, .T. ) ;
#30118=CARTESIAN_POINT ( 'NONE',  ( -35.00000000000000000, -6.891188680298757419, -9.512294188640973758 ) ) ;
#30121=VERTEX_POINT ( 'NONE', #55191 ) ;
#30122=AXIS2_PLACEMENT_3D ( 'NONE', #38150, #7927, #28198 ) ;
#30127=VECTOR ( 'NONE', #39283, 1000.000000000000000 ) ;
#30128=CARTESIAN_POINT ( 'NONE',  ( -35.00000000000000000, -1.488153103997047033, 11.65150730582934102 ) ) ;
#30130=CIRCLE ( 'NONE', #26959, 5.000000000000000888 ) ;
#30131=ORIENTED_EDGE ( 'NONE', *, *, #61027, .T. ) ;
#30132=DIRECTION ( 'NONE',  ( 0.000000000000000000, -0.01356324068817998940, 0.9999080150203990547 ) ) ;
#30135=VECTOR ( 'NONE', #5940, 1000.000000000000000 ) ;
#30138=CARTESIAN_POINT ( 'NONE',  ( -35.00000000000000000, 0.000000000000000000, 0.000000000000000000 ) ) ;
#30139=CARTESIAN_POINT ( 'NONE',  ( -27.45775109278351067, -10.51123867646838050, -8.471355351200609007 ) ) ;
#30141=AXIS2_PLACEMENT_3D ( 'NONE', #34112, #23508, #60064 ) ;
#30143=ORIENTED_EDGE ( 'NONE', *, *, #60637, .F. ) ;
#30144=CARTESIAN_POINT ( 'NONE',  ( -9.809773280085975600, -12.34599478600513578, -5.464898509519898084 ) ) ;
#30146=DIRECTION ( 'NONE',  ( 0.000000000000000000, -0.6478160128812002760, 0.7617968321374830598 ) ) ;
#30147=ORIENTED_EDGE ( 'NONE', *, *, #51569, .T. ) ;
#30149=CARTESIAN_POINT ( 'NONE',  ( -9.246430435658307800, 11.49892766232029295, -7.081925484302661999 ) ) ;
#30150=DIRECTION ( 'NONE',  ( 0.000000000000000000, -0.01356324068817998940, 0.9999080150203990547 ) ) ;
#30153=VECTOR ( 'NONE', #38444, 1000.000000000000000 ) ;
#30154=FACE_OUTER_BOUND ( 'NONE', #56136, .T. ) ;
#30156=ORIENTED_EDGE ( 'NONE', *, *, #12115, .F. ) ;
#30157=CYLINDRICAL_SURFACE ( 'NONE', #20417, 5.000000000000000888 ) ;
#30160=EDGE_CURVE ( 'NONE', #17913, #60517, #34773, .T. ) ;
#30161=DIRECTION ( 'NONE',  ( 0.7932577242209934987, -0.6088860180392799970, 0.000000000000000000 ) ) ;
#30162=ORIENTED_EDGE ( 'NONE', *, *, #19283, .F. ) ;
#30163=CARTESIAN_POINT ( 'NONE',  ( -27.45775109278350712, -13.35262336282553441, -1.989333891161978674 ) ) ;
#30164=CARTESIAN_POINT ( 'NONE',  ( 11.94227997924816087, 11.73039363638092247, -2.534770156389862361 ) ) ;
#30165=EDGE_CURVE ( 'NONE', #28743, #52094, #39237, .T. ) ;
#30169=CARTESIAN_POINT ( 'NONE',  ( 35.00000000000000000, 4.705694406421931860E-17, -3.469127814946512892E-15 ) ) ;
#30170=EDGE_CURVE ( 'NONE', #23325, #9488, #43285, .T. ) ;
#30171=AXIS2_PLACEMENT_3D ( 'NONE', #55754, #50761, #61704 ) ;
#30172=VECTOR ( 'NONE', #50313, 1000.000000000000000 ) ;
#30173=EDGE_LOOP ( 'NONE', ( #9152, #10353, #11097, #15244 ) ) ;
#30174=CARTESIAN_POINT ( 'NONE',  ( 37.00000000000000711, -2.216820770815006725, 11.53507381115585417 ) ) ;
#30175=CYLINDRICAL_SURFACE ( 'NONE', #28907, 5.000000000000000888 ) ;
#30176=CARTESIAN_POINT ( 'NONE',  ( -47.00000000000000711, 0.000000000000000000, 0.000000000000000000 ) ) ;
#30177=CARTESIAN_POINT ( 'NONE',  ( -29.65104263560079545, -0.5515657081232090420, 11.98927152364481685 ) ) ;
#30178=CARTESIAN_POINT ( 'NONE',  ( 35.00000000000000000, 4.705694406421931860E-17, -3.469127814946512892E-15 ) ) ;
#30179=CARTESIAN_POINT ( 'NONE',  ( -14.11589373245165469, 8.250315036047107142, 10.68561190601526611 ) ) ;
#30181=EDGE_LOOP ( 'NONE', ( #12398, #40003, #42680, #4653 ) ) ;
#30182=CARTESIAN_POINT ( 'NONE',  ( 37.00000000000000711, 11.07407352312218052, 3.916263239775223504 ) ) ;
#30183=EDGE_CURVE ( 'NONE', #38380, #47639, #40215, .T. ) ;
#30185=EDGE_CURVE ( 'NONE', #6763, #62669, #58172, .T. ) ;
#30186=FACE_OUTER_BOUND ( 'NONE', #31431, .T. ) ;
#30187=CARTESIAN_POINT ( 'NONE',  ( -21.17861794710831091, 13.00977982294135593, -3.604945070120774808 ) ) ;
#30189=DIRECTION ( 'NONE',  ( 0.000000000000000000, -0.01356324068817998940, 0.9999080150203990547 ) ) ;
#30190=CARTESIAN_POINT ( 'NONE',  ( -35.00000000000000000, 11.72195762423408816, 0.7536123767500589876 ) ) ;
#30192=CARTESIAN_POINT ( 'NONE',  ( -35.00000000000000000, 5.130401251914729954, 11.05394794832831451 ) ) ;
#30193=EDGE_CURVE ( 'NONE', #20774, #26468, #65170, .T. ) ;
#30194=AXIS2_PLACEMENT_3D ( 'NONE', #52817, #2288, #56496 ) ;
#30196=EDGE_LOOP ( 'NONE', ( #55929, #22803, #30488, #2375 ) ) ;
#30197=DIRECTION ( 'NONE',  ( 1.000000000000000000, -0.000000000000000000, 0.000000000000000000 ) ) ;
#30200=CARTESIAN_POINT ( 'NONE',  ( -2.927828093388545661, -11.04426939139958463, 4.708968905878549549 ) ) ;
#30202=VECTOR ( 'NONE', #51923, 1000.000000000000000 ) ;
#30203=CARTESIAN_POINT ( 'NONE',  ( -17.96022329889432001, 6.012774911231331565, -12.08928202576066369 ) ) ;
#30204=EDGE_CURVE ( 'NONE', #9138, #35622, #13577, .T. ) ;
#30207=ORIENTED_EDGE ( 'NONE', *, *, #44652, .F. ) ;
#30209=CARTESIAN_POINT ( 'NONE',  ( -36.00000000000000711, 10.84030624090606665, 6.711949091238182064 ) ) ;
#30210=DIRECTION ( 'NONE',  ( 1.000000000000000000, 0.000000000000000000, -0.000000000000000000 ) ) ;
#30213=AXIS2_PLACEMENT_3D ( 'NONE', #53180, #28554, #7629 ) ;
#30217=DIRECTION ( 'NONE',  ( -1.000000000000000000, -0.000000000000000000, 0.000000000000000000 ) ) ;
#30218=ORIENTED_EDGE ( 'NONE', *, *, #62738, .T. ) ;
#30221=CIRCLE ( 'NONE', #480, 12.75000000000000178 ) ;
#30222=DIRECTION ( 'NONE',  ( 0.000000000000000000, 0.8827602140260299990, -0.4698238015817395308 ) ) ;
#30223=CARTESIAN_POINT ( 'NONE',  ( 37.00000000000000711, 12.74613886779084737, -0.3137578094509725357 ) ) ;
#30224=EDGE_CURVE ( 'NONE', #48664, #17397, #56057, .T. ) ;
#30225=ORIENTED_EDGE ( 'NONE', *, *, #31647, .T. ) ;
#30226=ORIENTED_EDGE ( 'NONE', *, *, #56123, .T. ) ;
#30227=DIRECTION ( 'NONE',  ( 1.000000000000000000, 0.000000000000000000, 0.000000000000000000 ) ) ;
#30229=DIRECTION ( 'NONE',  ( 0.000000000000000000, -0.5243256840888622650, -0.8515178078024832065 ) ) ;
#30230=DIRECTION ( 'NONE',  ( 0.000000000000000000, -0.8696919319575239227, -0.4935949184179166394 ) ) ;
#30231=VECTOR ( 'NONE', #23839, 1000.000000000000000 ) ;
#30232=DIRECTION ( 'NONE',  ( -0.000000000000000000, -1.000000000000000000, -0.000000000000000000 ) ) ;
#30233=CARTESIAN_POINT ( 'NONE',  ( 35.00000000000000000, -6.950793414699864670, -10.68873102412840304 ) ) ;
#30234=CYLINDRICAL_SURFACE ( 'NONE', #39620, 12.18649999999999878 ) ;
#30235=CARTESIAN_POINT ( 'NONE',  ( -17.29244623348158783, 2.525873743887551814, 11.73115347397430597 ) ) ;
#30236=DIRECTION ( 'NONE',  ( 0.9996161839461982224, 0.02770351589312032917, -0.000000000000000000 ) ) ;
#30238=VECTOR ( 'NONE', #32530, 1000.000000000000000 ) ;
#30239=EDGE_CURVE ( 'NONE', #38324, #39393, #49914, .T. ) ;
#30241=VERTEX_POINT ( 'NONE', #54874 ) ;
#30242=CARTESIAN_POINT ( 'NONE',  ( -35.00000000000000000, -10.91536515067645041, -4.339012074900068683 ) ) ;
#30243=AXIS2_PLACEMENT_3D ( 'NONE', #34407, #23798, #64330 ) ;
#30244=CARTESIAN_POINT ( 'NONE',  ( -35.00000000000000000, 0.000000000000000000, 0.000000000000000000 ) ) ;
#30248=ORIENTED_EDGE ( 'NONE', *, *, #22215, .T. ) ;
#30249=LINE ( 'NONE', #60494, #59897 ) ;
#30250=DIRECTION ( 'NONE',  ( 0.000000000000000000, -0.01356324068817999114, 0.9999080150203989437 ) ) ;
#30251=CARTESIAN_POINT ( 'NONE',  ( -37.00000000000000711, 5.672855678558835102, -10.28547182238001767 ) ) ;
#30252=CARTESIAN_POINT ( 'NONE',  ( 4.200159495149293321, -10.86999738484834666, 5.085916799879192318 ) ) ;
#30253=ORIENTED_EDGE ( 'NONE', *, *, #44004, .T. ) ;
#30257=VERTEX_POINT ( 'NONE', #61172 ) ;
#30260=ORIENTED_EDGE ( 'NONE', *, *, #17751, .F. ) ;
#30262=LINE ( 'NONE', #25261, #4412 ) ;
#30264=AXIS2_PLACEMENT_3D ( 'NONE', #32697, #20865, #41133 ) ;
#30265=CARTESIAN_POINT ( 'NONE',  ( 37.00000000000000711, 4.705694406421931860E-17, -3.469127814946512892E-15 ) ) ;
#30266=CARTESIAN_POINT ( 'NONE',  ( -35.00000000000000000, 0.000000000000000000, 0.000000000000000000 ) ) ;
#30271=DIRECTION ( 'NONE',  ( 0.000000000000000000, 0.01356324068817998940, -0.9999080150203989437 ) ) ;
#30273=CIRCLE ( 'NONE', #36630, 12.74999999999999822 ) ;
#30274=VERTEX_POINT ( 'NONE', #63360 ) ;
#30275=CYLINDRICAL_SURFACE ( 'NONE', #1010, 4.999999999999999112 ) ;
#30276=CARTESIAN_POINT ( 'NONE',  ( -35.00000000000000000, 0.000000000000000000, 0.000000000000000000 ) ) ;
#30277=CARTESIAN_POINT ( 'NONE',  ( 35.00000000000000000, 3.287724142101414504, -11.73463472867577373 ) ) ;
#30282=AXIS2_PLACEMENT_3D ( 'NONE', #52229, #15323, #35596 ) ;
#30285=CARTESIAN_POINT ( 'NONE',  ( 36.00000000000000711, 10.23119532541072552, -7.608228585767763619 ) ) ;
#30287=EDGE_CURVE ( 'NONE', #59819, #59561, #26569, .T. ) ;
#30289=DIRECTION ( 'NONE',  ( -1.000000000000000000, 0.000000000000000000, -0.000000000000000000 ) ) ;
#30295=AXIS2_PLACEMENT_3D ( 'NONE', #46358, #60325, #20096 ) ;
#30299=LINE ( 'NONE', #50595, #12865 ) ;
#30302=CIRCLE ( 'NONE', #55801, 12.75000000000000178 ) ;
#30303=ADVANCED_FACE ( 'NONE', ( #51857 ), #27800, .T. ) ;
#30305=VERTEX_POINT ( 'NONE', #56171 ) ;
#30308=EDGE_CURVE ( 'NONE', #60184, #817, #15603, .T. ) ;
#30309=ORIENTED_EDGE ( 'NONE', *, *, #43234, .F. ) ;
#30310=DIRECTION ( 'NONE',  ( 0.000000000000000000, -1.000000000000000000, 0.000000000000000000 ) ) ;
#30314=EDGE_LOOP ( 'NONE', ( #52332, #7154, #46442, #58696 ) ) ;
#30315=EDGE_CURVE ( 'NONE', #40551, #55012, #63462, .T. ) ;
#30316=ORIENTED_EDGE ( 'NONE', *, *, #16439, .F. ) ;
#30317=VERTEX_POINT ( 'NONE', #48102 ) ;
#30321=DIRECTION ( 'NONE',  ( 1.000000000000000000, 0.000000000000000000, 0.000000000000000000 ) ) ;
#30322=CYLINDRICAL_SURFACE ( 'NONE', #34670, 5.000000000000000888 ) ;
#30324=ORIENTED_EDGE ( 'NONE', *, *, #59320, .T. ) ;
#30325=VECTOR ( 'NONE', #54174, 1000.000000000000000 ) ;
#30330=VERTEX_POINT ( 'NONE', #41198 ) ;
#30331=DIRECTION ( 'NONE',  ( 0.000000000000000000, -1.000000000000000000, 0.000000000000000000 ) ) ;
#30332=EDGE_CURVE ( 'NONE', #48986, #56955, #35875, .T. ) ;
#30333=ORIENTED_EDGE ( 'NONE', *, *, #22697, .F. ) ;
#30334=DIRECTION ( 'NONE',  ( -1.000000000000000000, 0.000000000000000000, -0.000000000000000000 ) ) ;
#30335=ORIENTED_EDGE ( 'NONE', *, *, #59834, .T. ) ;
#30336=LINE ( 'NONE', #50628, #59240 ) ;
#30337=CARTESIAN_POINT ( 'NONE',  ( -35.00000000000000000, 0.000000000000000000, 0.000000000000000000 ) ) ;
#30339=AXIS2_PLACEMENT_3D ( 'NONE', #58391, #12816, #48428 ) ;
#30341=FACE_OUTER_BOUND ( 'NONE', #6114, .T. ) ;
#30342=DIRECTION ( 'NONE',  ( 0.000000000000000000, -0.9937233664769772323, 0.1118654143051511785 ) ) ;
#30343=CARTESIAN_POINT ( 'NONE',  ( -35.00000000000000000, -10.28547182238004076, -5.672855678558794246 ) ) ;
#30345=DIRECTION ( 'NONE',  ( -1.000000000000000000, 0.000000000000000000, 0.000000000000000000 ) ) ;
#30346=CYLINDRICAL_SURFACE ( 'NONE', #30060, 5.000000000000000888 ) ;
#30347=CARTESIAN_POINT ( 'NONE',  ( -18.58686583997218733, 4.908862989891756179, -12.57862506157752236 ) ) ;
#30349=DIRECTION ( 'NONE',  ( 0.000000000000000000, 0.9467777615094583599, 0.3218879778915939571 ) ) ;
#30351=CARTESIAN_POINT ( 'NONE',  ( 11.66906220897710433, -13.41085082018220298, -1.554662609128065975 ) ) ;
#30352=ORIENTED_EDGE ( 'NONE', *, *, #12684, .F. ) ;
#30358=EDGE_CURVE ( 'NONE', #53925, #14785, #62411, .T. ) ;
#30362=EDGE_CURVE ( 'NONE', #11339, #59141, #51814, .T. ) ;
#30363=EDGE_LOOP ( 'NONE', ( #46501, #30716, #39310, #18416 ) ) ;
#30364=DIRECTION ( 'NONE',  ( 0.000000000000000000, 0.4935949184179201366, -0.8696919319575218132 ) ) ;
#30365=DIRECTION ( 'NONE',  ( 0.000000000000000000, -0.01356324068817998073, 0.9999080150203990547 ) ) ;
#30367=ORIENTED_EDGE ( 'NONE', *, *, #9649, .F. ) ;
#30369=ADVANCED_FACE ( 'NONE', ( #26252 ), #46526, .T. ) ;
#30370=AXIS2_PLACEMENT_3D ( 'NONE', #61905, #1066, #36635 ) ;
#30371=DIRECTION ( 'NONE',  ( 0.000000000000000000, -0.01356324068818685717, 0.9999080150203989437 ) ) ;
#30374=CARTESIAN_POINT ( 'NONE',  ( -35.00000000000000000, 0.000000000000000000, 0.000000000000000000 ) ) ;
#30376=CARTESIAN_POINT ( 'NONE',  ( 3.940939162714027333, 6.015482101771779888, 10.38582757690980785 ) ) ;
#30377=CIRCLE ( 'NONE', #59074, 12.18650000000000055 ) ;
#30378=CARTESIAN_POINT ( 'NONE',  ( 47.00000000000000711, 4.705694406421931860E-17, -3.469127814946512892E-15 ) ) ;
#30379=CARTESIAN_POINT ( 'NONE',  ( 35.00000000000000000, 8.854740511458958352, 7.717887834988148121 ) ) ;
#30380=EDGE_CURVE ( 'NONE', #24055, #7923, #54061, .T. ) ;
#30381=ORIENTED_EDGE ( 'NONE', *, *, #28080, .F. ) ;
#30386=CARTESIAN_POINT ( 'NONE',  ( 10.39737752511405056, 0.7512156450559613896, 13.48016586525701932 ) ) ;
#30387=DIRECTION ( 'NONE',  ( -1.000000000000000000, -0.000000000000000000, 0.000000000000000000 ) ) ;
#30388=ORIENTED_EDGE ( 'NONE', *, *, #40007, .F. ) ;
#30390=VERTEX_POINT ( 'NONE', #34426 ) ;
#30391=ADVANCED_FACE ( 'NONE', ( #48752 ), #3204, .T. ) ;
#30392=ORIENTED_EDGE ( 'NONE', *, *, #51147, .T. ) ;
#30393=DIRECTION ( 'NONE',  ( 1.000000000000000000, 0.000000000000000000, -0.000000000000000000 ) ) ;
#30394=DIRECTION ( 'NONE',  ( 1.000000000000000000, 0.000000000000000000, 0.000000000000000000 ) ) ;
#30395=DIRECTION ( 'NONE',  ( 0.000000000000000000, 0.01356324068817998940, -0.9999080150203989437 ) ) ;
#30397=CARTESIAN_POINT ( 'NONE',  ( 22.57855258442564761, -4.427776684447072952, -11.15324139578564910 ) ) ;
#30399=CARTESIAN_POINT ( 'NONE',  ( 23.19604530331957903, -4.580399580743265808, -12.70184690977379383 ) ) ;
#30400=CYLINDRICAL_SURFACE ( 'NONE', #47, 14.69297241773857188 ) ;
#30404=ORIENTED_EDGE ( 'NONE', *, *, #23826, .T. ) ;
#30412=DIRECTION ( 'NONE',  ( -1.000000000000000000, 0.000000000000000000, 0.000000000000000000 ) ) ;
#30413=AXIS2_PLACEMENT_3D ( 'NONE', #38406, #23446, #2858 ) ;
#30414=CARTESIAN_POINT ( 'NONE',  ( -19.16415376008873750, 11.99999999999999822, -0.3279367020959012557 ) ) ;
#30415=DIRECTION ( 'NONE',  ( 0.000000000000000000, -0.9970832820307030664, -0.07632122047557567124 ) ) ;
#30416=ORIENTED_EDGE ( 'NONE', *, *, #11188, .F. ) ;
#30417=AXIS2_PLACEMENT_3D ( 'NONE', #20314, #14983, #65214 ) ;
#30418=ORIENTED_EDGE ( 'NONE', *, *, #35696, .F. ) ;
#30419=DIRECTION ( 'NONE',  ( 1.000000000000000000, 0.000000000000000000, 0.000000000000000000 ) ) ;
#30422=CARTESIAN_POINT ( 'NONE',  ( 37.00000000000000711, -9.896810808925339487, 7.110831038798382409 ) ) ;
#30424=CARTESIAN_POINT ( 'NONE',  ( 35.00000000000000000, -2.527899948230725613, -12.49688848680883346 ) ) ;
#30425=CARTESIAN_POINT ( 'NONE',  ( 16.78263030916553333, -10.48479066935623827, 5.836879698929882565 ) ) ;
#30428=CARTESIAN_POINT ( 'NONE',  ( -8.377090426847601634, -1.945797233010116312, -11.84431829273728098 ) ) ;
#30429=CARTESIAN_POINT ( 'NONE',  ( 27.08396654187716024, -12.95140485128378138, 3.821959039601221075 ) ) ;
#30430=VERTEX_POINT ( 'NONE', #54404 ) ;
#30431=ORIENTED_EDGE ( 'NONE', *, *, #1469, .F. ) ;
#30432=CYLINDRICAL_SURFACE ( 'NONE', #4163, 12.18650000000000055 ) ;
#30437=LINE ( 'NONE', #56724, #4580 ) ;
#30438=CARTESIAN_POINT ( 'NONE',  ( 23.11736814598171108, 2.555106763338435893, -13.25897843685541844 ) ) ;
#30440=CARTESIAN_POINT ( 'NONE',  ( -37.00000000000000711, 8.052525312710004712, -8.551552972816995890 ) ) ;
#30441=EDGE_LOOP ( 'NONE', ( #3761, #36583, #65550, #55854 ) ) ;
#30445=VECTOR ( 'NONE', #62877, 1000.000000000000000 ) ;
#30449=EDGE_CURVE ( 'NONE', #64737, #6776, #55029, .T. ) ;
#30451=CARTESIAN_POINT ( 'NONE',  ( -17.28371300127619037, -6.351468865812872622, -11.91715882903726076 ) ) ;
#30454=VERTEX_POINT ( 'NONE', #28781 ) ;
#30455=EDGE_CURVE ( 'NONE', #45140, #786, #42226, .T. ) ;
#30457=DIRECTION ( 'NONE',  ( 0.000000000000000000, 0.6269146997507986097, 0.7790879021242506086 ) ) ;
#30459=CYLINDRICAL_SURFACE ( 'NONE', #14790, 12.74999999999999822 ) ;
#30464=VERTEX_POINT ( 'NONE', #29430 ) ;
#30468=CARTESIAN_POINT ( 'NONE',  ( 23.10852454909521470, -3.964659581577253178, -11.32972118890850943 ) ) ;
#30469=CARTESIAN_POINT ( 'NONE',  ( 37.00000000000000711, -11.72195762423410414, -0.7536123767498126291 ) ) ;
#30470=CARTESIAN_POINT ( 'NONE',  ( -35.00000000000000000, 11.47561260193584687, -5.556331110570288168 ) ) ;
#30471=FACE_OUTER_BOUND ( 'NONE', #664, .T. ) ;
#30473=ORIENTED_EDGE ( 'NONE', *, *, #62763, .T. ) ;
#30474=CARTESIAN_POINT ( 'NONE',  ( -10.90165637462999726, -7.508992741355383416, 25.00000000000000000 ) ) ;
#30476=DIRECTION ( 'NONE',  ( -1.000000000000000000, 0.000000000000000000, 0.000000000000000000 ) ) ;
#30478=ADVANCED_FACE ( 'NONE', ( #44384 ), #43405, .T. ) ;
#30482=CARTESIAN_POINT ( 'NONE',  ( -35.00000000000000000, 8.017674001891920810, -9.913596905230031453 ) ) ;
#30485=ORIENTED_EDGE ( 'NONE', *, *, #41950, .F. ) ;
#30488=ORIENTED_EDGE ( 'NONE', *, *, #1284, .F. ) ;
#30490=AXIS2_PLACEMENT_3D ( 'NONE', #4259, #33202, #18601 ) ;
#30491=DIRECTION ( 'NONE',  ( 1.000000000000000000, 0.000000000000000000, 0.000000000000000000 ) ) ;
#30493=FACE_OUTER_BOUND ( 'NONE', #18726, .T. ) ;
#30495=DIRECTION ( 'NONE',  ( 0.4622435816439414147, -0.000000000000000000, 0.8867529933577789070 ) ) ;
#30496=AXIS2_PLACEMENT_3D ( 'NONE', #46434, #62692, #11194 ) ;
#30497=LINE ( 'NONE', #5243, #51405 ) ;
#30498=ORIENTED_EDGE ( 'NONE', *, *, #8853, .F. ) ;
#30499=DIRECTION ( 'NONE',  ( -1.000000000000000000, 0.000000000000000000, -0.000000000000000000 ) ) ;
#30500=DIRECTION ( 'NONE',  ( 0.000000000000000000, -0.8696919319575131535, -0.4935949184179356797 ) ) ;
#30502=CARTESIAN_POINT ( 'NONE',  ( 12.70623083740922432, 11.80103865657056872, -6.559203751279317096 ) ) ;
#30504=LINE ( 'NONE', #9552, #27675 ) ;
#30505=CARTESIAN_POINT ( 'NONE',  ( 35.00000000000000000, -6.891188680298889757, -9.512294188640879611 ) ) ;
#30506=LINE ( 'NONE', #39838, #51238 ) ;
#30507=EDGE_CURVE ( 'NONE', #50026, #27033, #9302, .T. ) ;
#30508=ORIENTED_EDGE ( 'NONE', *, *, #16371, .T. ) ;
#30509=CARTESIAN_POINT ( 'NONE',  ( -37.00000000000000711, -12.63095688309030429, 1.738225594539952068 ) ) ;
#30510=VERTEX_POINT ( 'NONE', #59067 ) ;
#30511=CARTESIAN_POINT ( 'NONE',  ( -3.303901569720309350, -7.697936092459741531, 9.214473394900021930 ) ) ;
#30518=CARTESIAN_POINT ( 'NONE',  ( -30.18541646480307250, -1.815008380980587699, -11.86874821329540630 ) ) ;
#30522=EDGE_CURVE ( 'NONE', #56863, #63134, #31610, .T. ) ;
#30523=CARTESIAN_POINT ( 'NONE',  ( -18.47557885490082796, -4.422014522762156119, 11.15615431079476672 ) ) ;
#30524=CARTESIAN_POINT ( 'NONE',  ( -35.00000000000000000, 10.49626516989271074, 7.238157050195666464 ) ) ;
#30525=ORIENTED_EDGE ( 'NONE', *, *, #23684, .T. ) ;
#30526=EDGE_CURVE ( 'NONE', #27983, #60081, #11449, .T. ) ;
#30527=CARTESIAN_POINT ( 'NONE',  ( -37.00000000000000711, -9.896810808925444292, 7.110831038798244741 ) ) ;
#30528=ORIENTED_EDGE ( 'NONE', *, *, #15773, .F. ) ;
#30530=DIRECTION ( 'NONE',  ( 0.000000000000000000, -0.01356324068817998940, 0.9999080150203990547 ) ) ;
#30535=ORIENTED_EDGE ( 'NONE', *, *, #25616, .F. ) ;
#30537=EDGE_CURVE ( 'NONE', #2479, #58998, #29746, .T. ) ;
#30540=ORIENTED_EDGE ( 'NONE', *, *, #65162, .T. ) ;
#30541=DIRECTION ( 'NONE',  ( 0.000000000000000000, -0.01356324068817998940, 0.9999080150203990547 ) ) ;
#30542=CARTESIAN_POINT ( 'NONE',  ( 8.621148270653568702, 25.00000000000000000, -5.251012286260225537 ) ) ;
#30551=ORIENTED_EDGE ( 'NONE', *, *, #63178, .T. ) ;
#30555=EDGE_CURVE ( 'NONE', #32620, #2528, #45065, .T. ) ;
#30556=FACE_BOUND ( 'NONE', #38319, .T. ) ;
#30559=CARTESIAN_POINT ( 'NONE',  ( 6.776769869547749181, -5.711596899239616221, -12.23794304267072874 ) ) ;
#30560=DIRECTION ( 'NONE',  ( 0.000000000000000000, -0.5987040770935562195, 0.8009703041134252910 ) ) ;
#30561=CARTESIAN_POINT ( 'NONE',  ( 5.258427716898767201, -10.28439498637095006, 6.186120577954387301 ) ) ;
#30562=EDGE_LOOP ( 'NONE', ( #5720, #6278, #25586, #17008 ) ) ;
#30563=ORIENTED_EDGE ( 'NONE', *, *, #5702, .F. ) ;
#30566=ORIENTED_EDGE ( 'NONE', *, *, #15979, .T. ) ;
#30567=DIRECTION ( 'NONE',  ( 1.000000000000000000, 0.000000000000000000, 0.000000000000000000 ) ) ;
#30568=ORIENTED_EDGE ( 'NONE', *, *, #51138, .T. ) ;
#30569=ORIENTED_EDGE ( 'NONE', *, *, #46763, .T. ) ;
#30570=ORIENTED_EDGE ( 'NONE', *, *, #36785, .T. ) ;
#30573=DIRECTION ( 'NONE',  ( 0.000000000000000000, 0.01356324068817998940, -0.9999080150203990547 ) ) ;
#30575=FACE_OUTER_BOUND ( 'NONE', #169, .T. ) ;
#30580=CARTESIAN_POINT ( 'NONE',  ( 35.00000000000000000, 4.705694406421931860E-17, -3.469127814946512892E-15 ) ) ;
#30581=AXIS2_PLACEMENT_3D ( 'NONE', #45311, #25041, #9385 ) ;
#30583=LINE ( 'NONE', #50888, #10521 ) ;
#30584=CARTESIAN_POINT ( 'NONE',  ( 29.10170639864063702, 8.929942550509162302, 8.028710125001698117 ) ) ;
#30586=AXIS2_PLACEMENT_3D ( 'NONE', #35970, #6085, #53176 ) ;
#30587=EDGE_CURVE ( 'NONE', #42316, #11282, #36930, .T. ) ;
#30588=EDGE_CURVE ( 'NONE', #63500, #56480, #41365, .T. ) ;
#30589=ORIENTED_EDGE ( 'NONE', *, *, #35288, .T. ) ;
#30591=VERTEX_POINT ( 'NONE', #36394 ) ;
#30594=CYLINDRICAL_SURFACE ( 'NONE', #62746, 4.999999999999999112 ) ;
#30598=LINE ( 'NONE', #697, #2739 ) ;
#30599=DIRECTION ( 'NONE',  ( 1.000000000000000000, 0.000000000000000000, 0.000000000000000000 ) ) ;
#30600=DIRECTION ( 'NONE',  ( 0.000000000000000000, 0.01356324068817998940, -0.9999080150203990547 ) ) ;
#30601=CARTESIAN_POINT ( 'NONE',  ( 22.27688490018784506, -12.54606834907711210, -4.987630095507642913 ) ) ;
#30602=EDGE_CURVE ( 'NONE', #58290, #26820, #15116, .T. ) ;
#30610=ORIENTED_EDGE ( 'NONE', *, *, #816, .T. ) ;
#30612=ORIENTED_EDGE ( 'NONE', *, *, #18300, .T. ) ;
#30616=ADVANCED_FACE ( 'NONE', ( #60344 ), #14769, .T. ) ;
#30618=ORIENTED_EDGE ( 'NONE', *, *, #7823, .F. ) ;
#30619=ADVANCED_FACE ( 'NONE', ( #51043 ), #10140, .T. ) ;
#30620=ORIENTED_EDGE ( 'NONE', *, *, #54370, .T. ) ;
#30622=ORIENTED_EDGE ( 'NONE', *, *, #24013, .T. ) ;
#30624=EDGE_CURVE ( 'NONE', #7430, #25248, #6207, .T. ) ;
#30625=CARTESIAN_POINT ( 'NONE',  ( 37.00000000000000711, -1.286231064351218478, 12.68495603654572612 ) ) ;
#30626=ORIENTED_EDGE ( 'NONE', *, *, #39526, .T. ) ;
#30627=EDGE_CURVE ( 'NONE', #27370, #1032, #2992, .T. ) ;
#30628=DIRECTION ( 'NONE',  ( 0.000000000000000000, 0.01356324068817992175, -0.9999080150203990547 ) ) ;
#30630=ORIENTED_EDGE ( 'NONE', *, *, #54628, .F. ) ;
#30631=DIRECTION ( 'NONE',  ( 0.8751623310228197061, 0.000000000000000000, -0.4838294062566934617 ) ) ;
#30633=CARTESIAN_POINT ( 'NONE',  ( 35.00000000000000000, 10.30098186818249673, -5.644643009979106729 ) ) ;
#30634=ORIENTED_EDGE ( 'NONE', *, *, #36881, .F. ) ;
#30636=DIRECTION ( 'NONE',  ( 0.000000000000000000, 0.01356324068817992175, -0.9999080150203990547 ) ) ;
#30638=FACE_OUTER_BOUND ( 'NONE', #59299, .T. ) ;
#30639=ORIENTED_EDGE ( 'NONE', *, *, #34886, .T. ) ;
#30644=DIRECTION ( 'NONE',  ( 0.000000000000000000, -0.01356324068817991828, 0.9999080150203990547 ) ) ;
#30647=DIRECTION ( 'NONE',  ( -1.000000000000000000, 0.000000000000000000, 0.000000000000000000 ) ) ;
#30648=CARTESIAN_POINT ( 'NONE',  ( 6.812204945636112896, -4.138731716409435712, 12.84993773446340803 ) ) ;
#30655=DIRECTION ( 'NONE',  ( 0.000000000000000000, 0.01356324068818000848, -0.9999080150203990547 ) ) ;
#30661=LINE ( 'NONE', #29679, #32701 ) ;
#30663=EDGE_CURVE ( 'NONE', #44780, #65264, #42238, .T. ) ;
#30664=VERTEX_POINT ( 'NONE', #42664 ) ;
#30665=CARTESIAN_POINT ( 'NONE',  ( -18.11037611196539387, -4.786480602738535595, -11.00804596661986068 ) ) ;
#30667=AXIS2_PLACEMENT_3D ( 'NONE', #14407, #34684, #24736 ) ;
#30668=( BOUNDED_CURVE ( )  B_SPLINE_CURVE ( 3, ( #32357, #2458, #57661, #52669 ),
 .UNSPECIFIED., .F., .F. ) 
 B_SPLINE_CURVE_WITH_KNOTS ( ( 4, 4 ),
 ( 4.675538416354898530, 4.712388980384690562 ),
 .UNSPECIFIED. ) 
 CURVE ( )  GEOMETRIC_REPRESENTATION_ITEM ( )  RATIONAL_B_SPLINE_CURVE ( ( 1.000000000000000000, 0.9998868395290251287, 0.9998868395290251287, 1.000000000000000000 ) ) 
 REPRESENTATION_ITEM ( '' )  );
#30669=ORIENTED_EDGE ( 'NONE', *, *, #37443, .F. ) ;
#30672=VECTOR ( 'NONE', #64128, 1000.000000000000000 ) ;
#30674=ORIENTED_EDGE ( 'NONE', *, *, #45102, .T. ) ;
#30675=EDGE_CURVE ( 'NONE', #42736, #57376, #43349, .T. ) ;
#30676=CARTESIAN_POINT ( 'NONE',  ( 35.00000000000000000, 11.96656215839374759, 4.400442035670817376 ) ) ;
#30680=ADVANCED_FACE ( 'NONE', ( #36719 ), #6468, .T. ) ;
#30681=ORIENTED_EDGE ( 'NONE', *, *, #50744, .T. ) ;
#30682=CARTESIAN_POINT ( 'NONE',  ( 35.00000000000000000, 11.70009620280413110, 1.039216533672774112 ) ) ;
#30683=CARTESIAN_POINT ( 'NONE',  ( -37.00000000000000711, 2.346765782874606465, -11.95840593935198903 ) ) ;
#30686=AXIS2_PLACEMENT_3D ( 'NONE', #32882, #32241, #32551 ) ;
#30687=DIRECTION ( 'NONE',  ( 1.000000000000000000, 0.000000000000000000, 0.000000000000000000 ) ) ;
#30688=DIRECTION ( 'NONE',  ( 1.000000000000000000, 0.000000000000000000, -0.000000000000000000 ) ) ;
#30689=ORIENTED_EDGE ( 'NONE', *, *, #58148, .T. ) ;
#30690=CARTESIAN_POINT ( 'NONE',  ( -37.00000000000000711, -11.73555825188280011, 4.983891302653540301 ) ) ;
#30691=LINE ( 'NONE', #51671, #42743 ) ;
#30692=CARTESIAN_POINT ( 'NONE',  ( 35.00000000000000000, 11.74614673114903773, 0.01609748574448878478 ) ) ;
#30693=ORIENTED_EDGE ( 'NONE', *, *, #44218, .T. ) ;
#30695=CARTESIAN_POINT ( 'NONE',  ( -27.45775109278351067, -8.499184579339635448, -8.471355351200609007 ) ) ;
#30697=ORIENTED_EDGE ( 'NONE', *, *, #39857, .F. ) ;
#30698=EDGE_LOOP ( 'NONE', ( #47745, #49554, #53595, #60828 ) ) ;
#30701=CIRCLE ( 'NONE', #2057, 5.000000000000000888 ) ;
#30702=ORIENTED_EDGE ( 'NONE', *, *, #53555, .T. ) ;
#30706=AXIS2_PLACEMENT_3D ( 'NONE', #28576, #48879, #45181 ) ;
#30711=CARTESIAN_POINT ( 'NONE',  ( 12.10998784662220729, -10.46621227226782835, -8.526922110106905706 ) ) ;
#30714=EDGE_CURVE ( 'NONE', #12400, #2234, #25273, .T. ) ;
#30716=ORIENTED_EDGE ( 'NONE', *, *, #170, .F. ) ;
#30718=VERTEX_POINT ( 'NONE', #16759 ) ;
#30721=CARTESIAN_POINT ( 'NONE',  ( -37.00000000000000711, 0.000000000000000000, 0.000000000000000000 ) ) ;
#30723=FACE_OUTER_BOUND ( 'NONE', #36201, .T. ) ;
#30724=CARTESIAN_POINT ( 'NONE',  ( 35.00000000000000000, 4.705694406421931860E-17, -3.469127814946512892E-15 ) ) ;
#30725=ADVANCED_FACE ( 'NONE', ( #57019 ), #46696, .F. ) ;
#30728=AXIS2_PLACEMENT_3D ( 'NONE', #24631, #13987, #34594 ) ;
#30729=ORIENTED_EDGE ( 'NONE', *, *, #22453, .T. ) ;
#30732=ORIENTED_EDGE ( 'NONE', *, *, #53413, .F. ) ;
#30733=ORIENTED_EDGE ( 'NONE', *, *, #16731, .T. ) ;
#30734=LINE ( 'NONE', #60348, #17953 ) ;
#30735=DIRECTION ( 'NONE',  ( 0.000000000000000000, 0.01356324068817998940, -0.9999080150203990547 ) ) ;
#30739=DIRECTION ( 'NONE',  ( -1.000000000000000000, 0.000000000000000000, 0.000000000000000000 ) ) ;
#30740=CIRCLE ( 'NONE', #12694, 4.999999999999999112 ) ;
#30741=EDGE_CURVE ( 'NONE', #19851, #34326, #37367, .T. ) ;
#30742=ORIENTED_EDGE ( 'NONE', *, *, #7007, .F. ) ;
#30743=AXIS2_PLACEMENT_3D ( 'NONE', #57941, #12354, #22688 ) ;
#30744=ORIENTED_EDGE ( 'NONE', *, *, #55133, .T. ) ;
#30745=CARTESIAN_POINT ( 'NONE',  ( -35.00000000000000000, 9.063649021439076137, -8.146229107149299153 ) ) ;
#30747=VECTOR ( 'NONE', #42064, 1000.000000000000000 ) ;
#30748=CARTESIAN_POINT ( 'NONE',  ( 4.190943541829291519, -10.32976040564048681, 6.108679903397304045 ) ) ;
#30749=CARTESIAN_POINT ( 'NONE',  ( -35.00000000000000000, -10.42955799785324444, 6.303578524886909840 ) ) ;
#30751=CARTESIAN_POINT ( 'NONE',  ( -37.00000000000000711, 0.000000000000000000, 0.000000000000000000 ) ) ;
#30754=EDGE_CURVE ( 'NONE', #63926, #30777, #37708, .T. ) ;
#30758=CARTESIAN_POINT ( 'NONE',  ( -37.00000000000000711, 0.000000000000000000, 0.000000000000000000 ) ) ;
#30759=VECTOR ( 'NONE', #62454, 1000.000000000000000 ) ;
#30762=CARTESIAN_POINT ( 'NONE',  ( 37.00000000000000711, 12.73293890771483916, 0.6593684648219071409 ) ) ;
#30763=ORIENTED_EDGE ( 'NONE', *, *, #15701, .T. ) ;
#30765=CARTESIAN_POINT ( 'NONE',  ( 37.00000000000000711, -0.9416912585475287756, -12.71517666308947625 ) ) ;
#30770=CARTESIAN_POINT ( 'NONE',  ( 35.00000000000000000, 4.705694406421931860E-17, -3.469127814946512892E-15 ) ) ;
#30772=ORIENTED_EDGE ( 'NONE', *, *, #14048, .T. ) ;
#30774=EDGE_CURVE ( 'NONE', #1623, #46377, #63609, .T. ) ;
#30777=VERTEX_POINT ( 'NONE', #54662 ) ;
#30778=DIRECTION ( 'NONE',  ( 1.000000000000000000, 0.000000000000000000, -0.000000000000000000 ) ) ;
#30779=CARTESIAN_POINT ( 'NONE',  ( -9.276318581089137538, 12.47567835156090865, -5.170372665552285696 ) ) ;
#30780=DIRECTION ( 'NONE',  ( 0.000000000000000000, -0.01356324068817998940, 0.9999080150203990547 ) ) ;
#30784=FACE_OUTER_BOUND ( 'NONE', #54255, .T. ) ;
#30785=ORIENTED_EDGE ( 'NONE', *, *, #46551, .F. ) ;
#30790=CIRCLE ( 'NONE', #64779, 12.18649999999999878 ) ;
#30791=ADVANCED_FACE ( 'NONE', ( #58322 ), #24366, .F. ) ;
#30793=CYLINDRICAL_SURFACE ( 'NONE', #36209, 12.18649999999999878 ) ;
#30795=ORIENTED_EDGE ( 'NONE', *, *, #28309, .F. ) ;
#30797=CARTESIAN_POINT ( 'NONE',  ( -35.00000000000000000, -9.913596905230058098, -8.017674001891892388 ) ) ;
#30798=FACE_BOUND ( 'NONE', #64375, .T. ) ;
#30799=ORIENTED_EDGE ( 'NONE', *, *, #15601, .F. ) ;
#30800=EDGE_LOOP ( 'NONE', ( #10938, #30895, #35525, #62792 ) ) ;
#30803=AXIS2_PLACEMENT_3D ( 'NONE', #38768, #9719, #43747 ) ;
#30806=DIRECTION ( 'NONE',  ( 0.000000000000000000, -0.01356324068817998940, 0.9999080150203990547 ) ) ;
#30808=CARTESIAN_POINT ( 'NONE',  ( 35.00000000000000000, 11.59095880812004964, -1.903127969211395598 ) ) ;
#30811=VECTOR ( 'NONE', #21160, 1000.000000000000000 ) ;
#30813=ORIENTED_EDGE ( 'NONE', *, *, #14613, .F. ) ;
#30814=DIRECTION ( 'NONE',  ( 0.000000000000000000, 0.2355298848897516562, 0.9718671068226459875 ) ) ;
#30815=EDGE_CURVE ( 'NONE', #65337, #1946, #55032, .T. ) ;
#30816=AXIS2_PLACEMENT_3D ( 'NONE', #59424, #34143, #44440 ) ;
#30817=CARTESIAN_POINT ( 'NONE',  ( 22.12488133644825439, 11.11891314965964561, -4.528710933524925153 ) ) ;
#30818=CARTESIAN_POINT ( 'NONE',  ( -35.00000000000000000, -0.4993900848166508144, -12.17626345777664554 ) ) ;
#30820=DIRECTION ( 'NONE',  ( 0.9318405276259970060, 0.3628680629012471237, 0.000000000000000000 ) ) ;
#30822=DIRECTION ( 'NONE',  ( 0.000000000000000000, -0.01356324068817998940, 0.9999080150203990547 ) ) ;
#30825=CIRCLE ( 'NONE', #39340, 5.000000000000000000 ) ;
#30826=AXIS2_PLACEMENT_3D ( 'NONE', #33636, #16775, #38626 ) ;
#30827=AXIS2_PLACEMENT_3D ( 'NONE', #16688, #25692, #56266 ) ;
#30828=VERTEX_POINT ( 'NONE', #13408 ) ;
#30829=EDGE_CURVE ( 'NONE', #16276, #18362, #44631, .T. ) ;
#30831=CARTESIAN_POINT ( 'NONE',  ( 8.437200413559441614, 4.476360154859203355, 12.73625532737111143 ) ) ;
#30832=ORIENTED_EDGE ( 'NONE', *, *, #27600, .F. ) ;
#30838=ORIENTED_EDGE ( 'NONE', *, *, #35678, .F. ) ;
#30839=FACE_OUTER_BOUND ( 'NONE', #729, .T. ) ;
#30843=AXIS2_PLACEMENT_3D ( 'NONE', #10769, #31389, #52005 ) ;
#30844=AXIS2_PLACEMENT_3D ( 'NONE', #2180, #32733, #1548 ) ;
#30850=AXIS2_PLACEMENT_3D ( 'NONE', #6240, #52118, #36815 ) ;
#30851=CARTESIAN_POINT ( 'NONE',  ( -35.00000000000000000, -4.237620530777717498, -11.42599468261433771 ) ) ;
#30854=DIRECTION ( 'NONE',  ( -1.000000000000000000, 0.000000000000000000, -0.000000000000000000 ) ) ;
#30855=AXIS2_PLACEMENT_3D ( 'NONE', #8344, #48927, #13332 ) ;
#30858=ORIENTED_EDGE ( 'NONE', *, *, #9330, .F. ) ;
#30860=CARTESIAN_POINT ( 'NONE',  ( -29.95627872347045084, 0.8329649216453900440, 11.97914056345418565 ) ) ;
#30864=CARTESIAN_POINT ( 'NONE',  ( -8.891032880924175430, -12.93614229090407974, -3.860857758255645589 ) ) ;
#30866=FACE_OUTER_BOUND ( 'NONE', #26094, .T. ) ;
#30869=CYLINDRICAL_SURFACE ( 'NONE', #38252, 5.000000000000000888 ) ;
#30873=CARTESIAN_POINT ( 'NONE',  ( -9.218674071044169693, -9.592100768695239310, -7.220698992947784056 ) ) ;
#30874=ORIENTED_EDGE ( 'NONE', *, *, #27050, .T. ) ;
#30875=DIRECTION ( 'NONE',  ( 0.000000000000000000, 0.8696919319575165952, 0.4935949184179292404 ) ) ;
#30881=VECTOR ( 'NONE', #32425, 1000.000000000000000 ) ;
#30886=DIRECTION ( 'NONE',  ( 0.000000000000000000, -0.3807014730195085739, 0.9246979985058777496 ) ) ;
#30887=AXIS2_PLACEMENT_3D ( 'NONE', #45716, #50720, #176 ) ;
#30891=ORIENTED_EDGE ( 'NONE', *, *, #35188, .T. ) ;
#30893=ORIENTED_EDGE ( 'NONE', *, *, #22901, .F. ) ;
#30894=DIRECTION ( 'NONE',  ( 1.000000000000000000, 0.000000000000000000, 0.000000000000000000 ) ) ;
#30895=ORIENTED_EDGE ( 'NONE', *, *, #12968, .T. ) ;
#30897=ORIENTED_EDGE ( 'NONE', *, *, #9816, .F. ) ;
#30898=DIRECTION ( 'NONE',  ( -1.000000000000000000, 0.000000000000000000, 0.000000000000000000 ) ) ;
#30900=EDGE_CURVE ( 'NONE', #26984, #23983, #35888, .T. ) ;
#30903=LINE ( 'NONE', #60189, #5867 ) ;
#30904=VERTEX_POINT ( 'NONE', #44009 ) ;
#30905=AXIS2_PLACEMENT_3D ( 'NONE', #6668, #11959, #36904 ) ;
#30906=FACE_OUTER_BOUND ( 'NONE', #40889, .T. ) ;
#30907=CIRCLE ( 'NONE', #16041, 12.18650000000000055 ) ;
#30909=ORIENTED_EDGE ( 'NONE', *, *, #41807, .F. ) ;
#30910=LINE ( 'NONE', #6969, #58270 ) ;
#30911=ADVANCED_FACE ( 'NONE', ( #2813 ), #18428, .T. ) ;
#30912=DIRECTION ( 'NONE',  ( 0.000000000000000000, 0.9903235168508545128, 0.1387779952735854194 ) ) ;
#30913=AXIS2_PLACEMENT_3D ( 'NONE', #30242, #44529, #60488 ) ;
#30914=EDGE_CURVE ( 'NONE', #36353, #15972, #43332, .T. ) ;
#30917=CARTESIAN_POINT ( 'NONE',  ( -35.00000000000000000, 4.400442035671113139, -11.96656215839364457 ) ) ;
#30920=ORIENTED_EDGE ( 'NONE', *, *, #37092, .F. ) ;
#30921=ADVANCED_FACE ( 'NONE', ( #18082 ), #38349, .T. ) ;
#30925=EDGE_CURVE ( 'NONE', #41767, #14897, #47776, .T. ) ;
#30926=CARTESIAN_POINT ( 'NONE',  ( -24.47698661514656848, -11.24106201439485275, 7.478403204343472055 ) ) ;
#30930=VECTOR ( 'NONE', #38394, 1000.000000000000000 ) ;
#30933=DIRECTION ( 'NONE',  ( 1.000000000000000000, 0.000000000000000000, -0.000000000000000000 ) ) ;
#30936=CARTESIAN_POINT ( 'NONE',  ( 21.44973177390235364, 11.47610357474619747, -3.531383847275154864 ) ) ;
#30937=CARTESIAN_POINT ( 'NONE',  ( -35.00000000000000000, 11.99999999999998579, 1.469576158976822172E-15 ) ) ;
#30938=AXIS2_PLACEMENT_3D ( 'NONE', #59838, #60149, #14268 ) ;
#30939=VECTOR ( 'NONE', #54009, 1000.000000000000000 ) ;
#30940=AXIS2_PLACEMENT_3D ( 'NONE', #2160, #37400, #52716 ) ;
#30941=EDGE_CURVE ( 'NONE', #64485, #42804, #1925, .T. ) ;
#30942=CARTESIAN_POINT ( 'NONE',  ( -35.00000000000000000, -4.732539170486343316, 11.23004253107762906 ) ) ;
#30945=FACE_OUTER_BOUND ( 'NONE', #54579, .T. ) ;
#30947=B_SPLINE_CURVE_WITH_KNOTS ( 'NONE', 3,
 ( #46303, #11048, #40303, #45972, #60595, #742, #41284, #50639, #15035, #25347, #40972, #51628, #46614, #55628, #10372, #1070, #45625, #20362, #40642, #30648 ),
 .UNSPECIFIED., .F., .F.,
 ( 4, 2, 2, 2, 2, 2, 2, 2, 2, 4 ),
 ( 1.939479807224432123E-18, 0.001283480623487103997, 0.001925220935230654044, 0.002566961246974203657, 0.003850441870461304619, 0.005133922493948405580, 0.006417403117435506107, 0.007700883740922607502, 0.008984364364409708897, 0.01026784498789680942 ),
 .UNSPECIFIED. ) ;
#30949=CIRCLE ( 'NONE', #4392, 5.000000000000001776 ) ;
#30950=ORIENTED_EDGE ( 'NONE', *, *, #30741, .T. ) ;
#30951=ORIENTED_EDGE ( 'NONE', *, *, #11104, .F. ) ;
#30953=FACE_OUTER_BOUND ( 'NONE', #15345, .T. ) ;
#30954=AXIS2_PLACEMENT_3D ( 'NONE', #15435, #35703, #60664 ) ;
#30955=CARTESIAN_POINT ( 'NONE',  ( 47.00000000000000711, 4.705694406421931860E-17, -3.469127814946512892E-15 ) ) ;
#30956=VERTEX_POINT ( 'NONE', #34979 ) ;
#30958=ORIENTED_EDGE ( 'NONE', *, *, #2018, .F. ) ;
#30960=EDGE_CURVE ( 'NONE', #8976, #1587, #49731, .T. ) ;
#30961=DIRECTION ( 'NONE',  ( 0.000000000000000000, -0.01356324068817998940, 0.9999080150203990547 ) ) ;
#30963=CARTESIAN_POINT ( 'NONE',  ( 35.00000000000000000, 9.752226076388984310, 6.547236723513913503 ) ) ;
#30965=DIRECTION ( 'NONE',  ( 0.000000000000000000, -0.01356324068817992001, 0.9999080150203990547 ) ) ;
#30966=ORIENTED_EDGE ( 'NONE', *, *, #60909, .T. ) ;
#30970=CYLINDRICAL_SURFACE ( 'NONE', #1640, 13.50000000000000178 ) ;
#30972=CIRCLE ( 'NONE', #39466, 12.18650000000000233 ) ;
#30974=AXIS2_PLACEMENT_3D ( 'NONE', #2440, #2090, #53638 ) ;
#30977=ORIENTED_EDGE ( 'NONE', *, *, #6981, .T. ) ;
#30980=CARTESIAN_POINT ( 'NONE',  ( -35.00000000000000000, 0.000000000000000000, 0.000000000000000000 ) ) ;
#30981=CARTESIAN_POINT ( 'NONE',  ( -35.00000000000000000, -2.936739658819952581, 11.37311665002362560 ) ) ;
#30982=FACE_OUTER_BOUND ( 'NONE', #65709, .T. ) ;
#30984=CIRCLE ( 'NONE', #35190, 5.000000000000000000 ) ;
#30985=DIRECTION ( 'NONE',  ( -1.000000000000000000, 0.000000000000000000, -0.000000000000000000 ) ) ;
#30986=AXIS2_PLACEMENT_3D ( 'NONE', #19093, #34689, #64958 ) ;
#30987=ADVANCED_FACE ( 'NONE', ( #5089 ), #10705, .T. ) ;
#30988=CARTESIAN_POINT ( 'NONE',  ( -35.00000000000000000, 11.05394794832836780, -5.130401251914613603 ) ) ;
#30989=CARTESIAN_POINT ( 'NONE',  ( 35.00000000000000000, -3.827046518385000429, 11.56998259273181162 ) ) ;
#30991=DIRECTION ( 'NONE',  ( 1.000000000000000000, 0.000000000000000000, -0.000000000000000000 ) ) ;
#30992=EDGE_LOOP ( 'NONE', ( #34084, #28635, #20714, #58802 ) ) ;
#30995=CARTESIAN_POINT ( 'NONE',  ( 12.29669898719158638, -13.32434165500316148, -2.178069250421873715 ) ) ;
#30996=EDGE_CURVE ( 'NONE', #16803, #29123, #19401, .T. ) ;
#30997=FACE_OUTER_BOUND ( 'NONE', #50947, .T. ) ;
#30998=EDGE_CURVE ( 'NONE', #18081, #65768, #65572, .T. ) ;
#30999=VERTEX_POINT ( 'NONE', #26023 ) ;
#31002=CARTESIAN_POINT ( 'NONE',  ( 37.00000000000000711, 4.705694406421931860E-17, -3.469127814946512892E-15 ) ) ;
#31003=CYLINDRICAL_SURFACE ( 'NONE', #64557, 12.75000000000000178 ) ;
#31004=CIRCLE ( 'NONE', #50143, 5.000000000000000888 ) ;
#31005=AXIS2_PLACEMENT_3D ( 'NONE', #62422, #16236, #17877 ) ;
#31006=LINE ( 'NONE', #51316, #56357 ) ;
#31008=DIRECTION ( 'NONE',  ( -1.000000000000000000, -0.000000000000000000, 0.000000000000000000 ) ) ;
#31009=AXIS2_PLACEMENT_3D ( 'NONE', #34999, #9750, #50351 ) ;
#31010=ORIENTED_EDGE ( 'NONE', *, *, #50842, .T. ) ;
#31011=EDGE_CURVE ( 'NONE', #64161, #13910, #8445, .T. ) ;
#31012=CIRCLE ( 'NONE', #10830, 12.18649999999999878 ) ;
#31013=DIRECTION ( 'NONE',  ( 0.000000000000000000, 0.01356324068817992001, -0.9999080150203990547 ) ) ;
#31016=ORIENTED_EDGE ( 'NONE', *, *, #31609, .T. ) ;
#31018=EDGE_CURVE ( 'NONE', #33456, #60735, #39122, .T. ) ;
#31020=AXIS2_PLACEMENT_3D ( 'NONE', #54734, #48441, #17834 ) ;
#31024=DIRECTION ( 'NONE',  ( -1.000000000000000000, 0.000000000000000000, 0.000000000000000000 ) ) ;
#31025=CARTESIAN_POINT ( 'NONE',  ( 10.48620311856346454, 8.250315036047107142, 10.68561190601526611 ) ) ;
#31027=DIRECTION ( 'NONE',  ( 1.000000000000000000, -0.000000000000000000, 0.000000000000000000 ) ) ;
#31029=AXIS2_PLACEMENT_3D ( 'NONE', #24336, #38072, #53391 ) ;
#31030=AXIS2_PLACEMENT_3D ( 'NONE', #54175, #24231, #58187 ) ;
#31033=ORIENTED_EDGE ( 'NONE', *, *, #57917, .T. ) ;
#31035=FACE_OUTER_BOUND ( 'NONE', #29889, .T. ) ;
#31037=ORIENTED_EDGE ( 'NONE', *, *, #41219, .F. ) ;
#31038=CARTESIAN_POINT ( 'NONE',  ( -17.29244623348158783, 2.525873743887551814, 11.73115347397430597 ) ) ;
#31039=DIRECTION ( 'NONE',  ( 0.000000000000000000, 0.6478160128811893959, -0.7617968321374922747 ) ) ;
#31043=CIRCLE ( 'NONE', #48053, 12.74999999999999822 ) ;
#31045=CARTESIAN_POINT ( 'NONE',  ( 145.1370849898475797, 3.309064568108273190E-14, 0.000000000000000000 ) ) ;
#31046=ADVANCED_FACE ( 'NONE', ( #31333 ), #52614, .T. ) ;
#31047=ORIENTED_EDGE ( 'NONE', *, *, #23895, .F. ) ;
#31048=FACE_OUTER_BOUND ( 'NONE', #12745, .T. ) ;
#31050=LINE ( 'NONE', #37008, #60910 ) ;
#31051=CARTESIAN_POINT ( 'NONE',  ( 35.00000000000000000, 8.389074212634284322, -8.839356091080075473 ) ) ;
#31052=VERTEX_POINT ( 'NONE', #36308 ) ;
#31053=AXIS2_PLACEMENT_3D ( 'NONE', #11432, #62296, #11748 ) ;
#31054=CARTESIAN_POINT ( 'NONE',  ( -35.00000000000000000, 0.000000000000000000, 0.000000000000000000 ) ) ;
#31057=CARTESIAN_POINT ( 'NONE',  ( 24.65531244048388615, -2.290097230841563913, -13.30568042842709531 ) ) ;
#31058=CARTESIAN_POINT ( 'NONE',  ( -35.00000000000000000, 12.17626345777664376, -0.4993900848166082374 ) ) ;
#31060=FACE_OUTER_BOUND ( 'NONE', #26660, .T. ) ;
#31061=ORIENTED_EDGE ( 'NONE', *, *, #34472, .T. ) ;
#31062=DIRECTION ( 'NONE',  ( 0.000000000000000000, -0.01356324068817998940, 0.9999080150203990547 ) ) ;
#31064=ADVANCED_FACE ( 'NONE', ( #27001 ), #57929, .T. ) ;
#31065=EDGE_LOOP ( 'NONE', ( #44046, #61057, #28889, #58149 ) ) ;
#31066=FACE_OUTER_BOUND ( 'NONE', #58511, .T. ) ;
#31070=FACE_OUTER_BOUND ( 'NONE', #2719, .T. ) ;
#31073=ORIENTED_EDGE ( 'NONE', *, *, #22076, .T. ) ;
#31074=AXIS2_PLACEMENT_3D ( 'NONE', #25515, #41451, #60437 ) ;
#31075=( BOUNDED_CURVE ( )  B_SPLINE_CURVE ( 3, ( #20854, #41445, #37119, #11851 ),
 .UNSPECIFIED., .F., .F. ) 
 B_SPLINE_CURVE_WITH_KNOTS ( ( 4, 4 ),
 ( 4.992524338435286424, 5.029647046869825999 ),
 .UNSPECIFIED. ) 
 CURVE ( )  GEOMETRIC_REPRESENTATION_ITEM ( )  RATIONAL_B_SPLINE_CURVE ( ( 1.000000000000000000, 0.9998851620069661994, 0.9998851620069661994, 1.000000000000000000 ) ) 
 REPRESENTATION_ITEM ( '' )  );
#31076=ORIENTED_EDGE ( 'NONE', *, *, #17325, .F. ) ;
#31078=VERTEX_POINT ( 'NONE', #51632 ) ;
#31080=VECTOR ( 'NONE', #1775, 1000.000000000000000 ) ;
#31081=ORIENTED_EDGE ( 'NONE', *, *, #1969, .F. ) ;
#31082=DIRECTION ( 'NONE',  ( 0.000000000000000000, 0.01356324068817998940, -0.9999080150203989437 ) ) ;
#31085=CARTESIAN_POINT ( 'NONE',  ( 35.00000000000000000, -12.14284015767850455, -1.030638227056526413 ) ) ;
#31087=DIRECTION ( 'NONE',  ( 1.000000000000000000, 0.000000000000000000, 0.000000000000000000 ) ) ;
#31088=AXIS2_PLACEMENT_3D ( 'NONE', #31197, #22185, #6588 ) ;
#31089=CYLINDRICAL_SURFACE ( 'NONE', #10793, 5.000000000000000888 ) ;
#31090=CIRCLE ( 'NONE', #62923, 12.75000000000000178 ) ;
#31091=DIRECTION ( 'NONE',  ( 0.000000000000000000, 0.5767582926624970074, 0.8169148498130275327 ) ) ;
#31092=EDGE_LOOP ( 'NONE', ( #29952, #37767, #63882, #10335 ) ) ;
#31093=DIRECTION ( 'NONE',  ( 0.000000000000000000, 0.8827602140260299990, -0.4698238015817395308 ) ) ;
#31094=CYLINDRICAL_SURFACE ( 'NONE', #54209, 4.999999999999999112 ) ;
#31097=AXIS2_PLACEMENT_3D ( 'NONE', #39214, #12971, #13303 ) ;
#31098=DIRECTION ( 'NONE',  ( 0.000000000000000000, 0.01356324068817992175, -0.9999080150203990547 ) ) ;
#31100=EDGE_CURVE ( 'NONE', #39541, #2304, #31638, .T. ) ;
#31101=CARTESIAN_POINT ( 'NONE',  ( 23.76403068109624073, 1.692630664537227769, -13.39737798747508890 ) ) ;
#31103=AXIS2_PLACEMENT_3D ( 'NONE', #36953, #41946, #21999 ) ;
#31104=ADVANCED_FACE ( 'NONE', ( #36644 ), #56947, .T. ) ;
#31105=DIRECTION ( 'NONE',  ( 1.000000000000000000, 0.000000000000000000, -0.000000000000000000 ) ) ;
#31106=ORIENTED_EDGE ( 'NONE', *, *, #35123, .F. ) ;
#31107=DIRECTION ( 'NONE',  ( 1.000000000000000000, 0.000000000000000000, -0.000000000000000000 ) ) ;
#31109=DIRECTION ( 'NONE',  ( 1.000000000000000000, 0.000000000000000000, 0.000000000000000000 ) ) ;
#31110=CARTESIAN_POINT ( 'NONE',  ( -25.95111430559885690, 10.26727955753690580, 6.212991851984511982 ) ) ;
#31111=DIRECTION ( 'NONE',  ( 0.000000000000000000, -0.9970832820307047317, -0.07632122047555403577 ) ) ;
#31112=ORIENTED_EDGE ( 'NONE', *, *, #54678, .F. ) ;
#31113=CARTESIAN_POINT ( 'NONE',  ( -17.14841977825820507, -7.768776852921657650, -11.04569896549689290 ) ) ;
#31114=DIRECTION ( 'NONE',  ( 1.000000000000000000, 0.000000000000000000, -0.000000000000000000 ) ) ;
#31117=CYLINDRICAL_SURFACE ( 'NONE', #34443, 12.18650000000000055 ) ;
#31119=DIRECTION ( 'NONE',  ( 1.000000000000000000, -0.000000000000000000, 0.000000000000000000 ) ) ;
#31121=AXIS2_PLACEMENT_3D ( 'NONE', #8901, #49486, #24186 ) ;
#31124=CARTESIAN_POINT ( 'NONE',  ( -35.00000000000000000, 0.000000000000000000, 0.000000000000000000 ) ) ;
#31125=VECTOR ( 'NONE', #54616, 1000.000000000000000 ) ;
#31127=AXIS2_PLACEMENT_3D ( 'NONE', #62770, #22210, #17238 ) ;
#31128=EDGE_CURVE ( 'NONE', #26214, #61654, #16684, .T. ) ;
#31129=FACE_OUTER_BOUND ( 'NONE', #39514, .T. ) ;
#31130=ORIENTED_EDGE ( 'NONE', *, *, #1728, .F. ) ;
#31132=ADVANCED_FACE ( 'NONE', ( #31964 ), #6727, .T. ) ;
#31133=DIRECTION ( 'NONE',  ( 1.000000000000000000, 0.000000000000000000, 0.000000000000000000 ) ) ;
#31135=CARTESIAN_POINT ( 'NONE',  ( 8.437200413559441614, 4.476360154859202467, -12.73625532737110966 ) ) ;
#31136=CARTESIAN_POINT ( 'NONE',  ( -9.351388602708162523, 11.42638970207765681, -3.665735721005252135 ) ) ;
#31138=CARTESIAN_POINT ( 'NONE',  ( -18.14978613422465870, 3.488173043128369066, 13.04371742822381819 ) ) ;
#31140=ORIENTED_EDGE ( 'NONE', *, *, #62016, .F. ) ;
#31141=ORIENTED_EDGE ( 'NONE', *, *, #1162, .T. ) ;
#31142=CARTESIAN_POINT ( 'NONE',  ( -35.00000000000000000, -11.70009620280410978, -1.039216533673027243 ) ) ;
#31143=AXIS2_PLACEMENT_3D ( 'NONE', #62110, #16562, #26856 ) ;
#31144=ORIENTED_EDGE ( 'NONE', *, *, #40135, .F. ) ;
#31147=CARTESIAN_POINT ( 'NONE',  ( 35.00000000000000000, 4.725891942574903304, 10.75351884295722193 ) ) ;
#31148=CIRCLE ( 'NONE', #20517, 4.999999999999998224 ) ;
#31150=CARTESIAN_POINT ( 'NONE',  ( -37.00000000000000711, -9.390600770287932164, -8.624332853796161658 ) ) ;
#31152=CYLINDRICAL_SURFACE ( 'NONE', #55281, 14.69297241773857188 ) ;
#31154=CARTESIAN_POINT ( 'NONE',  ( -24.32900315761321153, -7.891165000983839661, 9.051290049333715615 ) ) ;
#31155=CARTESIAN_POINT ( 'NONE',  ( 9.575800908719084958, 25.00000000000000000, -1.072919909436247154 ) ) ;
#31157=AXIS2_PLACEMENT_3D ( 'NONE', #51869, #37548, #32532 ) ;
#31158=ORIENTED_EDGE ( 'NONE', *, *, #51670, .F. ) ;
#31159=CARTESIAN_POINT ( 'NONE',  ( 28.81710800639762482, -11.52178284190103064, 7.047181458019091238 ) ) ;
#31160=EDGE_CURVE ( 'NONE', #41185, #16429, #34270, .T. ) ;
#31161=EDGE_CURVE ( 'NONE', #37463, #55813, #36982, .T. ) ;
#31162=EDGE_LOOP ( 'NONE', ( #24028, #38108, #53115, #55109 ) ) ;
#31163=DIRECTION ( 'NONE',  ( 0.000000000000000000, 0.4380125133593973930, -0.8989688749565157844 ) ) ;
#31165=DIRECTION ( 'NONE',  ( -1.000000000000000000, 0.000000000000000000, 0.000000000000000000 ) ) ;
#31166=EDGE_CURVE ( 'NONE', #1524, #60735, #23318, .T. ) ;
#31167=CARTESIAN_POINT ( 'NONE',  ( -29.46763719790810754, 0.7246786509642640928, 11.98539570541942112 ) ) ;
#31169=DIRECTION ( 'NONE',  ( 0.000000000000000000, -0.01356324068817998593, 0.9999080150203990547 ) ) ;
#31170=VECTOR ( 'NONE', #29450, 1000.000000000000000 ) ;
#31171=CARTESIAN_POINT ( 'NONE',  ( 47.00000000000000711, 4.705694406421931860E-17, -3.469127814946512892E-15 ) ) ;
#31172=ORIENTED_EDGE ( 'NONE', *, *, #65528, .T. ) ;
#31174=CARTESIAN_POINT ( 'NONE',  ( -4.806344283790351390, -7.508992741355383416, 25.00000000000000000 ) ) ;
#31175=DIRECTION ( 'NONE',  ( 0.000000000000000000, 0.5767582926624970074, 0.8169148498130275327 ) ) ;
#31176=AXIS2_PLACEMENT_3D ( 'NONE', #23876, #54461, #23537 ) ;
#31177=DIRECTION ( 'NONE',  ( -1.000000000000000000, 0.000000000000000000, -0.000000000000000000 ) ) ;
#31181=CARTESIAN_POINT ( 'NONE',  ( -35.00000000000000000, -3.340853584269456888, -11.26103545359859304 ) ) ;
#31182=ADVANCED_FACE ( 'NONE', ( #43580 ), #48294, .T. ) ;
#31183=VERTEX_POINT ( 'NONE', #3055 ) ;
#31184=AXIS2_PLACEMENT_3D ( 'NONE', #26295, #51259, #21648 ) ;
#31189=ORIENTED_EDGE ( 'NONE', *, *, #49275, .F. ) ;
#31190=FACE_OUTER_BOUND ( 'NONE', #21998, .T. ) ;
#31191=CARTESIAN_POINT ( 'NONE',  ( -14.40132519092765939, 7.823324605749410132, -11.00218777330444020 ) ) ;
#31192=CIRCLE ( 'NONE', #54560, 12.74999999999999822 ) ;
#31195=ORIENTED_EDGE ( 'NONE', *, *, #30829, .F. ) ;
#31196=PLANE ( 'NONE',  #11244 ) ;
#31197=CARTESIAN_POINT ( 'NONE',  ( 35.00000000000000000, 6.307491713049029336, -9.908974237959670361 ) ) ;
#31200=VECTOR ( 'NONE', #53720, 1000.000000000000000 ) ;
#31201=CARTESIAN_POINT ( 'NONE',  ( -17.15271379239874250, -7.063395208604966058, 9.707307756281583266 ) ) ;
#31203=ORIENTED_EDGE ( 'NONE', *, *, #38771, .F. ) ;
#31205=DIRECTION ( 'NONE',  ( -0.000000000000000000, -1.000000000000000000, -0.000000000000000000 ) ) ;
#31206=ORIENTED_EDGE ( 'NONE', *, *, #19856, .T. ) ;
#31207=CARTESIAN_POINT ( 'NONE',  ( 35.00000000000000000, 12.74613886779084559, -0.3137578094509725357 ) ) ;
#31208=CARTESIAN_POINT ( 'NONE',  ( 37.00000000000000711, 4.705694406421931860E-17, -3.469127814946512892E-15 ) ) ;
#31209=CARTESIAN_POINT ( 'NONE',  ( -7.181456785175555524, -5.890186129966251904, -10.45493698471458188 ) ) ;
#31210=DIRECTION ( 'NONE',  ( 1.000000000000000000, 0.000000000000000000, 0.000000000000000000 ) ) ;
#31211=AXIS2_PLACEMENT_3D ( 'NONE', #20914, #4990, #41516 ) ;
#31212=ORIENTED_EDGE ( 'NONE', *, *, #6692, .F. ) ;
#31218=CARTESIAN_POINT ( 'NONE',  ( 0.6920704694426910164, 0.4803808886326909056, -13.50000000000000178 ) ) ;
#31220=DIRECTION ( 'NONE',  ( 0.000000000000000000, -0.7381862504171878836, 0.6745969609292743474 ) ) ;
#31221=DIRECTION ( 'NONE',  ( 0.000000000000000000, 0.01356324068817998940, -0.9999080150203989437 ) ) ;
#31223=DIRECTION ( 'NONE',  ( 0.000000000000000000, 0.01356324068817998940, -0.9999080150203990547 ) ) ;
#31225=CIRCLE ( 'NONE', #1485, 5.000000000000001776 ) ;
#31226=CARTESIAN_POINT ( 'NONE',  ( 35.00000000000000000, 8.258652103341434625, -8.352657516904704593 ) ) ;
#31228=LINE ( 'NONE', #26238, #58900 ) ;
#31229=AXIS2_PLACEMENT_3D ( 'NONE', #54692, #45024, #19097 ) ;
#31230=CARTESIAN_POINT ( 'NONE',  ( 17.57949967008812209, 9.831142232691801652, 9.259614918201451772 ) ) ;
#31231=ADVANCED_FACE ( 'NONE', ( #28964 ), #33625, .T. ) ;
#31232=ORIENTED_EDGE ( 'NONE', *, *, #28219, .F. ) ;
#31235=DIRECTION ( 'NONE',  ( 1.000000000000000000, 0.000000000000000000, 0.000000000000000000 ) ) ;
#31236=VECTOR ( 'NONE', #56742, 1000.000000000000000 ) ;
#31240=VERTEX_POINT ( 'NONE', #38264 ) ;
#31242=CARTESIAN_POINT ( 'NONE',  ( -35.00000000000000000, -7.717887834988307105, 8.854740511458828678 ) ) ;
#31243=VERTEX_POINT ( 'NONE', #18349 ) ;
#31244=ADVANCED_FACE ( 'NONE', ( #3728 ), #18989, .T. ) ;
#31245=CARTESIAN_POINT ( 'NONE',  ( -37.00000000000000711, 0.000000000000000000, 0.000000000000000000 ) ) ;
#31246=ORIENTED_EDGE ( 'NONE', *, *, #34886, .F. ) ;
#31247=VECTOR ( 'NONE', #7795, 1000.000000000000000 ) ;
#31248=ORIENTED_EDGE ( 'NONE', *, *, #57082, .F. ) ;
#31249=ORIENTED_EDGE ( 'NONE', *, *, #45035, .F. ) ;
#31253=CARTESIAN_POINT ( 'NONE',  ( 35.00000000000000000, -6.307491713048959170, 9.908974237959705889 ) ) ;
#31254=DIRECTION ( 'NONE',  ( 0.000000000000000000, -0.01356324068817992001, 0.9999080150203990547 ) ) ;
#31259=CIRCLE ( 'NONE', #38707, 5.000000000000000888 ) ;
#31260=CARTESIAN_POINT ( 'NONE',  ( -3.026545681158347101, 9.064712759764015360, 10.02988752212787738 ) ) ;
#31261=FACE_OUTER_BOUND ( 'NONE', #49640, .T. ) ;
#31266=AXIS2_PLACEMENT_3D ( 'NONE', #46962, #62242, #31972 ) ;
#31267=VERTEX_POINT ( 'NONE', #64212 ) ;
#31268=CYLINDRICAL_SURFACE ( 'NONE', #7797, 4.999999999999999112 ) ;
#31274=DIRECTION ( 'NONE',  ( 0.000000000000000000, -0.01356324068817998593, 0.9999080150203990547 ) ) ;
#31276=ORIENTED_EDGE ( 'NONE', *, *, #24110, .T. ) ;
#31278=AXIS2_PLACEMENT_3D ( 'NONE', #30138, #60074, #45753 ) ;
#31279=FACE_OUTER_BOUND ( 'NONE', #34888, .T. ) ;
#31283=ADVANCED_FACE ( 'NONE', ( #18684 ), #38942, .T. ) ;
#31287=CARTESIAN_POINT ( 'NONE',  ( 16.78263030916553333, -10.48479066935623827, 5.836879698929882565 ) ) ;
#31288=FACE_OUTER_BOUND ( 'NONE', #6360, .T. ) ;
#31289=AXIS2_PLACEMENT_3D ( 'NONE', #65385, #48817, #3266 ) ;
#31294=LINE ( 'NONE', #56911, #27950 ) ;
#31295=CARTESIAN_POINT ( 'NONE',  ( -27.27855387000350262, 25.00000000000000000, 5.631341004100471892 ) ) ;
#31296=CARTESIAN_POINT ( 'NONE',  ( -35.00000000000000000, 0.000000000000000000, 0.000000000000000000 ) ) ;
#31297=EDGE_CURVE ( 'NONE', #59054, #42105, #40159, .T. ) ;
#31299=ORIENTED_EDGE ( 'NONE', *, *, #63400, .T. ) ;
#31304=ADVANCED_FACE ( 'NONE', ( #65185 ), #9309, .T. ) ;
#31305=ORIENTED_EDGE ( 'NONE', *, *, #61991, .T. ) ;
#31306=CARTESIAN_POINT ( 'NONE',  ( -18.08686583997218378, 4.948971728452300489, -10.93424994070406697 ) ) ;
#31308=VERTEX_POINT ( 'NONE', #34899 ) ;
#31312=EDGE_LOOP ( 'NONE', ( #38464, #4844, #33126, #48165 ) ) ;
#31315=ADVANCED_FACE ( 'NONE', ( #49902 ), #50241, .T. ) ;
#31316=STYLED_ITEM ( 'NONE', ( #48496 ), #65033 ) ;
#31317=DIRECTION ( 'NONE',  ( 0.000000000000000000, 0.9796553971857748788, 0.2006870767258854826 ) ) ;
#31318=EDGE_LOOP ( 'NONE', ( #47985, #65743, #58077, #1652 ) ) ;
#31320=DIRECTION ( 'NONE',  ( -1.000000000000000000, 0.000000000000000000, 0.000000000000000000 ) ) ;
#31322=CARTESIAN_POINT ( 'NONE',  ( 37.00000000000000711, -10.62137734850271364, -5.015831474386272859 ) ) ;
#31323=CARTESIAN_POINT ( 'NONE',  ( 37.00000000000000711, -10.54834585426224081, -6.102719229070642015 ) ) ;
#31324=DIRECTION ( 'NONE',  ( -1.000000000000000000, -0.000000000000000000, 0.000000000000000000 ) ) ;
#31325=LINE ( 'NONE', #10699, #45242 ) ;
#31326=CARTESIAN_POINT ( 'NONE',  ( 8.437200413559441614, 4.476360154859203355, -11.13383131558893346 ) ) ;
#31327=DIRECTION ( 'NONE',  ( 0.000000000000000000, 0.01356324068817998940, -0.9999080150203990547 ) ) ;
#31328=ORIENTED_EDGE ( 'NONE', *, *, #30925, .F. ) ;
#31329=EDGE_CURVE ( 'NONE', #38122, #44608, #59242, .T. ) ;
#31330=CARTESIAN_POINT ( 'NONE',  ( -37.00000000000000711, -10.99909370905153772, -5.246972444134135216 ) ) ;
#31333=FACE_OUTER_BOUND ( 'NONE', #65495, .T. ) ;
#31335=VERTEX_POINT ( 'NONE', #59887 ) ;
#31336=CYLINDRICAL_SURFACE ( 'NONE', #4185, 4.999999999999999112 ) ;
#31342=CARTESIAN_POINT ( 'NONE',  ( -18.73298729874495905, -4.205490829016433452, -11.23957459224111588 ) ) ;
#31346=CARTESIAN_POINT ( 'NONE',  ( -35.00000000000000000, 2.968224442958403486, 11.81949347079748058 ) ) ;
#31347=ORIENTED_EDGE ( 'NONE', *, *, #54324, .T. ) ;
#31349=EDGE_CURVE ( 'NONE', #46774, #20824, #19960, .T. ) ;
#31350=AXIS2_PLACEMENT_3D ( 'NONE', #54676, #59650, #59317 ) ;
#31353=DIRECTION ( 'NONE',  ( -1.000000000000000000, 0.000000000000000000, -0.000000000000000000 ) ) ;
#31354=CARTESIAN_POINT ( 'NONE',  ( 10.16520822268187807, 8.041842148762462728, 10.84657292646973659 ) ) ;
#31355=CARTESIAN_POINT ( 'NONE',  ( -9.197504613504056792, -11.40546504581821630, -3.730959538268487474 ) ) ;
#31359=EDGE_CURVE ( 'NONE', #40151, #42493, #1981, .T. ) ;
#31360=ORIENTED_EDGE ( 'NONE', *, *, #39260, .F. ) ;
#31361=CARTESIAN_POINT ( 'NONE',  ( -14.29135464769095520, 7.782112657557433977, 11.03126115115966499 ) ) ;
#31362=CARTESIAN_POINT ( 'NONE',  ( 35.00000000000000000, 4.705694406421931860E-17, -3.469127814946512892E-15 ) ) ;
#31363=ORIENTED_EDGE ( 'NONE', *, *, #11142, .F. ) ;
#31364=EDGE_CURVE ( 'NONE', #61571, #24621, #29935, .T. ) ;
#31366=DIRECTION ( 'NONE',  ( -0.000000000000000000, -0.000000000000000000, -1.000000000000000000 ) ) ;
#31367=CARTESIAN_POINT ( 'NONE',  ( -9.067636645460236622, 10.05071032021384703, -9.020536413389423913 ) ) ;
#31368=ORIENTED_EDGE ( 'NONE', *, *, #6962, .F. ) ;
#31369=CARTESIAN_POINT ( 'NONE',  ( 37.00000000000000711, -11.67026961469347768, -4.564151185897032725 ) ) ;
#31371=EDGE_CURVE ( 'NONE', #24519, #10393, #57192, .T. ) ;
#31372=VERTEX_POINT ( 'NONE', #14951 ) ;
#31374=VERTEX_POINT ( 'NONE', #4701 ) ;
#31375=ORIENTED_EDGE ( 'NONE', *, *, #2929, .T. ) ;
#31376=VECTOR ( 'NONE', #23967, 1000.000000000000000 ) ;
#31377=DIRECTION ( 'NONE',  ( 0.000000000000000000, -1.000000000000000000, 0.000000000000000000 ) ) ;
#31378=EDGE_CURVE ( 'NONE', #15712, #63812, #29579, .T. ) ;
#31379=EDGE_LOOP ( 'NONE', ( #63994, #20153, #16880, #53585 ) ) ;
#31380=CARTESIAN_POINT ( 'NONE',  ( -26.91209319802521449, -10.55322015549179682, 5.712709916062060245 ) ) ;
#31383=DIRECTION ( 'NONE',  ( 0.000000000000000000, -0.8009703041134234036, -0.5987040770935587730 ) ) ;
#31384=ORIENTED_EDGE ( 'NONE', *, *, #42803, .F. ) ;
#31385=CARTESIAN_POINT ( 'NONE',  ( -18.58686583997225839, 5.151216734910813777, 10.83812558286603789 ) ) ;
#31386=EDGE_CURVE ( 'NONE', #39606, #61650, #28492, .T. ) ;
#31388=CARTESIAN_POINT ( 'NONE',  ( 37.00000000000000711, -0.2661492558802491804, 12.18359334611896294 ) ) ;
#31389=DIRECTION ( 'NONE',  ( 1.000000000000000000, 0.000000000000000000, 0.000000000000000000 ) ) ;
#31390=VERTEX_POINT ( 'NONE', #45236 ) ;
#31394=ORIENTED_EDGE ( 'NONE', *, *, #8513, .T. ) ;
#31395=VERTEX_POINT ( 'NONE', #65493 ) ;
#31396=DIRECTION ( 'NONE',  ( 0.000000000000000000, -0.4380125133594037767, 0.8989688749565126757 ) ) ;
#31397=ADVANCED_FACE ( 'NONE', ( #60519 ), #25271, .T. ) ;
#31398=DIRECTION ( 'NONE',  ( -1.000000000000000000, 0.000000000000000000, 0.000000000000000000 ) ) ;
#31399=LINE ( 'NONE', #16096, #9906 ) ;
#31401=EDGE_LOOP ( 'NONE', ( #16977, #19488, #5374, #9603 ) ) ;
#31402=FACE_OUTER_BOUND ( 'NONE', #18935, .T. ) ;
#31405=EDGE_CURVE ( 'NONE', #16904, #52157, #55873, .T. ) ;
#31407=ORIENTED_EDGE ( 'NONE', *, *, #38182, .F. ) ;
#31408=CARTESIAN_POINT ( 'NONE',  ( 37.00000000000000711, 4.705694406421931860E-17, -3.469127814946512892E-15 ) ) ;
#31409=VERTEX_POINT ( 'NONE', #15302 ) ;
#31412=DIRECTION ( 'NONE',  ( -0.8514458006899927600, 0.000000000000000000, -0.5244426074294281648 ) ) ;
#31413=CARTESIAN_POINT ( 'NONE',  ( -25.54417658651491863, -7.498517398407823720, 11.22596262356930197 ) ) ;
#31416=DIRECTION ( 'NONE',  ( -1.000000000000000000, 0.000000000000000000, 0.000000000000000000 ) ) ;
#31418=PLANE ( 'NONE',  #17436 ) ;
#31419=CIRCLE ( 'NONE', #2774, 5.000000000000001776 ) ;
#31420=ORIENTED_EDGE ( 'NONE', *, *, #49969, .T. ) ;
#31422=CARTESIAN_POINT ( 'NONE',  ( 35.00000000000000000, 11.98254675519227952, -2.220215194441947482 ) ) ;
#31424=EDGE_CURVE ( 'NONE', #9122, #16609, #25316, .T. ) ;
#31426=ADVANCED_FACE ( 'NONE', ( #1979 ), #32222, .T. ) ;
#31428=DIRECTION ( 'NONE',  ( 1.000000000000000000, 0.000000000000000000, 0.000000000000000000 ) ) ;
#31430=CARTESIAN_POINT ( 'NONE',  ( 10.39074034058834428, 0.7556363488327733080, -11.97742577131518971 ) ) ;
#31431=EDGE_LOOP ( 'NONE', ( #52006, #21328, #31689, #42854 ) ) ;
#31432=CARTESIAN_POINT ( 'NONE',  ( -35.00000000000000000, -9.060822531526103063, 7.474872387600973944 ) ) ;
#31434=DIRECTION ( 'NONE',  ( -1.000000000000000000, 0.000000000000000000, -0.000000000000000000 ) ) ;
#31435=EDGE_CURVE ( 'NONE', #64587, #40917, #22248, .T. ) ;
#31438=CARTESIAN_POINT ( 'NONE',  ( 12.52750123246316249, 0.4973700281276248192, -13.49083477977253764 ) ) ;
#31439=CARTESIAN_POINT ( 'NONE',  ( -47.00000000000000711, 0.000000000000000000, 0.000000000000000000 ) ) ;
#31441=CYLINDRICAL_SURFACE ( 'NONE', #58847, 5.000000000000000888 ) ;
#31442=FACE_OUTER_BOUND ( 'NONE', #25174, .T. ) ;
#31448=ADVANCED_FACE ( 'NONE', ( #26266 ), #36891, .T. ) ;
#31450=ORIENTED_EDGE ( 'NONE', *, *, #52496, .T. ) ;
#31451=DIRECTION ( 'NONE',  ( 1.000000000000000000, 0.000000000000000000, 0.000000000000000000 ) ) ;
#31452=VECTOR ( 'NONE', #50635, 1000.000000000000000 ) ;
#31456=CARTESIAN_POINT ( 'NONE',  ( 35.00000000000000000, -7.817492529713787164, 9.348667969174485393 ) ) ;
#31458=DIRECTION ( 'NONE',  ( -0.6151304903148129277, 0.000000000000000000, -0.7884253166185480888 ) ) ;
#31460=CARTESIAN_POINT ( 'NONE',  ( -27.01437459610461644, -10.69338818478079922, -8.240233560378637634 ) ) ;
#31461=EDGE_CURVE ( 'NONE', #51508, #6431, #30910, .T. ) ;
#31462=CARTESIAN_POINT ( 'NONE',  ( 35.00000000000000000, 12.57916205664484188, 2.080187960898425281 ) ) ;
#31464=ORIENTED_EDGE ( 'NONE', *, *, #53555, .F. ) ;
#31465=EDGE_CURVE ( 'NONE', #28103, #55517, #11548, .T. ) ;
#31466=ORIENTED_EDGE ( 'NONE', *, *, #23326, .F. ) ;
#31467=ORIENTED_EDGE ( 'NONE', *, *, #27432, .F. ) ;
#31470=EDGE_CURVE ( 'NONE', #38028, #22451, #24317, .T. ) ;
#31472=EDGE_CURVE ( 'NONE', #3051, #53717, #24172, .T. ) ;
#31474=EDGE_LOOP ( 'NONE', ( #32567, #28366, #6608, #8049 ) ) ;
#31476=CARTESIAN_POINT ( 'NONE',  ( -36.00000000000000711, 7.608228585767727203, 10.23119532541075394 ) ) ;
#31478=EDGE_LOOP ( 'NONE', ( #51707, #27311, #40127, #59600 ) ) ;
#31480=EDGE_CURVE ( 'NONE', #37413, #20683, #5678, .T. ) ;
#31481=CARTESIAN_POINT ( 'NONE',  ( 28.12675480332037736, -12.24425775564703045, 5.696251083233389245 ) ) ;
#31482=VERTEX_POINT ( 'NONE', #16290 ) ;
#31483=CARTESIAN_POINT ( 'NONE',  ( 21.95708534023389191, -11.48706736601068990, -3.476045417500702062 ) ) ;
#31485=DIRECTION ( 'NONE',  ( 0.000000000000000000, -0.9987865678893281807, 0.04924826701373505311 ) ) ;
#31486=DIRECTION ( 'NONE',  ( 0.000000000000000000, -0.9970832820307031774, -0.07632122047557582389 ) ) ;
#31487=CYLINDRICAL_SURFACE ( 'NONE', #5454, 12.18650000000000055 ) ;
#31488=LINE ( 'NONE', #51787, #21118 ) ;
#31490=ORIENTED_EDGE ( 'NONE', *, *, #51300, .T. ) ;
#31491=DIRECTION ( 'NONE',  ( 0.000000000000000000, -0.01356324068817991481, 0.9999080150203990547 ) ) ;
#31493=DIRECTION ( 'NONE',  ( -1.000000000000000000, 0.000000000000000000, 0.000000000000000000 ) ) ;
#31494=CARTESIAN_POINT ( 'NONE',  ( 36.00000000000000711, -12.74613886779084382, 0.3137578094510532489 ) ) ;
#31496=CARTESIAN_POINT ( 'NONE',  ( -37.00000000000000711, -11.30684963584386260, -4.545979934229533725 ) ) ;
#31498=EDGE_CURVE ( 'NONE', #49238, #47989, #43887, .T. ) ;
#31499=ORIENTED_EDGE ( 'NONE', *, *, #32616, .F. ) ;
#31500=CARTESIAN_POINT ( 'NONE',  ( 36.00000000000000711, -7.608228585767796481, -10.23119532541070420 ) ) ;
#31501=VECTOR ( 'NONE', #14109, 1000.000000000000000 ) ;
#31507=DIRECTION ( 'NONE',  ( 0.000000000000000000, 0.2006870767258890631, -0.9796553971857742127 ) ) ;
#31510=EDGE_CURVE ( 'NONE', #9279, #46246, #11940, .T. ) ;
#31515=VERTEX_POINT ( 'NONE', #47534 ) ;
#31516=DIRECTION ( 'NONE',  ( 0.000000000000000000, 0.8169148498130255343, -0.5767582926624998940 ) ) ;
#31517=VERTEX_POINT ( 'NONE', #42509 ) ;
#31521=ADVANCED_FACE ( 'NONE', ( #16621 ), #52204, .T. ) ;
#31522=CARTESIAN_POINT ( 'NONE',  ( -35.00000000000000000, 11.35427606708812753, -4.426194442447117794 ) ) ;
#31524=LINE ( 'NONE', #51176, #63875 ) ;
#31525=ORIENTED_EDGE ( 'NONE', *, *, #48536, .F. ) ;
#31527=CARTESIAN_POINT ( 'NONE',  ( -29.58743033447366244, 2.139843039584942375, 11.81524931570010395 ) ) ;
#31528=VERTEX_POINT ( 'NONE', #56875 ) ;
#31529=CARTESIAN_POINT ( 'NONE',  ( 3.381510803510703322, 5.478318359161011841, 10.67863534124962221 ) ) ;
#31530=CARTESIAN_POINT ( 'NONE',  ( -36.00000000000000711, 11.80185301892987582, -4.824807283153996096 ) ) ;
#31532=CARTESIAN_POINT ( 'NONE',  ( 35.00000000000000000, 10.80631716521673447, 4.603882218679430594 ) ) ;
#31534=CARTESIAN_POINT ( 'NONE',  ( 10.66583743953262342, 7.973724152180637681, -8.969682718315050707 ) ) ;
#31535=CARTESIAN_POINT ( 'NONE',  ( 37.00000000000000711, 10.93004082984027825, 6.564808257521646873 ) ) ;
#31537=CARTESIAN_POINT ( 'NONE',  ( -9.326486438888442976, -10.62366522422245296, -5.593402933327412008 ) ) ;
#31538=ORIENTED_EDGE ( 'NONE', *, *, #63955, .F. ) ;
#31539=AXIS2_PLACEMENT_3D ( 'NONE', #17992, #52606, #32288 ) ;
#31540=EDGE_CURVE ( 'NONE', #64820, #17169, #11643, .T. ) ;
#31541=FACE_OUTER_BOUND ( 'NONE', #22173, .T. ) ;
#31542=CARTESIAN_POINT ( 'NONE',  ( -35.00000000000000000, -11.73463472867573643, -3.287724142101541958 ) ) ;
#31543=VERTEX_POINT ( 'NONE', #11301 ) ;
#31544=AXIS2_PLACEMENT_3D ( 'NONE', #47578, #48907, #43903 ) ;
#31546=CARTESIAN_POINT ( 'NONE',  ( -35.00000000000000000, -12.16632754454237464, 0.7008968033238341944 ) ) ;
#31547=ORIENTED_EDGE ( 'NONE', *, *, #32575, .T. ) ;
#31548=CARTESIAN_POINT ( 'NONE',  ( 36.00000000000000711, -11.96656215839371917, -4.400442035670902641 ) ) ;
#31551=ORIENTED_EDGE ( 'NONE', *, *, #25371, .T. ) ;
#31554=CARTESIAN_POINT ( 'NONE',  ( -9.351388602708162523, 11.42638970207765681, -3.665735721005252135 ) ) ;
#31555=ORIENTED_EDGE ( 'NONE', *, *, #11134, .F. ) ;
#31560=DIRECTION ( 'NONE',  ( 1.000000000000000000, 0.000000000000000000, -0.000000000000000000 ) ) ;
#31564=CARTESIAN_POINT ( 'NONE',  ( 35.00000000000000000, 1.113475361586666157, 12.70128625845191017 ) ) ;
#31567=ORIENTED_EDGE ( 'NONE', *, *, #2249, .T. ) ;
#31568=DIRECTION ( 'NONE',  ( 0.000000000000000000, 0.9847383929261610547, -0.1740410799127650732 ) ) ;
#31570=DIRECTION ( 'NONE',  ( 1.000000000000000000, 0.000000000000000000, -0.000000000000000000 ) ) ;
#31571=CARTESIAN_POINT ( 'NONE',  ( -37.00000000000000711, -0.06441628369844948354, 12.18632975068353019 ) ) ;
#31572=CARTESIAN_POINT ( 'NONE',  ( -35.00000000000000000, 1.262958560998759472, 12.12087942037210198 ) ) ;
#31574=( GEOMETRIC_REPRESENTATION_CONTEXT ( 3 ) GLOBAL_UNCERTAINTY_ASSIGNED_CONTEXT ( ( #12377 ) ) GLOBAL_UNIT_ASSIGNED_CONTEXT ( ( #22659, #37934, #28294 ) ) REPRESENTATION_CONTEXT ( 'NONE', 'WORKASPACE' ) );
#31577=EDGE_CURVE ( 'NONE', #1650, #10081, #65684, .T. ) ;
#31582=DIRECTION ( 'NONE',  ( 0.000000000000000000, -0.01356324068817991828, 0.9999080150203990547 ) ) ;
#31583=CARTESIAN_POINT ( 'NONE',  ( 12.93723047338301058, 4.476360154859203355, 25.00000000000000000 ) ) ;
#31587=CARTESIAN_POINT ( 'NONE',  ( 21.62857653820161019, 11.91062359620538658, -1.517306329825557576 ) ) ;
#31588=AXIS2_PLACEMENT_3D ( 'NONE', #57098, #32128, #11522 ) ;
#31595=CARTESIAN_POINT ( 'NONE',  ( -19.10799584608659885, -11.93643250936202271, -1.402863707794529846 ) ) ;
#31599=EDGE_LOOP ( 'NONE', ( #38157, #40129, #20485, #11121 ) ) ;
#31600=ORIENTED_EDGE ( 'NONE', *, *, #42795, .F. ) ;
#31601=CYLINDRICAL_SURFACE ( 'NONE', #9820, 5.000000000000000888 ) ;
#31603=DIRECTION ( 'NONE',  ( 0.000000000000000000, 0.9999080150203989437, 0.01356324068818348313 ) ) ;
#31604=CYLINDRICAL_SURFACE ( 'NONE', #15887, 12.18650000000000055 ) ;
#31605=ORIENTED_EDGE ( 'NONE', *, *, #64683, .T. ) ;
#31606=ORIENTED_EDGE ( 'NONE', *, *, #38374, .T. ) ;
#31607=ORIENTED_EDGE ( 'NONE', *, *, #2793, .T. ) ;
#31608=CARTESIAN_POINT ( 'NONE',  ( 27.16179963944285447, -11.36021166003125593, 3.882017433740367895 ) ) ;
#31609=EDGE_CURVE ( 'NONE', #12385, #48435, #58164, .T. ) ;
#31610=CIRCLE ( 'NONE', #2984, 12.74999999999999822 ) ;
#31612=ORIENTED_EDGE ( 'NONE', *, *, #24767, .F. ) ;
#31613=CARTESIAN_POINT ( 'NONE',  ( 35.00000000000000000, 11.70009620280413110, 1.039216533672774112 ) ) ;
#31614=FACE_OUTER_BOUND ( 'NONE', #43222, .T. ) ;
#31615=AXIS2_PLACEMENT_3D ( 'NONE', #57105, #62389, #26833 ) ;
#31616=ORIENTED_EDGE ( 'NONE', *, *, #45035, .T. ) ;
#31619=CARTESIAN_POINT ( 'NONE',  ( 24.65204228265436726, -2.300319471321356612, 11.77898663366571341 ) ) ;
#31620=ORIENTED_EDGE ( 'NONE', *, *, #49771, .T. ) ;
#31621=AXIS2_PLACEMENT_3D ( 'NONE', #15763, #5840, #50399 ) ;
#31625=AXIS2_PLACEMENT_3D ( 'NONE', #39677, #9393, #49985 ) ;
#31628=CARTESIAN_POINT ( 'NONE',  ( -35.00000000000000000, -10.23119532541078058, 7.608228585767690788 ) ) ;
#31630=DIRECTION ( 'NONE',  ( -1.000000000000000000, -0.000000000000000000, 0.000000000000000000 ) ) ;
#31632=VECTOR ( 'NONE', #49646, 1000.000000000000000 ) ;
#31633=DIRECTION ( 'NONE',  ( 0.000000000000000000, 0.01356324068817998940, -0.9999080150203990547 ) ) ;
#31634=CYLINDRICAL_SURFACE ( 'NONE', #63176, 4.999999999999999112 ) ;
#31635=ORIENTED_EDGE ( 'NONE', *, *, #4956, .F. ) ;
#31637=ORIENTED_EDGE ( 'NONE', *, *, #12712, .T. ) ;
#31638=LINE ( 'NONE', #16370, #38076 ) ;
#31640=ORIENTED_EDGE ( 'NONE', *, *, #64780, .F. ) ;
#31641=CARTESIAN_POINT ( 'NONE',  ( -18.35103012267012446, 6.403183891280330720, 10.15237553557610717 ) ) ;
#31642=DIRECTION ( 'NONE',  ( 0.000000000000000000, 0.000000000000000000, -1.000000000000000000 ) ) ;
#31643=DIRECTION ( 'NONE',  ( 0.000000000000000000, 0.9346839223284553189, -0.3554799084908935036 ) ) ;
#31644=CARTESIAN_POINT ( 'NONE',  ( -35.00000000000000000, 0.000000000000000000, 0.000000000000000000 ) ) ;
#31645=EDGE_LOOP ( 'NONE', ( #23330, #4297, #51008, #63302 ) ) ;
#31647=EDGE_CURVE ( 'NONE', #59346, #7701, #23573, .T. ) ;
#31648=VERTEX_POINT ( 'NONE', #48212 ) ;
#31650=DIRECTION ( 'NONE',  ( 0.000000000000000000, 0.9551603052523489623, -0.2960891610144475994 ) ) ;
#31652=FACE_OUTER_BOUND ( 'NONE', #19889, .T. ) ;
#31656=VECTOR ( 'NONE', #20536, 1000.000000000000000 ) ;
#31657=EDGE_CURVE ( 'NONE', #55363, #3924, #22592, .T. ) ;
#31658=CIRCLE ( 'NONE', #45475, 5.000000000000001776 ) ;
#31661=DIRECTION ( 'NONE',  ( 1.000000000000000000, -0.000000000000000000, 0.000000000000000000 ) ) ;
#31662=DIRECTION ( 'NONE',  ( 0.000000000000000000, -0.7196168960969868689, -0.6943713148249562872 ) ) ;
#31665=CYLINDRICAL_SURFACE ( 'NONE', #16097, 12.75000000000000178 ) ;
#31666=EDGE_CURVE ( 'NONE', #27200, #14515, #27345, .T. ) ;
#31670=VERTEX_POINT ( 'NONE', #33211 ) ;
#31671=DIRECTION ( 'NONE',  ( -0.000000000000000000, -0.000000000000000000, -1.000000000000000000 ) ) ;
#31673=VERTEX_POINT ( 'NONE', #38184 ) ;
#31676=VERTEX_POINT ( 'NONE', #53836 ) ;
#31677=CARTESIAN_POINT ( 'NONE',  ( 22.57855258442565116, 3.026812727784649493, 25.00000000000000000 ) ) ;
#31680=ORIENTED_EDGE ( 'NONE', *, *, #44432, .F. ) ;
#31682=DIRECTION ( 'NONE',  ( -1.000000000000000000, 0.000000000000000000, 0.000000000000000000 ) ) ;
#31684=VERTEX_POINT ( 'NONE', #7277 ) ;
#31685=CARTESIAN_POINT ( 'NONE',  ( -25.69578604477335659, -5.442779444386042442, 10.69993300052666640 ) ) ;
#31687=DIRECTION ( 'NONE',  ( 0.000000000000000000, 0.01356324068817998940, -0.9999080150203990547 ) ) ;
#31688=FACE_OUTER_BOUND ( 'NONE', #31312, .T. ) ;
#31689=ORIENTED_EDGE ( 'NONE', *, *, #44167, .T. ) ;
#31690=CARTESIAN_POINT ( 'NONE',  ( -37.00000000000000711, 3.473736367725253960, 12.26766708251992988 ) ) ;
#31691=AXIS2_PLACEMENT_3D ( 'NONE', #32450, #63052, #28144 ) ;
#31694=DIRECTION ( 'NONE',  ( -1.000000000000000000, -0.000000000000000000, 0.000000000000000000 ) ) ;
#31695=ORIENTED_EDGE ( 'NONE', *, *, #35602, .F. ) ;
#31696=CARTESIAN_POINT ( 'NONE',  ( -27.45775109278351067, 8.499184579339635448, -8.471355351200609007 ) ) ;
#31697=ORIENTED_EDGE ( 'NONE', *, *, #24387, .T. ) ;
#31698=DIRECTION ( 'NONE',  ( 1.000000000000000000, -0.000000000000000000, 0.000000000000000000 ) ) ;
#31699=ORIENTED_EDGE ( 'NONE', *, *, #12968, .F. ) ;
#31700=CYLINDRICAL_SURFACE ( 'NONE', #8202, 5.000000000000000888 ) ;
#31701=DIRECTION ( 'NONE',  ( -1.000000000000000000, 0.000000000000000000, 0.000000000000000000 ) ) ;
#31704=EDGE_CURVE ( 'NONE', #14785, #3974, #2974, .T. ) ;
#31710=AXIS2_PLACEMENT_3D ( 'NONE', #2423, #43607, #57628 ) ;
#31712=ORIENTED_EDGE ( 'NONE', *, *, #28003, .F. ) ;
#31713=DIRECTION ( 'NONE',  ( 1.000000000000000000, 0.000000000000000000, -0.000000000000000000 ) ) ;
#31714=ORIENTED_EDGE ( 'NONE', *, *, #22036, .T. ) ;
#31717=DIRECTION ( 'NONE',  ( 0.000000000000000000, -0.01356324068817998940, 0.9999080150203990547 ) ) ;
#31718=CARTESIAN_POINT ( 'NONE',  ( -35.00000000000000000, -2.021542716731318912, -12.01765980939844169 ) ) ;
#31722=CARTESIAN_POINT ( 'NONE',  ( 35.00000000000000000, 4.946702696913328090, 11.13736569743268845 ) ) ;
#31724=CARTESIAN_POINT ( 'NONE',  ( 35.00000000000000000, 5.921969905510355403, -10.14408668126215929 ) ) ;
#31725=EDGE_CURVE ( 'NONE', #38332, #5898, #23911, .T. ) ;
#31727=EDGE_CURVE ( 'NONE', #41185, #6776, #16867, .T. ) ;
#31730=CIRCLE ( 'NONE', #30686, 12.75000000000000178 ) ;
#31731=DIRECTION ( 'NONE',  ( -1.000000000000000000, -0.000000000000000000, 0.000000000000000000 ) ) ;
#31736=CARTESIAN_POINT ( 'NONE',  ( 1.499544914656756101, 0.6073691993713128401, -11.98564492472154086 ) ) ;
#31737=DIRECTION ( 'NONE',  ( 1.000000000000000000, -0.000000000000000000, 0.000000000000000000 ) ) ;
#31740=DIRECTION ( 'NONE',  ( -1.000000000000000000, 0.000000000000000000, 0.000000000000000000 ) ) ;
#31741=CARTESIAN_POINT ( 'NONE',  ( -37.00000000000000711, 0.000000000000000000, 0.000000000000000000 ) ) ;
#31743=CIRCLE ( 'NONE', #38112, 5.000000000000001776 ) ;
#31744=AXIS2_PLACEMENT_3D ( 'NONE', #46738, #4886, #5884 ) ;
#31746=CARTESIAN_POINT ( 'NONE',  ( 8.937200413559443390, 4.476360154859203355, -12.73625532737111143 ) ) ;
#31751=DIRECTION ( 'NONE',  ( -0.000000000000000000, -1.000000000000000000, -0.000000000000000000 ) ) ;
#31753=EDGE_CURVE ( 'NONE', #46246, #63372, #35823, .T. ) ;
#31755=FACE_OUTER_BOUND ( 'NONE', #53095, .T. ) ;
#31756=CARTESIAN_POINT ( 'NONE',  ( -18.08686583997218733, 5.151216734910788908, -10.83812558286602012 ) ) ;
#31757=DIRECTION ( 'NONE',  ( 0.000000000000000000, -0.01356324068817998940, 0.9999080150203990547 ) ) ;
#31758=DIRECTION ( 'NONE',  ( -1.000000000000000000, 0.000000000000000000, 0.000000000000000000 ) ) ;
#31761=CARTESIAN_POINT ( 'NONE',  ( -9.351388602708162523, 12.99278190472488248, -3.665735721005250358 ) ) ;
#31762=ORIENTED_EDGE ( 'NONE', *, *, #29300, .T. ) ;
#31763=CARTESIAN_POINT ( 'NONE',  ( 35.00000000000000000, -1.488153103996881610, 11.65150730582935701 ) ) ;
#31764=DIRECTION ( 'NONE',  ( 1.000000000000000000, 0.000000000000000000, -0.000000000000000000 ) ) ;
#31765=CARTESIAN_POINT ( 'NONE',  ( 22.57855258442565116, 3.026812727784649493, -11.61199400236326973 ) ) ;
#31766=CYLINDRICAL_SURFACE ( 'NONE', #41450, 5.000000000000000000 ) ;
#31770=ORIENTED_EDGE ( 'NONE', *, *, #16469, .F. ) ;
#31773=ORIENTED_EDGE ( 'NONE', *, *, #33094, .F. ) ;
#31774=B_SPLINE_CURVE_WITH_KNOTS ( 'NONE', 3,
 ( #2393, #22669, #49499, #65083, #19558, #42935, #33290, #12656, #22309, #17998, #44464, #42580, #53594, #39488, #29504, #39821, #63214, #52610, #17347, #62882 ),
 .UNSPECIFIED., .F., .F.,
 ( 4, 2, 2, 2, 2, 2, 2, 2, 2, 4 ),
 ( 9.341771812940338307E-18, 0.001217729388623014488, 0.001826594082934518155, 0.002435458777246022038, 0.003653188165869029370, 0.004870917554492038871, 0.006088646943115048372, 0.007306376331738057874, 0.008524105720361066507, 0.009741835108984076008 ),
 .UNSPECIFIED. ) ;
#31775=DIRECTION ( 'NONE',  ( 0.000000000000000000, -0.01356324068817991828, 0.9999080150203990547 ) ) ;
#31776=LINE ( 'NONE', #41771, #17319 ) ;
#31778=VECTOR ( 'NONE', #52783, 1000.000000000000000 ) ;
#31779=CARTESIAN_POINT ( 'NONE',  ( -36.00000000000000711, -7.882940143791846488, 10.02106554660705839 ) ) ;
#31780=VERTEX_POINT ( 'NONE', #34513 ) ;
#31781=LINE ( 'NONE', #52090, #30811 ) ;
#31783=VECTOR ( 'NONE', #87, 1000.000000000000000 ) ;
#31784=CARTESIAN_POINT ( 'NONE',  ( 37.00000000000000711, 4.705694406421931860E-17, -3.469127814946512892E-15 ) ) ;
#31785=VERTEX_POINT ( 'NONE', #54813 ) ;
#31789=ORIENTED_EDGE ( 'NONE', *, *, #12297, .F. ) ;
#31792=CARTESIAN_POINT ( 'NONE',  ( 37.00000000000000711, -12.68495603654572612, -1.286231064351273989 ) ) ;
#31794=AXIS2_PLACEMENT_3D ( 'NONE', #35543, #29256, #14908 ) ;
#31795=CYLINDRICAL_SURFACE ( 'NONE', #41547, 4.999999999999999112 ) ;
#31796=DIRECTION ( 'NONE',  ( 0.000000000000000000, -0.7196168960969719919, -0.6943713148249714973 ) ) ;
#31797=EDGE_CURVE ( 'NONE', #12400, #26236, #62514, .T. ) ;
#31798=DIRECTION ( 'NONE',  ( 1.000000000000000000, -0.000000000000000000, -0.000000000000000000 ) ) ;
#31799=CIRCLE ( 'NONE', #26496, 12.75000000000000178 ) ;
#31802=EDGE_LOOP ( 'NONE', ( #60615, #10994, #20588, #24493 ) ) ;
#31803=DIRECTION ( 'NONE',  ( -1.000000000000000000, -1.836970198721029688E-16, 0.000000000000000000 ) ) ;
#31805=CARTESIAN_POINT ( 'NONE',  ( -9.221157027727812761, 9.600812269888216122, -7.209108748489196472 ) ) ;
#31807=CARTESIAN_POINT ( 'NONE',  ( -17.87894447371643025, 11.34875452035183052, 3.899500356681838475 ) ) ;
#31809=VERTEX_POINT ( 'NONE', #41794 ) ;
#31810=ORIENTED_EDGE ( 'NONE', *, *, #63768, .T. ) ;
#31816=CARTESIAN_POINT ( 'NONE',  ( -14.29135464769095520, 7.782112657557433089, -11.03126115115966854 ) ) ;
#31818=CARTESIAN_POINT ( 'NONE',  ( -35.00000000000000000, 10.32377448871677039, -6.475373545682193033 ) ) ;
#31820=EDGE_LOOP ( 'NONE', ( #63473, #55489, #42125, #41481 ) ) ;
#31826=AXIS2_PLACEMENT_3D ( 'NONE', #54159, #31177, #46462 ) ;
#31827=EDGE_CURVE ( 'NONE', #6027, #28214, #10538, .T. ) ;
#31828=EDGE_CURVE ( 'NONE', #44540, #60515, #19014, .T. ) ;
#31829=DIRECTION ( 'NONE',  ( -1.000000000000000000, 0.000000000000000000, 0.000000000000000000 ) ) ;
#31830=CARTESIAN_POINT ( 'NONE',  ( 37.00000000000000711, 4.705694406421931860E-17, -3.469127814946512892E-15 ) ) ;
#31834=EDGE_CURVE ( 'NONE', #59342, #30274, #64645, .T. ) ;
#31836=DIRECTION ( 'NONE',  ( 0.000000000000000000, 0.8369827122275325104, 0.5472293298355300761 ) ) ;
#31837=CYLINDRICAL_SURFACE ( 'NONE', #17195, 12.18650000000000055 ) ;
#31838=DIRECTION ( 'NONE',  ( 1.000000000000000000, -0.000000000000000000, 0.000000000000000000 ) ) ;
#31841=CARTESIAN_POINT ( 'NONE',  ( -10.25468736929027536, -4.747758800244201716, 11.02689688273352075 ) ) ;
#31842=ORIENTED_EDGE ( 'NONE', *, *, #54721, .T. ) ;
#31843=ORIENTED_EDGE ( 'NONE', *, *, #42208, .F. ) ;
#31844=DIRECTION ( 'NONE',  ( 0.000000000000000000, 0.1740410799127612429, 0.9847383929261617208 ) ) ;
#31845=EDGE_LOOP ( 'NONE', ( #25319, #33820, #59886, #41866 ) ) ;
#31846=CARTESIAN_POINT ( 'NONE',  ( 3.467905914750478491, 6.588911164890562944, 10.03839023354865034 ) ) ;
#31847=CARTESIAN_POINT ( 'NONE',  ( 37.00000000000000711, -9.040300684349746874, -7.499679039484027143 ) ) ;
#31848=FACE_OUTER_BOUND ( 'NONE', #14269, .T. ) ;
#31849=CYLINDRICAL_SURFACE ( 'NONE', #20543, 1.750000000000000000 ) ;
#31852=CARTESIAN_POINT ( 'NONE',  ( -11.40165637462999904, -7.508992741355383416, 9.360289953322597611 ) ) ;
#31853=VERTEX_POINT ( 'NONE', #61100 ) ;
#31855=CIRCLE ( 'NONE', #25459, 11.99999999999998579 ) ;
#31858=CARTESIAN_POINT ( 'NONE',  ( 35.00000000000000000, -12.18359334611896294, -0.2661492558802951991 ) ) ;
#31861=FACE_OUTER_BOUND ( 'NONE', #30314, .T. ) ;
#31862=VERTEX_POINT ( 'NONE', #35800 ) ;
#31863=CARTESIAN_POINT ( 'NONE',  ( 36.00000000000000711, -5.300372733891561161, 11.59605747147791810 ) ) ;
#31864=DIRECTION ( 'NONE',  ( 1.000000000000000000, -0.000000000000000000, 0.000000000000000000 ) ) ;
#31865=CARTESIAN_POINT ( 'NONE',  ( -35.00000000000000000, 6.917234959366964198, -9.493370459201624811 ) ) ;
#31867=VERTEX_POINT ( 'NONE', #62088 ) ;
#31868=CARTESIAN_POINT ( 'NONE',  ( -35.00000000000000000, -12.18359334611896472, -0.2661492558804631203 ) ) ;
#31869=ORIENTED_EDGE ( 'NONE', *, *, #32785, .F. ) ;
#31870=VERTEX_POINT ( 'NONE', #41126 ) ;
#31871=ADVANCED_FACE ( 'NONE', ( #5593 ), #51791, .T. ) ;
#31872=VERTEX_POINT ( 'NONE', #25862 ) ;
#31876=CARTESIAN_POINT ( 'NONE',  ( -37.00000000000000711, -11.10408318471063716, 6.265926637539457111 ) ) ;
#31877=AXIS2_PLACEMENT_3D ( 'NONE', #35523, #55820, #21205 ) ;
#31878=CYLINDRICAL_SURFACE ( 'NONE', #5521, 5.000000000000000888 ) ;
#31879=VECTOR ( 'NONE', #19815, 1000.000000000000000 ) ;
#31880=CARTESIAN_POINT ( 'NONE',  ( -36.00000000000000711, -6.564808257521847601, 10.93004082984016456 ) ) ;
#31881=LINE ( 'NONE', #26918, #65632 ) ;
#31882=AXIS2_PLACEMENT_3D ( 'NONE', #23949, #13610, #34551 ) ;
#31883=ORIENTED_EDGE ( 'NONE', *, *, #7586, .F. ) ;
#31885=ORIENTED_EDGE ( 'NONE', *, *, #22635, .T. ) ;
#31886=CARTESIAN_POINT ( 'NONE',  ( -10.95212338237647920, -9.902220863987562183, -9.175839033069911110 ) ) ;
#31889=ADVANCED_FACE ( 'NONE', ( #15848 ), #42104, .T. ) ;
#31890=CARTESIAN_POINT ( 'NONE',  ( -35.00000000000000000, 9.348667969174405457, 7.817492529713891081 ) ) ;
#31891=DIRECTION ( 'NONE',  ( 0.000000000000000000, -0.01356324068817991481, 0.9999080150203990547 ) ) ;
#31892=CARTESIAN_POINT ( 'NONE',  ( -19.47984447937493613, -3.750539801530005768, -11.39883551934754102 ) ) ;
#31893=AXIS2_PLACEMENT_3D ( 'NONE', #60326, #59049, #59688 ) ;
#31896=VECTOR ( 'NONE', #6241, 1000.000000000000000 ) ;
#31897=ORIENTED_EDGE ( 'NONE', *, *, #15701, .F. ) ;
#31898=CARTESIAN_POINT ( 'NONE',  ( 29.51976981715666781, -7.690765383426355406, 11.09513982864076276 ) ) ;
#31900=CARTESIAN_POINT ( 'NONE',  ( -47.00000000000000711, 0.000000000000000000, 0.000000000000000000 ) ) ;
#31903=ORIENTED_EDGE ( 'NONE', *, *, #44712, .F. ) ;
#31904=DIRECTION ( 'NONE',  ( -1.000000000000000000, -0.000000000000000000, 0.000000000000000000 ) ) ;
#31906=CIRCLE ( 'NONE', #37177, 5.000000000000001776 ) ;
#31908=CARTESIAN_POINT ( 'NONE',  ( -3.838337227274802643, 9.927591105267911331, 9.157165592576390623 ) ) ;
#31909=EDGE_CURVE ( 'NONE', #64690, #22968, #15659, .T. ) ;
#31910=EDGE_CURVE ( 'NONE', #39733, #37251, #52855, .T. ) ;
#31911=EDGE_CURVE ( 'NONE', #11560, #64240, #58176, .T. ) ;
#31912=CIRCLE ( 'NONE', #29767, 12.75000000000000178 ) ;
#31914=ORIENTED_EDGE ( 'NONE', *, *, #27322, .T. ) ;
#31915=CARTESIAN_POINT ( 'NONE',  ( -37.00000000000000711, -2.696588552978969044, -12.46157735505192399 ) ) ;
#31916=EDGE_CURVE ( 'NONE', #63728, #27622, #50763, .T. ) ;
#31917=CIRCLE ( 'NONE', #19160, 5.000000000000000000 ) ;
#31919=CIRCLE ( 'NONE', #18129, 5.000000000000000000 ) ;
#31920=VECTOR ( 'NONE', #33811, 1000.000000000000000 ) ;
#31922=ORIENTED_EDGE ( 'NONE', *, *, #33147, .F. ) ;
#31923=DIRECTION ( 'NONE',  ( 0.000000000000000000, -0.01356324068817991828, 0.9999080150203990547 ) ) ;
#31924=VECTOR ( 'NONE', #2219, 1000.000000000000000 ) ;
#31925=DIRECTION ( 'NONE',  ( -0.000000000000000000, -1.000000000000000000, -0.000000000000000000 ) ) ;
#31926=DIRECTION ( 'NONE',  ( 1.000000000000000000, -0.000000000000000000, 0.000000000000000000 ) ) ;
#31927=CARTESIAN_POINT ( 'NONE',  ( 37.00000000000000711, -3.916263239775270577, 11.07407352312216453 ) ) ;
#31930=ORIENTED_EDGE ( 'NONE', *, *, #5809, .T. ) ;
#31931=CARTESIAN_POINT ( 'NONE',  ( 26.76925746416558383, -11.45732145772444710, 3.578150596242692050 ) ) ;
#31932=AXIS2_PLACEMENT_3D ( 'NONE', #40120, #4243, #35472 ) ;
#31935=VERTEX_POINT ( 'NONE', #17525 ) ;
#31937=AXIS2_PLACEMENT_3D ( 'NONE', #50077, #4535, #40401 ) ;
#31938=AXIS2_PLACEMENT_3D ( 'NONE', #42807, #16237, #26871 ) ;
#31939=CYLINDRICAL_SURFACE ( 'NONE', #11968, 13.50000000000000178 ) ;
#31940=EDGE_CURVE ( 'NONE', #26553, #20972, #29496, .T. ) ;
#31941=ORIENTED_EDGE ( 'NONE', *, *, #13868, .F. ) ;
#31943=CARTESIAN_POINT ( 'NONE',  ( -35.00000000000000000, 0.000000000000000000, 0.000000000000000000 ) ) ;
#31944=DIRECTION ( 'NONE',  ( 0.000000000000000000, 0.01356324068817992175, -0.9999080150203990547 ) ) ;
#31946=AXIS2_PLACEMENT_3D ( 'NONE', #33093, #32745, #649 ) ;
#31947=CARTESIAN_POINT ( 'NONE',  ( 37.00000000000000711, 4.705694406421931860E-17, -3.469127814946512892E-15 ) ) ;
#31953=FACE_OUTER_BOUND ( 'NONE', #59944, .T. ) ;
#31954=DIRECTION ( 'NONE',  ( -0.000000000000000000, -1.000000000000000000, -0.000000000000000000 ) ) ;
#31955=CARTESIAN_POINT ( 'NONE',  ( 37.00000000000000711, -7.251710744571640888, -9.240395740215610942 ) ) ;
#31956=CARTESIAN_POINT ( 'NONE',  ( 36.00000000000000711, 12.74068829017553917, 0.4871980014161889083 ) ) ;
#31962=CIRCLE ( 'NONE', #45785, 5.000000000000000888 ) ;
#31963=VERTEX_POINT ( 'NONE', #23156 ) ;
#31964=FACE_OUTER_BOUND ( 'NONE', #2729, .T. ) ;
#31965=DIRECTION ( 'NONE',  ( 0.000000000000000000, -0.01356324068818000848, 0.9999080150203990547 ) ) ;
#31966=CIRCLE ( 'NONE', #3337, 12.75000000000000178 ) ;
#31967=EDGE_CURVE ( 'NONE', #55740, #22166, #834, .T. ) ;
#31969=ORIENTED_EDGE ( 'NONE', *, *, #4307, .T. ) ;
#31972=DIRECTION ( 'NONE',  ( 0.000000000000000000, -0.01356324068817998940, 0.9999080150203990547 ) ) ;
#31976=AXIS2_PLACEMENT_3D ( 'NONE', #11079, #6100, #30371 ) ;
#31977=EDGE_LOOP ( 'NONE', ( #44213, #6387, #60505, #51385 ) ) ;
#31979=CARTESIAN_POINT ( 'NONE',  ( 8.437200413559441614, 4.476360154859203355, -11.13383131558893346 ) ) ;
#31983=DIRECTION ( 'NONE',  ( -1.000000000000000000, 0.000000000000000000, 0.000000000000000000 ) ) ;
#31985=VECTOR ( 'NONE', #32563, 1000.000000000000000 ) ;
#31986=AXIS2_PLACEMENT_3D ( 'NONE', #49526, #3964, #24227 ) ;
#31987=EDGE_CURVE ( 'NONE', #52675, #46377, #47580, .T. ) ;
#31991=DIRECTION ( 'NONE',  ( 1.000000000000000000, 0.000000000000000000, 0.000000000000000000 ) ) ;
#31993=DIRECTION ( 'NONE',  ( 0.000000000000000000, -0.01356324068817998940, 0.9999080150203990547 ) ) ;
#31994=DIRECTION ( 'NONE',  ( 0.000000000000000000, 0.1118654143051546479, 0.9937233664769768993 ) ) ;
#31995=CYLINDRICAL_SURFACE ( 'NONE', #64065, 12.18650000000000055 ) ;
#31998=CYLINDRICAL_SURFACE ( 'NONE', #8694, 4.999999999999999112 ) ;
#32000=AXIS2_PLACEMENT_3D ( 'NONE', #12920, #22583, #17600 ) ;
#32003=CARTESIAN_POINT ( 'NONE',  ( -35.00000000000000000, -4.946702696913093611, -11.13736569743279681 ) ) ;
#32004=ORIENTED_EDGE ( 'NONE', *, *, #18933, .T. ) ;
#32005=AXIS2_PLACEMENT_3D ( 'NONE', #4, #16293, #56185 ) ;
#32006=AXIS2_PLACEMENT_3D ( 'NONE', #25732, #56981, #56303 ) ;
#32009=DIRECTION ( 'NONE',  ( -1.000000000000000000, 0.000000000000000000, 0.000000000000000000 ) ) ;
#32011=ORIENTED_EDGE ( 'NONE', *, *, #39260, .T. ) ;
#32012=CIRCLE ( 'NONE', #54413, 12.75000000000000178 ) ;
#32015=VECTOR ( 'NONE', #13437, 1000.000000000000000 ) ;
#32016=ORIENTED_EDGE ( 'NONE', *, *, #42888, .F. ) ;
#32017=DIRECTION ( 'NONE',  ( 1.000000000000000000, 0.000000000000000000, 0.000000000000000000 ) ) ;
#32021=EDGE_CURVE ( 'NONE', #21361, #21283, #48119, .T. ) ;
#32022=ORIENTED_EDGE ( 'NONE', *, *, #6903, .T. ) ;
#32024=CARTESIAN_POINT ( 'NONE',  ( -4.989057617119011745, -0.9162120371760335003, -11.96497202265568660 ) ) ;
#32028=VERTEX_POINT ( 'NONE', #63373 ) ;
#32029=CARTESIAN_POINT ( 'NONE',  ( 36.00000000000000711, -12.70128625845191728, 1.113475361586617307 ) ) ;
#32034=VECTOR ( 'NONE', #49541, 1000.000000000000000 ) ;
#32035=FACE_OUTER_BOUND ( 'NONE', #54943, .T. ) ;
#32038=ORIENTED_EDGE ( 'NONE', *, *, #5555, .F. ) ;
#32039=EDGE_CURVE ( 'NONE', #23644, #64143, #35883, .T. ) ;
#32040=DIRECTION ( 'NONE',  ( 0.000000000000000000, 0.01356324068817998940, -0.9999080150203990547 ) ) ;
#32045=ORIENTED_EDGE ( 'NONE', *, *, #65454, .F. ) ;
#32047=VERTEX_POINT ( 'NONE', #18176 ) ;
#32048=EDGE_LOOP ( 'NONE', ( #7157, #6375, #29757, #25153 ) ) ;
#32049=AXIS2_PLACEMENT_3D ( 'NONE', #33384, #53680, #8119 ) ;
#32050=CARTESIAN_POINT ( 'NONE',  ( -35.00000000000000000, 0.000000000000000000, 0.000000000000000000 ) ) ;
#32051=CYLINDRICAL_SURFACE ( 'NONE', #28360, 13.50000000000000178 ) ;
#32052=CARTESIAN_POINT ( 'NONE',  ( -35.00000000000000000, -9.733281772932219411, 8.235637554476609168 ) ) ;
#32056=B_SPLINE_CURVE_WITH_KNOTS ( 'NONE', 3,
 ( #20677, #31306, #62524, #51927, #10676, #55919, #52259, #51607, #21317, #5729 ),
 .UNSPECIFIED., .F., .F.,
 ( 4, 2, 2, 2, 4 ),
 ( 0.005844473438883908585, 0.006520250652290781289, 0.007196027865697654860, 0.007871805079104527564, 0.008547582292511400268 ),
 .UNSPECIFIED. ) ;
#32058=AXIS2_PLACEMENT_3D ( 'NONE', #16623, #56186, #14394 ) ;
#32061=AXIS2_PLACEMENT_3D ( 'NONE', #4256, #58235, #2045 ) ;
#32063=CIRCLE ( 'NONE', #38484, 12.18650000000000055 ) ;
#32064=DIRECTION ( 'NONE',  ( -1.000000000000000000, 0.000000000000000000, 0.000000000000000000 ) ) ;
#32066=DIRECTION ( 'NONE',  ( -0.4298323628305344979, -0.9029087107030918657, 0.000000000000000000 ) ) ;
#32067=ORIENTED_EDGE ( 'NONE', *, *, #50831, .F. ) ;
#32069=EDGE_CURVE ( 'NONE', #31780, #62820, #22165, .T. ) ;
#32070=DIRECTION ( 'NONE',  ( 1.000000000000000000, -0.000000000000000000, 0.000000000000000000 ) ) ;
#32071=DIRECTION ( 'NONE',  ( -1.000000000000000000, 0.000000000000000000, 0.000000000000000000 ) ) ;
#32072=CARTESIAN_POINT ( 'NONE',  ( -25.74864769002726561, -4.845157721295400677, 10.98320407977280055 ) ) ;
#32073=AXIS2_PLACEMENT_3D ( 'NONE', #55093, #14832, #35117 ) ;
#32075=CIRCLE ( 'NONE', #261, 5.000000000000000000 ) ;
#32076=CARTESIAN_POINT ( 'NONE',  ( 9.042385582766643282, 3.534140635374256600, -13.03150467260951295 ) ) ;
#32077=CARTESIAN_POINT ( 'NONE',  ( -25.68256394590837033, -11.85982374565230124, 6.450774052159548688 ) ) ;
#32079=CARTESIAN_POINT ( 'NONE',  ( 37.00000000000000711, -2.968224442958486975, -11.81949347079746282 ) ) ;
#32081=LINE ( 'NONE', #52398, #42688 ) ;
#32082=AXIS2_PLACEMENT_3D ( 'NONE', #48507, #28529, #7602 ) ;
#32086=DIRECTION ( 'NONE',  ( -1.000000000000000000, 0.000000000000000000, -0.000000000000000000 ) ) ;
#32088=ORIENTED_EDGE ( 'NONE', *, *, #29089, .F. ) ;
#32089=DIRECTION ( 'NONE',  ( -1.000000000000000000, 0.000000000000000000, 0.000000000000000000 ) ) ;
#32090=ADVANCED_FACE ( 'NONE', ( #42766 ), #32775, .T. ) ;
#32091=DIRECTION ( 'NONE',  ( 0.000000000000000000, 0.3807014730195220631, -0.9246979985058721985 ) ) ;
#32092=ORIENTED_EDGE ( 'NONE', *, *, #47148, .F. ) ;
#32093=DIRECTION ( 'NONE',  ( 0.000000000000000000, 0.01356324068818000848, -0.9999080150203990547 ) ) ;
#32094=CIRCLE ( 'NONE', #55468, 5.000000000000000888 ) ;
#32095=CARTESIAN_POINT ( 'NONE',  ( -35.00000000000000000, -9.752226076388847531, -6.547236723514122225 ) ) ;
#32096=CARTESIAN_POINT ( 'NONE',  ( -37.00000000000000711, -11.56998259273174945, -3.827046518385204266 ) ) ;
#32097=DIRECTION ( 'NONE',  ( 0.7884253166185480888, 0.000000000000000000, -0.6151304903148129277 ) ) ;
#32098=ADVANCED_FACE ( 'NONE', ( #43099 ), #26382, .T. ) ;
#32102=CARTESIAN_POINT ( 'NONE',  ( 37.00000000000000711, -9.348667969174460524, -7.817492529713823579 ) ) ;
#32104=ORIENTED_EDGE ( 'NONE', *, *, #41227, .T. ) ;
#32105=EDGE_CURVE ( 'NONE', #42804, #31183, #11453, .T. ) ;
#32108=DIRECTION ( 'NONE',  ( -1.000000000000000000, -0.000000000000000000, 0.000000000000000000 ) ) ;
#32109=VERTEX_POINT ( 'NONE', #37002 ) ;
#32112=VECTOR ( 'NONE', #37894, 1000.000000000000000 ) ;
#32113=CARTESIAN_POINT ( 'NONE',  ( -35.00000000000000000, 5.143145423404449801, -11.66664283989674367 ) ) ;
#32114=CIRCLE ( 'NONE', #3493, 5.000000000000000888 ) ;
#32115=EDGE_CURVE ( 'NONE', #27902, #63537, #6774, .T. ) ;
#32116=DIRECTION ( 'NONE',  ( 1.000000000000000000, 0.000000000000000000, 0.000000000000000000 ) ) ;
#32118=DIRECTION ( 'NONE',  ( 1.000000000000000000, -0.000000000000000000, -0.000000000000000000 ) ) ;
#32120=ADVANCED_FACE ( 'NONE', ( #7083 ), #46665, .T. ) ;
#32121=ORIENTED_EDGE ( 'NONE', *, *, #10407, .F. ) ;
#32122=ORIENTED_EDGE ( 'NONE', *, *, #35984, .F. ) ;
#32124=EDGE_LOOP ( 'NONE', ( #44990, #52365, #12381, #25135 ) ) ;
#32125=CARTESIAN_POINT ( 'NONE',  ( 35.00000000000000000, 4.705694406421931860E-17, -3.469127814946512892E-15 ) ) ;
#32127=CARTESIAN_POINT ( 'NONE',  ( 12.52750123246316072, 0.4973700281276248192, 13.49083477977253764 ) ) ;
#32128=DIRECTION ( 'NONE',  ( 1.000000000000000000, -0.000000000000000000, 0.000000000000000000 ) ) ;
#32130=CARTESIAN_POINT ( 'NONE',  ( 37.00000000000000711, 11.68758509253246558, -1.171570255487653700 ) ) ;
#32131=EDGE_CURVE ( 'NONE', #52959, #64071, #6161, .T. ) ;
#32133=ORIENTED_EDGE ( 'NONE', *, *, #25523, .F. ) ;
#32135=ORIENTED_EDGE ( 'NONE', *, *, #63274, .T. ) ;
#32136=CIRCLE ( 'NONE', #1415, 5.000000000000000888 ) ;
#32137=CARTESIAN_POINT ( 'NONE',  ( 35.00000000000000000, -11.68758509253247091, 1.171570255487570655 ) ) ;
#32139=LINE ( 'NONE', #31494, #58396 ) ;
#32142=VERTEX_POINT ( 'NONE', #51679 ) ;
#32144=DIRECTION ( 'NONE',  ( 0.000000000000000000, 0.01356324068817992695, -0.9999080150203990547 ) ) ;
#32146=FACE_OUTER_BOUND ( 'NONE', #17251, .T. ) ;
#32148=DIRECTION ( 'NONE',  ( 1.000000000000000000, 0.000000000000000000, 0.000000000000000000 ) ) ;
#32150=ORIENTED_EDGE ( 'NONE', *, *, #32469, .F. ) ;
#32151=CIRCLE ( 'NONE', #3530, 12.74999999999999822 ) ;
#32154=CARTESIAN_POINT ( 'NONE',  ( -29.68541646480307605, -0.9874700634933176735, -13.47073127497727363 ) ) ;
#32156=CIRCLE ( 'NONE', #31088, 4.999999999999999112 ) ;
#32157=ADVANCED_FACE ( 'NONE', ( #26072 ), #62594, .T. ) ;
#32160=ORIENTED_EDGE ( 'NONE', *, *, #56771, .T. ) ;
#32161=CIRCLE ( 'NONE', #50284, 12.18650000000000055 ) ;
#32166=AXIS2_PLACEMENT_3D ( 'NONE', #60364, #14792, #9822 ) ;
#32167=CARTESIAN_POINT ( 'NONE',  ( -35.00000000000000000, 0.000000000000000000, 0.000000000000000000 ) ) ;
#32168=CARTESIAN_POINT ( 'NONE',  ( -3.740102306720532788, 25.00000000000000000, -6.044082642436763742 ) ) ;
#32169=VECTOR ( 'NONE', #26152, 1000.000000000000000 ) ;
#32170=EDGE_CURVE ( 'NONE', #49222, #42435, #61300, .T. ) ;
#32171=ORIENTED_EDGE ( 'NONE', *, *, #37615, .F. ) ;
#32173=LINE ( 'NONE', #17565, #27632 ) ;
#32174=VERTEX_POINT ( 'NONE', #37338 ) ;
#32175=CARTESIAN_POINT ( 'NONE',  ( 2.091509324218079335, 2.103201000890800199, 11.81927150886677502 ) ) ;
#32177=CARTESIAN_POINT ( 'NONE',  ( 22.36482863261543486, -13.46837713145126791, -0.9234811557364140944 ) ) ;
#32179=CARTESIAN_POINT ( 'NONE',  ( -35.00000000000000000, 6.917234959366964198, -9.493370459201624811 ) ) ;
#32183=CARTESIAN_POINT ( 'NONE',  ( -10.25071159343468352, -3.780199704946288985, 11.39050396304778268 ) ) ;
#32184=ORIENTED_EDGE ( 'NONE', *, *, #20418, .T. ) ;
#32185=EDGE_CURVE ( 'NONE', #53581, #57915, #10757, .T. ) ;
#32186=ORIENTED_EDGE ( 'NONE', *, *, #40830, .T. ) ;
#32187=DIRECTION ( 'NONE',  ( 0.000000000000000000, 0.01356324068818000328, -0.9999080150203990547 ) ) ;
#32188=VERTEX_POINT ( 'NONE', #16422 ) ;
#32189=FILL_AREA_STYLE_COLOUR ( '', #52602 ) ;
#32192=AXIS2_PLACEMENT_3D ( 'NONE', #64372, #15142, #24147 ) ;
#32196=CARTESIAN_POINT ( 'NONE',  ( 35.00000000000000000, 11.74226168163341377, 0.3025107581129941048 ) ) ;
#32201=ORIENTED_EDGE ( 'NONE', *, *, #12436, .T. ) ;
#32202=CARTESIAN_POINT ( 'NONE',  ( 3.369063103260706793, 5.393734308210048845, 12.37743201445020347 ) ) ;
#32204=ORIENTED_EDGE ( 'NONE', *, *, #31011, .T. ) ;
#32208=ORIENTED_EDGE ( 'NONE', *, *, #44443, .T. ) ;
#32212=CIRCLE ( 'NONE', #40718, 12.18650000000000055 ) ;
#32213=B_SPLINE_CURVE_WITH_KNOTS ( 'NONE', 3,
 ( #34535, #30518, #15557, #35817, #50822, #24560 ),
 .UNSPECIFIED., .F., .F.,
 ( 4, 2, 4 ),
 ( 0.005435758617312099611, 0.006631938927966533892, 0.007828119238620968173 ),
 .UNSPECIFIED. ) ;
#32216=CARTESIAN_POINT ( 'NONE',  ( -37.00000000000000711, -8.029056188533626681, -8.573591947375405198 ) ) ;
#32217=DIRECTION ( 'NONE',  ( 0.7884253166185480888, 0.000000000000000000, -0.6151304903148129277 ) ) ;
#32218=ORIENTED_EDGE ( 'NONE', *, *, #49724, .F. ) ;
#32219=EDGE_CURVE ( 'NONE', #815, #26332, #48634, .T. ) ;
#32221=ORIENTED_EDGE ( 'NONE', *, *, #42615, .T. ) ;
#32222=CYLINDRICAL_SURFACE ( 'NONE', #35924, 5.000000000000000888 ) ;
#32223=AXIS2_PLACEMENT_3D ( 'NONE', #58512, #12278, #2676 ) ;
#32228=AXIS2_PLACEMENT_3D ( 'NONE', #23601, #48870, #64154 ) ;
#32229=CARTESIAN_POINT ( 'NONE',  ( -37.00000000000000711, 10.91072401419410554, 5.428340790341743549 ) ) ;
#32230=CYLINDRICAL_SURFACE ( 'NONE', #65234, 5.000000000000000888 ) ;
#32232=ORIENTED_EDGE ( 'NONE', *, *, #21823, .F. ) ;
#32234=CIRCLE ( 'NONE', #62992, 5.000000000000000888 ) ;
#32235=VERTEX_POINT ( 'NONE', #17401 ) ;
#32238=AXIS2_PLACEMENT_3D ( 'NONE', #11613, #37872, #42853 ) ;
#32241=DIRECTION ( 'NONE',  ( -1.000000000000000000, 0.000000000000000000, -0.000000000000000000 ) ) ;
#32242=VERTEX_POINT ( 'NONE', #7396 ) ;
#32245=DIRECTION ( 'NONE',  ( -0.000000000000000000, -0.000000000000000000, -1.000000000000000000 ) ) ;
#32246=CARTESIAN_POINT ( 'NONE',  ( -3.992466187133344668, 11.80999507292766992, 6.552767039380011482 ) ) ;
#32248=AXIS2_PLACEMENT_3D ( 'NONE', #55183, #25580, #40204 ) ;
#32253=CIRCLE ( 'NONE', #19604, 5.000000000000000000 ) ;
#32254=ADVANCED_FACE ( 'NONE', ( #43274 ), #47624, .T. ) ;
#32258=ORIENTED_EDGE ( 'NONE', *, *, #25069, .F. ) ;
#32260=CIRCLE ( 'NONE', #17430, 5.000000000000000000 ) ;
#32262=CARTESIAN_POINT ( 'NONE',  ( 37.00000000000000711, 4.705694406421931860E-17, -3.469127814946512892E-15 ) ) ;
#32263=CIRCLE ( 'NONE', #25929, 5.000000000000000000 ) ;
#32264=LINE ( 'NONE', #57562, #26491 ) ;
#32266=EDGE_CURVE ( 'NONE', #34799, #30454, #18025, .T. ) ;
#32267=AXIS2_PLACEMENT_3D ( 'NONE', #11686, #51310, #31965 ) ;
#32268=VERTEX_POINT ( 'NONE', #18370 ) ;
#32269=ORIENTED_EDGE ( 'NONE', *, *, #24719, .F. ) ;
#32270=CARTESIAN_POINT ( 'NONE',  ( 27.85875306725328571, -11.11252398976967903, 4.542717126716967257 ) ) ;
#32273=ORIENTED_EDGE ( 'NONE', *, *, #5034, .F. ) ;
#32274=DIRECTION ( 'NONE',  ( -1.000000000000000000, 0.000000000000000000, 0.000000000000000000 ) ) ;
#32276=ORIENTED_EDGE ( 'NONE', *, *, #25601, .T. ) ;
#32277=DIRECTION ( 'NONE',  ( -1.000000000000000000, 0.000000000000000000, 0.000000000000000000 ) ) ;
#32278=VECTOR ( 'NONE', #29511, 1000.000000000000000 ) ;
#32279=DIRECTION ( 'NONE',  ( 0.000000000000000000, 0.01356324068817992175, -0.9999080150203990547 ) ) ;
#32280=CARTESIAN_POINT ( 'NONE',  ( 24.51709394181822432, -2.671539114876285037, 11.70037924786635486 ) ) ;
#32283=ORIENTED_EDGE ( 'NONE', *, *, #29958, .F. ) ;
#32284=DIRECTION ( 'NONE',  ( -0.000000000000000000, -0.000000000000000000, -1.000000000000000000 ) ) ;
#32286=EDGE_CURVE ( 'NONE', #18418, #50038, #16771, .T. ) ;
#32287=CARTESIAN_POINT ( 'NONE',  ( -19.69476066079020171, -4.201994156881551312, 11.24025111398909615 ) ) ;
#32288=DIRECTION ( 'NONE',  ( 0.000000000000000000, 0.01356324068817992175, -0.9999080150203990547 ) ) ;
#32290=CYLINDRICAL_SURFACE ( 'NONE', #62208, 12.75000000000000178 ) ;
#32291=CARTESIAN_POINT ( 'NONE',  ( 35.00000000000000000, 4.705694406421931860E-17, -3.469127814946512892E-15 ) ) ;
#32293=CARTESIAN_POINT ( 'NONE',  ( -27.70104025454409680, -11.17792676666258878, -4.374904684088040341 ) ) ;
#32294=ORIENTED_EDGE ( 'NONE', *, *, #40446, .F. ) ;
#32295=ADVANCED_FACE ( 'NONE', ( #13033 ), #47316, .T. ) ;
#32297=ORIENTED_EDGE ( 'NONE', *, *, #32474, .T. ) ;
#32299=DIRECTION ( 'NONE',  ( 0.000000000000000000, -0.5243256840888443904, -0.8515178078024941977 ) ) ;
#32300=EDGE_CURVE ( 'NONE', #6547, #19851, #37976, .T. ) ;
#32301=CIRCLE ( 'NONE', #3678, 5.000000000000000888 ) ;
#32304=AXIS2_PLACEMENT_3D ( 'NONE', #64707, #39447, #35446 ) ;
#32307=ORIENTED_EDGE ( 'NONE', *, *, #35423, .F. ) ;
#32308=ORIENTED_EDGE ( 'NONE', *, *, #21039, .T. ) ;
#32310=ORIENTED_EDGE ( 'NONE', *, *, #36737, .T. ) ;
#32312=DIRECTION ( 'NONE',  ( 0.000000000000000000, 0.3218879778915972878, -0.9467777615094571386 ) ) ;
#32318=AXIS2_PLACEMENT_3D ( 'NONE', #33817, #39802, #34784 ) ;
#32319=EDGE_CURVE ( 'NONE', #55560, #24405, #43288, .T. ) ;
#32320=EDGE_CURVE ( 'NONE', #34385, #12941, #53945, .T. ) ;
#32322=CARTESIAN_POINT ( 'NONE',  ( 47.00000000000000711, 4.705694406421931860E-17, -3.469127814946512892E-15 ) ) ;
#32323=AXIS2_PLACEMENT_3D ( 'NONE', #28350, #63259, #18724 ) ;
#32325=CARTESIAN_POINT ( 'NONE',  ( 35.00000000000000000, 4.705694406421931860E-17, -3.469127814946512892E-15 ) ) ;
#32326=CARTESIAN_POINT ( 'NONE',  ( -37.00000000000000711, 7.146664589318047156, -9.321877890560362090 ) ) ;
#32327=FACE_OUTER_BOUND ( 'NONE', #9041, .T. ) ;
#32333=DIRECTION ( 'NONE',  ( -1.000000000000000000, 0.000000000000000000, 0.000000000000000000 ) ) ;
#32335=VERTEX_POINT ( 'NONE', #57621 ) ;
#32338=ORIENTED_EDGE ( 'NONE', *, *, #53392, .F. ) ;
#32339=LINE ( 'NONE', #37331, #17172 ) ;
#32340=ORIENTED_EDGE ( 'NONE', *, *, #52590, .F. ) ;
#32341=ADVANCED_FACE ( 'NONE', ( #53618 ), #8059, .T. ) ;
#32342=CARTESIAN_POINT ( 'NONE',  ( 37.00000000000000711, 0.4871980014161481631, -12.74068829017554272 ) ) ;
#32343=ORIENTED_EDGE ( 'NONE', *, *, #42275, .T. ) ;
#32346=DIRECTION ( 'NONE',  ( 1.000000000000000000, 0.000000000000000000, -0.000000000000000000 ) ) ;
#32347=ORIENTED_EDGE ( 'NONE', *, *, #21290, .F. ) ;
#32348=CARTESIAN_POINT ( 'NONE',  ( -24.84395261982345104, -8.877669242773048808, 8.075961097281444623 ) ) ;
#32350=DIRECTION ( 'NONE',  ( 0.000000000000000000, 0.01356324068817998940, -0.9999080150203990547 ) ) ;
#32351=DIRECTION ( 'NONE',  ( 1.000000000000000000, 0.000000000000000000, -0.000000000000000000 ) ) ;
#32352=ORIENTED_EDGE ( 'NONE', *, *, #1465, .T. ) ;
#32354=DIRECTION ( 'NONE',  ( -1.000000000000000000, 0.000000000000000000, 0.000000000000000000 ) ) ;
#32357=CARTESIAN_POINT ( 'NONE',  ( 12.52750123246316249, 0.4973700281276248192, -13.49083477977253764 ) ) ;
#32358=ORIENTED_EDGE ( 'NONE', *, *, #23683, .F. ) ;
#32359=CARTESIAN_POINT ( 'NONE',  ( 29.51976981715666781, 4.571419055710094881, 11.09513982864076276 ) ) ;
#32362=DIRECTION ( 'NONE',  ( 0.000000000000000000, -0.01356324068817991828, 0.9999080150203990547 ) ) ;
#32364=DIRECTION ( 'NONE',  ( -1.000000000000000000, 0.000000000000000000, 0.000000000000000000 ) ) ;
#32365=DIRECTION ( 'NONE',  ( 1.000000000000000000, 0.000000000000000000, 0.000000000000000000 ) ) ;
#32366=EDGE_CURVE ( 'NONE', #64587, #12570, #49675, .T. ) ;
#32369=ORIENTED_EDGE ( 'NONE', *, *, #36334, .F. ) ;
#32372=CARTESIAN_POINT ( 'NONE',  ( 35.00000000000000000, -8.699265615723042799, -8.534258022646065811 ) ) ;
#32374=EDGE_CURVE ( 'NONE', #40614, #5549, #28485, .T. ) ;
#32377=ORIENTED_EDGE ( 'NONE', *, *, #19598, .F. ) ;
#32378=ORIENTED_EDGE ( 'NONE', *, *, #44113, .F. ) ;
#32379=DIRECTION ( 'NONE',  ( 1.000000000000000000, -0.000000000000000000, -0.000000000000000000 ) ) ;
#32380=DIRECTION ( 'NONE',  ( 0.000000000000000000, 0.01356324068817998940, -0.9999080150203989437 ) ) ;
#32383=DIRECTION ( 'NONE',  ( 0.000000000000000000, 0.01356324068817998940, -0.9999080150203989437 ) ) ;
#32384=DIRECTION ( 'NONE',  ( 0.000000000000000000, -0.01356324068817991828, 0.9999080150203990547 ) ) ;
#32385=CIRCLE ( 'NONE', #5887, 12.18650000000000055 ) ;
#32392=DIRECTION ( 'NONE',  ( 0.000000000000000000, 0.01356324068817998940, -0.9999080150203990547 ) ) ;
#32393=CARTESIAN_POINT ( 'NONE',  ( 37.00000000000000711, -10.80478261802178075, 5.636262487437428526 ) ) ;
#32395=AXIS2_PLACEMENT_3D ( 'NONE', #53194, #58186, #7641 ) ;
#32396=DIRECTION ( 'NONE',  ( 0.000000000000000000, 0.07632122047555796318, -0.9970832820307045097 ) ) ;
#32397=CARTESIAN_POINT ( 'NONE',  ( 9.949876586531372524, 1.099362317746359841, -11.95077892412715492 ) ) ;
#32398=VERTEX_POINT ( 'NONE', #39608 ) ;
#32400=CYLINDRICAL_SURFACE ( 'NONE', #33511, 12.18650000000000055 ) ;
#32404=EDGE_CURVE ( 'NONE', #2532, #59070, #56582, .T. ) ;
#32405=DIRECTION ( 'NONE',  ( 0.000000000000000000, 0.01356324068817998940, -0.9999080150203989437 ) ) ;
#32407=( BOUNDED_CURVE ( )  B_SPLINE_CURVE ( 3, ( #417, #54649, #29656, #9066 ),
 .UNSPECIFIED., .F., .F. ) 
 B_SPLINE_CURVE_WITH_KNOTS ( ( 4, 4 ),
 ( 1.252925267387244856, 1.262475676102403632 ),
 .UNSPECIFIED. ) 
 CURVE ( )  GEOMETRIC_REPRESENTATION_ITEM ( )  RATIONAL_B_SPLINE_CURVE ( ( 1.000000000000000000, 0.9999923991555577096, 0.9999923991555577096, 1.000000000000000000 ) ) 
 REPRESENTATION_ITEM ( '' )  );
#32408=EDGE_LOOP ( 'NONE', ( #32184, #13843, #43647, #1059 ) ) ;
#32409=DIRECTION ( 'NONE',  ( 0.000000000000000000, -0.07632122047555069122, 0.9970832820307048427 ) ) ;
#32410=FACE_OUTER_BOUND ( 'NONE', #65555, .T. ) ;
#32411=CARTESIAN_POINT ( 'NONE',  ( -35.00000000000000000, -4.426194442447158650, -11.35427606708811155 ) ) ;
#32413=ORIENTED_EDGE ( 'NONE', *, *, #6237, .T. ) ;
#32414=CARTESIAN_POINT ( 'NONE',  ( -35.00000000000000000, 10.54834585426219995, 6.102719229070713070 ) ) ;
#32415=LINE ( 'NONE', #56388, #59567 ) ;
#32418=ORIENTED_EDGE ( 'NONE', *, *, #12976, .T. ) ;
#32420=ADVANCED_FACE ( 'NONE', ( #19677 ), #53932, .T. ) ;
#32421=CIRCLE ( 'NONE', #21822, 12.74999999999999822 ) ;
#32422=DIRECTION ( 'NONE',  ( -1.836970198721029688E-16, 1.000000000000000000, 0.000000000000000000 ) ) ;
#32425=DIRECTION ( 'NONE',  ( 1.000000000000000000, 0.000000000000000000, 0.000000000000000000 ) ) ;
#32426=CYLINDRICAL_SURFACE ( 'NONE', #13109, 4.999999999999999112 ) ;
#32427=CARTESIAN_POINT ( 'NONE',  ( -3.762821804695729799, -12.34140757501883989, 5.486078560323296216 ) ) ;
#32428=DIRECTION ( 'NONE',  ( 0.000000000000000000, 0.01356324068817998940, -0.9999080150203990547 ) ) ;
#32429=CARTESIAN_POINT ( 'NONE',  ( -10.48620311856347875, -9.720786832536937538, 9.367833439828908482 ) ) ;
#32430=EDGE_LOOP ( 'NONE', ( #36717, #27891, #41506, #19441 ) ) ;
#32431=LINE ( 'NONE', #57742, #52147 ) ;
#32434=ORIENTED_EDGE ( 'NONE', *, *, #12383, .T. ) ;
#32436=CARTESIAN_POINT ( 'NONE',  ( -14.29135464769095520, 7.782112657557433089, 25.00000000000000000 ) ) ;
#32437=CARTESIAN_POINT ( 'NONE',  ( 24.82652845881425208, 8.390869743685042792, -8.578654028722157321 ) ) ;
#32438=EDGE_CURVE ( 'NONE', #665, #48033, #57187, .T. ) ;
#32439=CARTESIAN_POINT ( 'NONE',  ( 36.00000000000000711, -4.824807283154208370, -11.80185301892979410 ) ) ;
#32442=ORIENTED_EDGE ( 'NONE', *, *, #16548, .T. ) ;
#32443=CIRCLE ( 'NONE', #19751, 12.18650000000000055 ) ;
#32445=CARTESIAN_POINT ( 'NONE',  ( 1.657328813023050129, 0.7084331564875310239, -13.50016122470280244 ) ) ;
#32447=VERTEX_POINT ( 'NONE', #34291 ) ;
#32449=VERTEX_POINT ( 'NONE', #54605 ) ;
#32450=CARTESIAN_POINT ( 'NONE',  ( -47.00000000000000711, 0.000000000000000000, 0.000000000000000000 ) ) ;
#32451=CARTESIAN_POINT ( 'NONE',  ( -37.00000000000000711, -11.60979404548637639, 3.704519465651264110 ) ) ;
#32452=CARTESIAN_POINT ( 'NONE',  ( 10.10417271913525106, 1.641784628707440685, 13.40109299532181986 ) ) ;
#32453=AXIS2_PLACEMENT_3D ( 'NONE', #19727, #30345, #40640 ) ;
#32459=ORIENTED_EDGE ( 'NONE', *, *, #55556, .F. ) ;
#32462=DIRECTION ( 'NONE',  ( -1.000000000000000000, -0.000000000000000000, -0.000000000000000000 ) ) ;
#32463=LINE ( 'NONE', #36812, #10460 ) ;
#32464=DIRECTION ( 'NONE',  ( 0.000000000000000000, 0.000000000000000000, -1.000000000000000000 ) ) ;
#32465=DIRECTION ( 'NONE',  ( 0.000000000000000000, -0.6745969609292555846, -0.7381862504172050921 ) ) ;
#32467=ORIENTED_EDGE ( 'NONE', *, *, #55409, .T. ) ;
#32469=EDGE_CURVE ( 'NONE', #61052, #60345, #48690, .T. ) ;
#32472=CARTESIAN_POINT ( 'NONE',  ( -28.41827485489077532, 3.509237424706437292, -11.47541949982828413 ) ) ;
#32474=EDGE_CURVE ( 'NONE', #42325, #60445, #44578, .T. ) ;
#32475=CARTESIAN_POINT ( 'NONE',  ( 36.00000000000000711, 4.074242145636175039, 12.08151691381185167 ) ) ;
#32476=ORIENTED_EDGE ( 'NONE', *, *, #11242, .T. ) ;
#32477=CARTESIAN_POINT ( 'NONE',  ( -35.00000000000000000, -12.46157735505190978, 2.696588552979012121 ) ) ;
#32481=EDGE_CURVE ( 'NONE', #28364, #8833, #65516, .T. ) ;
#32482=VECTOR ( 'NONE', #32676, 1000.000000000000000 ) ;
#32484=DIRECTION ( 'NONE',  ( 0.000000000000000000, 0.01356324068817992001, -0.9999080150203990547 ) ) ;
#32485=ORIENTED_EDGE ( 'NONE', *, *, #3552, .T. ) ;
#32487=ORIENTED_EDGE ( 'NONE', *, *, #61329, .T. ) ;
#32488=DIRECTION ( 'NONE',  ( 1.000000000000000000, -0.000000000000000000, 0.000000000000000000 ) ) ;
#32493=ORIENTED_EDGE ( 'NONE', *, *, #31371, .T. ) ;
#32494=ORIENTED_EDGE ( 'NONE', *, *, #21642, .F. ) ;
#32496=ADVANCED_FACE ( 'NONE', ( #24649 ), #58945, .T. ) ;
#32498=CARTESIAN_POINT ( 'NONE',  ( 3.142368856636166274, 4.338277973535410226, 11.19578891466989212 ) ) ;
#32502=DIRECTION ( 'NONE',  ( 1.000000000000000000, 0.000000000000000000, -0.000000000000000000 ) ) ;
#32506=ORIENTED_EDGE ( 'NONE', *, *, #16389, .F. ) ;
#32509=CARTESIAN_POINT ( 'NONE',  ( 23.57534446543221307, -11.05662876997433486, -7.751112723597799459 ) ) ;
#32510=CYLINDRICAL_SURFACE ( 'NONE', #36438, 4.285769192180103992 ) ;
#32514=LINE ( 'NONE', #47514, #56670 ) ;
#32515=DIRECTION ( 'NONE',  ( -1.000000000000000000, 0.000000000000000000, 0.000000000000000000 ) ) ;
#32517=ORIENTED_EDGE ( 'NONE', *, *, #54965, .F. ) ;
#32518=ORIENTED_EDGE ( 'NONE', *, *, #2489, .T. ) ;
#32519=DIRECTION ( 'NONE',  ( 1.000000000000000000, -0.000000000000000000, 0.000000000000000000 ) ) ;
#32520=ORIENTED_EDGE ( 'NONE', *, *, #21091, .F. ) ;
#32522=CYLINDRICAL_SURFACE ( 'NONE', #58882, 4.000030059823568074 ) ;
#32523=ORIENTED_EDGE ( 'NONE', *, *, #7728, .T. ) ;
#32524=ORIENTED_EDGE ( 'NONE', *, *, #62909, .T. ) ;
#32528=PLANE ( 'NONE',  #53308 ) ;
#32530=DIRECTION ( 'NONE',  ( 1.000000000000000000, 0.000000000000000000, -0.000000000000000000 ) ) ;
#32532=DIRECTION ( 'NONE',  ( 0.000000000000000000, -0.01356324068817998940, 0.9999080150203990547 ) ) ;
#32533=ORIENTED_EDGE ( 'NONE', *, *, #18549, .T. ) ;
#32534=DIRECTION ( 'NONE',  ( -1.000000000000000000, 0.000000000000000000, 0.000000000000000000 ) ) ;
#32535=DIRECTION ( 'NONE',  ( 1.000000000000000000, -0.000000000000000000, 0.000000000000000000 ) ) ;
#32538=FACE_OUTER_BOUND ( 'NONE', #54800, .T. ) ;
#32541=EDGE_CURVE ( 'NONE', #47095, #36349, #46539, .T. ) ;
#32543=FACE_OUTER_BOUND ( 'NONE', #11824, .T. ) ;
#32544=ORIENTED_EDGE ( 'NONE', *, *, #54484, .T. ) ;
#32547=CARTESIAN_POINT ( 'NONE',  ( -37.00000000000000711, -3.287724142101498437, 11.73463472867575064 ) ) ;
#32551=DIRECTION ( 'NONE',  ( 0.000000000000000000, -0.01356324068817998940, 0.9999080150203990547 ) ) ;
#32552=ORIENTED_EDGE ( 'NONE', *, *, #55172, .T. ) ;
#32556=CARTESIAN_POINT ( 'NONE',  ( -35.00000000000000000, 7.817492529713985228, -9.348667969174325520 ) ) ;
#32560=EDGE_CURVE ( 'NONE', #7338, #28155, #50908, .T. ) ;
#32563=DIRECTION ( 'NONE',  ( -0.000000000000000000, -0.000000000000000000, -1.000000000000000000 ) ) ;
#32564=AXIS2_PLACEMENT_3D ( 'NONE', #16522, #57086, #51462 ) ;
#32565=B_SPLINE_CURVE_WITH_KNOTS ( 'NONE', 3,
 ( #55756, #10187, #30468, #870, #11182, #564, #61706, #16164, #47425, #20827, #57066, #11494, #61069, #1861, #6201, #21141, #56398, #31765 ),
 .UNSPECIFIED., .F., .F.,
 ( 4, 2, 2, 2, 2, 2, 2, 2, 4 ),
 ( 4.336808689942017736E-18, 0.001081547705042592211, 0.002163095410085180085, 0.003244643115127768176, 0.004326190820170354966, 0.005407738525212942189, 0.006489286230255530280, 0.007570833935298119238, 0.008652381640340704727 ),
 .UNSPECIFIED. ) ;
#32566=AXIS2_PLACEMENT_3D ( 'NONE', #28598, #32274, #57906 ) ;
#32567=ORIENTED_EDGE ( 'NONE', *, *, #57357, .T. ) ;
#32568=DIRECTION ( 'NONE',  ( 0.000000000000000000, -0.01356324068817992175, 0.9999080150203990547 ) ) ;
#32569=ADVANCED_FACE ( 'NONE', ( #20309 ), #25973, .T. ) ;
#32571=CARTESIAN_POINT ( 'NONE',  ( 12.52750123246316249, 0.4973700281276248192, -13.49083477977253764 ) ) ;
#32573=FACE_OUTER_BOUND ( 'NONE', #63290, .T. ) ;
#32574=CARTESIAN_POINT ( 'NONE',  ( -29.43980975494970309, -3.641506875706030488, 12.99959336572439561 ) ) ;
#32575=EDGE_CURVE ( 'NONE', #41887, #41521, #34435, .T. ) ;
#32578=EDGE_LOOP ( 'NONE', ( #13623, #3058, #47368, #38055 ) ) ;
#32579=ORIENTED_EDGE ( 'NONE', *, *, #52349, .T. ) ;
#32582=VERTEX_POINT ( 'NONE', #26289 ) ;
#32584=DIRECTION ( 'NONE',  ( -1.000000000000000000, 0.000000000000000000, 0.000000000000000000 ) ) ;
#32585=ORIENTED_EDGE ( 'NONE', *, *, #669, .F. ) ;
#32587=DIRECTION ( 'NONE',  ( 1.000000000000000000, 0.000000000000000000, 0.000000000000000000 ) ) ;
#32590=EDGE_CURVE ( 'NONE', #60004, #12123, #54955, .T. ) ;
#32591=ORIENTED_EDGE ( 'NONE', *, *, #57622, .T. ) ;
#32592=ORIENTED_EDGE ( 'NONE', *, *, #52298, .F. ) ;
#32593=DIRECTION ( 'NONE',  ( 0.000000000000000000, -0.01356324068817991828, 0.9999080150203990547 ) ) ;
#32594=ORIENTED_EDGE ( 'NONE', *, *, #31461, .T. ) ;
#32595=CARTESIAN_POINT ( 'NONE',  ( 9.960423179593171028, 1.090233323514599340, -13.45698435061968290 ) ) ;
#32596=ORIENTED_EDGE ( 'NONE', *, *, #59320, .F. ) ;
#32599=CARTESIAN_POINT ( 'NONE',  ( 35.00000000000000000, -11.53507381115584529, -2.216820770815045805 ) ) ;
#32600=EDGE_CURVE ( 'NONE', #55701, #14200, #51582, .T. ) ;
#32601=CARTESIAN_POINT ( 'NONE',  ( -47.00000000000000711, 0.000000000000000000, 0.000000000000000000 ) ) ;
#32602=CARTESIAN_POINT ( 'NONE',  ( 8.553317268354581060, 3.425949070068618152, 11.50390082272593162 ) ) ;
#32604=DIRECTION ( 'NONE',  ( 0.000000000000000000, -0.2006870767258961963, 0.9796553971857727694 ) ) ;
#32605=ORIENTED_EDGE ( 'NONE', *, *, #9674, .T. ) ;
#32606=DIRECTION ( 'NONE',  ( -1.000000000000000000, -1.836970198721029688E-16, -0.000000000000000000 ) ) ;
#32607=ORIENTED_EDGE ( 'NONE', *, *, #56614, .T. ) ;
#32610=EDGE_LOOP ( 'NONE', ( #46399, #59557, #53502, #33800 ) ) ;
#32611=EDGE_CURVE ( 'NONE', #49577, #55976, #6200, .T. ) ;
#32614=CIRCLE ( 'NONE', #12442, 12.18650000000000055 ) ;
#32616=EDGE_CURVE ( 'NONE', #60341, #30241, #35918, .T. ) ;
#32617=ORIENTED_EDGE ( 'NONE', *, *, #4440, .T. ) ;
#32618=CIRCLE ( 'NONE', #35796, 12.18650000000000411 ) ;
#32619=DIRECTION ( 'NONE',  ( 0.000000000000000000, -0.5243256840888443904, -0.8515178078024941977 ) ) ;
#32620=VERTEX_POINT ( 'NONE', #32556 ) ;
#32621=CARTESIAN_POINT ( 'NONE',  ( -35.00000000000000000, 0.000000000000000000, 0.000000000000000000 ) ) ;
#32622=DIRECTION ( 'NONE',  ( -1.000000000000000000, 0.000000000000000000, 0.000000000000000000 ) ) ;
#32625=CARTESIAN_POINT ( 'NONE',  ( -18.51055391882387369, -5.103712865905460916, 10.86121933613184787 ) ) ;
#32626=ORIENTED_EDGE ( 'NONE', *, *, #61217, .F. ) ;
#32627=CARTESIAN_POINT ( 'NONE',  ( -35.00000000000000000, 8.766823244862097297, -7.817610399097422835 ) ) ;
#32630=ADVANCED_FACE ( 'NONE', ( #21957 ), #2000, .T. ) ;
#32631=CYLINDRICAL_SURFACE ( 'NONE', #45805, 5.000000000000000888 ) ;
#32633=EDGE_CURVE ( 'NONE', #19473, #52495, #19995, .T. ) ;
#32634=CARTESIAN_POINT ( 'NONE',  ( 37.00000000000000711, -12.21925492305364713, -3.640372113593511649 ) ) ;
#32635=DIRECTION ( 'NONE',  ( -1.000000000000000000, 0.000000000000000000, 0.000000000000000000 ) ) ;
#32637=EDGE_CURVE ( 'NONE', #26131, #16803, #25723, .T. ) ;
#32638=ORIENTED_EDGE ( 'NONE', *, *, #10086, .T. ) ;
#32640=DIRECTION ( 'NONE',  ( 0.000000000000000000, -0.9105187689795999351, 0.4134677391718417638 ) ) ;
#32641=CARTESIAN_POINT ( 'NONE',  ( 5.412955401783937859, -9.519507165005897775, 9.576690525650159103 ) ) ;
#32642=VECTOR ( 'NONE', #52844, 1000.000000000000000 ) ;
#32643=ORIENTED_EDGE ( 'NONE', *, *, #40381, .T. ) ;
#32648=CARTESIAN_POINT ( 'NONE',  ( -3.740102306720532788, 25.00000000000000000, -6.044082642436763742 ) ) ;
#32649=VERTEX_POINT ( 'NONE', #65121 ) ;
#32650=DIRECTION ( 'NONE',  ( 1.000000000000000000, -0.000000000000000000, 0.000000000000000000 ) ) ;
#32651=ORIENTED_EDGE ( 'NONE', *, *, #49546, .F. ) ;
#32652=CIRCLE ( 'NONE', #880, 5.000000000000000000 ) ;
#32655=CIRCLE ( 'NONE', #6170, 5.000000000000000000 ) ;
#32657=CYLINDRICAL_SURFACE ( 'NONE', #1575, 12.75000000000000178 ) ;
#32658=FACE_OUTER_BOUND ( 'NONE', #55691, .T. ) ;
#32659=FACE_OUTER_BOUND ( 'NONE', #7392, .T. ) ;
#32660=DIRECTION ( 'NONE',  ( 0.000000000000000000, 0.2960891610144510966, 0.9551603052523479631 ) ) ;
#32661=VERTEX_POINT ( 'NONE', #49841 ) ;
#32662=CARTESIAN_POINT ( 'NONE',  ( 37.00000000000000711, -11.32068061209299259, -5.865551165831043079 ) ) ;
#32665=DIRECTION ( 'NONE',  ( -1.000000000000000000, -0.000000000000000000, -0.000000000000000000 ) ) ;
#32666=EDGE_LOOP ( 'NONE', ( #48783, #54561, #63204, #3787 ) ) ;
#32668=ORIENTED_EDGE ( 'NONE', *, *, #6962, .T. ) ;
#32670=ORIENTED_EDGE ( 'NONE', *, *, #25219, .F. ) ;
#32673=CARTESIAN_POINT ( 'NONE',  ( -35.00000000000000000, -15.00000000000000000, 0.000000000000000000 ) ) ;
#32675=ADVANCED_FACE ( 'NONE', ( #38555 ), #44500, .T. ) ;
#32676=DIRECTION ( 'NONE',  ( -1.000000000000000000, -0.000000000000000000, 0.000000000000000000 ) ) ;
#32677=DIRECTION ( 'NONE',  ( 1.000000000000000000, 0.000000000000000000, 0.000000000000000000 ) ) ;
#32678=CARTESIAN_POINT ( 'NONE',  ( 13.33580375564548781, 12.01919014649627293, -6.162572361761344375 ) ) ;
#32680=ORIENTED_EDGE ( 'NONE', *, *, #10421, .F. ) ;
#32684=EDGE_LOOP ( 'NONE', ( #62964, #48399, #64178, #47924 ) ) ;
#32685=EDGE_CURVE ( 'NONE', #50474, #12842, #31658, .T. ) ;
#32686=CARTESIAN_POINT ( 'NONE',  ( 47.00000000000000711, 4.705694406421931860E-17, -3.469127814946512892E-15 ) ) ;
#32690=CYLINDRICAL_SURFACE ( 'NONE', #52260, 12.75000000000000178 ) ;
#32691=CARTESIAN_POINT ( 'NONE',  ( 37.00000000000000711, 12.09831040184923978, -1.463443770872822736 ) ) ;
#32692=AXIS2_PLACEMENT_3D ( 'NONE', #5317, #19303, #25591 ) ;
#32693=DIRECTION ( 'NONE',  ( -1.000000000000000000, -0.000000000000000000, 0.000000000000000000 ) ) ;
#32694=DIRECTION ( 'NONE',  ( 1.000000000000000000, 0.000000000000000000, 0.000000000000000000 ) ) ;
#32695=VECTOR ( 'NONE', #41676, 1000.000000000000000 ) ;
#32696=ORIENTED_EDGE ( 'NONE', *, *, #26179, .T. ) ;
#32697=CARTESIAN_POINT ( 'NONE',  ( 35.00000000000000000, -11.47758908105696207, -2.497432891016804657 ) ) ;
#32698=AXIS2_PLACEMENT_3D ( 'NONE', #31408, #52685, #7112 ) ;
#32700=ADVANCED_FACE ( 'NONE', ( #39525 ), #44194, .T. ) ;
#32701=VECTOR ( 'NONE', #39997, 1000.000000000000000 ) ;
#32702=EDGE_CURVE ( 'NONE', #39567, #55842, #50808, .T. ) ;
#32703=DIRECTION ( 'NONE',  ( 0.000000000000000000, -0.01356324068817999114, 0.9999080150203989437 ) ) ;
#32704=LINE ( 'NONE', #58020, #18478 ) ;
#32706=CARTESIAN_POINT ( 'NONE',  ( -37.00000000000000711, 12.74068829017554094, 0.4871980014161925165 ) ) ;
#32709=VERTEX_POINT ( 'NONE', #34537 ) ;
#32711=DIRECTION ( 'NONE',  ( -1.000000000000000000, -1.836970198721029688E-16, -0.000000000000000000 ) ) ;
#32714=AXIS2_PLACEMENT_3D ( 'NONE', #26502, #5931, #11533 ) ;
#32716=DIRECTION ( 'NONE',  ( 0.000000000000000000, -0.01356324068817998940, 0.9999080150203990547 ) ) ;
#32717=CARTESIAN_POINT ( 'NONE',  ( -26.63135098142518942, -12.18341857921932458, 5.815336232052954912 ) ) ;
#32719=CIRCLE ( 'NONE', #28471, 4.999999999999999112 ) ;
#32720=CARTESIAN_POINT ( 'NONE',  ( 19.08051869631892572, -3.535630671987933127, 11.50449325566757075 ) ) ;
#32722=DIRECTION ( 'NONE',  ( 0.000000000000000000, 0.9903235168508544017, 0.1387779952735853917 ) ) ;
#32725=ADVANCED_FACE ( 'NONE', ( #19903 ), #14882, .T. ) ;
#32727=DIRECTION ( 'NONE',  ( 1.000000000000000000, 0.000000000000000000, 0.000000000000000000 ) ) ;
#32729=VERTEX_POINT ( 'NONE', #5618 ) ;
#32730=DIRECTION ( 'NONE',  ( -1.000000000000000000, -0.000000000000000000, 0.000000000000000000 ) ) ;
#32731=AXIS2_PLACEMENT_3D ( 'NONE', #22588, #42852, #10970 ) ;
#32733=DIRECTION ( 'NONE',  ( -1.000000000000000000, 0.000000000000000000, 0.000000000000000000 ) ) ;
#32734=ORIENTED_EDGE ( 'NONE', *, *, #49756, .T. ) ;
#32735=DIRECTION ( 'NONE',  ( 0.000000000000000000, 0.01356324068817298112, -0.9999080150203990547 ) ) ;
#32736=FACE_OUTER_BOUND ( 'NONE', #950, .T. ) ;
#32738=AXIS2_PLACEMENT_3D ( 'NONE', #38333, #28052, #29032 ) ;
#32739=CARTESIAN_POINT ( 'NONE',  ( -10.48620311856347875, -9.720786832536937538, 25.00000000000000000 ) ) ;
#32740=DIRECTION ( 'NONE',  ( 0.000000000000000000, -0.01356324068817992175, 0.9999080150203990547 ) ) ;
#32741=FACE_OUTER_BOUND ( 'NONE', #36184, .T. ) ;
#32744=VECTOR ( 'NONE', #27988, 1000.000000000000000 ) ;
#32745=DIRECTION ( 'NONE',  ( -1.000000000000000000, 0.000000000000000000, -0.000000000000000000 ) ) ;
#32747=CARTESIAN_POINT ( 'NONE',  ( -2.532614230583026593, -5.020478806276874373, 10.89930238848911337 ) ) ;
#32749=AXIS2_PLACEMENT_3D ( 'NONE', #44397, #58766, #8509 ) ;
#32750=VERTEX_POINT ( 'NONE', #4638 ) ;
#32751=SHAPE_DEFINITION_REPRESENTATION ( #22274, #45039 ) ;
#32756=CARTESIAN_POINT ( 'NONE',  ( 35.00000000000000000, -4.426194442447322075, -11.35427606708804937 ) ) ;
#32757=ORIENTED_EDGE ( 'NONE', *, *, #24265, .F. ) ;
#32762=EDGE_LOOP ( 'NONE', ( #58305, #18246, #2635, #50442 ) ) ;
#32764=DIRECTION ( 'NONE',  ( 1.000000000000000000, 0.000000000000000000, 0.000000000000000000 ) ) ;
#32765=ORIENTED_EDGE ( 'NONE', *, *, #9834, .F. ) ;
#32766=CARTESIAN_POINT ( 'NONE',  ( -37.00000000000000711, -1.463443770872689953, -12.09831040184925754 ) ) ;
#32768=CARTESIAN_POINT ( 'NONE',  ( 35.00000000000000000, -0.4353888892049205261, -11.73808581813437968 ) ) ;
#32769=CARTESIAN_POINT ( 'NONE',  ( 17.27839441901508621, -12.20388373500082224, 5.771933972472480967 ) ) ;
#32771=DIRECTION ( 'NONE',  ( 1.000000000000000000, 0.000000000000000000, 0.000000000000000000 ) ) ;
#32772=AXIS2_PLACEMENT_3D ( 'NONE', #57614, #36969, #22015 ) ;
#32775=CYLINDRICAL_SURFACE ( 'NONE', #13580, 12.75000000000000178 ) ;
#32776=VECTOR ( 'NONE', #5844, 1000.000000000000000 ) ;
#32780=CARTESIAN_POINT ( 'NONE',  ( -7.181456785175555524, -8.540743096806455270, -10.45493698471458188 ) ) ;
#32781=ADVANCED_FACE ( 'NONE', ( #61432 ), #45175, .T. ) ;
#32784=CIRCLE ( 'NONE', #50909, 5.000000000000000000 ) ;
#32785=EDGE_CURVE ( 'NONE', #19909, #24505, #20880, .T. ) ;
#32786=VECTOR ( 'NONE', #13057, 1000.000000000000000 ) ;
#32787=ORIENTED_EDGE ( 'NONE', *, *, #12029, .T. ) ;
#32789=CYLINDRICAL_SURFACE ( 'NONE', #8926, 5.000000000000002665 ) ;
#32790=( BOUNDED_CURVE ( )  B_SPLINE_CURVE ( 3, ( #46507, #31534, #61796, #36854 ),
 .UNSPECIFIED., .F., .F. ) 
 B_SPLINE_CURVE_WITH_KNOTS ( ( 4, 4 ),
 ( 5.423376644452276629, 5.470465898410777683 ),
 .UNSPECIFIED. ) 
 CURVE ( )  GEOMETRIC_REPRESENTATION_ITEM ( )  RATIONAL_B_SPLINE_CURVE ( ( 1.000000000000000000, 0.9998152253828482827, 0.9998152253828482827, 1.000000000000000000 ) ) 
 REPRESENTATION_ITEM ( '' )  );
#32791=ORIENTED_EDGE ( 'NONE', *, *, #47064, .F. ) ;
#32793=CARTESIAN_POINT ( 'NONE',  ( -37.00000000000000711, 7.718225330433808651, 9.430788938294078605 ) ) ;
#32797=VERTEX_POINT ( 'NONE', #4951 ) ;
#32804=LINE ( 'NONE', #53113, #24579 ) ;
#32805=CYLINDRICAL_SURFACE ( 'NONE', #24473, 12.75000000000000178 ) ;
#32808=CARTESIAN_POINT ( 'NONE',  ( 35.00000000000000000, 5.391785509271111110, 10.43555801961468887 ) ) ;
#32810=ORIENTED_EDGE ( 'NONE', *, *, #4708, .T. ) ;
#32811=CARTESIAN_POINT ( 'NONE',  ( -18.08686583997219799, 4.944984469693710416, -12.56371394453824841 ) ) ;
#32812=DIRECTION ( 'NONE',  ( 0.000000000000000000, 0.000000000000000000, -1.000000000000000000 ) ) ;
#32814=CARTESIAN_POINT ( 'NONE',  ( -14.11589373245165469, 8.250315036047107142, 25.00000000000000000 ) ) ;
#32817=AXIS2_PLACEMENT_3D ( 'NONE', #39071, #49422, #43740 ) ;
#32818=ORIENTED_EDGE ( 'NONE', *, *, #23845, .T. ) ;
#32819=EDGE_LOOP ( 'NONE', ( #60106, #12645, #43236, #51614 ) ) ;
#32822=CARTESIAN_POINT ( 'NONE',  ( 37.00000000000000711, 1.262958560998929558, 12.12087942037208066 ) ) ;
#32823=DIRECTION ( 'NONE',  ( 1.000000000000000000, -0.000000000000000000, 0.000000000000000000 ) ) ;
#32826=AXIS2_PLACEMENT_3D ( 'NONE', #22596, #33860, #18612 ) ;
#32827=FACE_OUTER_BOUND ( 'NONE', #53434, .T. ) ;
#32829=CARTESIAN_POINT ( 'NONE',  ( -37.00000000000000711, 5.015831474386455824, -10.62137734850263016 ) ) ;
#32830=VERTEX_POINT ( 'NONE', #26208 ) ;
#32832=DIRECTION ( 'NONE',  ( 0.000000000000000000, 0.8169148498130297531, -0.5767582926624941209 ) ) ;
#32833=VERTEX_POINT ( 'NONE', #47478 ) ;
#32834=DIRECTION ( 'NONE',  ( 0.000000000000000000, -0.1387779952735885280, 0.9903235168508540687 ) ) ;
#32835=CIRCLE ( 'NONE', #16911, 4.999999999999998224 ) ;
#32836=FACE_OUTER_BOUND ( 'NONE', #41593, .T. ) ;
#32839=ORIENTED_EDGE ( 'NONE', *, *, #4596, .T. ) ;
#32840=DIRECTION ( 'NONE',  ( 0.000000000000000000, 0.01356324068817998940, -0.9999080150203990547 ) ) ;
#32841=ADVANCED_FACE ( 'NONE', ( #46807 ), #1916, .T. ) ;
#32843=DIRECTION ( 'NONE',  ( 1.000000000000000000, 0.000000000000000000, 0.000000000000000000 ) ) ;
#32844=EDGE_LOOP ( 'NONE', ( #24754, #8484, #23183, #49584 ) ) ;
#32847=EDGE_CURVE ( 'NONE', #19477, #9113, #17867, .T. ) ;
#32849=EDGE_LOOP ( 'NONE', ( #41364, #37582, #48367, #20919 ) ) ;
#32851=ORIENTED_EDGE ( 'NONE', *, *, #23742, .T. ) ;
#32853=EDGE_LOOP ( 'NONE', ( #56156, #10422, #11156, #5833 ) ) ;
#32856=CARTESIAN_POINT ( 'NONE',  ( -21.17861794710831091, -11.44571409049744481, -3.604945070120774808 ) ) ;
#32858=EDGE_CURVE ( 'NONE', #62960, #14197, #62111, .T. ) ;
#32862=DIRECTION ( 'NONE',  ( 0.000000000000000000, -0.01356324068817992175, 0.9999080150203990547 ) ) ;
#32866=EDGE_CURVE ( 'NONE', #53501, #7090, #42445, .T. ) ;
#32867=DIRECTION ( 'NONE',  ( -1.000000000000000000, -0.000000000000000000, 0.000000000000000000 ) ) ;
#32868=CYLINDRICAL_SURFACE ( 'NONE', #65722, 12.74999999999999822 ) ;
#32869=DIRECTION ( 'NONE',  ( 1.000000000000000000, 0.000000000000000000, 0.000000000000000000 ) ) ;
#32871=CARTESIAN_POINT ( 'NONE',  ( -4.979813338170842485, -1.249770091004171357, 11.93591655830499931 ) ) ;
#32872=AXIS2_PLACEMENT_3D ( 'NONE', #60793, #61118, #55474 ) ;
#32873=AXIS2_PLACEMENT_3D ( 'NONE', #7626, #48219, #26927 ) ;
#32877=ORIENTED_EDGE ( 'NONE', *, *, #45180, .F. ) ;
#32878=CARTESIAN_POINT ( 'NONE',  ( -11.19266278829386252, -9.205500726053108096, 7.720277079051165892 ) ) ;
#32880=CARTESIAN_POINT ( 'NONE',  ( -36.00000000000000711, 11.66664283989680051, 5.143145423404322791 ) ) ;
#32882=CARTESIAN_POINT ( 'NONE',  ( -35.00000000000000000, 0.000000000000000000, 0.000000000000000000 ) ) ;
#32883=EDGE_LOOP ( 'NONE', ( #63425, #34526, #46938, #49327 ) ) ;
#32884=CARTESIAN_POINT ( 'NONE',  ( 35.00000000000000000, 12.09831040184923978, -1.463443770872822736 ) ) ;
#32885=CARTESIAN_POINT ( 'NONE',  ( 35.00000000000000000, -8.839356091080105671, -8.389074212634254124 ) ) ;
#32886=CARTESIAN_POINT ( 'NONE',  ( 37.00000000000000711, -11.39945968423467448, 5.710938531231826154 ) ) ;
#32888=CIRCLE ( 'NONE', #11640, 12.18650000000000233 ) ;
#32890=CARTESIAN_POINT ( 'NONE',  ( -4.975205859172449507, -1.416020129149132778, -13.42553116244733680 ) ) ;
#32896=CIRCLE ( 'NONE', #29717, 5.000000000000000888 ) ;
#32897=ADVANCED_FACE ( 'NONE', ( #53110 ), #7547, .T. ) ;
#32898=ORIENTED_EDGE ( 'NONE', *, *, #62336, .T. ) ;
#32899=CARTESIAN_POINT ( 'NONE',  ( -8.907762356386051295, 9.802223273060290509, -9.289308028724567734 ) ) ;
#32900=ORIENTED_EDGE ( 'NONE', *, *, #35659, .T. ) ;
#32902=CARTESIAN_POINT ( 'NONE',  ( 36.00000000000000711, 8.496612874013157679, -9.506317355798405089 ) ) ;
#32906=ORIENTED_EDGE ( 'NONE', *, *, #8083, .T. ) ;
#32907=VERTEX_POINT ( 'NONE', #63394 ) ;
#32908=ORIENTED_EDGE ( 'NONE', *, *, #59076, .F. ) ;
#32909=DIRECTION ( 'NONE',  ( 1.000000000000000000, 0.000000000000000000, -0.000000000000000000 ) ) ;
#32912=ADVANCED_FACE ( 'NONE', ( #38127 ), #41821, .T. ) ;
#32913=AXIS2_PLACEMENT_3D ( 'NONE', #56101, #5598, #912 ) ;
#32914=ORIENTED_EDGE ( 'NONE', *, *, #60369, .T. ) ;
#32917=ORIENTED_EDGE ( 'NONE', *, *, #615, .F. ) ;
#32918=CARTESIAN_POINT ( 'NONE',  ( -35.00000000000000000, 11.81949347079751256, -2.968224442958276921 ) ) ;
#32921=B_SPLINE_CURVE_WITH_KNOTS ( 'NONE', 3,
 ( #47815, #36530, #52804, #17234, #42146, #32175, #58128, #57813, #2274, #32498, #42467, #62433, #31529, #62128, #11575, #31846, #27518, #52160, #26880, #16895 ),
 .UNSPECIFIED., .F., .F.,
 ( 4, 2, 2, 2, 2, 2, 2, 2, 2, 4 ),
 ( 2.874676074482899647E-18, 0.001273611734732489056, 0.002547223469464975510, 0.003820835204197461313, 0.005094446938929947551, 0.006368058673662434221, 0.007004864541028676256, 0.007641670408394919158, 0.008915282143127404094, 0.01018889387785988643 ),
 .UNSPECIFIED. ) ;
#32923=CARTESIAN_POINT ( 'NONE',  ( -35.00000000000000000, 8.954052073409602741, 9.076753354954030684 ) ) ;
#32924=ORIENTED_EDGE ( 'NONE', *, *, #61286, .T. ) ;
#32928=ORIENTED_EDGE ( 'NONE', *, *, #10300, .F. ) ;
#32929=CARTESIAN_POINT ( 'NONE',  ( 11.13055501096828692, 0.3454441929252254906, -13.49618539646086113 ) ) ;
#32930=VERTEX_POINT ( 'NONE', #23175 ) ;
#32932=CIRCLE ( 'NONE', #62638, 5.000000000000000888 ) ;
#32934=CARTESIAN_POINT ( 'NONE',  ( 35.00000000000000000, 4.074242145636174151, 12.08151691381185167 ) ) ;
#32936=DIRECTION ( 'NONE',  ( -1.000000000000000000, -0.000000000000000000, 0.000000000000000000 ) ) ;
#32937=EDGE_CURVE ( 'NONE', #2547, #40853, #38468, .T. ) ;
#32938=CARTESIAN_POINT ( 'NONE',  ( -35.00000000000000000, -0.7008968033237865658, -12.16632754454237819 ) ) ;
#32939=DIRECTION ( 'NONE',  ( 1.000000000000000000, 0.000000000000000000, 0.000000000000000000 ) ) ;
#32940=ORIENTED_EDGE ( 'NONE', *, *, #61102, .F. ) ;
#32941=CIRCLE ( 'NONE', #43528, 12.18649999999999878 ) ;
#32943=ORIENTED_EDGE ( 'NONE', *, *, #22188, .F. ) ;
#32945=EDGE_CURVE ( 'NONE', #23983, #2293, #43441, .T. ) ;
#32947=VERTEX_POINT ( 'NONE', #9751 ) ;
#32948=CARTESIAN_POINT ( 'NONE',  ( 25.05309951391468459, 10.77522019223767558, -8.132934882857098202 ) ) ;
#32954=DIRECTION ( 'NONE',  ( 1.000000000000000000, 0.000000000000000000, 0.000000000000000000 ) ) ;
#32956=AXIS2_PLACEMENT_3D ( 'NONE', #53665, #28372, #48670 ) ;
#32957=ORIENTED_EDGE ( 'NONE', *, *, #54324, .F. ) ;
#32959=DIRECTION ( 'NONE',  ( 0.000000000000000000, -0.5472293298355157543, 0.8369827122275419473 ) ) ;
#32960=DIRECTION ( 'NONE',  ( -1.000000000000000000, -0.000000000000000000, 0.000000000000000000 ) ) ;
#32962=VERTEX_POINT ( 'NONE', #38801 ) ;
#32963=DIRECTION ( 'NONE',  ( 0.000000000000000000, -0.01356324068817992175, 0.9999080150203990547 ) ) ;
#32967=CARTESIAN_POINT ( 'NONE',  ( 35.00000000000000000, -9.390600770288049404, -8.624332853796024878 ) ) ;
#32968=CARTESIAN_POINT ( 'NONE',  ( -35.00000000000000000, -11.61175578952785159, -1.771820996347277966 ) ) ;
#32970=DIRECTION ( 'NONE',  ( 0.000000000000000000, -1.000000000000000000, 0.000000000000000000 ) ) ;
#32972=FACE_OUTER_BOUND ( 'NONE', #32578, .T. ) ;
#32974=VECTOR ( 'NONE', #15433, 1000.000000000000000 ) ;
#32975=EDGE_CURVE ( 'NONE', #45713, #64338, #63553, .T. ) ;
#32976=AXIS2_PLACEMENT_3D ( 'NONE', #14952, #55208, #48934 ) ;
#32978=CARTESIAN_POINT ( 'NONE',  ( -37.00000000000000711, -4.237174932027140350, -12.02534193257725725 ) ) ;
#32979=AXIS2_PLACEMENT_3D ( 'NONE', #49112, #58423, #7200 ) ;
#32980=CIRCLE ( 'NONE', #50002, 12.18650000000000055 ) ;
#32982=ORIENTED_EDGE ( 'NONE', *, *, #5687, .T. ) ;
#32986=ORIENTED_EDGE ( 'NONE', *, *, #32945, .F. ) ;
#32988=CYLINDRICAL_SURFACE ( 'NONE', #2335, 12.74999999999999822 ) ;
#32990=CIRCLE ( 'NONE', #6486, 4.999999999999998224 ) ;
#32992=ORIENTED_EDGE ( 'NONE', *, *, #38692, .F. ) ;
#32993=VERTEX_POINT ( 'NONE', #43786 ) ;
#32994=CARTESIAN_POINT ( 'NONE',  ( 29.60171417218365519, -10.89687559552093532, 7.981938771698986912 ) ) ;
#32996=EDGE_CURVE ( 'NONE', #15001, #1502, #59099, .T. ) ;
#32997=VERTEX_POINT ( 'NONE', #35346 ) ;
#32998=LINE ( 'NONE', #33349, #27092 ) ;
#32999=CYLINDRICAL_SURFACE ( 'NONE', #36768, 14.99999999999998757 ) ;
#33001=AXIS2_PLACEMENT_3D ( 'NONE', #34260, #4015, #13970 ) ;
#33002=CYLINDRICAL_SURFACE ( 'NONE', #18458, 12.74999999999999822 ) ;
#33004=FACE_OUTER_BOUND ( 'NONE', #41258, .T. ) ;
#33005=EDGE_CURVE ( 'NONE', #51673, #18713, #20053, .T. ) ;
#33007=DIRECTION ( 'NONE',  ( 1.000000000000000000, 0.000000000000000000, 0.000000000000000000 ) ) ;
#33008=CARTESIAN_POINT ( 'NONE',  ( -37.00000000000000711, 9.348667969174405457, 7.817492529713891081 ) ) ;
#33009=ORIENTED_EDGE ( 'NONE', *, *, #48177, .T. ) ;
#33010=CARTESIAN_POINT ( 'NONE',  ( -2.952869152607111136, 25.00000000000000000, 11.17020052527586138 ) ) ;
#33011=CIRCLE ( 'NONE', #46839, 12.75000000000000178 ) ;
#33012=ADVANCED_FACE ( 'NONE', ( #45014 ), #65288, .T. ) ;
#33015=VERTEX_POINT ( 'NONE', #57287 ) ;
#33016=CARTESIAN_POINT ( 'NONE',  ( 35.00000000000000000, -10.93004082984022851, -6.564808257521735690 ) ) ;
#33017=CARTESIAN_POINT ( 'NONE',  ( 35.00000000000000000, 11.59095880812004964, -1.903127969211395598 ) ) ;
#33018=CYLINDRICAL_SURFACE ( 'NONE', #22325, 5.000000000000000888 ) ;
#33020=AXIS2_PLACEMENT_3D ( 'NONE', #39363, #33407, #63640 ) ;
#33024=DIRECTION ( 'NONE',  ( 1.000000000000000000, 0.000000000000000000, 0.000000000000000000 ) ) ;
#33025=ORIENTED_EDGE ( 'NONE', *, *, #27685, .F. ) ;
#33026=VECTOR ( 'NONE', #61732, 1000.000000000000000 ) ;
#33027=DIRECTION ( 'NONE',  ( -1.000000000000000000, -0.000000000000000000, -0.000000000000000000 ) ) ;
#33029=EDGE_CURVE ( 'NONE', #31267, #56700, #23234, .T. ) ;
#33030=EDGE_CURVE ( 'NONE', #55094, #57486, #6752, .T. ) ;
#33032=CARTESIAN_POINT ( 'NONE',  ( -36.00000000000000711, -12.70128625845193859, 1.113475361586445000 ) ) ;
#33033=FACE_OUTER_BOUND ( 'NONE', #52791, .T. ) ;
#33034=DIRECTION ( 'NONE',  ( 1.000000000000000000, 0.000000000000000000, -0.000000000000000000 ) ) ;
#33036=EDGE_CURVE ( 'NONE', #57471, #39575, #10401, .T. ) ;
#33037=LINE ( 'NONE', #64595, #58227 ) ;
#33038=CIRCLE ( 'NONE', #21367, 5.000000000000000000 ) ;
#33039=AXIS2_PLACEMENT_3D ( 'NONE', #54614, #23026, #9034 ) ;
#33040=DIRECTION ( 'NONE',  ( -1.000000000000000000, 0.000000000000000000, 0.000000000000000000 ) ) ;
#33041=CARTESIAN_POINT ( 'NONE',  ( 145.1370849898475797, 3.309064568108273190E-14, 0.000000000000000000 ) ) ;
#33043=EDGE_CURVE ( 'NONE', #63537, #11428, #41302, .T. ) ;
#33044=ORIENTED_EDGE ( 'NONE', *, *, #21483, .F. ) ;
#33048=CARTESIAN_POINT ( 'NONE',  ( -17.78890373828789606, -5.238151136051769186, 12.44321837383489893 ) ) ;
#33049=CIRCLE ( 'NONE', #119, 5.000000000000000888 ) ;
#33053=FACE_OUTER_BOUND ( 'NONE', #25478, .T. ) ;
#33055=VECTOR ( 'NONE', #57642, 1000.000000000000000 ) ;
#33057=CARTESIAN_POINT ( 'NONE',  ( 47.00000000000000711, 4.705694406421931860E-17, -3.469127814946512892E-15 ) ) ;
#33061=B_SPLINE_CURVE_WITH_KNOTS ( 'NONE', 3,
 ( #44259, #38955, #13667, #33310, #33951, #23999, #39268, #13998, #64532, #59564 ),
 .UNSPECIFIED., .F., .F.,
 ( 4, 2, 2, 2, 4 ),
 ( 8.673617379884035472E-19, 0.002710955585989774201, 0.003388694482487217101, 0.004066433378984660868, 0.005421911171979544933 ),
 .UNSPECIFIED. ) ;
#33063=AXIS2_PLACEMENT_3D ( 'NONE', #53018, #2505, #48388 ) ;
#33066=CARTESIAN_POINT ( 'NONE',  ( -26.47815227414952233, -12.15021249753662325, 5.884769607083862653 ) ) ;
#33067=VERTEX_POINT ( 'NONE', #15710 ) ;
#33068=CARTESIAN_POINT ( 'NONE',  ( -35.00000000000000000, -7.238157050195700215, 10.49626516989268588 ) ) ;
#33078=DIRECTION ( 'NONE',  ( -1.000000000000000000, 0.000000000000000000, -0.000000000000000000 ) ) ;
#33083=AXIS2_PLACEMENT_3D ( 'NONE', #24465, #9486, #44745 ) ;
#33086=CARTESIAN_POINT ( 'NONE',  ( 37.00000000000000711, 4.705694406421931860E-17, -3.469127814946512892E-15 ) ) ;
#33088=CARTESIAN_POINT ( 'NONE',  ( -27.70115331877724785, 11.17762196442450850, -4.375698238583000332 ) ) ;
#33091=DIRECTION ( 'NONE',  ( -1.000000000000000000, -0.000000000000000000, 0.000000000000000000 ) ) ;
#33092=ORIENTED_EDGE ( 'NONE', *, *, #8229, .T. ) ;
#33093=CARTESIAN_POINT ( 'NONE',  ( -35.00000000000000000, 0.000000000000000000, 0.000000000000000000 ) ) ;
#33094=EDGE_CURVE ( 'NONE', #39393, #16656, #57093, .T. ) ;
#33095=ORIENTED_EDGE ( 'NONE', *, *, #46672, .F. ) ;
#33097=AXIS2_PLACEMENT_3D ( 'NONE', #50724, #21100, #15461 ) ;
#33099=VERTEX_POINT ( 'NONE', #26359 ) ;
#33100=CARTESIAN_POINT ( 'NONE',  ( -24.96502833112928244, 11.16032118974457887, 7.597682957678232540 ) ) ;
#33104=CARTESIAN_POINT ( 'NONE',  ( 35.00000000000000000, -3.827046518385000429, 11.56998259273181162 ) ) ;
#33105=ORIENTED_EDGE ( 'NONE', *, *, #669, .T. ) ;
#33106=VECTOR ( 'NONE', #21519, 1000.000000000000000 ) ;
#33107=CARTESIAN_POINT ( 'NONE',  ( -27.19357181888462094, -10.84410562793472543, 5.138615876886901468 ) ) ;
#33110=ORIENTED_EDGE ( 'NONE', *, *, #11209, .T. ) ;
#33112=CARTESIAN_POINT ( 'NONE',  ( -37.00000000000000711, -11.16627499335652374, -3.645068577060142978 ) ) ;
#33115=CARTESIAN_POINT ( 'NONE',  ( -36.00000000000000711, 12.42372387097882580, 2.865935305911670561 ) ) ;
#33116=CARTESIAN_POINT ( 'NONE',  ( -35.00000000000000000, 9.076753354954126607, -8.954052073409506818 ) ) ;
#33117=ADVANCED_FACE ( 'NONE', ( #56967 ), #11390, .T. ) ;
#33119=VECTOR ( 'NONE', #61698, 1000.000000000000000 ) ;
#33120=AXIS2_PLACEMENT_3D ( 'NONE', #7613, #48205, #2657 ) ;
#33123=AXIS2_PLACEMENT_3D ( 'NONE', #45341, #65602, #20074 ) ;
#33124=EDGE_CURVE ( 'NONE', #63543, #25796, #21723, .T. ) ;
#33125=CARTESIAN_POINT ( 'NONE',  ( -7.181456785175555524, -8.540743096806455270, -10.45493698471458188 ) ) ;
#33126=ORIENTED_EDGE ( 'NONE', *, *, #9794, .T. ) ;
#33128=ORIENTED_EDGE ( 'NONE', *, *, #60637, .T. ) ;
#33129=EDGE_CURVE ( 'NONE', #61044, #32174, #57221, .T. ) ;
#33130=CYLINDRICAL_SURFACE ( 'NONE', #23285, 12.18650000000000055 ) ;
#33131=CARTESIAN_POINT ( 'NONE',  ( 35.00000000000000000, -10.01317267707881165, 6.946017217730044990 ) ) ;
#33133=VECTOR ( 'NONE', #44006, 1000.000000000000000 ) ;
#33135=ORIENTED_EDGE ( 'NONE', *, *, #2353, .T. ) ;
#33137=ORIENTED_EDGE ( 'NONE', *, *, #18551, .F. ) ;
#33138=DIRECTION ( 'NONE',  ( 0.000000000000000000, 0.01356324068817992175, -0.9999080150203990547 ) ) ;
#33139=CARTESIAN_POINT ( 'NONE',  ( 9.388378107225753055, 7.267209807330653248, 9.555403925956888145 ) ) ;
#33144=CARTESIAN_POINT ( 'NONE',  ( 18.90132044483814155, 7.635003998667697189, 11.15574165374908056 ) ) ;
#33147=EDGE_CURVE ( 'NONE', #46634, #44827, #12047, .T. ) ;
#33150=DIRECTION ( 'NONE',  ( 0.000000000000000000, -0.01356324068817998940, 0.9999080150203990547 ) ) ;
#33151=ORIENTED_EDGE ( 'NONE', *, *, #3241, .F. ) ;
#33155=VERTEX_POINT ( 'NONE', #42279 ) ;
#33156=CARTESIAN_POINT ( 'NONE',  ( -11.38914276748393739, -7.969851211656610701, -8.976043701440310940 ) ) ;
#33158=CARTESIAN_POINT ( 'NONE',  ( -35.00000000000000000, -1.903127969211109383, -11.59095880812010471 ) ) ;
#33159=B_SPLINE_CURVE_WITH_KNOTS ( 'NONE', 3,
 ( #58886, #36680, #1112, #32899, #31367, #22628, #51672, #8309, #7309, #6113, #58542, #12967, #26372, #23614, #41665, #37906, #13300, #33584 ),
 .UNSPECIFIED., .F., .F.,
 ( 4, 2, 2, 2, 2, 2, 2, 2, 4 ),
 ( 1.309687503460227108E-17, 0.002358234771816867213, 0.003537352157725295616, 0.004716469543633724885, 0.005895586929542152854, 0.007074704315450581690, 0.007664263008404797843, 0.008253821701359013996, 0.009432939087267441097 ),
 .UNSPECIFIED. ) ;
#33160=EDGE_CURVE ( 'NONE', #34567, #54444, #13361, .T. ) ;
#33161=AXIS2_PLACEMENT_3D ( 'NONE', #14193, #13851, #3917 ) ;
#33162=DIRECTION ( 'NONE',  ( 1.000000000000000000, 0.000000000000000000, 0.000000000000000000 ) ) ;
#33164=AXIS2_PLACEMENT_3D ( 'NONE', #23105, #63644, #59670 ) ;
#33168=CARTESIAN_POINT ( 'NONE',  ( 37.00000000000000711, 12.70128625845192794, -1.113475361586537593 ) ) ;
#33169=CYLINDRICAL_SURFACE ( 'NONE', #40681, 12.75000000000000178 ) ;
#33171=DIRECTION ( 'NONE',  ( 1.000000000000000000, 0.000000000000000000, -0.000000000000000000 ) ) ;
#33172=DIRECTION ( 'NONE',  ( 1.000000000000000000, 0.000000000000000000, -0.000000000000000000 ) ) ;
#33174=CARTESIAN_POINT ( 'NONE',  ( 47.00000000000000711, 4.705694406421931860E-17, -3.469127814946512892E-15 ) ) ;
#33176=ADVANCED_FACE ( 'NONE', ( #63901 ), #28332, .T. ) ;
#33177=EDGE_CURVE ( 'NONE', #63912, #30828, #65678, .T. ) ;
#33179=FACE_OUTER_BOUND ( 'NONE', #18586, .T. ) ;
#33183=CARTESIAN_POINT ( 'NONE',  ( -35.00000000000000000, -9.908974237959601084, -6.307491713049132365 ) ) ;
#33189=CIRCLE ( 'NONE', #47018, 5.000000000000000888 ) ;
#33193=VECTOR ( 'NONE', #65167, 1000.000000000000000 ) ;
#33194=ORIENTED_EDGE ( 'NONE', *, *, #10893, .T. ) ;
#33195=DIRECTION ( 'NONE',  ( 1.000000000000000000, 0.000000000000000000, 0.000000000000000000 ) ) ;
#33198=VERTEX_POINT ( 'NONE', #28016 ) ;
#33199=VERTEX_POINT ( 'NONE', #63242 ) ;
#33201=EDGE_CURVE ( 'NONE', #63114, #43224, #42964, .T. ) ;
#33202=DIRECTION ( 'NONE',  ( -1.000000000000000000, 0.000000000000000000, 0.000000000000000000 ) ) ;
#33203=CARTESIAN_POINT ( 'NONE',  ( 37.00000000000000711, 5.927257550915316919, -10.64792938439757641 ) ) ;
#33207=DIRECTION ( 'NONE',  ( 0.000000000000000000, -1.000000000000000000, 0.000000000000000000 ) ) ;
#33208=VECTOR ( 'NONE', #21861, 1000.000000000000000 ) ;
#33211=CARTESIAN_POINT ( 'NONE',  ( -2.532614230583026593, 5.020478806276888584, 10.89930238848911337 ) ) ;
#33215=VECTOR ( 'NONE', #3833, 1000.000000000000000 ) ;
#33217=LINE ( 'NONE', #2669, #52034 ) ;
#33219=DIRECTION ( 'NONE',  ( -1.000000000000000000, 0.000000000000000000, 0.000000000000000000 ) ) ;
#33222=CIRCLE ( 'NONE', #60853, 12.18650000000000233 ) ;
#33225=DIRECTION ( 'NONE',  ( 0.000000000000000000, 0.4380125133593973930, -0.8989688749565157844 ) ) ;
#33226=ORIENTED_EDGE ( 'NONE', *, *, #28406, .F. ) ;
#33227=CARTESIAN_POINT ( 'NONE',  ( 35.00000000000000000, 7.376655759824880754, -9.700295462048687867 ) ) ;
#33229=DIRECTION ( 'NONE',  ( 0.000000000000000000, 0.01356324068817998940, -0.9999080150203989437 ) ) ;
#33232=ORIENTED_EDGE ( 'NONE', *, *, #50486, .T. ) ;
#33233=CIRCLE ( 'NONE', #6712, 12.18650000000000055 ) ;
#33236=CARTESIAN_POINT ( 'NONE',  ( -18.23022800145057687, -13.26592958674785194, 2.588920604642957368 ) ) ;
#33239=EDGE_CURVE ( 'NONE', #12285, #31390, #35975, .T. ) ;
#33242=AXIS2_PLACEMENT_3D ( 'NONE', #51630, #46616, #60938 ) ;
#33248=EDGE_LOOP ( 'NONE', ( #8012, #42716, #11545, #35752 ) ) ;
#33249=CARTESIAN_POINT ( 'NONE',  ( 9.779306477119707353, 6.953054007709951634, -9.784907511924334500 ) ) ;
#33250=ORIENTED_EDGE ( 'NONE', *, *, #64253, .T. ) ;
#33255=CARTESIAN_POINT ( 'NONE',  ( -27.27855387000350262, 25.00000000000000000, 5.631341004100471892 ) ) ;
#33256=ORIENTED_EDGE ( 'NONE', *, *, #36005, .F. ) ;
#33257=EDGE_CURVE ( 'NONE', #6726, #19811, #38068, .T. ) ;
#33258=CIRCLE ( 'NONE', #24770, 12.18650000000000055 ) ;
#33260=ORIENTED_EDGE ( 'NONE', *, *, #16255, .T. ) ;
#33261=ORIENTED_EDGE ( 'NONE', *, *, #49184, .F. ) ;
#33264=AXIS2_PLACEMENT_3D ( 'NONE', #45018, #44664, #8792 ) ;
#33265=DIRECTION ( 'NONE',  ( -1.000000000000000000, 0.000000000000000000, 0.000000000000000000 ) ) ;
#33266=CIRCLE ( 'NONE', #38584, 12.18650000000000055 ) ;
#33267=ORIENTED_EDGE ( 'NONE', *, *, #49265, .F. ) ;
#33270=ORIENTED_EDGE ( 'NONE', *, *, #61213, .F. ) ;
#33273=DIRECTION ( 'NONE',  ( -1.000000000000000000, 0.000000000000000000, -0.000000000000000000 ) ) ;
#33274=ORIENTED_EDGE ( 'NONE', *, *, #56123, .F. ) ;
#33275=VECTOR ( 'NONE', #65277, 1000.000000000000000 ) ;
#33276=ORIENTED_EDGE ( 'NONE', *, *, #17950, .T. ) ;
#33277=DIRECTION ( 'NONE',  ( 0.000000000000000000, -0.3218879778915842427, 0.9467777615094616905 ) ) ;
#33278=ORIENTED_EDGE ( 'NONE', *, *, #21231, .T. ) ;
#33279=CARTESIAN_POINT ( 'NONE',  ( -20.79170840334646542, 11.34110549087207076, -3.921648409140116698 ) ) ;
#33283=CARTESIAN_POINT ( 'NONE',  ( -37.00000000000000711, -10.39746860227885428, -7.379373053628982326 ) ) ;
#33284=EDGE_CURVE ( 'NONE', #14592, #58711, #42331, .T. ) ;
#33285=AXIS2_PLACEMENT_3D ( 'NONE', #46425, #52416, #27129 ) ;
#33290=CARTESIAN_POINT ( 'NONE',  ( 5.014783254242184185, -9.842758936301256867, -6.866372042166331013 ) ) ;
#33292=CYLINDRICAL_SURFACE ( 'NONE', #41779, 12.18649999999999878 ) ;
#33296=CIRCLE ( 'NONE', #64094, 5.000000000000000888 ) ;
#33298=VERTEX_POINT ( 'NONE', #9668 ) ;
#33302=EDGE_LOOP ( 'NONE', ( #13376, #54876, #55551, #55670 ) ) ;
#33304=CIRCLE ( 'NONE', #10998, 5.000000000000000000 ) ;
#33305=ORIENTED_EDGE ( 'NONE', *, *, #61526, .F. ) ;
#33306=DIRECTION ( 'NONE',  ( 0.4826047536471247956, 0.8758382566188793739, -0.000000000000000000 ) ) ;
#33307=ORIENTED_EDGE ( 'NONE', *, *, #32590, .F. ) ;
#33309=CARTESIAN_POINT ( 'NONE',  ( -3.673220185152842099, -7.076978035560978597, 9.701075964846328503 ) ) ;
#33310=CARTESIAN_POINT ( 'NONE',  ( -29.90001358305153545, 1.049925265473337754, 13.46092060699443671 ) ) ;
#33312=DIRECTION ( 'NONE',  ( -1.000000000000000000, -0.000000000000000000, 0.000000000000000000 ) ) ;
#33313=ORIENTED_EDGE ( 'NONE', *, *, #33545, .T. ) ;
#33314=AXIS2_PLACEMENT_3D ( 'NONE', #54318, #12404, #53666 ) ;
#33318=AXIS2_PLACEMENT_3D ( 'NONE', #39781, #60070, #30132 ) ;
#33319=VECTOR ( 'NONE', #62176, 1000.000000000000000 ) ;
#33323=ADVANCED_FACE ( 'NONE', ( #34294 ), #54273, .T. ) ;
#33325=CARTESIAN_POINT ( 'NONE',  ( 7.137737543050354461, -4.955906025390103942, -10.93869909733096613 ) ) ;
#33327=AXIS2_PLACEMENT_3D ( 'NONE', #50427, #13509, #14166 ) ;
#33328=AXIS2_PLACEMENT_3D ( 'NONE', #27689, #58298, #32350 ) ;
#33330=EDGE_LOOP ( 'NONE', ( #17621, #1812, #44713, #46664 ) ) ;
#33331=CARTESIAN_POINT ( 'NONE',  ( 12.90521571632873865, -10.89702685051559072, -5.029477694709124869 ) ) ;
#33332=ORIENTED_EDGE ( 'NONE', *, *, #44705, .T. ) ;
#33333=CARTESIAN_POINT ( 'NONE',  ( 35.00000000000000000, 4.705694406421931860E-17, -3.469127814946512892E-15 ) ) ;
#33335=DIRECTION ( 'NONE',  ( 1.000000000000000000, -0.000000000000000000, 0.000000000000000000 ) ) ;
#33336=VECTOR ( 'NONE', #64041, 1000.000000000000000 ) ;
#33337=ORIENTED_EDGE ( 'NONE', *, *, #30056, .F. ) ;
#33339=ORIENTED_EDGE ( 'NONE', *, *, #42888, .T. ) ;
#33342=ORIENTED_EDGE ( 'NONE', *, *, #6773, .F. ) ;
#33344=CARTESIAN_POINT ( 'NONE',  ( -10.90165637462999726, -7.721945941999268648, -9.189455070444248364 ) ) ;
#33346=AXIS2_PLACEMENT_3D ( 'NONE', #16689, #1420, #36961 ) ;
#33348=EDGE_CURVE ( 'NONE', #1474, #58929, #50594, .T. ) ;
#33349=CARTESIAN_POINT ( 'NONE',  ( 35.00000000000000000, 5.246972444134017977, -10.99909370905159101 ) ) ;
#33350=CARTESIAN_POINT ( 'NONE',  ( 3.990895163589245787, 6.918992358595912329, 11.62617458216422861 ) ) ;
#33351=DIRECTION ( 'NONE',  ( -0.000000000000000000, -0.000000000000000000, -1.000000000000000000 ) ) ;
#33352=DIRECTION ( 'NONE',  ( -1.000000000000000000, -0.000000000000000000, 0.000000000000000000 ) ) ;
#33356=CARTESIAN_POINT ( 'NONE',  ( -35.00000000000000000, 2.905556151562625811, 11.38112321385051651 ) ) ;
#33357=CARTESIAN_POINT ( 'NONE',  ( -26.97113089360557225, 10.82592580676787186, 5.176981052598353727 ) ) ;
#33359=DIRECTION ( 'NONE',  ( 0.000000000000000000, -0.8169148498130339719, 0.5767582926624881257 ) ) ;
#33360=VERTEX_POINT ( 'NONE', #13680 ) ;
#33361=CIRCLE ( 'NONE', #30171, 5.000000000000000000 ) ;
#33362=CARTESIAN_POINT ( 'NONE',  ( -20.56770621847863723, 13.00092155042986519, -3.647989838260398798 ) ) ;
#33363=CIRCLE ( 'NONE', #28054, 5.000000000000000888 ) ;
#33366=DIRECTION ( 'NONE',  ( -1.000000000000000000, 0.000000000000000000, 0.000000000000000000 ) ) ;
#33367=FACE_OUTER_BOUND ( 'NONE', #24348, .T. ) ;
#33368=DIRECTION ( 'NONE',  ( 0.000000000000000000, 0.9796553971857749898, 0.2006870767258855104 ) ) ;
#33369=CARTESIAN_POINT ( 'NONE',  ( -5.792881964653834537, -1.480264921545251688, -13.41892255734878958 ) ) ;
#33371=ORIENTED_EDGE ( 'NONE', *, *, #65711, .F. ) ;
#33372=DIRECTION ( 'NONE',  ( 1.000000000000000000, 0.000000000000000000, 0.000000000000000000 ) ) ;
#33373=VERTEX_POINT ( 'NONE', #44271 ) ;
#33375=AXIS2_PLACEMENT_3D ( 'NONE', #11771, #7122, #6160 ) ;
#33380=CARTESIAN_POINT ( 'NONE',  ( 35.00000000000000000, -9.348667969174460524, -7.817492529713823579 ) ) ;
#33381=AXIS2_PLACEMENT_3D ( 'NONE', #17780, #42696, #37731 ) ;
#33384=CARTESIAN_POINT ( 'NONE',  ( 37.00000000000000711, 4.705694406421931860E-17, -3.469127814946512892E-15 ) ) ;
#33385=CARTESIAN_POINT ( 'NONE',  ( 35.00000000000000000, 5.556331110570566167, 11.47561260193570654 ) ) ;
#33386=EDGE_LOOP ( 'NONE', ( #11169, #65483, #45521, #56874 ) ) ;
#33389=CARTESIAN_POINT ( 'NONE',  ( -37.00000000000000711, 0.000000000000000000, 0.000000000000000000 ) ) ;
#33391=CARTESIAN_POINT ( 'NONE',  ( -35.00000000000000000, -9.821084925794513865, -7.215058775251364409 ) ) ;
#33392=CARTESIAN_POINT ( 'NONE',  ( 47.00000000000000711, 4.705694406421931860E-17, -3.469127814946512892E-15 ) ) ;
#33393=AXIS2_PLACEMENT_3D ( 'NONE', #4617, #54497, #29521 ) ;
#33396=CARTESIAN_POINT ( 'NONE',  ( -11.06236561744495717, -5.410674147974703807, 12.37007031003713742 ) ) ;
#33400=VERTEX_POINT ( 'NONE', #31915 ) ;
#33401=CARTESIAN_POINT ( 'NONE',  ( -47.00000000000000711, 0.000000000000000000, 0.000000000000000000 ) ) ;
#33402=AXIS2_PLACEMENT_3D ( 'NONE', #54705, #19110, #53718 ) ;
#33403=DIRECTION ( 'NONE',  ( 0.000000000000000000, -0.3807014730195286134, 0.9246979985058695339 ) ) ;
#33405=ADVANCED_FACE ( 'NONE', ( #25300 ), #25633, .T. ) ;
#33407=DIRECTION ( 'NONE',  ( -1.000000000000000000, 0.000000000000000000, 0.000000000000000000 ) ) ;
#33408=AXIS2_PLACEMENT_3D ( 'NONE', #60706, #16128, #31098 ) ;
#33409=ORIENTED_EDGE ( 'NONE', *, *, #43132, .F. ) ;
#33411=EDGE_CURVE ( 'NONE', #60515, #55740, #36597, .T. ) ;
#33416=LINE ( 'NONE', #53381, #30930 ) ;
#33417=VERTEX_POINT ( 'NONE', #35604 ) ;
#33418=ORIENTED_EDGE ( 'NONE', *, *, #40123, .T. ) ;
#33419=CYLINDRICAL_SURFACE ( 'NONE', #35247, 12.18650000000000055 ) ;
#33420=EDGE_CURVE ( 'NONE', #5624, #53395, #40596, .T. ) ;
#33422=CIRCLE ( 'NONE', #38740, 12.74999999999999822 ) ;
#33423=ORIENTED_EDGE ( 'NONE', *, *, #10118, .F. ) ;
#33426=DIRECTION ( 'NONE',  ( 0.000000000000000000, -0.01356324068817991828, 0.9999080150203990547 ) ) ;
#33429=DIRECTION ( 'NONE',  ( -1.000000000000000000, 0.000000000000000000, 0.000000000000000000 ) ) ;
#33430=EDGE_CURVE ( 'NONE', #1946, #54776, #14708, .T. ) ;
#33434=CARTESIAN_POINT ( 'NONE',  ( -47.00000000000000711, 0.000000000000000000, 0.000000000000000000 ) ) ;
#33435=VERTEX_POINT ( 'NONE', #45926 ) ;
#33436=CARTESIAN_POINT ( 'NONE',  ( 35.00000000000000000, -9.700295462048712736, -7.376655759824850556 ) ) ;
#33437=ORIENTED_EDGE ( 'NONE', *, *, #49628, .F. ) ;
#33440=CARTESIAN_POINT ( 'NONE',  ( -25.86628395826706850, 8.041618865309581921, 10.84354029019568522 ) ) ;
#33442=CARTESIAN_POINT ( 'NONE',  ( -25.73422511961580028, 12.22591596592855190, 5.729065348228939314 ) ) ;
#33443=CIRCLE ( 'NONE', #31350, 4.999999999999998224 ) ;
#33446=DIRECTION ( 'NONE',  ( -0.000000000000000000, -0.000000000000000000, -1.000000000000000000 ) ) ;
#33454=B_SPLINE_CURVE_WITH_KNOTS ( 'NONE', 3,
 ( #29751, #5171, #25120, #515, #14461, #25436, #65653, #30098, #14776, #55713, #15123, #10797, #50406, #35060, #5847, #26107, #10147, #4523, #24793, #15459, #20122, #19806, #60692, #10462, #40062, #51397, #36049, #46069, #60351, #50064, #56349, #30425 ),
 .UNSPECIFIED., .F., .F.,
 ( 4, 2, 2, 2, 2, 2, 2, 2, 2, 2, 2, 2, 2, 2, 2, 4 ),
 ( 1.941418318260282306E-17, 0.003213204025811739785, 0.004819806038717596233, 0.006426408051623453549, 0.008033010064529310865, 0.009639612077435168180, 0.01124621409034102550, 0.01204951509679395329, 0.01285281610324688281, 0.01606602012905859744, 0.01927922415487031207, 0.02008252516132323987, 0.02088582616777616766, 0.02249242818068202671, 0.02409903019358788576, 0.02570563220649374828 ),
 .UNSPECIFIED. ) ;
#33455=( GEOMETRIC_REPRESENTATION_CONTEXT ( 3 ) GLOBAL_UNCERTAINTY_ASSIGNED_CONTEXT ( ( #42977 ) ) GLOBAL_UNIT_ASSIGNED_CONTEXT ( ( #58470, #53144, #2286 ) ) REPRESENTATION_CONTEXT ( 'NONE', 'WORKASPACE' ) );
#33456=VERTEX_POINT ( 'NONE', #51905 ) ;
#33457=DIRECTION ( 'NONE',  ( 0.000000000000000000, 0.01356324068817992175, -0.9999080150203990547 ) ) ;
#33460=CYLINDRICAL_SURFACE ( 'NONE', #12943, 6.095312090839646757 ) ;
#33461=FACE_OUTER_BOUND ( 'NONE', #31599, .T. ) ;
#33463=ADVANCED_FACE ( 'NONE', ( #35911 ), #51256, .T. ) ;
#33465=DIRECTION ( 'NONE',  ( 0.000000000000000000, -0.9718671068226434340, 0.2355298848897617037 ) ) ;
#33466=CYLINDRICAL_SURFACE ( 'NONE', #38655, 5.000000000000000000 ) ;
#33467=ORIENTED_EDGE ( 'NONE', *, *, #3021, .F. ) ;
#33468=CARTESIAN_POINT ( 'NONE',  ( -17.87891481078355227, 12.92455976930240524, 3.899497271525859787 ) ) ;
#33470=DIRECTION ( 'NONE',  ( 0.000000000000000000, 0.01356324068817998940, -0.9999080150203990547 ) ) ;
#33472=EDGE_CURVE ( 'NONE', #53899, #40556, #46261, .T. ) ;
#33474=CIRCLE ( 'NONE', #541, 5.000000000000000888 ) ;
#33475=CARTESIAN_POINT ( 'NONE',  ( -35.00000000000000000, -10.75351884295731253, 4.725891942574718563 ) ) ;
#33476=ADVANCED_FACE ( 'NONE', ( #56901 ), #6346, .T. ) ;
#33478=EDGE_LOOP ( 'NONE', ( #11309, #11285, #34851, #52758 ) ) ;
#33479=DIRECTION ( 'NONE',  ( -1.000000000000000000, 0.000000000000000000, 0.000000000000000000 ) ) ;
#33481=CARTESIAN_POINT ( 'NONE',  ( -37.00000000000000711, 2.905556151562625811, 11.38112321385051651 ) ) ;
#33482=CARTESIAN_POINT ( 'NONE',  ( 37.00000000000000711, 4.705694406421931860E-17, -3.469127814946512892E-15 ) ) ;
#33488=CARTESIAN_POINT ( 'NONE',  ( -36.00000000000000711, -7.238157050195700215, 10.49626516989268588 ) ) ;
#33489=VECTOR ( 'NONE', #28896, 1000.000000000000000 ) ;
#33491=CARTESIAN_POINT ( 'NONE',  ( -27.86440745243244521, -9.318414989681810923, -7.586129753734442538 ) ) ;
#33492=ORIENTED_EDGE ( 'NONE', *, *, #65528, .F. ) ;
#33494=CYLINDRICAL_SURFACE ( 'NONE', #3638, 12.18649999999999878 ) ;
#33498=CARTESIAN_POINT ( 'NONE',  ( -35.00000000000000000, 6.303578524886947143, 10.42955799785322490 ) ) ;
#33499=CARTESIAN_POINT ( 'NONE',  ( 35.00000000000000000, -9.752226076388938125, -6.547236723513990775 ) ) ;
#33507=ORIENTED_EDGE ( 'NONE', *, *, #36841, .T. ) ;
#33509=DIRECTION ( 'NONE',  ( 1.000000000000000000, 0.000000000000000000, 0.000000000000000000 ) ) ;
#33510=CARTESIAN_POINT ( 'NONE',  ( -47.00000000000000711, 0.000000000000000000, 0.000000000000000000 ) ) ;
#33511=AXIS2_PLACEMENT_3D ( 'NONE', #1838, #17459, #41734 ) ;
#33514=CARTESIAN_POINT ( 'NONE',  ( 25.05309951391468459, 25.00000000000000000, -8.132934882857099979 ) ) ;
#33516=DIRECTION ( 'NONE',  ( 0.000000000000000000, -0.01356324068817998940, 0.9999080150203990547 ) ) ;
#33518=ORIENTED_EDGE ( 'NONE', *, *, #58672, .T. ) ;
#33522=AXIS2_PLACEMENT_3D ( 'NONE', #48913, #58908, #13632 ) ;
#33523=DIRECTION ( 'NONE',  ( 0.000000000000000000, 0.01356324068817998940, -0.9999080150203990547 ) ) ;
#33526=VERTEX_POINT ( 'NONE', #17307 ) ;
#33527=CARTESIAN_POINT ( 'NONE',  ( -35.00000000000000000, -3.511814412392038953, -11.66953048682403171 ) ) ;
#33530=ORIENTED_EDGE ( 'NONE', *, *, #41807, .T. ) ;
#33532=CARTESIAN_POINT ( 'NONE',  ( 3.291290029914074378, 8.250315036047103590, 25.00000000000000000 ) ) ;
#33533=ORIENTED_EDGE ( 'NONE', *, *, #52381, .F. ) ;
#33535=ORIENTED_EDGE ( 'NONE', *, *, #54192, .F. ) ;
#33536=EDGE_LOOP ( 'NONE', ( #47618, #29503, #57677, #63329 ) ) ;
#33537=CARTESIAN_POINT ( 'NONE',  ( -35.00000000000000000, -2.905556151562544986, -11.38112321385053960 ) ) ;
#33538=DIRECTION ( 'NONE',  ( -1.000000000000000000, 0.000000000000000000, 0.000000000000000000 ) ) ;
#33539=VECTOR ( 'NONE', #2592, 1000.000000000000000 ) ;
#33545=EDGE_CURVE ( 'NONE', #21600, #51686, #28260, .T. ) ;
#33547=DIRECTION ( 'NONE',  ( 0.000000000000000000, -0.5472293298355157543, 0.8369827122275419473 ) ) ;
#33550=FACE_OUTER_BOUND ( 'NONE', #8164, .T. ) ;
#33551=CARTESIAN_POINT ( 'NONE',  ( -18.23163618117759910, 13.26827036841251584, 2.579412572229281775 ) ) ;
#33553=CARTESIAN_POINT ( 'NONE',  ( -35.00000000000000000, -7.499679039484122178, 9.040300684349668714 ) ) ;
#33555=ADVANCED_FACE ( 'NONE', ( #43208 ), #63484, .T. ) ;
#33556=LINE ( 'NONE', #3307, #23604 ) ;
#33558=LINE ( 'NONE', #52550, #21660 ) ;
#33559=AXIS2_PLACEMENT_3D ( 'NONE', #25343, #19726, #20033 ) ;
#33562=DIRECTION ( 'NONE',  ( 1.000000000000000000, 0.000000000000000000, 0.000000000000000000 ) ) ;
#33563=DIRECTION ( 'NONE',  ( 1.000000000000000000, 0.000000000000000000, -0.000000000000000000 ) ) ;
#33564=CARTESIAN_POINT ( 'NONE',  ( 12.66212018674185913, -11.71370580328924227, -6.722415854528632551 ) ) ;
#33566=CARTESIAN_POINT ( 'NONE',  ( 35.00000000000000000, 12.05416472667167760, 1.791059740004291578 ) ) ;
#33567=EDGE_CURVE ( 'NONE', #56695, #37848, #57272, .T. ) ;
#33568=EDGE_LOOP ( 'NONE', ( #6361, #10123, #59511, #60271 ) ) ;
#33569=DIRECTION ( 'NONE',  ( -1.000000000000000000, 0.000000000000000000, 0.000000000000000000 ) ) ;
#33571=CARTESIAN_POINT ( 'NONE',  ( 37.00000000000000711, 4.705694406421931860E-17, -3.469127814946512892E-15 ) ) ;
#33572=DIRECTION ( 'NONE',  ( 0.000000000000000000, -0.2618041379715704275, 0.9651210252299774472 ) ) ;
#33574=CIRCLE ( 'NONE', #12291, 12.18649999999999878 ) ;
#33576=CARTESIAN_POINT ( 'NONE',  ( 35.00000000000000000, -7.146664589317845540, 9.321877890560507751 ) ) ;
#33577=ORIENTED_EDGE ( 'NONE', *, *, #53660, .T. ) ;
#33578=DIRECTION ( 'NONE',  ( -1.000000000000000000, 0.000000000000000000, 0.000000000000000000 ) ) ;
#33580=DIRECTION ( 'NONE',  ( 1.000000000000000000, -0.000000000000000000, 0.000000000000000000 ) ) ;
#33582=ORIENTED_EDGE ( 'NONE', *, *, #45922, .F. ) ;
#33584=CARTESIAN_POINT ( 'NONE',  ( -9.351388602708162523, 12.99278190472488248, -3.665735721005250358 ) ) ;
#33585=EDGE_CURVE ( 'NONE', #27364, #45713, #64466, .T. ) ;
#33588=DIRECTION ( 'NONE',  ( 0.000000000000000000, 0.9105187689795939399, -0.4134677391718545314 ) ) ;
#33590=DIRECTION ( 'NONE',  ( 0.000000000000000000, 0.6269146997507987207, 0.7790879021242507196 ) ) ;
#33591=ADVANCED_FACE ( 'NONE', ( #40173 ), #65128, .T. ) ;
#33593=ORIENTED_EDGE ( 'NONE', *, *, #10788, .F. ) ;
#33595=VERTEX_POINT ( 'NONE', #29873 ) ;
#33599=EDGE_CURVE ( 'NONE', #49092, #42734, #24364, .T. ) ;
#33600=FACE_OUTER_BOUND ( 'NONE', #18481, .T. ) ;
#33602=ORIENTED_EDGE ( 'NONE', *, *, #59371, .F. ) ;
#33604=CARTESIAN_POINT ( 'NONE',  ( -37.00000000000000711, 0.000000000000000000, 0.000000000000000000 ) ) ;
#33607=FACE_OUTER_BOUND ( 'NONE', #30173, .T. ) ;
#33608=ORIENTED_EDGE ( 'NONE', *, *, #56435, .F. ) ;
#33609=ORIENTED_EDGE ( 'NONE', *, *, #11450, .T. ) ;
#33611=ORIENTED_EDGE ( 'NONE', *, *, #14771, .F. ) ;
#33612=DIRECTION ( 'NONE',  ( 0.000000000000000000, 0.01356324068817992175, -0.9999080150203990547 ) ) ;
#33617=CARTESIAN_POINT ( 'NONE',  ( -35.00000000000000000, -6.753013023069787124, 10.14433819232432477 ) ) ;
#33621=VERTEX_POINT ( 'NONE', #8303 ) ;
#33622=DIRECTION ( 'NONE',  ( 0.000000000000000000, -0.01356324068817998940, 0.9999080150203990547 ) ) ;
#33623=EDGE_CURVE ( 'NONE', #40116, #27547, #16915, .T. ) ;
#33624=ORIENTED_EDGE ( 'NONE', *, *, #65077, .F. ) ;
#33625=CYLINDRICAL_SURFACE ( 'NONE', #41252, 12.75000000000000178 ) ;
#33626=CARTESIAN_POINT ( 'NONE',  ( 35.00000000000000000, 4.705694406421931860E-17, -3.469127814946512892E-15 ) ) ;
#33627=ORIENTED_EDGE ( 'NONE', *, *, #44835, .F. ) ;
#33635=CARTESIAN_POINT ( 'NONE',  ( -25.31227681912704597, -12.03780878397515686, 6.112770619466626698 ) ) ;
#33636=CARTESIAN_POINT ( 'NONE',  ( 35.00000000000000000, -9.040300684349746874, -7.499679039484027143 ) ) ;
#33638=DIRECTION ( 'NONE',  ( -1.000000000000000000, -0.000000000000000000, 0.000000000000000000 ) ) ;
#33639=CARTESIAN_POINT ( 'NONE',  ( -18.02751974386707090, -5.811735475709186360, 10.50276896598090204 ) ) ;
#33642=CIRCLE ( 'NONE', #15585, 5.000000000000000000 ) ;
#33644=EDGE_CURVE ( 'NONE', #1816, #7740, #4195, .T. ) ;
#33645=CIRCLE ( 'NONE', #31544, 5.000000000000001776 ) ;
#33646=CARTESIAN_POINT ( 'NONE',  ( -27.16196273015728124, -13.32896842526023029, -2.143521441892683566 ) ) ;
#33647=CARTESIAN_POINT ( 'NONE',  ( 24.73620011133604280, 10.89680678806336545, -7.971846375286735231 ) ) ;
#33649=LINE ( 'NONE', #37970, #8652 ) ;
#33650=CARTESIAN_POINT ( 'NONE',  ( 5.887754249840907228, -9.753796435503998552, -7.002310812516553185 ) ) ;
#33653=ORIENTED_EDGE ( 'NONE', *, *, #38351, .F. ) ;
#33654=CARTESIAN_POINT ( 'NONE',  ( 12.83456828947878314, -10.33636979156220370, -6.108674021912653629 ) ) ;
#33655=ORIENTED_EDGE ( 'NONE', *, *, #37057, .F. ) ;
#33658=LINE ( 'NONE', #8725, #53410 ) ;
#33661=EDGE_LOOP ( 'NONE', ( #65573, #17598, #44139, #38412 ) ) ;
#33662=ORIENTED_EDGE ( 'NONE', *, *, #64051, .F. ) ;
#33663=ORIENTED_EDGE ( 'NONE', *, *, #37092, .T. ) ;
#33664=CARTESIAN_POINT ( 'NONE',  ( 29.51976981715666781, -7.690765383426355406, 11.09513982864076276 ) ) ;
#33667=ORIENTED_EDGE ( 'NONE', *, *, #39529, .F. ) ;
#33671=CARTESIAN_POINT ( 'NONE',  ( 19.28625800530496903, 1.699513388191793428, 11.87904264843580471 ) ) ;
#33673=CARTESIAN_POINT ( 'NONE',  ( -35.00000000000000000, -7.146664589317976102, 9.321877890560418933 ) ) ;
#33675=CARTESIAN_POINT ( 'NONE',  ( -29.76537318338591120, -3.714251817591042393, 11.41077529405956170 ) ) ;
#33676=DIRECTION ( 'NONE',  ( 1.000000000000000000, -0.000000000000000000, 0.000000000000000000 ) ) ;
#33677=ORIENTED_EDGE ( 'NONE', *, *, #28085, .F. ) ;
#33679=ORIENTED_EDGE ( 'NONE', *, *, #29268, .F. ) ;
#33680=CARTESIAN_POINT ( 'NONE',  ( -19.19594308705144314, 13.42342342571188674, -1.564108210525256171 ) ) ;
#33681=ORIENTED_EDGE ( 'NONE', *, *, #25769, .T. ) ;
#33683=DIRECTION ( 'NONE',  ( 1.000000000000000000, 0.000000000000000000, -0.000000000000000000 ) ) ;
#33684=CYLINDRICAL_SURFACE ( 'NONE', #12869, 4.999999999999999112 ) ;
#33685=FACE_OUTER_BOUND ( 'NONE', #40862, .T. ) ;
#33688=VECTOR ( 'NONE', #33747, 1000.000000000000000 ) ;
#33689=CARTESIAN_POINT ( 'NONE',  ( -10.90165637463000614, -7.508992741355389633, -11.21895841913464764 ) ) ;
#33691=EDGE_CURVE ( 'NONE', #2755, #36879, #2340, .T. ) ;
#33692=ORIENTED_EDGE ( 'NONE', *, *, #33821, .F. ) ;
#33693=DIRECTION ( 'NONE',  ( -1.000000000000000000, 0.000000000000000000, 0.000000000000000000 ) ) ;
#33694=VERTEX_POINT ( 'NONE', #59832 ) ;
#33696=ORIENTED_EDGE ( 'NONE', *, *, #28512, .T. ) ;
#33697=DIRECTION ( 'NONE',  ( -1.000000000000000000, -0.000000000000000000, 0.000000000000000000 ) ) ;
#33698=DIRECTION ( 'NONE',  ( -1.000000000000000000, 0.000000000000000000, 0.000000000000000000 ) ) ;
#33699=DIRECTION ( 'NONE',  ( 0.000000000000000000, 0.01356324068817998940, -0.9999080150203990547 ) ) ;
#33701=CARTESIAN_POINT ( 'NONE',  ( -37.00000000000000711, -4.309077947445573820, -10.92721691015460550 ) ) ;
#33702=FACE_OUTER_BOUND ( 'NONE', #2493, .T. ) ;
#33703=EDGE_CURVE ( 'NONE', #31528, #44677, #48777, .T. ) ;
#33704=CARTESIAN_POINT ( 'NONE',  ( -35.00000000000000000, 0.000000000000000000, 0.000000000000000000 ) ) ;
#33705=VERTEX_POINT ( 'NONE', #20576 ) ;
#33708=LINE ( 'NONE', #18766, #51969 ) ;
#33710=AXIS2_PLACEMENT_3D ( 'NONE', #55616, #5396, #64906 ) ;
#33711=DIRECTION ( 'NONE',  ( -1.000000000000000000, 0.000000000000000000, 0.000000000000000000 ) ) ;
#33713=CARTESIAN_POINT ( 'NONE',  ( -9.818496758707208727, -3.216705815951581560, 13.11220466491898407 ) ) ;
#33715=ORIENTED_EDGE ( 'NONE', *, *, #63516, .T. ) ;
#33717=DIRECTION ( 'NONE',  ( -1.000000000000000000, 0.000000000000000000, 0.000000000000000000 ) ) ;
#33719=AXIS2_PLACEMENT_3D ( 'NONE', #13801, #58755, #28147 ) ;
#33720=CIRCLE ( 'NONE', #17839, 12.75000000000000178 ) ;
#33721=CARTESIAN_POINT ( 'NONE',  ( -37.00000000000000711, 1.791059740004591561, -12.05416472667163674 ) ) ;
#33722=CARTESIAN_POINT ( 'NONE',  ( -35.00000000000000000, 0.000000000000000000, 0.000000000000000000 ) ) ;
#33724=CARTESIAN_POINT ( 'NONE',  ( -17.71589014024121411, 3.739618266278695646, 12.97327105657033641 ) ) ;
#33726=CARTESIAN_POINT ( 'NONE',  ( 35.00000000000000000, -8.146229107149464355, -9.063649021438928699 ) ) ;
#33727=VERTEX_POINT ( 'NONE', #35526 ) ;
#33728=DIRECTION ( 'NONE',  ( 1.000000000000000000, 0.000000000000000000, -0.000000000000000000 ) ) ;
#33730=VERTEX_POINT ( 'NONE', #30527 ) ;
#33732=CARTESIAN_POINT ( 'NONE',  ( -37.00000000000000711, 8.496612874013289129, -9.506317355798284296 ) ) ;
#33733=EDGE_CURVE ( 'NONE', #2404, #21209, #51169, .T. ) ;
#33734=ORIENTED_EDGE ( 'NONE', *, *, #5113, .F. ) ;
#33737=CARTESIAN_POINT ( 'NONE',  ( -35.00000000000000000, 8.295159312811854591, 8.927548052240926069 ) ) ;
#33738=DIRECTION ( 'NONE',  ( -1.000000000000000000, 0.000000000000000000, -0.000000000000000000 ) ) ;
#33739=CARTESIAN_POINT ( 'NONE',  ( -35.00000000000000000, -1.908798535168293897, -12.60630747491665282 ) ) ;
#33740=PLANE ( 'NONE',  #31893 ) ;
#33741=ORIENTED_EDGE ( 'NONE', *, *, #35830, .T. ) ;
#33742=CARTESIAN_POINT ( 'NONE',  ( -47.00000000000000711, 0.000000000000000000, 0.000000000000000000 ) ) ;
#33743=VERTEX_POINT ( 'NONE', #50832 ) ;
#33744=DIRECTION ( 'NONE',  ( -1.000000000000000000, 0.000000000000000000, -0.000000000000000000 ) ) ;
#33745=ORIENTED_EDGE ( 'NONE', *, *, #12443, .T. ) ;
#33747=DIRECTION ( 'NONE',  ( 1.000000000000000000, 0.000000000000000000, -0.000000000000000000 ) ) ;
#33749=DIRECTION ( 'NONE',  ( 1.000000000000000000, -0.000000000000000000, 0.000000000000000000 ) ) ;
#33750=EDGE_CURVE ( 'NONE', #22729, #63981, #21208, .T. ) ;
#33751=CARTESIAN_POINT ( 'NONE',  ( 23.98519066662860411, -2.642583004929468959, 11.70655643947132241 ) ) ;
#33753=DIRECTION ( 'NONE',  ( 0.000000000000000000, -0.9999080150203988326, -0.01356324068819046366 ) ) ;
#33756=EDGE_CURVE ( 'NONE', #19313, #29924, #55118, .T. ) ;
#33757=DIRECTION ( 'NONE',  ( 0.000000000000000000, -0.2960891610144577024, -0.9551603052523457427 ) ) ;
#33763=AXIS2_PLACEMENT_3D ( 'NONE', #48028, #12750, #58679 ) ;
#33767=CARTESIAN_POINT ( 'NONE',  ( -36.00000000000000711, 12.02534193257726969, -4.237174932027097718 ) ) ;
#33768=CARTESIAN_POINT ( 'NONE',  ( 37.00000000000000711, 8.573591947375318156, -8.029056188533719052 ) ) ;
#33772=( BOUNDED_CURVE ( )  B_SPLINE_CURVE ( 3, ( #3211, #54069, #28457, #3556 ),
 .UNSPECIFIED., .F., .F. ) 
 B_SPLINE_CURVE_WITH_KNOTS ( ( 4, 4 ),
 ( 2.519937747667190919, 2.535468512986650769 ),
 .UNSPECIFIED. ) 
 CURVE ( )  GEOMETRIC_REPRESENTATION_ITEM ( )  RATIONAL_B_SPLINE_CURVE ( ( 1.000000000000000000, 0.9999798997117221866, 0.9999798997117221866, 1.000000000000000000 ) ) 
 REPRESENTATION_ITEM ( '' )  );
#33773=EDGE_CURVE ( 'NONE', #35253, #56493, #49860, .T. ) ;
#33778=LINE ( 'NONE', #49746, #30231 ) ;
#33779=CARTESIAN_POINT ( 'NONE',  ( -28.24214478236189052, 12.24469403912116761, -5.693128020442387083 ) ) ;
#33780=EDGE_CURVE ( 'NONE', #42105, #33067, #23274, .T. ) ;
#33781=VECTOR ( 'NONE', #40464, 1000.000000000000000 ) ;
#33782=CARTESIAN_POINT ( 'NONE',  ( 7.045079518374575578, -7.884504117378364541, -10.96637384480524524 ) ) ;
#33783=CARTESIAN_POINT ( 'NONE',  ( 35.00000000000000000, -2.772148766916200380, -11.86701198550355585 ) ) ;
#33784=EDGE_CURVE ( 'NONE', #8260, #25967, #10916, .T. ) ;
#33785=DIRECTION ( 'NONE',  ( -1.000000000000000000, 0.000000000000000000, 0.000000000000000000 ) ) ;
#33787=ORIENTED_EDGE ( 'NONE', *, *, #22856, .T. ) ;
#33789=CARTESIAN_POINT ( 'NONE',  ( 35.00000000000000000, -10.07641281632173325, 6.036400161834665212 ) ) ;
#33790=CYLINDRICAL_SURFACE ( 'NONE', #30141, 12.18650000000000055 ) ;
#33791=CIRCLE ( 'NONE', #46533, 12.75000000000000178 ) ;
#33794=AXIS2_PLACEMENT_3D ( 'NONE', #3669, #23602, #4290 ) ;
#33796=EDGE_LOOP ( 'NONE', ( #13965, #60406, #33261, #54713 ) ) ;
#33800=ORIENTED_EDGE ( 'NONE', *, *, #3226, .T. ) ;
#33803=DIRECTION ( 'NONE',  ( -1.000000000000000000, 0.000000000000000000, 0.000000000000000000 ) ) ;
#33804=B_SPLINE_CURVE_WITH_KNOTS ( 'NONE', 3,
 ( #35906, #11319, #31587, #41565, #52231, #30936, #51898, #373, #51250, #56205, #46255, #56555, #25972, #699, #47245, #46899, #20954, #11637 ),
 .UNSPECIFIED., .F., .F.,
 ( 4, 2, 2, 2, 2, 2, 2, 2, 4 ),
 ( 1.192622389734054877E-18, 0.001238680244670008462, 0.002477360489340016056, 0.003716040734010024084, 0.004954720978680030377, 0.006193401223350037538, 0.007432081468020046433, 0.008670761712690053594, 0.009909441957360059020 ),
 .UNSPECIFIED. ) ;
#33807=ADVANCED_FACE ( 'NONE', ( #5956 ), #26213, .T. ) ;
#33808=DIRECTION ( 'NONE',  ( 1.000000000000000000, 0.000000000000000000, -0.000000000000000000 ) ) ;
#33809=ORIENTED_EDGE ( 'NONE', *, *, #42781, .T. ) ;
#33811=DIRECTION ( 'NONE',  ( 1.000000000000000000, 0.000000000000000000, 0.000000000000000000 ) ) ;
#33817=CARTESIAN_POINT ( 'NONE',  ( 35.00000000000000000, -10.49591321039684289, -5.273331777780305707 ) ) ;
#33820=ORIENTED_EDGE ( 'NONE', *, *, #2025, .T. ) ;
#33821=EDGE_CURVE ( 'NONE', #45697, #167, #61520, .T. ) ;
#33822=CARTESIAN_POINT ( 'NONE',  ( -17.65458117747069267, -7.800522896528933714, -9.123980294853460293 ) ) ;
#33823=ORIENTED_EDGE ( 'NONE', *, *, #53341, .T. ) ;
#33825=CARTESIAN_POINT ( 'NONE',  ( 37.00000000000000711, -11.98254675519226531, 2.220215194442026974 ) ) ;
#33826=CARTESIAN_POINT ( 'NONE',  ( 3.347841273039249721, -10.61118957148187825, -8.345816669330458737 ) ) ;
#33828=EDGE_CURVE ( 'NONE', #25074, #311, #27191, .T. ) ;
#33829=LINE ( 'NONE', #17585, #35103 ) ;
#33830=ORIENTED_EDGE ( 'NONE', *, *, #42431, .T. ) ;
#33831=CARTESIAN_POINT ( 'NONE',  ( 37.00000000000000711, 8.839356091080166067, 8.389074212634184846 ) ) ;
#33833=CIRCLE ( 'NONE', #11529, 12.18649999999999700 ) ;
#33837=CARTESIAN_POINT ( 'NONE',  ( -35.00000000000000000, -9.896810808925444292, 7.110831038798244741 ) ) ;
#33838=EDGE_CURVE ( 'NONE', #37783, #14488, #48473, .T. ) ;
#33839=FACE_OUTER_BOUND ( 'NONE', #46292, .T. ) ;
#33840=ORIENTED_EDGE ( 'NONE', *, *, #49829, .F. ) ;
#33841=VERTEX_POINT ( 'NONE', #28184 ) ;
#33842=DIRECTION ( 'NONE',  ( -1.000000000000000000, 0.000000000000000000, 0.000000000000000000 ) ) ;
#33846=CARTESIAN_POINT ( 'NONE',  ( -35.00000000000000000, -1.171570255487366152, -11.68758509253249400 ) ) ;
#33848=DIRECTION ( 'NONE',  ( -1.000000000000000000, -1.836970198721029688E-16, 0.000000000000000000 ) ) ;
#33849=VECTOR ( 'NONE', #21376, 1000.000000000000000 ) ;
#33851=ORIENTED_EDGE ( 'NONE', *, *, #5961, .T. ) ;
#33853=EDGE_CURVE ( 'NONE', #55855, #36091, #38163, .T. ) ;
#33855=AXIS2_PLACEMENT_3D ( 'NONE', #30182, #29513, #4265 ) ;
#33857=CARTESIAN_POINT ( 'NONE',  ( -19.79851336404619744, -13.40886403912690206, -1.595110065591720083 ) ) ;
#33858=EDGE_CURVE ( 'NONE', #56666, #1032, #57799, .T. ) ;
#33859=FACE_OUTER_BOUND ( 'NONE', #29512, .T. ) ;
#33860=DIRECTION ( 'NONE',  ( -1.000000000000000000, 0.000000000000000000, -0.000000000000000000 ) ) ;
#33864=AXIS2_PLACEMENT_3D ( 'NONE', #22095, #62015, #1515 ) ;
#33865=LINE ( 'NONE', #40485, #45908 ) ;
#33867=ORIENTED_EDGE ( 'NONE', *, *, #47313, .T. ) ;
#33868=DIRECTION ( 'NONE',  ( 0.000000000000000000, 0.5243256840888502746, 0.8515178078024904229 ) ) ;
#33871=ORIENTED_EDGE ( 'NONE', *, *, #51656, .F. ) ;
#33872=CARTESIAN_POINT ( 'NONE',  ( -11.35260098629715309, -8.408840821862247239, 8.581102366670037895 ) ) ;
#33873=CARTESIAN_POINT ( 'NONE',  ( 37.00000000000000711, -12.16632754454236043, 0.7008968033240018380 ) ) ;
#33874=DIRECTION ( 'NONE',  ( 1.000000000000000000, 0.000000000000000000, 0.000000000000000000 ) ) ;
#33877=CARTESIAN_POINT ( 'NONE',  ( 37.00000000000000711, 11.95840593935204765, 2.346765782874299155 ) ) ;
#33878=ORIENTED_EDGE ( 'NONE', *, *, #59985, .T. ) ;
#33879=DIRECTION ( 'NONE',  ( 0.000000000000000000, -0.01356324068817991828, 0.9999080150203990547 ) ) ;
#33880=CARTESIAN_POINT ( 'NONE',  ( 22.68159425457230682, -4.559965384753717821, 12.70733236524612764 ) ) ;
#33883=AXIS2_PLACEMENT_3D ( 'NONE', #19127, #60030, #14447 ) ;
#33885=ORIENTED_EDGE ( 'NONE', *, *, #170, .T. ) ;
#33887=CARTESIAN_POINT ( 'NONE',  ( -18.11253622212529280, 11.56839684805698276, 3.263418409390943076 ) ) ;
#33892=DIRECTION ( 'NONE',  ( 0.000000000000000000, 0.01356324068817998940, -0.9999080150203990547 ) ) ;
#33898=AXIS2_PLACEMENT_3D ( 'NONE', #65760, #51509, #20886 ) ;
#33899=DIRECTION ( 'NONE',  ( 1.000000000000000000, -0.000000000000000000, -0.000000000000000000 ) ) ;
#33900=CARTESIAN_POINT ( 'NONE',  ( 37.00000000000000711, 11.05394794832829497, -5.130401251914769922 ) ) ;
#33901=CARTESIAN_POINT ( 'NONE',  ( 35.00000000000000000, 11.91791701451269780, 2.544412758415707909 ) ) ;
#33905=ORIENTED_EDGE ( 'NONE', *, *, #21521, .F. ) ;
#33907=ORIENTED_EDGE ( 'NONE', *, *, #535, .T. ) ;
#33908=FACE_OUTER_BOUND ( 'NONE', #25455, .T. ) ;
#33909=CARTESIAN_POINT ( 'NONE',  ( -36.00000000000000711, 11.96656215839369253, 4.400442035670988794 ) ) ;
#33911=CARTESIAN_POINT ( 'NONE',  ( -35.00000000000000000, 9.908974237959645492, 6.307491713049065751 ) ) ;
#33912=LINE ( 'NONE', #27288, #49168 ) ;
#33913=ORIENTED_EDGE ( 'NONE', *, *, #53199, .T. ) ;
#33917=VERTEX_POINT ( 'NONE', #21474 ) ;
#33918=VERTEX_POINT ( 'NONE', #52059 ) ;
#33920=EDGE_CURVE ( 'NONE', #58860, #9046, #34923, .T. ) ;
#33921=ORIENTED_EDGE ( 'NONE', *, *, #51716, .T. ) ;
#33922=CARTESIAN_POINT ( 'NONE',  ( 35.00000000000000000, -11.47758908105696207, -2.497432891016804657 ) ) ;
#33924=ORIENTED_EDGE ( 'NONE', *, *, #60292, .T. ) ;
#33925=VERTEX_POINT ( 'NONE', #1194 ) ;
#33926=CARTESIAN_POINT ( 'NONE',  ( 47.00000000000000711, 4.705694406421931860E-17, -3.469127814946512892E-15 ) ) ;
#33927=DIRECTION ( 'NONE',  ( 0.000000000000000000, 0.9718671068226467646, -0.2355298848897482977 ) ) ;
#33928=CIRCLE ( 'NONE', #42400, 4.999999999999998224 ) ;
#33930=CARTESIAN_POINT ( 'NONE',  ( -8.891032880924177206, 25.00000000000000000, -3.860857758255646921 ) ) ;
#33931=DIRECTION ( 'NONE',  ( 0.000000000000000000, 0.9999080150203990547, 0.01356324068817645230 ) ) ;
#33934=ORIENTED_EDGE ( 'NONE', *, *, #63129, .F. ) ;
#33935=AXIS2_PLACEMENT_3D ( 'NONE', #45990, #56276, #30364 ) ;
#33936=CARTESIAN_POINT ( 'NONE',  ( -35.00000000000000000, 11.30684963584389280, 4.545979934229452901 ) ) ;
#33937=CARTESIAN_POINT ( 'NONE',  ( -19.69476066079020171, -4.201994156881551312, -12.82938989607585789 ) ) ;
#33948=ORIENTED_EDGE ( 'NONE', *, *, #15529, .F. ) ;
#33949=DIRECTION ( 'NONE',  ( -1.000000000000000000, 0.000000000000000000, 0.000000000000000000 ) ) ;
#33950=DIRECTION ( 'NONE',  ( -1.000000000000000000, -0.000000000000000000, 0.000000000000000000 ) ) ;
#33951=CARTESIAN_POINT ( 'NONE',  ( -29.95040744112532494, 0.8263397880752897384, 13.47653596729246672 ) ) ;
#33954=CYLINDRICAL_SURFACE ( 'NONE', #4182, 12.18649999999999878 ) ;
#33955=ORIENTED_EDGE ( 'NONE', *, *, #9994, .T. ) ;
#33957=CARTESIAN_POINT ( 'NONE',  ( 37.00000000000000711, -11.13736569743270799, 4.946702696913285457 ) ) ;
#33958=CARTESIAN_POINT ( 'NONE',  ( 35.00000000000000000, -8.699265615723042799, -8.534258022646065811 ) ) ;
#33960=CARTESIAN_POINT ( 'NONE',  ( -35.00000000000000000, -4.725891942574680371, -10.75351884295732496 ) ) ;
#33963=DIRECTION ( 'NONE',  ( -1.000000000000000000, 0.000000000000000000, 0.000000000000000000 ) ) ;
#33964=DIRECTION ( 'NONE',  ( -1.000000000000000000, -0.000000000000000000, 0.000000000000000000 ) ) ;
#33969=CARTESIAN_POINT ( 'NONE',  ( -35.00000000000000000, 0.01609748574461371262, -11.74614673114903951 ) ) ;
#33970=ADVANCED_FACE ( 'NONE', ( #28106 ), #63993, .T. ) ;
#33974=DIRECTION ( 'NONE',  ( -1.000000000000000000, -0.000000000000000000, -0.000000000000000000 ) ) ;
#33976=DIRECTION ( 'NONE',  ( -1.000000000000000000, 0.000000000000000000, 0.000000000000000000 ) ) ;
#33980=VERTEX_POINT ( 'NONE', #53708 ) ;
#33982=VECTOR ( 'NONE', #11821, 1000.000000000000000 ) ;
#33984=CYLINDRICAL_SURFACE ( 'NONE', #16467, 12.75000000000000178 ) ;
#33988=CYLINDRICAL_SURFACE ( 'NONE', #51342, 3.309571291727934295 ) ;
#33990=DIRECTION ( 'NONE',  ( 1.000000000000000000, 0.000000000000000000, 0.000000000000000000 ) ) ;
#33991=DIRECTION ( 'NONE',  ( -1.000000000000000000, 0.000000000000000000, 0.000000000000000000 ) ) ;
#33992=FACE_OUTER_BOUND ( 'NONE', #783, .T. ) ;
#33994=ORIENTED_EDGE ( 'NONE', *, *, #24953, .T. ) ;
#33995=EDGE_CURVE ( 'NONE', #19006, #48895, #56209, .T. ) ;
#33997=VERTEX_POINT ( 'NONE', #29087 ) ;
#33999=AXIS2_PLACEMENT_3D ( 'NONE', #12173, #2558, #18159 ) ;
#34001=CARTESIAN_POINT ( 'NONE',  ( 21.62617364511530837, -11.90943727674767416, -1.526638328776592779 ) ) ;
#34003=ADVANCED_FACE ( 'NONE', ( #49057 ), #14099, .T. ) ;
#34005=CARTESIAN_POINT ( 'NONE',  ( -2.952869152607106251, 11.39722960915212724, 3.755417052241485365 ) ) ;
#34006=FACE_OUTER_BOUND ( 'NONE', #46456, .T. ) ;
#34007=FACE_OUTER_BOUND ( 'NONE', #48553, .T. ) ;
#34008=DIRECTION ( 'NONE',  ( 1.000000000000000000, 0.000000000000000000, 0.000000000000000000 ) ) ;
#34009=AXIS2_PLACEMENT_3D ( 'NONE', #35886, #45551, #30912 ) ;
#34010=ORIENTED_EDGE ( 'NONE', *, *, #27357, .T. ) ;
#34018=LINE ( 'NONE', #37715, #23147 ) ;
#34019=EDGE_CURVE ( 'NONE', #12979, #59777, #63305, .T. ) ;
#34021=AXIS2_PLACEMENT_3D ( 'NONE', #13918, #8956, #23606 ) ;
#34022=CIRCLE ( 'NONE', #30826, 4.999999999999998224 ) ;
#34023=CIRCLE ( 'NONE', #54210, 12.74999999999999822 ) ;
#34024=CIRCLE ( 'NONE', #3242, 12.18650000000000055 ) ;
#34026=EDGE_CURVE ( 'NONE', #38075, #20003, #31799, .T. ) ;
#34027=ORIENTED_EDGE ( 'NONE', *, *, #21713, .F. ) ;
#34028=CARTESIAN_POINT ( 'NONE',  ( -35.00000000000000000, 3.511814412392118445, 11.66953048682401040 ) ) ;
#34029=CARTESIAN_POINT ( 'NONE',  ( -35.00000000000000000, 6.475373545682302279, 10.32377448871670467 ) ) ;
#34030=CARTESIAN_POINT ( 'NONE',  ( -17.14880393894236832, -7.773003649151587702, 11.04270090464071075 ) ) ;
#34031=ORIENTED_EDGE ( 'NONE', *, *, #59994, .T. ) ;
#34032=CIRCLE ( 'NONE', #36156, 12.18650000000000233 ) ;
#34033=CIRCLE ( 'NONE', #6427, 5.000000000000001776 ) ;
#34034=AXIS2_PLACEMENT_3D ( 'NONE', #42455, #54447, #43799 ) ;
#34035=CARTESIAN_POINT ( 'NONE',  ( 35.00000000000000000, 11.01837265713072966, -6.415447294506745557 ) ) ;
#34036=AXIS2_PLACEMENT_3D ( 'NONE', #39178, #32869, #48220 ) ;
#34037=LINE ( 'NONE', #34683, #39495 ) ;
#34038=VERTEX_POINT ( 'NONE', #4138 ) ;
#34041=CARTESIAN_POINT ( 'NONE',  ( 37.00000000000000711, 4.705694406421931860E-17, -3.469127814946512892E-15 ) ) ;
#34042=AXIS2_PLACEMENT_3D ( 'NONE', #30266, #65179, #50562 ) ;
#34043=CARTESIAN_POINT ( 'NONE',  ( -35.00000000000000000, 0.000000000000000000, 0.000000000000000000 ) ) ;
#34044=CARTESIAN_POINT ( 'NONE',  ( 3.459614771489464946, -11.09853614738469396, 7.685863346768216253 ) ) ;
#34045=VECTOR ( 'NONE', #57085, 1000.000000000000000 ) ;
#34046=EDGE_CURVE ( 'NONE', #52529, #25546, #8464, .T. ) ;
#34047=ORIENTED_EDGE ( 'NONE', *, *, #32320, .F. ) ;
#34051=ORIENTED_EDGE ( 'NONE', *, *, #39285, .F. ) ;
#34052=CARTESIAN_POINT ( 'NONE',  ( 8.626064170299294176, 3.158121739564950126, 13.12798721807445368 ) ) ;
#34053=CIRCLE ( 'NONE', #57425, 4.999999999999999112 ) ;
#34055=VERTEX_POINT ( 'NONE', #60000 ) ;
#34057=ORIENTED_EDGE ( 'NONE', *, *, #51926, .F. ) ;
#34058=CARTESIAN_POINT ( 'NONE',  ( 37.00000000000000711, 8.258652103341434625, -8.352657516904704593 ) ) ;
#34060=EDGE_CURVE ( 'NONE', #48764, #43267, #24404, .T. ) ;
#34062=CARTESIAN_POINT ( 'NONE',  ( 19.13486214123187423, 6.258902428715833466, 11.96274114462061533 ) ) ;
#34066=DIRECTION ( 'NONE',  ( 1.000000000000000000, 0.000000000000000000, -0.000000000000000000 ) ) ;
#34068=ORIENTED_EDGE ( 'NONE', *, *, #50336, .T. ) ;
#34069=CARTESIAN_POINT ( 'NONE',  ( 35.00000000000000000, 4.705694406421931860E-17, -3.469127814946512892E-15 ) ) ;
#34070=VERTEX_POINT ( 'NONE', #39047 ) ;
#34071=DIRECTION ( 'NONE',  ( 0.000000000000000000, 0.01356324068818000848, -0.9999080150203990547 ) ) ;
#34074=CARTESIAN_POINT ( 'NONE',  ( -14.37447982603986141, 8.347221320025207447, 10.61079098056672620 ) ) ;
#34076=CARTESIAN_POINT ( 'NONE',  ( -24.30576933614230484, 10.54161591164828415, 8.435916383667265706 ) ) ;
#34078=DIRECTION ( 'NONE',  ( 1.000000000000000000, -0.000000000000000000, 0.000000000000000000 ) ) ;
#34080=EDGE_LOOP ( 'NONE', ( #3922, #49891, #52483, #26735 ) ) ;
#34082=AXIS2_PLACEMENT_3D ( 'NONE', #17656, #52886, #47907 ) ;
#34083=CARTESIAN_POINT ( 'NONE',  ( 37.00000000000000711, 6.891188680298960811, 9.512294188640820991 ) ) ;
#34084=ORIENTED_EDGE ( 'NONE', *, *, #25139, .T. ) ;
#34085=VECTOR ( 'NONE', #15527, 1000.000000000000000 ) ;
#34086=CARTESIAN_POINT ( 'NONE',  ( 35.00000000000000000, 1.791059740004421919, -12.05416472667166339 ) ) ;
#34088=DIRECTION ( 'NONE',  ( 0.000000000000000000, 0.01356324068817992175, -0.9999080150203990547 ) ) ;
#34089=DIRECTION ( 'NONE',  ( -1.000000000000000000, 0.000000000000000000, 0.000000000000000000 ) ) ;
#34092=DIRECTION ( 'NONE',  ( 1.000000000000000000, 0.000000000000000000, 0.000000000000000000 ) ) ;
#34094=ORIENTED_EDGE ( 'NONE', *, *, #34210, .T. ) ;
#34097=CARTESIAN_POINT ( 'NONE',  ( -35.00000000000000000, 0.000000000000000000, 0.000000000000000000 ) ) ;
#34098=CARTESIAN_POINT ( 'NONE',  ( 37.00000000000000711, -6.950793414699864670, -10.68873102412840304 ) ) ;
#34099=EDGE_CURVE ( 'NONE', #19106, #56769, #54365, .T. ) ;
#34101=AXIS2_PLACEMENT_3D ( 'NONE', #11388, #17035, #17379 ) ;
#34103=AXIS2_PLACEMENT_3D ( 'NONE', #40416, #60719, #55737 ) ;
#34104=CARTESIAN_POINT ( 'NONE',  ( -27.87914506689667959, 11.20956315821615412, -7.546760284812030761 ) ) ;
#34105=CARTESIAN_POINT ( 'NONE',  ( -6.413058664601522629, -1.625581343069429474, -11.88948361578930069 ) ) ;
#34106=DIRECTION ( 'NONE',  ( 0.000000000000000000, -1.000000000000000000, 0.000000000000000000 ) ) ;
#34111=CARTESIAN_POINT ( 'NONE',  ( -37.00000000000000711, 7.251710744571578715, 9.240395740215660680 ) ) ;
#34112=CARTESIAN_POINT ( 'NONE',  ( -35.00000000000000000, 0.000000000000000000, 0.000000000000000000 ) ) ;
#34113=B_SPLINE_CURVE_WITH_KNOTS ( 'NONE', 3,
 ( #59770, #60092, #4239, #34152, #33822, #53807, #14199, #59434, #29487, #44783, #65066, #39140, #24507, #39807, #28204, #8243, #44448, #3617, #64726, #3270 ),
 .UNSPECIFIED., .F., .F.,
 ( 4, 2, 2, 2, 2, 2, 2, 2, 2, 4 ),
 ( 4.906538933386796626E-18, 0.001836704664428997482, 0.002755056996643492646, 0.003673409328857988026, 0.004591761661072483840, 0.005050937827179729361, 0.005510113993286975750, 0.006428466325501474600, 0.006887642491608728795, 0.007346818657715982991 ),
 .UNSPECIFIED. ) ;
#34115=CIRCLE ( 'NONE', #42606, 4.999999999999999112 ) ;
#34116=EDGE_CURVE ( 'NONE', #62051, #3315, #18120, .T. ) ;
#34117=AXIS2_PLACEMENT_3D ( 'NONE', #30440, #19498, #55056 ) ;
#34120=EDGE_CURVE ( 'NONE', #11257, #63179, #23329, .T. ) ;
#34122=EDGE_CURVE ( 'NONE', #60252, #13554, #55163, .T. ) ;
#34124=CARTESIAN_POINT ( 'NONE',  ( 27.62838931380291996, 25.00000000000000000, -3.066727421130092779 ) ) ;
#34126=ORIENTED_EDGE ( 'NONE', *, *, #21728, .T. ) ;
#34128=CARTESIAN_POINT ( 'NONE',  ( -7.145635969647290864, -1.338498515901911157, -13.43367374991614227 ) ) ;
#34129=CARTESIAN_POINT ( 'NONE',  ( 35.00000000000000000, 11.38112321385050585, -2.905556151562669331 ) ) ;
#34131=CARTESIAN_POINT ( 'NONE',  ( 18.06755238356944204, -8.467740623938468048, 10.54028520740660646 ) ) ;
#34132=AXIS2_PLACEMENT_3D ( 'NONE', #10464, #30739, #25780 ) ;
#34134=B_SPLINE_CURVE_WITH_KNOTS ( 'NONE', 3,
 ( #37942, #53251, #7698, #22995, #27982, #24200, #58582, #8036, #38259, #32293, #59786, #48289, #2736, #43250 ),
 .UNSPECIFIED., .F., .F.,
 ( 4, 2, 2, 2, 2, 2, 4 ),
 ( 2.453269466693398698E-18, 0.001754878791416509013, 0.002632318187124761677, 0.003509757582833014124, 0.004387196978541266570, 0.005264636374249519017, 0.007019515165666019574 ),
 .UNSPECIFIED. ) ;
#34135=DIRECTION ( 'NONE',  ( 1.000000000000000000, 0.000000000000000000, 0.000000000000000000 ) ) ;
#34136=EDGE_CURVE ( 'NONE', #325, #11644, #46669, .T. ) ;
#34138=EDGE_LOOP ( 'NONE', ( #22164, #45723, #53316, #44632 ) ) ;
#34139=CARTESIAN_POINT ( 'NONE',  ( -35.00000000000000000, -1.030638227056651424, 12.14284015767849567 ) ) ;
#34140=CIRCLE ( 'NONE', #47936, 5.000000000000002665 ) ;
#34142=CARTESIAN_POINT ( 'NONE',  ( -17.54726996257253191, 12.93490414535030020, 3.865003848717349033 ) ) ;
#34143=DIRECTION ( 'NONE',  ( -1.000000000000000000, 0.000000000000000000, 0.000000000000000000 ) ) ;
#34145=DIRECTION ( 'NONE',  ( 1.000000000000000000, 0.000000000000000000, 0.000000000000000000 ) ) ;
#34146=ADVANCED_FACE ( 'NONE', ( #19767 ), #25077, .F. ) ;
#34147=CARTESIAN_POINT ( 'NONE',  ( -35.00000000000000000, 0.000000000000000000, 0.000000000000000000 ) ) ;
#34148=CARTESIAN_POINT ( 'NONE',  ( -35.00000000000000000, 0.000000000000000000, 0.000000000000000000 ) ) ;
#34151=ORIENTED_EDGE ( 'NONE', *, *, #14740, .T. ) ;
#34152=CARTESIAN_POINT ( 'NONE',  ( -17.68631299100147203, -8.034711453839296524, -8.918265921354986858 ) ) ;
#34156=DIRECTION ( 'NONE',  ( -1.000000000000000000, 0.000000000000000000, 0.000000000000000000 ) ) ;
#34158=AXIS2_PLACEMENT_3D ( 'NONE', #30378, #50997, #15410 ) ;
#34161=VERTEX_POINT ( 'NONE', #50364 ) ;
#34162=DIRECTION ( 'NONE',  ( -1.000000000000000000, 0.000000000000000000, 0.000000000000000000 ) ) ;
#34164=CARTESIAN_POINT ( 'NONE',  ( 35.00000000000000000, -1.030638227056475120, 12.14284015767850811 ) ) ;
#34165=CARTESIAN_POINT ( 'NONE',  ( 23.19610847111811935, -4.580350341167983785, 12.70186574010239866 ) ) ;
#34166=ORIENTED_EDGE ( 'NONE', *, *, #60195, .F. ) ;
#34169=CARTESIAN_POINT ( 'NONE',  ( 37.00000000000000711, -9.240395740215580744, 7.251710744571670197 ) ) ;
#34170=ORIENTED_EDGE ( 'NONE', *, *, #51064, .F. ) ;
#34171=ORIENTED_EDGE ( 'NONE', *, *, #32575, .F. ) ;
#34172=CIRCLE ( 'NONE', #10820, 4.999999999999999112 ) ;
#34174=DIRECTION ( 'NONE',  ( 0.000000000000000000, -0.9937233664769749009, 0.1118654143051720229 ) ) ;
#34176=CARTESIAN_POINT ( 'NONE',  ( 2.354167843600960097, -6.278647867796540716, 25.00000000000000000 ) ) ;
#34177=CARTESIAN_POINT ( 'NONE',  ( -35.00000000000000000, 11.53507381115580444, 2.216820770815288721 ) ) ;
#34178=VECTOR ( 'NONE', #53020, 1000.000000000000000 ) ;
#34180=VERTEX_POINT ( 'NONE', #9422 ) ;
#34183=AXIS2_PLACEMENT_3D ( 'NONE', #60923, #60580, #4759 ) ;
#34184=CARTESIAN_POINT ( 'NONE',  ( 35.00000000000000000, 10.14433819232443490, 6.753013023069603271 ) ) ;
#34186=CARTESIAN_POINT ( 'NONE',  ( 29.27326790309752980, 9.878007402510375456, 6.829635556393566453 ) ) ;
#34189=DIRECTION ( 'NONE',  ( 0.000000000000000000, 0.01356324068817998940, -0.9999080150203989437 ) ) ;
#34190=LINE ( 'NONE', #60124, #64205 ) ;
#34192=EDGE_CURVE ( 'NONE', #8491, #63532, #4479, .T. ) ;
#34193=VERTEX_POINT ( 'NONE', #10104 ) ;
#34194=CARTESIAN_POINT ( 'NONE',  ( -16.35799066125883527, 8.282504492528538265, -8.683502121879305591 ) ) ;
#34195=VECTOR ( 'NONE', #1507, 1000.000000000000000 ) ;
#34197=CARTESIAN_POINT ( 'NONE',  ( 37.00000000000000711, 1.457575200925545822, -12.66641127287626567 ) ) ;
#34202=ORIENTED_EDGE ( 'NONE', *, *, #12007, .F. ) ;
#34203=DIRECTION ( 'NONE',  ( 0.000000000000000000, 0.8009703041134188517, 0.5987040770935648792 ) ) ;
#34208=AXIS2_PLACEMENT_3D ( 'NONE', #23335, #18368, #53930 ) ;
#34209=VECTOR ( 'NONE', #37882, 1000.000000000000000 ) ;
#34210=EDGE_CURVE ( 'NONE', #58300, #53581, #16962, .T. ) ;
#34211=DIRECTION ( 'NONE',  ( -1.000000000000000000, 0.000000000000000000, 0.000000000000000000 ) ) ;
#34215=EDGE_LOOP ( 'NONE', ( #22441, #58381, #7562, #25687 ) ) ;
#34216=EDGE_CURVE ( 'NONE', #34377, #35057, #61569, .T. ) ;
#34219=CARTESIAN_POINT ( 'NONE',  ( 37.00000000000000711, 4.705694406421931860E-17, -3.469127814946512892E-15 ) ) ;
#34220=VECTOR ( 'NONE', #22140, 1000.000000000000000 ) ;
#34221=CARTESIAN_POINT ( 'NONE',  ( -29.43980975494970309, -3.641506875706034041, -12.99959336572439561 ) ) ;
#34222=AXIS2_PLACEMENT_3D ( 'NONE', #33333, #28026, #3762 ) ;
#34224=EDGE_CURVE ( 'NONE', #36765, #18385, #34695, .T. ) ;
#34225=VERTEX_POINT ( 'NONE', #48562 ) ;
#34226=DIRECTION ( 'NONE',  ( 0.000000000000000000, 0.3218879778915905709, -0.9467777615094595811 ) ) ;
#34227=DIRECTION ( 'NONE',  ( 1.000000000000000000, 0.000000000000000000, 0.000000000000000000 ) ) ;
#34228=CARTESIAN_POINT ( 'NONE',  ( 35.00000000000000000, 6.753013023069713405, -10.14433819232436917 ) ) ;
#34229=AXIS2_PLACEMENT_3D ( 'NONE', #12166, #15912, #61161 ) ;
#34231=DIRECTION ( 'NONE',  ( 0.000000000000000000, 0.7196168960969817618, 0.6943713148249615053 ) ) ;
#34232=EDGE_CURVE ( 'NONE', #44679, #2111, #28583, .T. ) ;
#34235=EDGE_LOOP ( 'NONE', ( #9464, #13549, #54215, #26957 ) ) ;
#34236=ORIENTED_EDGE ( 'NONE', *, *, #56532, .T. ) ;
#34238=EDGE_CURVE ( 'NONE', #51547, #8029, #3163, .T. ) ;
#34239=DIRECTION ( 'NONE',  ( -1.000000000000000000, -1.836970198721029688E-16, 0.000000000000000000 ) ) ;
#34240=EDGE_LOOP ( 'NONE', ( #55635, #63357, #11694, #48798 ) ) ;
#34241=LINE ( 'NONE', #49563, #19876 ) ;
#34242=EDGE_CURVE ( 'NONE', #40631, #60763, #23273, .T. ) ;
#34243=CIRCLE ( 'NONE', #46980, 5.000000000000000888 ) ;
#34245=ORIENTED_EDGE ( 'NONE', *, *, #18582, .T. ) ;
#34248=CARTESIAN_POINT ( 'NONE',  ( 35.00000000000000000, -9.063649021438894948, 8.146229107149494553 ) ) ;
#34249=VERTEX_POINT ( 'NONE', #11093 ) ;
#34251=EDGE_CURVE ( 'NONE', #28701, #63705, #45068, .T. ) ;
#34256=AXIS2_PLACEMENT_3D ( 'NONE', #63005, #18471, #63990 ) ;
#34257=AXIS2_PLACEMENT_3D ( 'NONE', #651, #35550, #61803 ) ;
#34259=EDGE_LOOP ( 'NONE', ( #15598, #20368, #17662, #11330 ) ) ;
#34260=CARTESIAN_POINT ( 'NONE',  ( 34.00000000000000000, 1.267509437117510519E-14, 0.000000000000000000 ) ) ;
#34262=CIRCLE ( 'NONE', #56578, 12.75000000000000178 ) ;
#34269=ORIENTED_EDGE ( 'NONE', *, *, #3729, .T. ) ;
#34270=LINE ( 'NONE', #63533, #928 ) ;
#34271=CYLINDRICAL_SURFACE ( 'NONE', #17100, 5.000000000000000888 ) ;
#34276=ORIENTED_EDGE ( 'NONE', *, *, #51600, .T. ) ;
#34277=AXIS2_PLACEMENT_3D ( 'NONE', #45857, #9594, #19921 ) ;
#34279=VERTEX_POINT ( 'NONE', #16413 ) ;
#34282=CARTESIAN_POINT ( 'NONE',  ( -24.67437105727481494, -11.54489660803197282, 7.000040830933849989 ) ) ;
#34283=DIRECTION ( 'NONE',  ( 1.000000000000000000, -0.000000000000000000, 0.000000000000000000 ) ) ;
#34287=CARTESIAN_POINT ( 'NONE',  ( 35.00000000000000000, 1.791059740004421919, -12.05416472667166339 ) ) ;
#34288=VERTEX_POINT ( 'NONE', #2357 ) ;
#34289=EDGE_CURVE ( 'NONE', #5802, #16616, #48828, .T. ) ;
#34291=CARTESIAN_POINT ( 'NONE',  ( 37.00000000000000711, -0.7008968033239626472, -12.16632754454236576 ) ) ;
#34292=EDGE_CURVE ( 'NONE', #7657, #34943, #33159, .T. ) ;
#34294=FACE_OUTER_BOUND ( 'NONE', #52801, .T. ) ;
#34295=EDGE_CURVE ( 'NONE', #9113, #2944, #42893, .T. ) ;
#34298=DIRECTION ( 'NONE',  ( -1.000000000000000000, 0.000000000000000000, 0.000000000000000000 ) ) ;
#34299=CIRCLE ( 'NONE', #7783, 12.74999999999999822 ) ;
#34300=AXIS2_PLACEMENT_3D ( 'NONE', #7856, #43398, #64342 ) ;
#34301=VECTOR ( 'NONE', #1770, 1000.000000000000000 ) ;
#34302=AXIS2_PLACEMENT_3D ( 'NONE', #61533, #25987, #20970 ) ;
#34303=ORIENTED_EDGE ( 'NONE', *, *, #7068, .T. ) ;
#34304=CARTESIAN_POINT ( 'NONE',  ( 9.575800908719084958, -11.95193887484098028, -1.072919909436247154 ) ) ;
#34305=ORIENTED_EDGE ( 'NONE', *, *, #63405, .F. ) ;
#34306=PLANE ( 'NONE',  #65019 ) ;
#34309=AXIS2_PLACEMENT_3D ( 'NONE', #13023, #32954, #17364 ) ;
#34311=ORIENTED_EDGE ( 'NONE', *, *, #43880, .F. ) ;
#34315=DIRECTION ( 'NONE',  ( -1.000000000000000000, -0.000000000000000000, 0.000000000000000000 ) ) ;
#34316=ADVANCED_FACE ( 'NONE', ( #7659 ), #27942, .F. ) ;
#34320=ORIENTED_EDGE ( 'NONE', *, *, #23042, .F. ) ;
#34323=CARTESIAN_POINT ( 'NONE',  ( 145.1370849898475797, 3.309064568108273190E-14, 0.000000000000000000 ) ) ;
#34326=VERTEX_POINT ( 'NONE', #54195 ) ;
#34327=CARTESIAN_POINT ( 'NONE',  ( -37.00000000000000711, 0.000000000000000000, 0.000000000000000000 ) ) ;
#34329=LINE ( 'NONE', #54643, #16483 ) ;
#34330=CARTESIAN_POINT ( 'NONE',  ( -27.01437459610461644, -11.79277645698183186, -2.220455681983952267 ) ) ;
#34333=CARTESIAN_POINT ( 'NONE',  ( 35.00000000000000000, 4.400442035670942609, -11.96656215839370674 ) ) ;
#34334=EDGE_LOOP ( 'NONE', ( #6, #37916, #11801, #44315 ) ) ;
#34336=VERTEX_POINT ( 'NONE', #8968 ) ;
#34340=CYLINDRICAL_SURFACE ( 'NONE', #44992, 4.999999999999999112 ) ;
#34341=VECTOR ( 'NONE', #53233, 1000.000000000000000 ) ;
#34342=PLANE ( 'NONE',  #6007 ) ;
#34343=CARTESIAN_POINT ( 'NONE',  ( -35.00000000000000000, -10.14433819232429812, -6.753013023069823539 ) ) ;
#34344=LINE ( 'NONE', #24703, #51357 ) ;
#34345=DIRECTION ( 'NONE',  ( 0.000000000000000000, 0.9105187689795969375, -0.4134677391718481476 ) ) ;
#34348=CARTESIAN_POINT ( 'NONE',  ( -36.00000000000000711, 6.265926637539496191, 11.10408318471061762 ) ) ;
#34349=ORIENTED_EDGE ( 'NONE', *, *, #31940, .F. ) ;
#34350=CIRCLE ( 'NONE', #47138, 5.000000000000001776 ) ;
#34351=ORIENTED_EDGE ( 'NONE', *, *, #3136, .F. ) ;
#34352=DIRECTION ( 'NONE',  ( 0.000000000000000000, 0.01356324068817992175, -0.9999080150203990547 ) ) ;
#34353=AXIS2_PLACEMENT_3D ( 'NONE', #65633, #503, #15442 ) ;
#34354=CARTESIAN_POINT ( 'NONE',  ( -35.00000000000000000, -11.95840593935199792, -2.346765782874564277 ) ) ;
#34357=DIRECTION ( 'NONE',  ( 0.000000000000000000, -0.01356324068817992175, 0.9999080150203990547 ) ) ;
#34365=CIRCLE ( 'NONE', #1501, 12.74999999999999822 ) ;
#34367=CARTESIAN_POINT ( 'NONE',  ( -17.54726996257253191, 25.00000000000000000, 3.865003848717349033 ) ) ;
#34369=CIRCLE ( 'NONE', #56708, 12.18650000000000055 ) ;
#34372=AXIS2_PLACEMENT_3D ( 'NONE', #54639, #4413, #45602 ) ;
#34373=LINE ( 'NONE', #3155, #45802 ) ;
#34375=DIRECTION ( 'NONE',  ( 1.000000000000000000, 0.000000000000000000, 0.000000000000000000 ) ) ;
#34376=ADVANCED_FACE ( 'NONE', ( #55499 ), #18643, .T. ) ;
#34377=VERTEX_POINT ( 'NONE', #64794 ) ;
#34378=DIRECTION ( 'NONE',  ( -1.000000000000000000, 0.000000000000000000, 0.000000000000000000 ) ) ;
#34380=DIRECTION ( 'NONE',  ( -1.000000000000000000, 0.000000000000000000, 0.000000000000000000 ) ) ;
#34381=ADVANCED_FACE ( 'NONE', ( #8638 ), #13933, .T. ) ;
#34382=VECTOR ( 'NONE', #60173, 1000.000000000000000 ) ;
#34383=DIRECTION ( 'NONE',  ( -0.000000000000000000, -1.000000000000000000, -0.000000000000000000 ) ) ;
#34384=CARTESIAN_POINT ( 'NONE',  ( -35.00000000000000000, 12.12087942037211263, -1.262958560998631796 ) ) ;
#34385=VERTEX_POINT ( 'NONE', #59843 ) ;
#34387=CARTESIAN_POINT ( 'NONE',  ( -8.292599671964985930, -6.469860207350497383, -10.13661589866336321 ) ) ;
#34388=B_SPLINE_CURVE_WITH_KNOTS ( 'NONE', 3,
 ( #31361, #35994, #7071, #56294, #26058, #46337, #61953, #61602, #46652, #46994, #51340, #1106, #6425, #51665, #1452, #56653, #6108, #777, #52321, #26367 ),
 .UNSPECIFIED., .F., .F.,
 ( 4, 2, 2, 2, 2, 2, 2, 2, 2, 4 ),
 ( 0.000000000000000000, 0.0007149072710670309949, 0.001429814542134061990, 0.001787268177667585348, 0.002144721813201108922, 0.002859629084268155638, 0.003574536355335202354, 0.004289443626402249070, 0.005004350897469296219, 0.005719258168536343369 ),
 .UNSPECIFIED. ) ;
#34389=DIRECTION ( 'NONE',  ( 0.5417962735734935809, -0.000000000000000000, 0.8405098440481683086 ) ) ;
#34390=ORIENTED_EDGE ( 'NONE', *, *, #21629, .F. ) ;
#34391=CARTESIAN_POINT ( 'NONE',  ( 21.90174657591892071, 13.47998113580524659, -0.7349207973210680755 ) ) ;
#34392=DIRECTION ( 'NONE',  ( 1.000000000000000000, 0.000000000000000000, 0.000000000000000000 ) ) ;
#34394=AXIS2_PLACEMENT_3D ( 'NONE', #21955, #1998, #42529 ) ;
#34395=CIRCLE ( 'NONE', #24866, 5.000000000000000888 ) ;
#34396=ORIENTED_EDGE ( 'NONE', *, *, #56355, .F. ) ;
#34397=DIRECTION ( 'NONE',  ( 1.000000000000000000, 0.000000000000000000, 0.000000000000000000 ) ) ;
#34398=EDGE_CURVE ( 'NONE', #63878, #19813, #22269, .T. ) ;
#34399=VECTOR ( 'NONE', #33974, 1000.000000000000000 ) ;
#34400=ORIENTED_EDGE ( 'NONE', *, *, #36672, .F. ) ;
#34401=EDGE_CURVE ( 'NONE', #46319, #43456, #57496, .T. ) ;
#34402=CARTESIAN_POINT ( 'NONE',  ( 19.28625800530496903, 6.413918128308424116, 11.87904264843580471 ) ) ;
#34403=CARTESIAN_POINT ( 'NONE',  ( 22.88594695219327235, 3.421158645304719137, -11.50198563395279194 ) ) ;
#34407=CARTESIAN_POINT ( 'NONE',  ( -37.00000000000000711, 0.000000000000000000, 0.000000000000000000 ) ) ;
#34408=DIRECTION ( 'NONE',  ( -0.000000000000000000, -0.000000000000000000, -1.000000000000000000 ) ) ;
#34409=EDGE_LOOP ( 'NONE', ( #20513, #64435, #40435, #41047 ) ) ;
#34410=EDGE_CURVE ( 'NONE', #17490, #19103, #59441, .T. ) ;
#34411=CARTESIAN_POINT ( 'NONE',  ( -29.43980975494970309, -3.641506875706030488, 25.00000000000000000 ) ) ;
#34413=FACE_OUTER_BOUND ( 'NONE', #11951, .T. ) ;
#34416=EDGE_LOOP ( 'NONE', ( #32133, #16760, #6532, #2272 ) ) ;
#34417=CARTESIAN_POINT ( 'NONE',  ( -25.13721231563192759, 11.42414658719028253, 7.194720236206205044 ) ) ;
#34419=VECTOR ( 'NONE', #18059, 1000.000000000000000 ) ;
#34420=PLANE ( 'NONE',  #22640 ) ;
#34426=CARTESIAN_POINT ( 'NONE',  ( -35.00000000000000000, -1.457575200925636416, 12.66641127287625324 ) ) ;
#34431=LINE ( 'NONE', #3210, #21446 ) ;
#34432=CARTESIAN_POINT ( 'NONE',  ( -37.00000000000000711, -7.376655759824951808, 9.700295462048636352 ) ) ;
#34434=AXIS2_PLACEMENT_3D ( 'NONE', #56952, #37294, #1081 ) ;
#34435=B_SPLINE_CURVE_WITH_KNOTS ( 'NONE', 3,
 ( #56206, #5358, #5701, #51899, #46564, #6340, #35599, #55894, #1022, #10325, #30601, #20955, #10645, #45920, #46256, #700, #41234, #61517, #15958, #36247 ),
 .UNSPECIFIED., .F., .F.,
 ( 4, 2, 2, 2, 2, 2, 2, 2, 2, 4 ),
 ( 0.000000000000000000, 0.001108655026528466330, 0.002217310053056931792, 0.003325965079585397905, 0.003880292592849631395, 0.004434620106113865319, 0.005543275132642328830, 0.006651930159170793208, 0.007760585185699257586, 0.008869240212227721964 ),
 .UNSPECIFIED. ) ;
#34439=ORIENTED_EDGE ( 'NONE', *, *, #33599, .T. ) ;
#34440=DIRECTION ( 'NONE',  ( 0.000000000000000000, -0.01356324068817999114, 0.9999080150203989437 ) ) ;
#34442=DIRECTION ( 'NONE',  ( 1.000000000000000000, 0.000000000000000000, -0.000000000000000000 ) ) ;
#34443=AXIS2_PLACEMENT_3D ( 'NONE', #26786, #47082, #57718 ) ;
#34444=CARTESIAN_POINT ( 'NONE',  ( -35.00000000000000000, -11.72195762423409349, -0.7536123767499773862 ) ) ;
#34445=CARTESIAN_POINT ( 'NONE',  ( -35.00000000000000000, -8.258652103341496797, 8.352657516904644197 ) ) ;
#34447=CARTESIAN_POINT ( 'NONE',  ( 37.00000000000000711, 4.705694406421931860E-17, -3.469127814946512892E-15 ) ) ;
#34448=CARTESIAN_POINT ( 'NONE',  ( -10.90165637462999904, -7.508992741355383416, -9.360289953322597611 ) ) ;
#34451=CARTESIAN_POINT ( 'NONE',  ( 37.00000000000000711, 4.705694406421931860E-17, -3.469127814946512892E-15 ) ) ;
#34452=EDGE_CURVE ( 'NONE', #55405, #40269, #65647, .T. ) ;
#34457=EDGE_CURVE ( 'NONE', #18427, #29901, #7401, .T. ) ;
#34458=AXIS2_PLACEMENT_3D ( 'NONE', #35461, #50454, #234 ) ;
#34459=AXIS2_PLACEMENT_3D ( 'NONE', #50889, #56537, #5339 ) ;
#34460=CARTESIAN_POINT ( 'NONE',  ( -18.08686583997218378, 5.151216734910788908, 25.00000000000000000 ) ) ;
#34461=DIRECTION ( 'NONE',  ( 0.000000000000000000, 0.01356324068817998940, -0.9999080150203989437 ) ) ;
#34462=ORIENTED_EDGE ( 'NONE', *, *, #28751, .F. ) ;
#34464=DIRECTION ( 'NONE',  ( -1.000000000000000000, 0.000000000000000000, 0.000000000000000000 ) ) ;
#34466=VERTEX_POINT ( 'NONE', #16244 ) ;
#34468=CARTESIAN_POINT ( 'NONE',  ( -28.13926220603491402, -11.82994279791709857, -6.511265657020829600 ) ) ;
#34471=DIRECTION ( 'NONE',  ( 0.000000000000000000, 0.01356324068817992175, -0.9999080150203990547 ) ) ;
#34472=EDGE_CURVE ( 'NONE', #3310, #51818, #6610, .T. ) ;
#34473=VECTOR ( 'NONE', #27733, 1000.000000000000000 ) ;
#34476=LINE ( 'NONE', #54777, #25914 ) ;
#34478=CARTESIAN_POINT ( 'NONE',  ( -18.43671985620534315, 6.169215440633483816, -12.01111733792950176 ) ) ;
#34482=CYLINDRICAL_SURFACE ( 'NONE', #31289, 4.999999999999999112 ) ;
#34484=ORIENTED_EDGE ( 'NONE', *, *, #16136, .T. ) ;
#34487=ORIENTED_EDGE ( 'NONE', *, *, #52274, .T. ) ;
#34488=EDGE_CURVE ( 'NONE', #45697, #56806, #1295, .T. ) ;
#34489=CARTESIAN_POINT ( 'NONE',  ( -35.00000000000000000, -12.74613886779085092, 0.3137578094508798321 ) ) ;
#34493=CIRCLE ( 'NONE', #5862, 12.18650000000000055 ) ;
#34499=AXIS2_PLACEMENT_3D ( 'NONE', #63528, #54575, #7697 ) ;
#34500=DIRECTION ( 'NONE',  ( 0.000000000000000000, -0.9467777615094536969, -0.3218879778916073908 ) ) ;
#34501=ORIENTED_EDGE ( 'NONE', *, *, #60195, .T. ) ;
#34502=DIRECTION ( 'NONE',  ( 0.000000000000000000, 0.8009703041134147439, 0.5987040770935704304 ) ) ;
#34503=EDGE_LOOP ( 'NONE', ( #62076, #48128, #46209, #11662 ) ) ;
#34504=FACE_OUTER_BOUND ( 'NONE', #52581, .T. ) ;
#34505=AXIS2_PLACEMENT_3D ( 'NONE', #5067, #4756, #39968 ) ;
#34506=CARTESIAN_POINT ( 'NONE',  ( -4.806344283790351390, -7.508992741355383416, 25.00000000000000000 ) ) ;
#34509=B_SPLINE_CURVE_WITH_KNOTS ( 'NONE', 3,
 ( #35931, #19367, #55914, #39634, #65232, #40948, #20007, #50612, #44953, #61228, #9690, #29980, #60563, #35287, #5053, #46589, #32270, #31608, #31931, #26307 ),
 .UNSPECIFIED., .F., .F.,
 ( 4, 2, 2, 2, 2, 2, 2, 2, 2, 4 ),
 ( 5.553824967135426632E-18, 0.002960076713079371011, 0.004440115069619054999, 0.005920153426158738554, 0.006660172604428579030, 0.007400191782698420373, 0.008140210960968261716, 0.008880230139238104795, 0.01036026849577778401, 0.01184030685231746323 ),
 .UNSPECIFIED. ) ;
#34512=ORIENTED_EDGE ( 'NONE', *, *, #48071, .T. ) ;
#34513=CARTESIAN_POINT ( 'NONE',  ( -19.69476066079020171, -4.201994156881551312, -11.24025111398909615 ) ) ;
#34515=ADVANCED_FACE ( 'NONE', ( #46827 ), #20239, .T. ) ;
#34517=DIRECTION ( 'NONE',  ( 0.000000000000000000, -0.8369827122275287357, -0.5472293298355360713 ) ) ;
#34519=CARTESIAN_POINT ( 'NONE',  ( 23.11060965093502162, -3.962616607205078356, 12.90843863291130411 ) ) ;
#34521=DIRECTION ( 'NONE',  ( 1.000000000000000000, 0.000000000000000000, 0.000000000000000000 ) ) ;
#34522=DIRECTION ( 'NONE',  ( 0.000000000000000000, 0.1740410799127612429, 0.9847383929261617208 ) ) ;
#34524=EDGE_CURVE ( 'NONE', #16616, #12178, #40339, .T. ) ;
#34526=ORIENTED_EDGE ( 'NONE', *, *, #10893, .F. ) ;
#34527=CARTESIAN_POINT ( 'NONE',  ( 35.00000000000000000, -11.72397916322011824, 0.7214809346829776926 ) ) ;
#34528=CARTESIAN_POINT ( 'NONE',  ( 37.00000000000000711, 11.44858830469736333, -2.627174906297124135 ) ) ;
#34531=DIRECTION ( 'NONE',  ( -1.000000000000000000, 0.000000000000000000, 0.000000000000000000 ) ) ;
#34533=ORIENTED_EDGE ( 'NONE', *, *, #37503, .T. ) ;
#34535=CARTESIAN_POINT ( 'NONE',  ( -30.18541646480307961, -1.416020129149133888, -11.91616074890920807 ) ) ;
#34536=CYLINDRICAL_SURFACE ( 'NONE', #23760, 4.999999999999999112 ) ;
#34537=CARTESIAN_POINT ( 'NONE',  ( 37.00000000000000711, 11.24036214326529048, 6.018036132182037257 ) ) ;
#34540=VERTEX_POINT ( 'NONE', #5288 ) ;
#34542=ORIENTED_EDGE ( 'NONE', *, *, #35161, .F. ) ;
#34545=DIRECTION ( 'NONE',  ( 0.000000000000000000, 0.01356324068817998940, -0.9999080150203990547 ) ) ;
#34546=CARTESIAN_POINT ( 'NONE',  ( 47.00000000000000711, 4.705694406421931860E-17, -3.469127814946512892E-15 ) ) ;
#34547=AXIS2_PLACEMENT_3D ( 'NONE', #1055, #21984, #17333 ) ;
#34548=ORIENTED_EDGE ( 'NONE', *, *, #33029, .F. ) ;
#34550=CARTESIAN_POINT ( 'NONE',  ( -27.25055598261694811, 10.68287079889101321, 5.469009518302880402 ) ) ;
#34551=DIRECTION ( 'NONE',  ( 0.000000000000000000, 0.1118654143051546757, 0.9937233664769770103 ) ) ;
#34552=( BOUNDED_CURVE ( )  B_SPLINE_CURVE ( 3, ( #56487, #642, #10933, #26230 ),
 .UNSPECIFIED., .F., .F. ) 
 B_SPLINE_CURVE_WITH_KNOTS ( ( 4, 4 ),
 ( 1.825784944079407834, 1.859903487831931601 ),
 .UNSPECIFIED. ) 
 CURVE ( )  GEOMETRIC_REPRESENTATION_ITEM ( )  RATIONAL_B_SPLINE_CURVE ( ( 1.000000000000000000, 0.9999029961002143807, 0.9999029961002143807, 1.000000000000000000 ) ) 
 REPRESENTATION_ITEM ( '' )  );
#34557=DIRECTION ( 'NONE',  ( 1.000000000000000000, 0.000000000000000000, 0.000000000000000000 ) ) ;
#34559=EDGE_LOOP ( 'NONE', ( #32434, #30528, #1747, #54914 ) ) ;
#34561=ORIENTED_EDGE ( 'NONE', *, *, #8248, .F. ) ;
#34563=AXIS2_PLACEMENT_3D ( 'NONE', #48947, #22689, #32959 ) ;
#34564=CARTESIAN_POINT ( 'NONE',  ( -36.00000000000000711, 6.950793414699792727, 10.68873102412845277 ) ) ;
#34566=FACE_OUTER_BOUND ( 'NONE', #59144, .T. ) ;
#34567=VERTEX_POINT ( 'NONE', #26223 ) ;
#34568=CARTESIAN_POINT ( 'NONE',  ( -14.29135464769095520, 7.782112657557433089, 25.00000000000000000 ) ) ;
#34569=DIRECTION ( 'NONE',  ( -1.000000000000000000, 0.000000000000000000, -0.000000000000000000 ) ) ;
#34571=ORIENTED_EDGE ( 'NONE', *, *, #27310, .T. ) ;
#34572=ORIENTED_EDGE ( 'NONE', *, *, #36121, .F. ) ;
#34574=VERTEX_POINT ( 'NONE', #56139 ) ;
#34575=DIRECTION ( 'NONE',  ( 0.000000000000000000, 0.4935949184179261873, -0.8696919319575183716 ) ) ;
#34577=ORIENTED_EDGE ( 'NONE', *, *, #18344, .T. ) ;
#34579=DIRECTION ( 'NONE',  ( 1.000000000000000000, 0.000000000000000000, 0.000000000000000000 ) ) ;
#34580=CARTESIAN_POINT ( 'NONE',  ( -35.00000000000000000, 2.185196060783882288, 11.54110654723649709 ) ) ;
#34584=VERTEX_POINT ( 'NONE', #48482 ) ;
#34588=DIRECTION ( 'NONE',  ( 1.000000000000000000, 0.000000000000000000, 0.000000000000000000 ) ) ;
#34589=EDGE_CURVE ( 'NONE', #17286, #743, #61604, .T. ) ;
#34590=CYLINDRICAL_SURFACE ( 'NONE', #58510, 12.18650000000000055 ) ;
#34594=DIRECTION ( 'NONE',  ( 0.000000000000000000, 0.01356324068818000848, -0.9999080150203990547 ) ) ;
#34596=ORIENTED_EDGE ( 'NONE', *, *, #36722, .F. ) ;
#34598=ORIENTED_EDGE ( 'NONE', *, *, #40602, .T. ) ;
#34601=ORIENTED_EDGE ( 'NONE', *, *, #222, .T. ) ;
#34602=ADVANCED_FACE ( 'NONE', ( #58126, #17884 ), #38486, .F. ) ;
#34603=CARTESIAN_POINT ( 'NONE',  ( 35.00000000000000000, 4.705694406421931860E-17, -3.469127814946512892E-15 ) ) ;
#34604=DIRECTION ( 'NONE',  ( 0.000000000000000000, -0.1740410799127470598, -0.9847383929261643853 ) ) ;
#34605=CYLINDRICAL_SURFACE ( 'NONE', #13312, 12.75000000000000178 ) ;
#34606=CARTESIAN_POINT ( 'NONE',  ( -3.517042058461139042, 9.903124696108923430, 6.789431062153663099 ) ) ;
#34607=CARTESIAN_POINT ( 'NONE',  ( 9.687175622948609899, 11.98570860552671391, -0.5854820436212360146 ) ) ;
#34609=DIRECTION ( 'NONE',  ( -1.000000000000000000, 0.000000000000000000, 0.000000000000000000 ) ) ;
#34610=CARTESIAN_POINT ( 'NONE',  ( -29.92777678363736626, -3.750539801530011985, 12.96855624952674724 ) ) ;
#34613=EDGE_CURVE ( 'NONE', #53149, #27041, #32173, .T. ) ;
#34616=DIRECTION ( 'NONE',  ( 0.000000000000000000, -0.01356324068817998940, 0.9999080150203990547 ) ) ;
#34617=VECTOR ( 'NONE', #50316, 1000.000000000000000 ) ;
#34618=ORIENTED_EDGE ( 'NONE', *, *, #39709, .T. ) ;
#34619=CARTESIAN_POINT ( 'NONE',  ( 35.00000000000000000, -0.4993900848168272288, -12.17626345777663488 ) ) ;
#34620=AXIS2_PLACEMENT_3D ( 'NONE', #22347, #32635, #31994 ) ;
#34624=DIRECTION ( 'NONE',  ( 0.000000000000000000, 0.01356324068817998940, -0.9999080150203989437 ) ) ;
#34626=VERTEX_POINT ( 'NONE', #2931 ) ;
#34628=EDGE_LOOP ( 'NONE', ( #52987, #59938, #41773, #1962 ) ) ;
#34629=ORIENTED_EDGE ( 'NONE', *, *, #31405, .T. ) ;
#34633=ORIENTED_EDGE ( 'NONE', *, *, #694, .T. ) ;
#34634=DIRECTION ( 'NONE',  ( 0.000000000000000000, 0.01356324068817992175, -0.9999080150203990547 ) ) ;
#34635=CARTESIAN_POINT ( 'NONE',  ( -37.00000000000000711, 0.000000000000000000, 0.000000000000000000 ) ) ;
#34636=DIRECTION ( 'NONE',  ( -0.000000000000000000, -1.000000000000000000, -0.000000000000000000 ) ) ;
#34637=ORIENTED_EDGE ( 'NONE', *, *, #52209, .F. ) ;
#34638=CARTESIAN_POINT ( 'NONE',  ( 36.00000000000000711, 9.076753354953998709, -8.954052073409638268 ) ) ;
#34640=FACE_OUTER_BOUND ( 'NONE', #32819, .T. ) ;
#34642=ORIENTED_EDGE ( 'NONE', *, *, #10514, .T. ) ;
#34645=CARTESIAN_POINT ( 'NONE',  ( 37.00000000000000711, 12.01765980939841860, -2.021542716731445921 ) ) ;
#34646=ADVANCED_FACE ( 'NONE', ( #53476 ), #18216, .T. ) ;
#34647=ORIENTED_EDGE ( 'NONE', *, *, #26864, .T. ) ;
#34648=DIRECTION ( 'NONE',  ( -0.7290028908350527637, 0.000000000000000000, 0.6845106172691086677 ) ) ;
#34649=CARTESIAN_POINT ( 'NONE',  ( 12.73158684737537349, -11.67291052772676885, -2.789930929895412248 ) ) ;
#34650=CARTESIAN_POINT ( 'NONE',  ( -37.00000000000000711, 11.35427606708812753, -4.426194442447118682 ) ) ;
#34651=DIRECTION ( 'NONE',  ( -1.000000000000000000, 0.000000000000000000, 0.000000000000000000 ) ) ;
#34652=FACE_OUTER_BOUND ( 'NONE', #49404, .T. ) ;
#34657=ORIENTED_EDGE ( 'NONE', *, *, #9356, .F. ) ;
#34658=EDGE_LOOP ( 'NONE', ( #11068, #1779, #58040, #52159 ) ) ;
#34659=CARTESIAN_POINT ( 'NONE',  ( 36.00000000000000711, -11.01837265713068703, 6.415447294506815723 ) ) ;
#34660=ORIENTED_EDGE ( 'NONE', *, *, #64560, .T. ) ;
#34662=ORIENTED_EDGE ( 'NONE', *, *, #2765, .T. ) ;
#34663=CYLINDRICAL_SURFACE ( 'NONE', #59333, 4.999999999999999112 ) ;
#34666=VECTOR ( 'NONE', #32118, 1000.000000000000000 ) ;
#34670=AXIS2_PLACEMENT_3D ( 'NONE', #15006, #25012, #44957 ) ;
#34672=VERTEX_POINT ( 'NONE', #13842 ) ;
#34676=CARTESIAN_POINT ( 'NONE',  ( -17.87652388884287191, -5.106857196458570947, 12.49754165357240510 ) ) ;
#34677=EDGE_CURVE ( 'NONE', #47206, #1585, #53130, .T. ) ;
#34678=EDGE_LOOP ( 'NONE', ( #30674, #36877, #36056, #53052 ) ) ;
#34680=EDGE_CURVE ( 'NONE', #22627, #26468, #14, .T. ) ;
#34683=CARTESIAN_POINT ( 'NONE',  ( -2.532614230583022152, 25.00000000000000000, 4.026315189028233377 ) ) ;
#34684=DIRECTION ( 'NONE',  ( -1.000000000000000000, 0.000000000000000000, 0.000000000000000000 ) ) ;
#34685=ORIENTED_EDGE ( 'NONE', *, *, #41921, .F. ) ;
#34687=CARTESIAN_POINT ( 'NONE',  ( 37.00000000000000711, -0.4993900848168272288, -12.17626345777663666 ) ) ;
#34688=CARTESIAN_POINT ( 'NONE',  ( 3.959660738498543608, 6.970283272837293431, 9.778486319596556342 ) ) ;
#34689=DIRECTION ( 'NONE',  ( 1.000000000000000000, 0.000000000000000000, 0.000000000000000000 ) ) ;
#34690=DIRECTION ( 'NONE',  ( 1.000000000000000000, 0.000000000000000000, 0.000000000000000000 ) ) ;
#34695=LINE ( 'NONE', #3012, #21221 ) ;
#34697=DIRECTION ( 'NONE',  ( 0.000000000000000000, 0.8696919319575167062, 0.4935949184179292404 ) ) ;
#34698=LINE ( 'NONE', #50023, #44675 ) ;
#34699=ORIENTED_EDGE ( 'NONE', *, *, #46551, .T. ) ;
#34701=EDGE_LOOP ( 'NONE', ( #52710, #59632, #36008, #4781 ) ) ;
#34702=CARTESIAN_POINT ( 'NONE',  ( -35.00000000000000000, -1.171570255487366152, -11.68758509253249400 ) ) ;
#34703=ADVANCED_FACE ( 'NONE', ( #49776 ), #60080, .T. ) ;
#34704=AXIS2_PLACEMENT_3D ( 'NONE', #30963, #41262, #30628 ) ;
#34707=CARTESIAN_POINT ( 'NONE',  ( -19.47984447937493613, -1.416020129149132334, 25.00000000000000000 ) ) ;
#34711=LINE ( 'NONE', #49075, #59975 ) ;
#34713=EDGE_LOOP ( 'NONE', ( #53444, #37834, #61196, #1463 ) ) ;
#34714=CARTESIAN_POINT ( 'NONE',  ( 35.00000000000000000, 5.391785509271111110, 10.43555801961468887 ) ) ;
#34715=ORIENTED_EDGE ( 'NONE', *, *, #34046, .F. ) ;
#34716=CARTESIAN_POINT ( 'NONE',  ( 35.00000000000000000, -7.215058775251181444, 9.821084925794645315 ) ) ;
#34717=VERTEX_POINT ( 'NONE', #60394 ) ;
#34718=EDGE_CURVE ( 'NONE', #53581, #7512, #12764, .T. ) ;
#34719=ORIENTED_EDGE ( 'NONE', *, *, #36737, .F. ) ;
#34724=DIRECTION ( 'NONE',  ( -1.000000000000000000, -0.000000000000000000, 0.000000000000000000 ) ) ;
#34726=VERTEX_POINT ( 'NONE', #28500 ) ;
#34728=ORIENTED_EDGE ( 'NONE', *, *, #24430, .T. ) ;
#34731=EDGE_CURVE ( 'NONE', #53501, #32268, #32941, .T. ) ;
#34732=ORIENTED_EDGE ( 'NONE', *, *, #22826, .F. ) ;
#34738=CARTESIAN_POINT ( 'NONE',  ( 8.937200413559443390, 4.476360154859203355, 25.00000000000000000 ) ) ;
#34739=LINE ( 'NONE', #4183, #7907 ) ;
#34743=FACE_OUTER_BOUND ( 'NONE', #36304, .T. ) ;
#34745=LINE ( 'NONE', #64679, #44656 ) ;
#34746=EDGE_CURVE ( 'NONE', #35130, #47761, #21276, .T. ) ;
#34747=ORIENTED_EDGE ( 'NONE', *, *, #33623, .T. ) ;
#34748=CARTESIAN_POINT ( 'NONE',  ( -27.74314290831961927, 13.27105638519637054, -2.536820231170034301 ) ) ;
#34749=AXIS2_PLACEMENT_3D ( 'NONE', #35467, #38917, #13624 ) ;
#34750=EDGE_CURVE ( 'NONE', #35169, #52094, #13806, .T. ) ;
#34752=DIRECTION ( 'NONE',  ( 1.000000000000000000, 0.000000000000000000, 0.000000000000000000 ) ) ;
#34753=EDGE_CURVE ( 'NONE', #29901, #37187, #8230, .T. ) ;
#34755=DIRECTION ( 'NONE',  ( 1.000000000000000000, 0.000000000000000000, 0.000000000000000000 ) ) ;
#34756=ORIENTED_EDGE ( 'NONE', *, *, #5950, .F. ) ;
#34759=DIRECTION ( 'NONE',  ( 1.000000000000000000, 0.000000000000000000, 0.000000000000000000 ) ) ;
#34761=DIRECTION ( 'NONE',  ( -0.8214942970785323872, -0.5702167306099040767, 0.000000000000000000 ) ) ;
#34762=CARTESIAN_POINT ( 'NONE',  ( 3.291290029914074378, 8.250315036047103590, 10.68561190601527855 ) ) ;
#34765=LINE ( 'NONE', #45750, #4670 ) ;
#34767=ORIENTED_EDGE ( 'NONE', *, *, #25523, .T. ) ;
#34768=LINE ( 'NONE', #20490, #49343 ) ;
#34772=CARTESIAN_POINT ( 'NONE',  ( -9.764253471131736362, -12.49999450231236153, -5.102826708558637847 ) ) ;
#34773=CIRCLE ( 'NONE', #61366, 12.18650000000000055 ) ;
#34774=DIRECTION ( 'NONE',  ( 0.000000000000000000, -0.2618041379715704275, 0.9651210252299774472 ) ) ;
#34777=EDGE_CURVE ( 'NONE', #16609, #63997, #45116, .T. ) ;
#34778=LINE ( 'NONE', #61068, #37242 ) ;
#34779=VECTOR ( 'NONE', #22333, 1000.000000000000000 ) ;
#34781=DIRECTION ( 'NONE',  ( -1.000000000000000000, 0.000000000000000000, -0.000000000000000000 ) ) ;
#34784=DIRECTION ( 'NONE',  ( 0.000000000000000000, 0.7790879021242484992, -0.6269146997508012742 ) ) ;
#34786=ORIENTED_EDGE ( 'NONE', *, *, #8748, .F. ) ;
#34787=ORIENTED_EDGE ( 'NONE', *, *, #22453, .F. ) ;
#34788=DIRECTION ( 'NONE',  ( 0.000000000000000000, -0.9346839223284501008, 0.3554799084909069928 ) ) ;
#34790=EDGE_CURVE ( 'NONE', #38454, #22430, #49951, .T. ) ;
#34791=CIRCLE ( 'NONE', #41160, 12.74999999999999822 ) ;
#34793=VECTOR ( 'NONE', #59779, 1000.000000000000000 ) ;
#34794=CARTESIAN_POINT ( 'NONE',  ( 35.00000000000000000, -11.07407352312215387, -3.916263239775311433 ) ) ;
#34795=VERTEX_POINT ( 'NONE', #56059 ) ;
#34796=CARTESIAN_POINT ( 'NONE',  ( -35.00000000000000000, 0.000000000000000000, 0.000000000000000000 ) ) ;
#34797=CARTESIAN_POINT ( 'NONE',  ( 35.00000000000000000, -12.21925492305364536, -3.640372113593510761 ) ) ;
#34798=CARTESIAN_POINT ( 'NONE',  ( 23.48675979904455957, 2.894400836696811918, 13.18980151006969415 ) ) ;
#34799=VERTEX_POINT ( 'NONE', #46113 ) ;
#34802=EDGE_CURVE ( 'NONE', #3877, #53943, #62050, .T. ) ;
#34804=ORIENTED_EDGE ( 'NONE', *, *, #34122, .T. ) ;
#34805=CARTESIAN_POINT ( 'NONE',  ( -47.00000000000000711, 0.000000000000000000, 0.000000000000000000 ) ) ;
#34807=CARTESIAN_POINT ( 'NONE',  ( 35.00000000000000000, 1.903127969211351189, 11.59095880812005497 ) ) ;
#34808=EDGE_CURVE ( 'NONE', #3067, #45140, #57358, .T. ) ;
#34815=FACE_OUTER_BOUND ( 'NONE', #57646, .T. ) ;
#34816=CARTESIAN_POINT ( 'NONE',  ( 35.00000000000000000, 6.102719229070673990, -10.54834585426222304 ) ) ;
#34817=DIRECTION ( 'NONE',  ( 1.000000000000000000, 0.000000000000000000, -0.000000000000000000 ) ) ;
#34818=CARTESIAN_POINT ( 'NONE',  ( 12.87184510392629200, 12.70280640453755794, -4.586614403938258810 ) ) ;
#34820=DIRECTION ( 'NONE',  ( -1.000000000000000000, -0.000000000000000000, 0.000000000000000000 ) ) ;
#34822=DIRECTION ( 'NONE',  ( -0.000000000000000000, -0.000000000000000000, -1.000000000000000000 ) ) ;
#34824=CIRCLE ( 'NONE', #3025, 5.000000000000000888 ) ;
#34825=ORIENTED_EDGE ( 'NONE', *, *, #4882, .T. ) ;
#34829=DIRECTION ( 'NONE',  ( 0.000000000000000000, 0.2618041379715633776, -0.9651210252299794456 ) ) ;
#34830=DIRECTION ( 'NONE',  ( 1.000000000000000000, 0.000000000000000000, 0.000000000000000000 ) ) ;
#34832=VECTOR ( 'NONE', #10068, 1000.000000000000000 ) ;
#34840=ADVANCED_FACE ( 'NONE', ( #36090 ), #35453, .T. ) ;
#34841=CARTESIAN_POINT ( 'NONE',  ( 36.00000000000000711, -11.90598845858536947, -4.561791185930373693 ) ) ;
#34842=VERTEX_POINT ( 'NONE', #50759 ) ;
#34844=ORIENTED_EDGE ( 'NONE', *, *, #43841, .F. ) ;
#34847=LINE ( 'NONE', #9585, #64971 ) ;
#34849=CIRCLE ( 'NONE', #5182, 5.000000000000000000 ) ;
#34851=ORIENTED_EDGE ( 'NONE', *, *, #47684, .T. ) ;
#34855=FACE_OUTER_BOUND ( 'NONE', #8258, .T. ) ;
#34856=DIRECTION ( 'NONE',  ( 1.000000000000000000, 0.000000000000000000, 0.000000000000000000 ) ) ;
#34859=AXIS2_PLACEMENT_3D ( 'NONE', #62377, #23146, #52759 ) ;
#34860=DIRECTION ( 'NONE',  ( 0.000000000000000000, -0.7790879021242573810, 0.6269146997507903940 ) ) ;
#34861=CARTESIAN_POINT ( 'NONE',  ( 35.00000000000000000, -5.921969905510278132, 10.14408668126219304 ) ) ;
#34862=FACE_OUTER_BOUND ( 'NONE', #42982, .T. ) ;
#34863=ORIENTED_EDGE ( 'NONE', *, *, #32021, .F. ) ;
#34865=ORIENTED_EDGE ( 'NONE', *, *, #5471, .T. ) ;
#34867=FACE_OUTER_BOUND ( 'NONE', #43240, .T. ) ;
#34869=CYLINDRICAL_SURFACE ( 'NONE', #54450, 13.50000000000000178 ) ;
#34871=VERTEX_POINT ( 'NONE', #10841 ) ;
#34875=CIRCLE ( 'NONE', #42276, 12.18649999999999878 ) ;
#34876=CYLINDRICAL_SURFACE ( 'NONE', #58823, 4.999999999999999112 ) ;
#34877=CARTESIAN_POINT ( 'NONE',  ( 3.709820702086316757, -10.52816917254576623, -8.451371970425016755 ) ) ;
#34879=CARTESIAN_POINT ( 'NONE',  ( 5.650485762548542290, -9.979623674447639203, 6.674921982999905801 ) ) ;
#34880=ORIENTED_EDGE ( 'NONE', *, *, #32637, .T. ) ;
#34882=AXIS2_PLACEMENT_3D ( 'NONE', #13651, #64517, #13981 ) ;
#34883=CARTESIAN_POINT ( 'NONE',  ( -47.00000000000000711, 0.000000000000000000, 0.000000000000000000 ) ) ;
#34885=ADVANCED_FACE ( 'NONE', ( #31129 ), #51440, .T. ) ;
#34886=EDGE_CURVE ( 'NONE', #28625, #43866, #7450, .T. ) ;
#34888=EDGE_LOOP ( 'NONE', ( #44143, #15153, #32218, #55686 ) ) ;
#34890=CIRCLE ( 'NONE', #5169, 5.000000000000000888 ) ;
#34891=VERTEX_POINT ( 'NONE', #2531 ) ;
#34892=DIRECTION ( 'NONE',  ( 0.000000000000000000, 0.01356324068817998940, -0.9999080150203990547 ) ) ;
#34899=CARTESIAN_POINT ( 'NONE',  ( 35.00000000000000000, 4.732539170486261604, -11.23004253107766282 ) ) ;
#34900=DIRECTION ( 'NONE',  ( -1.000000000000000000, 0.000000000000000000, 0.000000000000000000 ) ) ;
#34901=ORIENTED_EDGE ( 'NONE', *, *, #58894, .F. ) ;
#34902=CARTESIAN_POINT ( 'NONE',  ( -27.01437459610461644, 10.69338818478080455, -8.240233560378637634 ) ) ;
#34903=CARTESIAN_POINT ( 'NONE',  ( 26.47552525366476672, 11.32202890774585491, 3.984464554639796763 ) ) ;
#34905=AXIS2_PLACEMENT_3D ( 'NONE', #18811, #49087, #38425 ) ;
#34906=ORIENTED_EDGE ( 'NONE', *, *, #26868, .F. ) ;
#34909=ORIENTED_EDGE ( 'NONE', *, *, #19448, .F. ) ;
#34911=CYLINDRICAL_SURFACE ( 'NONE', #59519, 12.75000000000000178 ) ;
#34914=CARTESIAN_POINT ( 'NONE',  ( -37.00000000000000711, -10.59380114696474884, 7.094637218249319588 ) ) ;
#34915=ORIENTED_EDGE ( 'NONE', *, *, #62573, .F. ) ;
#34917=DIRECTION ( 'NONE',  ( -1.000000000000000000, 0.000000000000000000, -0.000000000000000000 ) ) ;
#34920=DIRECTION ( 'NONE',  ( 1.000000000000000000, 0.000000000000000000, 0.000000000000000000 ) ) ;
#34921=VECTOR ( 'NONE', #14496, 1000.000000000000000 ) ;
#34922=ADVANCED_FACE ( 'NONE', ( #47094 ), #36769, .T. ) ;
#34923=CIRCLE ( 'NONE', #3131, 12.75000000000000178 ) ;
#34924=DIRECTION ( 'NONE',  ( 0.000000000000000000, -0.01356324068817991828, 0.9999080150203990547 ) ) ;
#34925=( BOUNDED_CURVE ( )  B_SPLINE_CURVE ( 3, ( #21083, #61649, #16102, #36389 ),
 .UNSPECIFIED., .F., .F. ) 
 B_SPLINE_CURVE_WITH_KNOTS ( ( 4, 4 ),
 ( 3.908502672100578668, 3.937696279019239132 ),
 .UNSPECIFIED. ) 
 CURVE ( )  GEOMETRIC_REPRESENTATION_ITEM ( )  RATIONAL_B_SPLINE_CURVE ( ( 1.000000000000000000, 0.9999289790372866138, 0.9999289790372866138, 1.000000000000000000 ) ) 
 REPRESENTATION_ITEM ( '' )  );
#34928=DIRECTION ( 'NONE',  ( -1.000000000000000000, 0.000000000000000000, 0.000000000000000000 ) ) ;
#34929=DIRECTION ( 'NONE',  ( -1.000000000000000000, 0.000000000000000000, -0.000000000000000000 ) ) ;
#34930=AXIS2_PLACEMENT_3D ( 'NONE', #13425, #23412, #59011 ) ;
#34931=EDGE_CURVE ( 'NONE', #54137, #49507, #55259, .T. ) ;
#34933=DIRECTION ( 'NONE',  ( 0.000000000000000000, 0.9551603052523468529, -0.2960891610144545938 ) ) ;
#34935=ORIENTED_EDGE ( 'NONE', *, *, #17797, .F. ) ;
#34936=CARTESIAN_POINT ( 'NONE',  ( -14.11589373245165469, 8.250315036047107142, -8.713914264323175729 ) ) ;
#34937=CARTESIAN_POINT ( 'NONE',  ( 35.00000000000000000, -6.547236723513950807, 9.752226076388957665 ) ) ;
#34938=CARTESIAN_POINT ( 'NONE',  ( 35.00000000000000000, 4.705694406421931860E-17, -3.469127814946512892E-15 ) ) ;
#34942=ORIENTED_EDGE ( 'NONE', *, *, #21685, .F. ) ;
#34943=VERTEX_POINT ( 'NONE', #31761 ) ;
#34945=CIRCLE ( 'NONE', #8448, 5.000000000000000000 ) ;
#34946=CARTESIAN_POINT ( 'NONE',  ( -35.00000000000000000, 0.000000000000000000, 0.000000000000000000 ) ) ;
#34948=VERTEX_POINT ( 'NONE', #57728 ) ;
#34949=LINE ( 'NONE', #45951, #23881 ) ;
#34950=LINE ( 'NONE', #29986, #18791 ) ;
#34951=CYLINDRICAL_SURFACE ( 'NONE', #42869, 12.75000000000000178 ) ;
#34953=CARTESIAN_POINT ( 'NONE',  ( -27.22222364661110916, -10.76538614228702428, 5.304738902579489768 ) ) ;
#34955=ADVANCED_FACE ( 'NONE', ( #63335, #37084 ), #12149, .F. ) ;
#34958=CARTESIAN_POINT ( 'NONE',  ( 11.86932257037118532, -8.667155996924371664, -8.300945040779890149 ) ) ;
#34959=EDGE_LOOP ( 'NONE', ( #62690, #53973, #36407, #31276 ) ) ;
#34962=DIRECTION ( 'NONE',  ( -1.000000000000000000, 0.000000000000000000, 0.000000000000000000 ) ) ;
#34965=CARTESIAN_POINT ( 'NONE',  ( 13.33826709797422794, -11.16011261617231121, -4.415959474372655791 ) ) ;
#34967=DIRECTION ( 'NONE',  ( 0.000000000000000000, -0.01356324068817998940, 0.9999080150203990547 ) ) ;
#34968=DIRECTION ( 'NONE',  ( 0.000000000000000000, -0.01356324068817991828, 0.9999080150203990547 ) ) ;
#34972=CARTESIAN_POINT ( 'NONE',  ( 37.00000000000000711, 9.217970097227837556, 7.971186206369369032 ) ) ;
#34973=FACE_OUTER_BOUND ( 'NONE', #52364, .T. ) ;
#34974=DIRECTION ( 'NONE',  ( 1.000000000000000000, 0.000000000000000000, -0.000000000000000000 ) ) ;
#34975=VERTEX_POINT ( 'NONE', #27433 ) ;
#34976=EDGE_CURVE ( 'NONE', #6394, #52020, #41475, .T. ) ;
#34977=VECTOR ( 'NONE', #58199, 1000.000000000000000 ) ;
#34978=ORIENTED_EDGE ( 'NONE', *, *, #58580, .T. ) ;
#34979=CARTESIAN_POINT ( 'NONE',  ( 35.00000000000000000, 0.3137578094511070947, 12.74613886779083849 ) ) ;
#34980=ORIENTED_EDGE ( 'NONE', *, *, #29602, .T. ) ;
#34981=ORIENTED_EDGE ( 'NONE', *, *, #16291, .F. ) ;
#34982=CARTESIAN_POINT ( 'NONE',  ( 25.05309951391468459, 8.823569016628493245, -8.132934882857099979 ) ) ;
#34988=DIRECTION ( 'NONE',  ( 1.000000000000000000, 0.000000000000000000, -0.000000000000000000 ) ) ;
#34989=EDGE_LOOP ( 'NONE', ( #15728, #18045, #19217, #14615 ) ) ;
#34991=DIRECTION ( 'NONE',  ( 0.000000000000000000, 0.01356324068817998940, -0.9999080150203990547 ) ) ;
#34992=DIRECTION ( 'NONE',  ( -1.000000000000000000, 0.000000000000000000, 0.000000000000000000 ) ) ;
#34993=ORIENTED_EDGE ( 'NONE', *, *, #42145, .F. ) ;
#34994=EDGE_CURVE ( 'NONE', #12280, #26022, #12460, .T. ) ;
#34995=VECTOR ( 'NONE', #3003, 1000.000000000000000 ) ;
#34996=CIRCLE ( 'NONE', #32913, 12.18650000000000055 ) ;
#34999=CARTESIAN_POINT ( 'NONE',  ( 35.00000000000000000, 4.705694406421931860E-17, -3.469127814946512892E-15 ) ) ;
#35002=CYLINDRICAL_SURFACE ( 'NONE', #57454, 4.999999999999999112 ) ;
#35004=FACE_OUTER_BOUND ( 'NONE', #56542, .T. ) ;
#35005=AXIS2_PLACEMENT_3D ( 'NONE', #42473, #17892, #7582 ) ;
#35006=EDGE_CURVE ( 'NONE', #23475, #4911, #18155, .T. ) ;
#35007=LINE ( 'NONE', #59995, #58639 ) ;
#35008=DIRECTION ( 'NONE',  ( -1.000000000000000000, 0.000000000000000000, -0.000000000000000000 ) ) ;
#35010=ORIENTED_EDGE ( 'NONE', *, *, #3875, .F. ) ;
#35012=CARTESIAN_POINT ( 'NONE',  ( -37.00000000000000711, -11.65150730582933392, -1.488153103997089888 ) ) ;
#35013=CARTESIAN_POINT ( 'NONE',  ( -9.514691729518425234, -11.30278532684398485, -4.051020386293188835 ) ) ;
#35016=LINE ( 'NONE', #130, #9610 ) ;
#35017=DIRECTION ( 'NONE',  ( 1.000000000000000000, 0.000000000000000000, -0.000000000000000000 ) ) ;
#35018=EDGE_CURVE ( 'NONE', #25502, #29592, #35982, .T. ) ;
#35020=VECTOR ( 'NONE', #60418, 1000.000000000000000 ) ;
#35021=VERTEX_POINT ( 'NONE', #51649 ) ;
#35022=ORIENTED_EDGE ( 'NONE', *, *, #47465, .T. ) ;
#35024=LINE ( 'NONE', #36364, #54648 ) ;
#35025=DIRECTION ( 'NONE',  ( 0.000000000000000000, -0.8989688749565204473, -0.4380125133593880671 ) ) ;
#35030=CARTESIAN_POINT ( 'NONE',  ( 24.80306200676344019, -1.716780947678923308, -13.39180189726039316 ) ) ;
#35032=CARTESIAN_POINT ( 'NONE',  ( 47.00000000000000711, 4.705694406421931860E-17, -3.469127814946512892E-15 ) ) ;
#35034=DIRECTION ( 'NONE',  ( 0.9947400562552481951, -0.1024315404614497965, 0.000000000000000000 ) ) ;
#35035=EDGE_CURVE ( 'NONE', #8899, #3390, #54237, .T. ) ;
#35038=ORIENTED_EDGE ( 'NONE', *, *, #27876, .F. ) ;
#35039=ORIENTED_EDGE ( 'NONE', *, *, #43068, .T. ) ;
#35043=CYLINDRICAL_SURFACE ( 'NONE', #53508, 12.75000000000000178 ) ;
#35044=CIRCLE ( 'NONE', #21299, 12.74999999999999822 ) ;
#35045=VECTOR ( 'NONE', #45083, 1000.000000000000000 ) ;
#35046=AXIS2_PLACEMENT_3D ( 'NONE', #35968, #36313, #46312 ) ;
#35048=VECTOR ( 'NONE', #58712, 1000.000000000000000 ) ;
#35049=DIRECTION ( 'NONE',  ( 0.000000000000000000, -0.01356324068817991828, 0.9999080150203990547 ) ) ;
#35052=VERTEX_POINT ( 'NONE', #5106 ) ;
#35054=CARTESIAN_POINT ( 'NONE',  ( -35.00000000000000000, 7.817492529713985228, -9.348667969174325520 ) ) ;
#35056=EDGE_CURVE ( 'NONE', #36640, #39147, #34033, .T. ) ;
#35057=VERTEX_POINT ( 'NONE', #30676 ) ;
#35058=LINE ( 'NONE', #51047, #15740 ) ;
#35059=FACE_OUTER_BOUND ( 'NONE', #15776, .T. ) ;
#35060=CARTESIAN_POINT ( 'NONE',  ( 18.74194725139314954, 1.365073709202341279, 11.92510536682598676 ) ) ;
#35065=AXIS2_PLACEMENT_3D ( 'NONE', #21824, #52412, #17479 ) ;
#35066=EDGE_LOOP ( 'NONE', ( #8025, #2084, #49285, #27591 ) ) ;
#35068=CARTESIAN_POINT ( 'NONE',  ( -37.00000000000000711, 0.000000000000000000, 0.000000000000000000 ) ) ;
#35070=AXIS2_PLACEMENT_3D ( 'NONE', #23891, #24517, #65714 ) ;
#35073=CARTESIAN_POINT ( 'NONE',  ( 6.786836467603172274, -6.651659772632933176, 9.989835789978261715 ) ) ;
#35074=CARTESIAN_POINT ( 'NONE',  ( 3.347841273039249721, -10.61118957148187825, 5.603807266321171987 ) ) ;
#35075=CIRCLE ( 'NONE', #27645, 5.000000000000001776 ) ;
#35076=DIRECTION ( 'NONE',  ( -1.000000000000000000, -0.000000000000000000, 0.000000000000000000 ) ) ;
#35082=DIRECTION ( 'NONE',  ( -1.000000000000000000, 0.000000000000000000, 0.000000000000000000 ) ) ;
#35085=CIRCLE ( 'NONE', #59517, 12.75000000000000178 ) ;
#35087=CIRCLE ( 'NONE', #55293, 4.999999999999998224 ) ;
#35088=EDGE_CURVE ( 'NONE', #22685, #31409, #1094, .T. ) ;
#35090=DIRECTION ( 'NONE',  ( 0.000000000000000000, -0.01356324068817998940, 0.9999080150203990547 ) ) ;
#35091=ORIENTED_EDGE ( 'NONE', *, *, #42781, .F. ) ;
#35093=DIRECTION ( 'NONE',  ( 1.000000000000000000, 0.000000000000000000, 0.000000000000000000 ) ) ;
#35097=CARTESIAN_POINT ( 'NONE',  ( -28.25663979408810889, -12.49293946602661443, -5.125494512094520339 ) ) ;
#35098=DIRECTION ( 'NONE',  ( 0.000000000000000000, 0.01356324068817992175, -0.9999080150203990547 ) ) ;
#35100=FACE_OUTER_BOUND ( 'NONE', #11744, .T. ) ;
#35101=ORIENTED_EDGE ( 'NONE', *, *, #34026, .F. ) ;
#35102=DIRECTION ( 'NONE',  ( 0.000000000000000000, 0.6478160128811893959, -0.7617968321374922747 ) ) ;
#35103=VECTOR ( 'NONE', #12558, 1000.000000000000000 ) ;
#35104=DIRECTION ( 'NONE',  ( 0.000000000000000000, -0.3807014730195286134, 0.9246979985058695339 ) ) ;
#35105=ORIENTED_EDGE ( 'NONE', *, *, #54743, .T. ) ;
#35106=AXIS2_PLACEMENT_3D ( 'NONE', #25128, #10155, #25447 ) ;
#35108=AXIS2_PLACEMENT_3D ( 'NONE', #19051, #49647, #24696 ) ;
#35114=DIRECTION ( 'NONE',  ( 0.000000000000000000, 0.01356324068817998073, -0.9999080150203990547 ) ) ;
#35117=DIRECTION ( 'NONE',  ( 0.000000000000000000, 0.01356324068817998940, -0.9999080150203990547 ) ) ;
#35118=CIRCLE ( 'NONE', #44665, 5.000000000000000888 ) ;
#35119=ORIENTED_EDGE ( 'NONE', *, *, #20482, .T. ) ;
#35120=ADVANCED_FACE ( 'NONE', ( #41455 ), #11863, .T. ) ;
#35121=B_SPLINE_CURVE_WITH_KNOTS ( 'NONE', 3,
 ( #53706, #8140, #28411, #22443, #43708, #33724, #38728, #42708, #54021, #49055 ),
 .UNSPECIFIED., .F., .F.,
 ( 4, 2, 2, 2, 4 ),
 ( 0.005719258168536343369, 0.006386639034606452631, 0.007054019900676561892, 0.007721400766746672889, 0.008388781632816783018 ),
 .UNSPECIFIED. ) ;
#35123=EDGE_CURVE ( 'NONE', #51803, #61423, #15856, .T. ) ;
#35124=FACE_OUTER_BOUND ( 'NONE', #55946, .T. ) ;
#35125=ORIENTED_EDGE ( 'NONE', *, *, #10484, .T. ) ;
#35126=AXIS2_PLACEMENT_3D ( 'NONE', #53588, #63524, #12008 ) ;
#35128=CARTESIAN_POINT ( 'NONE',  ( 11.52778293799294396, 11.81657713697700629, -2.095136543809601903 ) ) ;
#35129=DIRECTION ( 'NONE',  ( 0.000000000000000000, 0.01356324068817992175, -0.9999080150203990547 ) ) ;
#35130=VERTEX_POINT ( 'NONE', #11537 ) ;
#35131=EDGE_LOOP ( 'NONE', ( #16261, #61535, #10307, #6730 ) ) ;
#35134=CIRCLE ( 'NONE', #42587, 12.18649999999999878 ) ;
#35135=ORIENTED_EDGE ( 'NONE', *, *, #24953, .F. ) ;
#35136=DIRECTION ( 'NONE',  ( -1.000000000000000000, 0.000000000000000000, 0.000000000000000000 ) ) ;
#35139=CARTESIAN_POINT ( 'NONE',  ( -29.67854887312627810, -0.9836058970513458233, 11.96157915316133113 ) ) ;
#35140=AXIS2_PLACEMENT_3D ( 'NONE', #51081, #41395, #21469 ) ;
#35141=CIRCLE ( 'NONE', #61737, 12.75000000000000178 ) ;
#35144=VECTOR ( 'NONE', #58111, 1000.000000000000000 ) ;
#35145=DIRECTION ( 'NONE',  ( -1.000000000000000000, 0.000000000000000000, 0.000000000000000000 ) ) ;
#35148=CARTESIAN_POINT ( 'NONE',  ( 22.48401433917421244, 10.66787085122025047, -5.506576138129045006 ) ) ;
#35149=DIRECTION ( 'NONE',  ( 0.000000000000000000, -0.9718671068226484300, 0.2355298848897412201 ) ) ;
#35150=CARTESIAN_POINT ( 'NONE',  ( 12.45309242253974880, 13.08615109455304726, -3.321667012947705722 ) ) ;
#35151=CARTESIAN_POINT ( 'NONE',  ( 37.00000000000000711, 5.273331777780336793, -10.49591321039682690 ) ) ;
#35152=CYLINDRICAL_SURFACE ( 'NONE', #22530, 5.000000000000000888 ) ;
#35153=DIRECTION ( 'NONE',  ( 0.000000000000000000, -0.01356324068817999114, 0.9999080150203989437 ) ) ;
#35156=AXIS2_PLACEMENT_3D ( 'NONE', #19684, #24990, #65522 ) ;
#35161=EDGE_CURVE ( 'NONE', #21899, #16286, #36491, .T. ) ;
#35163=CARTESIAN_POINT ( 'NONE',  ( 35.00000000000000000, -12.08216339958901564, -1.591260454995201412 ) ) ;
#35165=CARTESIAN_POINT ( 'NONE',  ( -36.00000000000000711, -12.16893194857547655, -3.805206332242601075 ) ) ;
#35167=CARTESIAN_POINT ( 'NONE',  ( 35.00000000000000000, 4.705694406421931860E-17, -3.469127814946512892E-15 ) ) ;
#35169=VERTEX_POINT ( 'NONE', #31496 ) ;
#35174=CARTESIAN_POINT ( 'NONE',  ( -37.00000000000000711, -11.59605747147783106, -5.300372733891765442 ) ) ;
#35175=DIRECTION ( 'NONE',  ( 0.000000000000000000, 0.01356324068817998940, -0.9999080150203990547 ) ) ;
#35177=CIRCLE ( 'NONE', #25658, 12.75000000000000178 ) ;
#35178=DIRECTION ( 'NONE',  ( 0.000000000000000000, 0.01356324068817991828, -0.9999080150203990547 ) ) ;
#35182=VECTOR ( 'NONE', #41172, 1000.000000000000000 ) ;
#35185=EDGE_CURVE ( 'NONE', #65463, #57020, #26506, .T. ) ;
#35187=LINE ( 'NONE', #60468, #32034 ) ;
#35188=EDGE_CURVE ( 'NONE', #9403, #60864, #62397, .T. ) ;
#35190=AXIS2_PLACEMENT_3D ( 'NONE', #6964, #63448, #57181 ) ;
#35191=AXIS2_PLACEMENT_3D ( 'NONE', #7818, #2516, #22787 ) ;
#35192=VERTEX_POINT ( 'NONE', #6573 ) ;
#35197=DIRECTION ( 'NONE',  ( -1.000000000000000000, 0.000000000000000000, 0.000000000000000000 ) ) ;
#35198=DIRECTION ( 'NONE',  ( 0.000000000000000000, -0.1740410799127470598, -0.9847383929261643853 ) ) ;
#35201=CARTESIAN_POINT ( 'NONE',  ( 37.00000000000000711, -10.39746860227895731, -7.379373053628834889 ) ) ;
#35202=B_SPLINE_CURVE_WITH_KNOTS ( 'NONE', 3,
 ( #28651, #33647, #17036, #13360, #8376, #57627, #62914, #52945, #47966, #2422, #22700, #58268, #12689, #53282, #7726, #28015, #48316, #2767 ),
 .UNSPECIFIED., .F., .F.,
 ( 4, 2, 2, 2, 2, 2, 2, 2, 4 ),
 ( 0.000000000000000000, 0.001109628529027648818, 0.002219257058055297636, 0.003328885587082946670, 0.004438514116110595271, 0.005548142645138243872, 0.006657771174165893341, 0.007767399703193541942, 0.008877028232221188808 ),
 .UNSPECIFIED. ) ;
#35203=DIRECTION ( 'NONE',  ( -1.000000000000000000, -0.000000000000000000, 0.000000000000000000 ) ) ;
#35204=CARTESIAN_POINT ( 'NONE',  ( -37.00000000000000711, -2.250029553613845934, 12.54989509947650284 ) ) ;
#35205=ORIENTED_EDGE ( 'NONE', *, *, #38568, .F. ) ;
#35210=EDGE_CURVE ( 'NONE', #6781, #36007, #16547, .T. ) ;
#35211=AXIS2_PLACEMENT_3D ( 'NONE', #65448, #8961, #49540 ) ;
#35212=FACE_OUTER_BOUND ( 'NONE', #47469, .T. ) ;
#35213=ORIENTED_EDGE ( 'NONE', *, *, #64943, .F. ) ;
#35215=ADVANCED_FACE ( 'NONE', ( #57778 ), #36817, .T. ) ;
#35216=LINE ( 'NONE', #9964, #30012 ) ;
#35218=CARTESIAN_POINT ( 'NONE',  ( -2.952869152607106251, -11.39722960915210592, 3.755417052241485365 ) ) ;
#35219=CARTESIAN_POINT ( 'NONE',  ( 35.00000000000000000, 4.705694406421931860E-17, -3.469127814946512892E-15 ) ) ;
#35220=DIRECTION ( 'NONE',  ( 1.000000000000000000, 0.000000000000000000, -0.000000000000000000 ) ) ;
#35221=CARTESIAN_POINT ( 'NONE',  ( 6.812204945636112896, -4.138731716409435712, 11.26369831714195335 ) ) ;
#35223=VECTOR ( 'NONE', #15746, 1000.000000000000000 ) ;
#35224=ORIENTED_EDGE ( 'NONE', *, *, #24929, .T. ) ;
#35228=ORIENTED_EDGE ( 'NONE', *, *, #52240, .F. ) ;
#35229=VECTOR ( 'NONE', #22086, 1000.000000000000000 ) ;
#35230=VERTEX_POINT ( 'NONE', #47464 ) ;
#35231=ORIENTED_EDGE ( 'NONE', *, *, #48735, .T. ) ;
#35234=DIRECTION ( 'NONE',  ( 1.000000000000000000, -0.000000000000000000, 0.000000000000000000 ) ) ;
#35235=DIRECTION ( 'NONE',  ( 0.000000000000000000, 0.000000000000000000, -1.000000000000000000 ) ) ;
#35236=ORIENTED_EDGE ( 'NONE', *, *, #36409, .F. ) ;
#35238=LINE ( 'NONE', #29593, #46019 ) ;
#35240=ORIENTED_EDGE ( 'NONE', *, *, #53758, .T. ) ;
#35241=DIRECTION ( 'NONE',  ( 0.000000000000000000, -0.9346839223284501008, 0.3554799084909069928 ) ) ;
#35245=CARTESIAN_POINT ( 'NONE',  ( 27.47563550582765757, 10.97366218211726974, 4.866891853559282666 ) ) ;
#35247=AXIS2_PLACEMENT_3D ( 'NONE', #6852, #47090, #17476 ) ;
#35248=VECTOR ( 'NONE', #7514, 1000.000000000000000 ) ;
#35250=ORIENTED_EDGE ( 'NONE', *, *, #55751, .T. ) ;
#35253=VERTEX_POINT ( 'NONE', #48454 ) ;
#35257=DIRECTION ( 'NONE',  ( 0.000000000000000000, -0.9105187689795999351, 0.4134677391718417638 ) ) ;
#35258=CARTESIAN_POINT ( 'NONE',  ( 12.36235005266927978, 8.714858184812433350, -8.258156698578600796 ) ) ;
#35259=ORIENTED_EDGE ( 'NONE', *, *, #22119, .T. ) ;
#35260=B_SPLINE_CURVE_WITH_KNOTS ( 'NONE', 3,
 ( #14406, #44660, #24735, #15064, #60625, #113, #9104, #29074 ),
 .UNSPECIFIED., .F., .F.,
 ( 4, 2, 2, 4 ),
 ( 0.009775493497823107072, 0.01050469463799914675, 0.01123389577817518817, 0.01269229805852726926 ),
 .UNSPECIFIED. ) ;
#35261=CARTESIAN_POINT ( 'NONE',  ( 37.00000000000000711, 4.705694406421931860E-17, -3.469127814946512892E-15 ) ) ;
#35262=LINE ( 'NONE', #23, #22738 ) ;
#35265=CIRCLE ( 'NONE', #63943, 12.75000000000000178 ) ;
#35266=AXIS2_PLACEMENT_3D ( 'NONE', #44943, #55245, #65530 ) ;
#35267=EDGE_CURVE ( 'NONE', #50238, #7848, #28725, .T. ) ;
#35269=AXIS2_PLACEMENT_3D ( 'NONE', #39971, #55266, #20345 ) ;
#35272=ADVANCED_FACE ( 'NONE', ( #22851 ), #27481, .T. ) ;
#35274=FACE_OUTER_BOUND ( 'NONE', #60103, .T. ) ;
#35275=EDGE_CURVE ( 'NONE', #51572, #6221, #43103, .T. ) ;
#35276=EDGE_LOOP ( 'NONE', ( #43568, #58657, #5841, #47748 ) ) ;
#35279=EDGE_LOOP ( 'NONE', ( #38146, #51171, #65503, #18792 ) ) ;
#35280=DIRECTION ( 'NONE',  ( 0.000000000000000000, -0.5472293298355157543, 0.8369827122275419473 ) ) ;
#35281=FACE_OUTER_BOUND ( 'NONE', #11796, .T. ) ;
#35283=VERTEX_POINT ( 'NONE', #63069 ) ;
#35285=VERTEX_POINT ( 'NONE', #53763 ) ;
#35286=ORIENTED_EDGE ( 'NONE', *, *, #56007, .F. ) ;
#35287=CARTESIAN_POINT ( 'NONE',  ( 28.68872621665320821, -10.58213401676968246, 5.662857775278662409 ) ) ;
#35288=EDGE_CURVE ( 'NONE', #33595, #44052, #43479, .T. ) ;
#35289=VECTOR ( 'NONE', #58871, 1000.000000000000000 ) ;
#35290=CARTESIAN_POINT ( 'NONE',  ( -20.79170840334646542, -11.34110549087206898, -3.921648409140116698 ) ) ;
#35291=CIRCLE ( 'NONE', #10860, 5.000000000000000000 ) ;
#35293=LINE ( 'NONE', #49950, #58097 ) ;
#35294=CARTESIAN_POINT ( 'NONE',  ( -17.83419946441818027, -9.720786832536937538, 7.036071585506806336 ) ) ;
#35295=ORIENTED_EDGE ( 'NONE', *, *, #51730, .T. ) ;
#35298=CYLINDRICAL_SURFACE ( 'NONE', #58989, 4.999999999999999112 ) ;
#35300=ORIENTED_EDGE ( 'NONE', *, *, #47085, .T. ) ;
#35301=CARTESIAN_POINT ( 'NONE',  ( -25.54417658651491863, 7.498517398407837931, 11.22596262356930197 ) ) ;
#35303=FACE_OUTER_BOUND ( 'NONE', #64987, .T. ) ;
#35304=ORIENTED_EDGE ( 'NONE', *, *, #59311, .T. ) ;
#35306=FACE_OUTER_BOUND ( 'NONE', #46350, .T. ) ;
#35310=CIRCLE ( 'NONE', #63985, 12.74999999999999822 ) ;
#35315=FACE_OUTER_BOUND ( 'NONE', #35827, .T. ) ;
#35316=CARTESIAN_POINT ( 'NONE',  ( -7.489022030332961322, -8.034049540753116503, -10.84914964302385521 ) ) ;
#35317=VERTEX_POINT ( 'NONE', #47783 ) ;
#35319=ORIENTED_EDGE ( 'NONE', *, *, #41410, .T. ) ;
#35322=AXIS2_PLACEMENT_3D ( 'NONE', #12256, #32519, #61478 ) ;
#35323=VERTEX_POINT ( 'NONE', #23161 ) ;
#35324=CARTESIAN_POINT ( 'NONE',  ( 37.00000000000000711, 11.59095880812004964, -1.903127969211395598 ) ) ;
#35325=DIRECTION ( 'NONE',  ( 1.000000000000000000, 0.000000000000000000, 0.000000000000000000 ) ) ;
#35327=DIRECTION ( 'NONE',  ( -1.000000000000000000, 0.000000000000000000, 0.000000000000000000 ) ) ;
#35329=LINE ( 'NONE', #54968, #12143 ) ;
#35330=EDGE_CURVE ( 'NONE', #52081, #1502, #63481, .T. ) ;
#35331=( BOUNDED_CURVE ( )  B_SPLINE_CURVE ( 3, ( #17822, #47755, #1876, #63356 ),
 .UNSPECIFIED., .F., .F. ) 
 B_SPLINE_CURVE_WITH_KNOTS ( ( 4, 4 ),
 ( 4.456175814406320157, 4.486258350949901441 ),
 .UNSPECIFIED. ) 
 CURVE ( )  GEOMETRIC_REPRESENTATION_ITEM ( )  RATIONAL_B_SPLINE_CURVE ( ( 1.000000000000000000, 0.9999245881713708650, 0.9999245881713708650, 1.000000000000000000 ) ) 
 REPRESENTATION_ITEM ( '' )  );
#35332=EDGE_LOOP ( 'NONE', ( #48311, #19121, #15113, #59535 ) ) ;
#35333=DIRECTION ( 'NONE',  ( 1.836970198721029688E-16, -1.000000000000000000, 0.000000000000000000 ) ) ;
#35334=CARTESIAN_POINT ( 'NONE',  ( 37.00000000000000711, 4.705694406421931860E-17, -3.469127814946512892E-15 ) ) ;
#35335=ADVANCED_FACE ( 'NONE', ( #43770 ), #43424, .T. ) ;
#35337=EDGE_LOOP ( 'NONE', ( #18620, #26338, #48106, #14347 ) ) ;
#35338=VECTOR ( 'NONE', #17648, 1000.000000000000000 ) ;
#35339=AXIS2_PLACEMENT_3D ( 'NONE', #29491, #18584, #54792 ) ;
#35341=AXIS2_PLACEMENT_3D ( 'NONE', #11013, #35615, #20324 ) ;
#35343=LINE ( 'NONE', #60623, #54320 ) ;
#35344=CIRCLE ( 'NONE', #42801, 12.18649999999999700 ) ;
#35345=DIRECTION ( 'NONE',  ( 0.000000000000000000, 0.4935949184179262983, -0.8696919319575183716 ) ) ;
#35346=CARTESIAN_POINT ( 'NONE',  ( 35.00000000000000000, -3.704519465651390675, -11.60979404548633731 ) ) ;
#35347=VERTEX_POINT ( 'NONE', #12195 ) ;
#35351=CARTESIAN_POINT ( 'NONE',  ( 3.878049410135225639, 5.417590671930183177, 10.70984159994429596 ) ) ;
#35352=VECTOR ( 'NONE', #20653, 1000.000000000000000 ) ;
#35353=AXIS2_PLACEMENT_3D ( 'NONE', #4229, #3914, #30150 ) ;
#35354=EDGE_CURVE ( 'NONE', #33621, #16066, #45721, .T. ) ;
#35359=CARTESIAN_POINT ( 'NONE',  ( 3.426384734005718524, 5.858157115608569221, -10.47507226477059383 ) ) ;
#35360=AXIS2_PLACEMENT_3D ( 'NONE', #17004, #16682, #22312 ) ;
#35361=DIRECTION ( 'NONE',  ( 0.000000000000000000, 0.9796553971857748788, 0.2006870767258854826 ) ) ;
#35363=CARTESIAN_POINT ( 'NONE',  ( 9.958180664929905390, 1.092159088654170329, 13.45683414571523429 ) ) ;
#35366=VERTEX_POINT ( 'NONE', #52773 ) ;
#35367=EDGE_LOOP ( 'NONE', ( #31106, #63795, #31842, #44454 ) ) ;
#35370=CARTESIAN_POINT ( 'NONE',  ( 37.00000000000000711, 4.705694406421931860E-17, -3.469127814946512892E-15 ) ) ;
#35371=CARTESIAN_POINT ( 'NONE',  ( 27.62838931380291996, 25.00000000000000000, -3.066727421130092779 ) ) ;
#35372=DIRECTION ( 'NONE',  ( 1.000000000000000000, 0.000000000000000000, 0.000000000000000000 ) ) ;
#35376=CARTESIAN_POINT ( 'NONE',  ( 24.67726771998958668, 0.8588187409780198012, -13.47840055350262212 ) ) ;
#35377=DIRECTION ( 'NONE',  ( -1.000000000000000000, 0.000000000000000000, 0.000000000000000000 ) ) ;
#35378=VERTEX_POINT ( 'NONE', #48771 ) ;
#35379=DIRECTION ( 'NONE',  ( 1.000000000000000000, 0.000000000000000000, 0.000000000000000000 ) ) ;
#35380=ORIENTED_EDGE ( 'NONE', *, *, #55385, .F. ) ;
#35382=DIRECTION ( 'NONE',  ( 1.000000000000000000, 0.000000000000000000, -0.000000000000000000 ) ) ;
#35383=ORIENTED_EDGE ( 'NONE', *, *, #28080, .T. ) ;
#35384=VECTOR ( 'NONE', #51700, 1000.000000000000000 ) ;
#35385=ORIENTED_EDGE ( 'NONE', *, *, #33567, .T. ) ;
#35388=AXIS2_PLACEMENT_3D ( 'NONE', #55660, #19759, #64951 ) ;
#35389=FACE_OUTER_BOUND ( 'NONE', #9880, .T. ) ;
#35391=DIRECTION ( 'NONE',  ( -1.000000000000000000, 0.000000000000000000, -0.000000000000000000 ) ) ;
#35393=LINE ( 'NONE', #64659, #12919 ) ;
#35395=VERTEX_POINT ( 'NONE', #34098 ) ;
#35397=VERTEX_POINT ( 'NONE', #45396 ) ;
#35398=CIRCLE ( 'NONE', #22699, 5.000000000000000888 ) ;
#35399=EDGE_LOOP ( 'NONE', ( #31680, #45094, #32506, #57236 ) ) ;
#35400=AXIS2_PLACEMENT_3D ( 'NONE', #57875, #52866, #7297 ) ;
#35402=CARTESIAN_POINT ( 'NONE',  ( 10.48620311856346454, 8.250315036047107142, -8.713914264323181058 ) ) ;
#35403=DIRECTION ( 'NONE',  ( 1.000000000000000000, 0.000000000000000000, 0.000000000000000000 ) ) ;
#35406=AXIS2_PLACEMENT_3D ( 'NONE', #59684, #55680, #19452 ) ;
#35407=DIRECTION ( 'NONE',  ( -0.000000000000000000, -1.000000000000000000, -0.000000000000000000 ) ) ;
#35408=EDGE_CURVE ( 'NONE', #7420, #30257, #39351, .T. ) ;
#35409=FACE_OUTER_BOUND ( 'NONE', #2406, .T. ) ;
#35410=VERTEX_POINT ( 'NONE', #29445 ) ;
#35411=AXIS2_PLACEMENT_3D ( 'NONE', #24761, #60995, #29725 ) ;
#35412=EDGE_CURVE ( 'NONE', #24790, #57555, #25632, .T. ) ;
#35413=ORIENTED_EDGE ( 'NONE', *, *, #51277, .T. ) ;
#35414=CIRCLE ( 'NONE', #51347, 5.000000000000000000 ) ;
#35416=DIRECTION ( 'NONE',  ( 0.000000000000000000, -0.01356324068817991828, 0.9999080150203990547 ) ) ;
#35418=B_SPLINE_CURVE_WITH_KNOTS ( 'NONE', 3,
 ( #42524, #17289, #56198, #25964, #23252, #58518, #37571, #43517, #48864, #22944, #2332, #58181, #7291, #63798, #2991, #8290, #3319, #27922, #18282, #8609, #38881, #33564, #38546, #58866, #13282, #18623 ),
 .UNSPECIFIED., .F., .F.,
 ( 4, 2, 2, 2, 2, 2, 2, 2, 2, 2, 2, 2, 4 ),
 ( 0.000000000000000000, 0.001187878019264044637, 0.001781817028896066739, 0.002375756038528089274, 0.002969695048160110509, 0.003563634057792131309, 0.004157573067424152544, 0.004751512077056174212, 0.005345451086688195012, 0.005939390096320216680, 0.007127268115584260884, 0.008315146134848305087, 0.009503024154112350158 ),
 .UNSPECIFIED. ) ;
#35419=CARTESIAN_POINT ( 'NONE',  ( 6.661533233520612107, -4.211056110068225777, -12.82664335996205196 ) ) ;
#35420=CARTESIAN_POINT ( 'NONE',  ( 6.529851256712529306, -4.705937351017101200, 11.04517589364730235 ) ) ;
#35421=CIRCLE ( 'NONE', #6775, 12.18650000000000055 ) ;
#35423=EDGE_CURVE ( 'NONE', #3983, #21953, #19184, .T. ) ;
#35424=CARTESIAN_POINT ( 'NONE',  ( 24.35413283551385177, -1.441936682210068099, -13.42734599445702415 ) ) ;
#35425=EDGE_CURVE ( 'NONE', #42626, #46347, #34745, .T. ) ;
#35426=CARTESIAN_POINT ( 'NONE',  ( -36.00000000000000711, -9.621072037177057723, 8.366449238204328509 ) ) ;
#35428=ORIENTED_EDGE ( 'NONE', *, *, #55773, .T. ) ;
#35429=VECTOR ( 'NONE', #42071, 1000.000000000000000 ) ;
#35432=VECTOR ( 'NONE', #23897, 1000.000000000000000 ) ;
#35436=ADVANCED_FACE ( 'NONE', ( #65662 ), #14150, .T. ) ;
#35440=CARTESIAN_POINT ( 'NONE',  ( -18.52069857313810175, -4.381854579544467221, -12.76954371343036954 ) ) ;
#35446=DIRECTION ( 'NONE',  ( 0.000000000000000000, -0.01356324068817992175, 0.9999080150203990547 ) ) ;
#35447=CYLINDRICAL_SURFACE ( 'NONE', #52295, 4.999999999999999112 ) ;
#35448=FACE_OUTER_BOUND ( 'NONE', #47220, .T. ) ;
#35449=CIRCLE ( 'NONE', #45009, 5.000000000000002665 ) ;
#35451=ORIENTED_EDGE ( 'NONE', *, *, #24358, .T. ) ;
#35452=FACE_OUTER_BOUND ( 'NONE', #18988, .T. ) ;
#35453=CYLINDRICAL_SURFACE ( 'NONE', #9575, 5.000000000000000888 ) ;
#35454=VERTEX_POINT ( 'NONE', #54745 ) ;
#35456=DIRECTION ( 'NONE',  ( -1.000000000000000000, 0.000000000000000000, 0.000000000000000000 ) ) ;
#35457=DIRECTION ( 'NONE',  ( 0.000000000000000000, -0.9346839223284580944, 0.3554799084908867868 ) ) ;
#35458=DIRECTION ( 'NONE',  ( 1.000000000000000000, 0.000000000000000000, 0.000000000000000000 ) ) ;
#35459=CARTESIAN_POINT ( 'NONE',  ( 37.00000000000000711, 4.705694406421931860E-17, -3.469127814946512892E-15 ) ) ;
#35460=CIRCLE ( 'NONE', #4702, 4.999999999999999112 ) ;
#35461=CARTESIAN_POINT ( 'NONE',  ( -37.00000000000000711, 0.000000000000000000, 0.000000000000000000 ) ) ;
#35463=ORIENTED_EDGE ( 'NONE', *, *, #59935, .F. ) ;
#35464=DIRECTION ( 'NONE',  ( -1.000000000000000000, 0.000000000000000000, 0.000000000000000000 ) ) ;
#35467=CARTESIAN_POINT ( 'NONE',  ( -47.00000000000000711, 0.000000000000000000, 0.000000000000000000 ) ) ;
#35468=CARTESIAN_POINT ( 'NONE',  ( 16.78263030916553333, -12.17295508002144011, 5.836879698929882565 ) ) ;
#35471=AXIS2_PLACEMENT_3D ( 'NONE', #50651, #20373, #20709 ) ;
#35472=DIRECTION ( 'NONE',  ( 0.000000000000000000, 0.01356324068817998940, -0.9999080150203990547 ) ) ;
#35473=VERTEX_POINT ( 'NONE', #9164 ) ;
#35474=CYLINDRICAL_SURFACE ( 'NONE', #8569, 12.18650000000000055 ) ;
#35477=ORIENTED_EDGE ( 'NONE', *, *, #39954, .F. ) ;
#35480=AXIS2_PLACEMENT_3D ( 'NONE', #22126, #17803, #52733 ) ;
#35481=EDGE_CURVE ( 'NONE', #14609, #8090, #6519, .T. ) ;
#35482=CIRCLE ( 'NONE', #17461, 5.000000000000000888 ) ;
#35483=ORIENTED_EDGE ( 'NONE', *, *, #52799, .T. ) ;
#35487=CARTESIAN_POINT ( 'NONE',  ( -29.63048194961400483, -0.3368890121124099024, 11.99716775028113425 ) ) ;
#35488=CARTESIAN_POINT ( 'NONE',  ( -35.00000000000000000, -11.66953048682402283, 3.511814412392074480 ) ) ;
#35490=EDGE_CURVE ( 'NONE', #2448, #27489, #108, .T. ) ;
#35492=VERTEX_POINT ( 'NONE', #3882 ) ;
#35494=CARTESIAN_POINT ( 'NONE',  ( 23.00365627137244573, 10.16437141043587289, -6.387237743053422179 ) ) ;
#35498=VECTOR ( 'NONE', #43025, 1000.000000000000000 ) ;
#35499=FACE_OUTER_BOUND ( 'NONE', #33386, .T. ) ;
#35502=CYLINDRICAL_SURFACE ( 'NONE', #11896, 5.000000000000000888 ) ;
#35503=AXIS2_PLACEMENT_3D ( 'NONE', #51105, #61710, #56764 ) ;
#35505=DIRECTION ( 'NONE',  ( -1.000000000000000000, 0.000000000000000000, 0.000000000000000000 ) ) ;
#35506=EDGE_LOOP ( 'NONE', ( #39373, #14389, #37189, #33871 ) ) ;
#35507=DIRECTION ( 'NONE',  ( 0.000000000000000000, -0.3218879778915842427, 0.9467777615094616905 ) ) ;
#35508=LINE ( 'NONE', #40838, #50028 ) ;
#35510=EDGE_CURVE ( 'NONE', #52527, #36765, #9678, .T. ) ;
#35514=ADVANCED_FACE ( 'NONE', ( #24804 ), #45085, .T. ) ;
#35522=CARTESIAN_POINT ( 'NONE',  ( -35.00000000000000000, -11.39945968423475264, 5.710938531231672499 ) ) ;
#35523=CARTESIAN_POINT ( 'NONE',  ( 35.00000000000000000, 4.705694406421931860E-17, -3.469127814946512892E-15 ) ) ;
#35524=( BOUNDED_CURVE ( )  B_SPLINE_CURVE ( 3, ( #38923, #38591, #7330, #12640 ),
 .UNSPECIFIED., .F., .F. ) 
 B_SPLINE_CURVE_WITH_KNOTS ( ( 4, 4 ),
 ( 1.632078076156195046, 1.647829253658086746 ),
 .UNSPECIFIED. ) 
 CURVE ( )  GEOMETRIC_REPRESENTATION_ITEM ( )  RATIONAL_B_SPLINE_CURVE ( ( 1.000000000000000000, 0.9999793251408052308, 0.9999793251408052308, 1.000000000000000000 ) ) 
 REPRESENTATION_ITEM ( '' )  );
#35525=ORIENTED_EDGE ( 'NONE', *, *, #35018, .F. ) ;
#35526=CARTESIAN_POINT ( 'NONE',  ( -35.00000000000000000, 2.968224442958403486, 11.81949347079748058 ) ) ;
#35527=EDGE_CURVE ( 'NONE', #2866, #41816, #5978, .T. ) ;
#35528=ORIENTED_EDGE ( 'NONE', *, *, #10879, .F. ) ;
#35530=DIRECTION ( 'NONE',  ( -1.000000000000000000, 0.000000000000000000, 0.000000000000000000 ) ) ;
#35531=CARTESIAN_POINT ( 'NONE',  ( 29.16097522612058413, -8.612999037061474183, 8.368222170583779373 ) ) ;
#35532=DIRECTION ( 'NONE',  ( 1.000000000000000000, -0.000000000000000000, 0.000000000000000000 ) ) ;
#35533=VERTEX_POINT ( 'NONE', #15468 ) ;
#35543=CARTESIAN_POINT ( 'NONE',  ( 3.291290029914074378, 8.250315036047103590, 25.00000000000000000 ) ) ;
#35545=AXIS2_PLACEMENT_3D ( 'NONE', #59543, #48597, #58581 ) ;
#35547=ORIENTED_EDGE ( 'NONE', *, *, #36805, .F. ) ;
#35549=AXIS2_PLACEMENT_3D ( 'NONE', #29651, #24687, #56241 ) ;
#35550=DIRECTION ( 'NONE',  ( -1.000000000000000000, 0.000000000000000000, 0.000000000000000000 ) ) ;
#35551=ADVANCED_FACE ( 'NONE', ( #62560 ), #56030, .T. ) ;
#35553=FACE_OUTER_BOUND ( 'NONE', #27420, .T. ) ;
#35554=EDGE_CURVE ( 'NONE', #23085, #55514, #35733, .T. ) ;
#35555=ORIENTED_EDGE ( 'NONE', *, *, #46326, .T. ) ;
#35556=CARTESIAN_POINT ( 'NONE',  ( 18.84867683979355846, 25.00000000000000000, 12.12095735156415088 ) ) ;
#35557=CARTESIAN_POINT ( 'NONE',  ( 6.192035194031760170, -8.543018847948518513, -10.45909626451002161 ) ) ;
#35559=CARTESIAN_POINT ( 'NONE',  ( 7.278301338833046863, -5.781067271407755115, 10.51827409704459093 ) ) ;
#35560=ORIENTED_EDGE ( 'NONE', *, *, #64246, .F. ) ;
#35563=ORIENTED_EDGE ( 'NONE', *, *, #31018, .F. ) ;
#35567=ORIENTED_EDGE ( 'NONE', *, *, #14987, .T. ) ;
#35572=DIRECTION ( 'NONE',  ( 0.000000000000000000, 0.9551603052523490733, -0.2960891610144476549 ) ) ;
#35573=DIRECTION ( 'NONE',  ( -1.000000000000000000, 0.000000000000000000, -0.000000000000000000 ) ) ;
#35574=EDGE_LOOP ( 'NONE', ( #40895, #35205, #60238, #40306 ) ) ;
#35578=CYLINDRICAL_SURFACE ( 'NONE', #20344, 5.000000000000000888 ) ;
#35579=ADVANCED_FACE ( 'NONE', ( #47955 ), #57617, .T. ) ;
#35580=VECTOR ( 'NONE', #48988, 1000.000000000000000 ) ;
#35581=ORIENTED_EDGE ( 'NONE', *, *, #33430, .F. ) ;
#35585=EDGE_CURVE ( 'NONE', #61650, #29988, #6481, .T. ) ;
#35586=EDGE_LOOP ( 'NONE', ( #35701, #42233, #35996, #44913, #2959, #52015 ) ) ;
#35587=DIRECTION ( 'NONE',  ( -1.000000000000000000, 0.000000000000000000, 0.000000000000000000 ) ) ;
#35588=AXIS2_PLACEMENT_3D ( 'NONE', #35261, #55570, #10010 ) ;
#35589=EDGE_LOOP ( 'NONE', ( #14262, #33226, #32310, #42142 ) ) ;
#35594=DIRECTION ( 'NONE',  ( -1.000000000000000000, 0.000000000000000000, 0.000000000000000000 ) ) ;
#35595=VERTEX_POINT ( 'NONE', #12035 ) ;
#35596=DIRECTION ( 'NONE',  ( 0.000000000000000000, -0.01356324068818000328, 0.9999080150203990547 ) ) ;
#35598=DIRECTION ( 'NONE',  ( -1.000000000000000000, -0.000000000000000000, 0.000000000000000000 ) ) ;
#35599=CARTESIAN_POINT ( 'NONE',  ( 21.98021488419000136, -12.96235417471537943, -3.789643664872785145 ) ) ;
#35602=EDGE_CURVE ( 'NONE', #28220, #8078, #50053, .T. ) ;
#35604=CARTESIAN_POINT ( 'NONE',  ( -35.00000000000000000, -5.814360711498210321, -10.70999494708499000 ) ) ;
#35607=CARTESIAN_POINT ( 'NONE',  ( -7.393613020821579340, -5.386680228572943818, -10.72686196631678968 ) ) ;
#35609=CIRCLE ( 'NONE', #8061, 12.18650000000000055 ) ;
#35611=VERTEX_POINT ( 'NONE', #64855 ) ;
#35613=DIRECTION ( 'NONE',  ( -1.000000000000000000, -1.836970198721029688E-16, -0.000000000000000000 ) ) ;
#35615=DIRECTION ( 'NONE',  ( 1.000000000000000000, 0.000000000000000000, 0.000000000000000000 ) ) ;
#35617=ORIENTED_EDGE ( 'NONE', *, *, #23972, .F. ) ;
#35618=ORIENTED_EDGE ( 'NONE', *, *, #7887, .F. ) ;
#35619=ORIENTED_EDGE ( 'NONE', *, *, #41590, .F. ) ;
#35622=VERTEX_POINT ( 'NONE', #13030 ) ;
#35624=DIRECTION ( 'NONE',  ( 1.000000000000000000, 0.000000000000000000, 0.000000000000000000 ) ) ;
#35625=DIRECTION ( 'NONE',  ( -1.000000000000000000, -0.000000000000000000, 0.000000000000000000 ) ) ;
#35627=ORIENTED_EDGE ( 'NONE', *, *, #61961, .T. ) ;
#35628=AXIS2_PLACEMENT_3D ( 'NONE', #64691, #3234, #58779 ) ;
#35631=CARTESIAN_POINT ( 'NONE',  ( -35.00000000000000000, -11.61175578952785159, -1.771820996347277966 ) ) ;
#35632=VERTEX_POINT ( 'NONE', #43271 ) ;
#35634=EDGE_LOOP ( 'NONE', ( #1381, #53337, #64504, #11530 ) ) ;
#35635=CARTESIAN_POINT ( 'NONE',  ( 37.00000000000000711, -7.717887834988180984, 8.854740511458926377 ) ) ;
#35636=ORIENTED_EDGE ( 'NONE', *, *, #24377, .F. ) ;
#35637=CARTESIAN_POINT ( 'NONE',  ( 13.18551377979218486, -11.38597202338936754, -3.795551372338616947 ) ) ;
#35638=CIRCLE ( 'NONE', #30339, 5.000000000000000000 ) ;
#35640=CARTESIAN_POINT ( 'NONE',  ( 35.00000000000000000, 11.54110654723649176, -2.185196060783925809 ) ) ;
#35641=CARTESIAN_POINT ( 'NONE',  ( -37.00000000000000711, 9.240395740215735287, -7.251710744571480127 ) ) ;
#35646=DIRECTION ( 'NONE',  ( -1.000000000000000000, 0.000000000000000000, 0.000000000000000000 ) ) ;
#35647=ORIENTED_EDGE ( 'NONE', *, *, #21466, .F. ) ;
#35648=DIRECTION ( 'NONE',  ( -1.000000000000000000, 0.000000000000000000, 0.000000000000000000 ) ) ;
#35651=ORIENTED_EDGE ( 'NONE', *, *, #65610, .F. ) ;
#35652=CARTESIAN_POINT ( 'NONE',  ( 35.00000000000000000, 12.66641127287627633, 1.457575200925409709 ) ) ;
#35653=EDGE_CURVE ( 'NONE', #14422, #31670, #13941, .T. ) ;
#35654=VERTEX_POINT ( 'NONE', #58941 ) ;
#35655=CARTESIAN_POINT ( 'NONE',  ( -35.00000000000000000, 0.000000000000000000, 0.000000000000000000 ) ) ;
#35657=CARTESIAN_POINT ( 'NONE',  ( 22.57855258442564761, -4.427776684447072952, 11.15324139578564910 ) ) ;
#35658=CYLINDRICAL_SURFACE ( 'NONE', #30586, 12.74999999999999822 ) ;
#35659=EDGE_CURVE ( 'NONE', #5010, #34891, #21370, .T. ) ;
#35660=CARTESIAN_POINT ( 'NONE',  ( 11.99083905025486629, 8.556418439408664867, -8.415045165346294098 ) ) ;
#35661=VERTEX_POINT ( 'NONE', #53929 ) ;
#35665=CARTESIAN_POINT ( 'NONE',  ( 35.00000000000000000, -10.49626516989275515, -7.238157050195593634 ) ) ;
#35667=VERTEX_POINT ( 'NONE', #13999 ) ;
#35669=ADVANCED_FACE ( 'NONE', ( #8367 ), #3406, .T. ) ;
#35672=FACE_OUTER_BOUND ( 'NONE', #6301, .T. ) ;
#35673=CARTESIAN_POINT ( 'NONE',  ( -35.00000000000000000, 11.86701198550360203, -2.772148766915989881 ) ) ;
#35674=ORIENTED_EDGE ( 'NONE', *, *, #45550, .F. ) ;
#35675=DIRECTION ( 'NONE',  ( 0.000000000000000000, 0.9346839223284554299, -0.3554799084908935036 ) ) ;
#35678=EDGE_CURVE ( 'NONE', #24291, #18737, #43677, .T. ) ;
#35679=CARTESIAN_POINT ( 'NONE',  ( 22.88594695219327235, 3.421158645304719137, 25.00000000000000000 ) ) ;
#35680=DIRECTION ( 'NONE',  ( -1.000000000000000000, 0.000000000000000000, -0.000000000000000000 ) ) ;
#35681=ORIENTED_EDGE ( 'NONE', *, *, #53660, .F. ) ;
#35686=CARTESIAN_POINT ( 'NONE',  ( 12.19629890822712426, 0.02883110402050519452, 13.50000000000000355 ) ) ;
#35688=ORIENTED_EDGE ( 'NONE', *, *, #41600, .T. ) ;
#35694=DIRECTION ( 'NONE',  ( 0.000000000000000000, -0.6478160128812003871, 0.7617968321374831708 ) ) ;
#35695=CARTESIAN_POINT ( 'NONE',  ( 8.937200413559445167, 4.820982231796476114, 10.99527590820397549 ) ) ;
#35696=EDGE_CURVE ( 'NONE', #43264, #58366, #19003, .T. ) ;
#35699=DIRECTION ( 'NONE',  ( 1.000000000000000000, 0.000000000000000000, 0.000000000000000000 ) ) ;
#35700=CARTESIAN_POINT ( 'NONE',  ( -32.16141091265169649, 25.00000000000000000, 5.384978440493686236 ) ) ;
#35701=ORIENTED_EDGE ( 'NONE', *, *, #30925, .T. ) ;
#35703=DIRECTION ( 'NONE',  ( 1.000000000000000000, -0.000000000000000000, 0.000000000000000000 ) ) ;
#35704=ORIENTED_EDGE ( 'NONE', *, *, #45442, .T. ) ;
#35706=VERTEX_POINT ( 'NONE', #41228 ) ;
#35710=LINE ( 'NONE', #15109, #38578 ) ;
#35711=EDGE_CURVE ( 'NONE', #56844, #64727, #44922, .T. ) ;
#35712=DIRECTION ( 'NONE',  ( 0.000000000000000000, 0.01356324068817998940, -0.9999080150203989437 ) ) ;
#35714=CARTESIAN_POINT ( 'NONE',  ( -35.00000000000000000, 10.01317267707896441, -6.946017217729827387 ) ) ;
#35719=ORIENTED_EDGE ( 'NONE', *, *, #38840, .T. ) ;
#35720=EDGE_CURVE ( 'NONE', #53292, #11231, #29949, .T. ) ;
#35721=ORIENTED_EDGE ( 'NONE', *, *, #24729, .T. ) ;
#35723=CARTESIAN_POINT ( 'NONE',  ( 9.517144231691849754, 7.406568589130381852, -9.443085440640070161 ) ) ;
#35728=CARTESIAN_POINT ( 'NONE',  ( -5.440908200706632059, -0.9287346933962611351, -11.96401310621655334 ) ) ;
#35729=ORIENTED_EDGE ( 'NONE', *, *, #29636, .F. ) ;
#35731=DIRECTION ( 'NONE',  ( -1.000000000000000000, 0.000000000000000000, -0.000000000000000000 ) ) ;
#35732=DIRECTION ( 'NONE',  ( 0.000000000000000000, 0.1118654143051615868, 0.9937233664769762331 ) ) ;
#35733=LINE ( 'NONE', #42269, #45765 ) ;
#35734=DIRECTION ( 'NONE',  ( -1.000000000000000000, 0.000000000000000000, -0.000000000000000000 ) ) ;
#35737=CARTESIAN_POINT ( 'NONE',  ( 1.957321625297526957, 1.110016547387106423, -11.94976366055458961 ) ) ;
#35739=ORIENTED_EDGE ( 'NONE', *, *, #20674, .F. ) ;
#35741=CARTESIAN_POINT ( 'NONE',  ( 35.00000000000000000, -2.905556151562703082, -11.38112321385050052 ) ) ;
#35742=DIRECTION ( 'NONE',  ( -1.000000000000000000, 0.000000000000000000, -0.000000000000000000 ) ) ;
#35743=CIRCLE ( 'NONE', #19826, 5.000000000000000000 ) ;
#35744=EDGE_CURVE ( 'NONE', #27609, #41185, #37261, .T. ) ;
#35745=AXIS2_PLACEMENT_3D ( 'NONE', #60245, #64563, #4071 ) ;
#35746=PLANE ( 'NONE',  #42593 ) ;
#35749=CARTESIAN_POINT ( 'NONE',  ( -17.29080932782789048, -8.561852795175090236, -10.44285877056046452 ) ) ;
#35752=ORIENTED_EDGE ( 'NONE', *, *, #53472, .F. ) ;
#35754=CARTESIAN_POINT ( 'NONE',  ( -17.89006668746826989, 6.205840224181938147, -10.27317841523973385 ) ) ;
#35757=VERTEX_POINT ( 'NONE', #368 ) ;
#35758=DIRECTION ( 'NONE',  ( 1.000000000000000000, 0.000000000000000000, -0.000000000000000000 ) ) ;
#35759=EDGE_CURVE ( 'NONE', #65068, #53931, #8604, .T. ) ;
#35761=ORIENTED_EDGE ( 'NONE', *, *, #32300, .F. ) ;
#35762=CARTESIAN_POINT ( 'NONE',  ( -35.00000000000000000, -4.561791185930498926, 11.90598845858532151 ) ) ;
#35765=CARTESIAN_POINT ( 'NONE',  ( 35.00000000000000000, -9.677500615117850202, 6.657191900728419043 ) ) ;
#35767=CARTESIAN_POINT ( 'NONE',  ( 0.09505445835107248498, -0.1369421331495652150, -13.50000000000000355 ) ) ;
#35768=ADVANCED_FACE ( 'NONE', ( #36239 ), #9654, .T. ) ;
#35769=CARTESIAN_POINT ( 'NONE',  ( -18.36869280200905408, 3.942838040574673464, 12.91355658646968685 ) ) ;
#35771=ADVANCED_FACE ( 'NONE', ( #46250 ), #60533, .T. ) ;
#35772=ORIENTED_EDGE ( 'NONE', *, *, #42650, .F. ) ;
#35773=CARTESIAN_POINT ( 'NONE',  ( 35.00000000000000000, -9.752226076388938125, -6.547236723513990775 ) ) ;
#35778=EDGE_CURVE ( 'NONE', #20776, #12091, #48971, .T. ) ;
#35779=CARTESIAN_POINT ( 'NONE',  ( -37.00000000000000711, 10.75351884295727700, -4.725891942574793170 ) ) ;
#35785=ORIENTED_EDGE ( 'NONE', *, *, #6903, .F. ) ;
#35788=ORIENTED_EDGE ( 'NONE', *, *, #57958, .T. ) ;
#35790=VECTOR ( 'NONE', #4017, 1000.000000000000000 ) ;
#35793=CARTESIAN_POINT ( 'NONE',  ( -29.54875962971174630, 0.3031974620720156444, 12.00375708844796030 ) ) ;
#35796=AXIS2_PLACEMENT_3D ( 'NONE', #9139, #25419, #39734 ) ;
#35797=ADVANCED_FACE ( 'NONE', ( #55888 ), #30594, .T. ) ;
#35800=CARTESIAN_POINT ( 'NONE',  ( -37.00000000000000711, -2.544412758415929066, 11.91791701451265340 ) ) ;
#35801=CARTESIAN_POINT ( 'NONE',  ( 24.44951845548068547, 9.131659704386734688, -7.789979626095448140 ) ) ;
#35803=CARTESIAN_POINT ( 'NONE',  ( 12.53742808369427131, 13.03983582561033927, -3.499595080473846487 ) ) ;
#35804=CARTESIAN_POINT ( 'NONE',  ( -37.00000000000000711, 10.49626516989271074, 7.238157050195668241 ) ) ;
#35807=CARTESIAN_POINT ( 'NONE',  ( 37.00000000000000711, 8.534258022646096009, -8.699265615723016154 ) ) ;
#35808=ORIENTED_EDGE ( 'NONE', *, *, #31161, .T. ) ;
#35810=ORIENTED_EDGE ( 'NONE', *, *, #53963, .T. ) ;
#35815=VERTEX_POINT ( 'NONE', #63163 ) ;
#35817=CARTESIAN_POINT ( 'NONE',  ( -30.07590672654234254, -2.992774906073117247, -11.62765303320213128 ) ) ;
#35820=EDGE_CURVE ( 'NONE', #47279, #38770, #51097, .T. ) ;
#35821=CARTESIAN_POINT ( 'NONE',  ( 29.36289517528272697, -4.666195979332560917, 11.05608984446922527 ) ) ;
#35823=CIRCLE ( 'NONE', #47685, 12.75000000000000178 ) ;
#35824=EDGE_CURVE ( 'NONE', #28364, #42839, #59585, .T. ) ;
#35825=EDGE_LOOP ( 'NONE', ( #8659, #63510, #49936, #16870 ) ) ;
#35827=EDGE_LOOP ( 'NONE', ( #20616, #49816, #42224, #62440, #49943, #39901 ) ) ;
#35830=EDGE_CURVE ( 'NONE', #53824, #32797, #1016, .T. ) ;
#35832=CARTESIAN_POINT ( 'NONE',  ( 29.23591692263869390, -7.592124157161351583, 9.304424942147701216 ) ) ;
#35833=CARTESIAN_POINT ( 'NONE',  ( -9.211673578334142576, -3.291588394019901553, 11.54079650380478483 ) ) ;
#35836=CIRCLE ( 'NONE', #15676, 5.000000000000000000 ) ;
#35837=ORIENTED_EDGE ( 'NONE', *, *, #28570, .F. ) ;
#35839=ORIENTED_EDGE ( 'NONE', *, *, #61850, .T. ) ;
#35840=FACE_OUTER_BOUND ( 'NONE', #28944, .T. ) ;
#35843=CARTESIAN_POINT ( 'NONE',  ( 9.687175622948608122, -13.48729812737142986, -0.5854820436212360146 ) ) ;
#35844=CARTESIAN_POINT ( 'NONE',  ( 35.00000000000000000, 4.705694406421931860E-17, -3.469127814946512892E-15 ) ) ;
#35845=ADVANCED_FACE ( 'NONE', ( #47549 ), #26280, .T. ) ;
#35846=DIRECTION ( 'NONE',  ( 1.000000000000000000, 0.000000000000000000, 0.000000000000000000 ) ) ;
#35847=FACE_OUTER_BOUND ( 'NONE', #57664, .T. ) ;
#35848=ORIENTED_EDGE ( 'NONE', *, *, #56293, .F. ) ;
#35850=DIRECTION ( 'NONE',  ( 1.000000000000000000, -0.000000000000000000, 0.000000000000000000 ) ) ;
#35851=ORIENTED_EDGE ( 'NONE', *, *, #31753, .T. ) ;
#35854=CARTESIAN_POINT ( 'NONE',  ( 47.00000000000000711, 4.705694406421931860E-17, -3.469127814946512892E-15 ) ) ;
#35855=ORIENTED_EDGE ( 'NONE', *, *, #12359, .F. ) ;
#35858=CARTESIAN_POINT ( 'NONE',  ( -35.00000000000000000, -3.614449339633411196, -11.17622378668010441 ) ) ;
#35859=CARTESIAN_POINT ( 'NONE',  ( 4.496966607327446575, -10.17674880801902404, -8.871149476859031324 ) ) ;
#35860=CARTESIAN_POINT ( 'NONE',  ( 35.00000000000000000, 9.896810808925392777, -7.110831038798317572 ) ) ;
#35861=ADVANCED_FACE ( 'NONE', ( #42199 ), #57869, .T. ) ;
#35862=CARTESIAN_POINT ( 'NONE',  ( 7.302528884010846433, -6.186995576375307060, 10.28474183025580047 ) ) ;
#35864=ORIENTED_EDGE ( 'NONE', *, *, #56963, .T. ) ;
#35865=LINE ( 'NONE', #5661, #33193 ) ;
#35869=ORIENTED_EDGE ( 'NONE', *, *, #42942, .F. ) ;
#35870=EDGE_LOOP ( 'NONE', ( #10439, #16451, #34825, #17848 ) ) ;
#35872=EDGE_CURVE ( 'NONE', #36323, #64793, #27577, .T. ) ;
#35873=DIRECTION ( 'NONE',  ( -1.000000000000000000, 0.000000000000000000, -0.000000000000000000 ) ) ;
#35875=CIRCLE ( 'NONE', #50758, 5.000000000000000000 ) ;
#35878=CARTESIAN_POINT ( 'NONE',  ( -35.00000000000000000, 11.66953048682404415, -3.511814412391998541 ) ) ;
#35879=VERTEX_POINT ( 'NONE', #16954 ) ;
#35880=EDGE_CURVE ( 'NONE', #38116, #886, #24549, .T. ) ;
#35882=DIRECTION ( 'NONE',  ( -0.7738190875236917732, 0.000000000000000000, 0.6334066780386838902 ) ) ;
#35883=CIRCLE ( 'NONE', #56064, 12.18649999999999878 ) ;
#35885=CARTESIAN_POINT ( 'NONE',  ( -35.00000000000000000, 11.59095880812008161, -1.903127969211228621 ) ) ;
#35886=CARTESIAN_POINT ( 'NONE',  ( -37.00000000000000711, 0.000000000000000000, 0.000000000000000000 ) ) ;
#35888=CIRCLE ( 'NONE', #62420, 5.000000000000000888 ) ;
#35890=CARTESIAN_POINT ( 'NONE',  ( -27.72177753345763307, 12.14326761761198092, -5.905282218285447193 ) ) ;
#35891=DIRECTION ( 'NONE',  ( 1.000000000000000000, 0.000000000000000000, 0.000000000000000000 ) ) ;
#35893=AXIS2_PLACEMENT_3D ( 'NONE', #27906, #48216, #7624 ) ;
#35894=ORIENTED_EDGE ( 'NONE', *, *, #40975, .F. ) ;
#35897=EDGE_LOOP ( 'NONE', ( #584, #60182, #41033, #8319 ) ) ;
#35898=CARTESIAN_POINT ( 'NONE',  ( -24.29429707091690815, -10.54430068311935464, 8.439581701646471146 ) ) ;
#35899=DIRECTION ( 'NONE',  ( 0.000000000000000000, 0.4134677391718450945, 0.9105187689795982697 ) ) ;
#35903=ORIENTED_EDGE ( 'NONE', *, *, #50243, .F. ) ;
#35904=DIRECTION ( 'NONE',  ( 1.000000000000000000, -0.000000000000000000, 0.000000000000000000 ) ) ;
#35905=DIRECTION ( 'NONE',  ( -1.000000000000000000, 0.000000000000000000, 0.000000000000000000 ) ) ;
#35906=CARTESIAN_POINT ( 'NONE',  ( 21.90174657591892071, 11.97747433400151884, -0.7349207973210698519 ) ) ;
#35908=EDGE_CURVE ( 'NONE', #42345, #15993, #63890, .T. ) ;
#35909=DIRECTION ( 'NONE',  ( -1.000000000000000000, 0.000000000000000000, 0.000000000000000000 ) ) ;
#35911=FACE_OUTER_BOUND ( 'NONE', #32666, .T. ) ;
#35914=CARTESIAN_POINT ( 'NONE',  ( 37.00000000000000711, 11.86701198550356295, -2.772148766916162632 ) ) ;
#35916=AXIS2_PLACEMENT_3D ( 'NONE', #12926, #58495, #58843 ) ;
#35917=VERTEX_POINT ( 'NONE', #58867 ) ;
#35918=CIRCLE ( 'NONE', #13627, 5.000000000000000000 ) ;
#35919=CIRCLE ( 'NONE', #7275, 12.74999999999999822 ) ;
#35920=ORIENTED_EDGE ( 'NONE', *, *, #54291, .T. ) ;
#35921=DIRECTION ( 'NONE',  ( -1.000000000000000000, 0.000000000000000000, -0.000000000000000000 ) ) ;
#35923=CARTESIAN_POINT ( 'NONE',  ( 35.00000000000000000, 8.927548052240892318, -8.295159312811890118 ) ) ;
#35924=AXIS2_PLACEMENT_3D ( 'NONE', #42185, #41211, #51875 ) ;
#35926=ORIENTED_EDGE ( 'NONE', *, *, #34216, .T. ) ;
#35929=AXIS2_PLACEMENT_3D ( 'NONE', #29443, #59386, #7880 ) ;
#35931=CARTESIAN_POINT ( 'NONE',  ( 29.51976981715666781, -4.571419055710073565, 11.09513982864076276 ) ) ;
#35933=ORIENTED_EDGE ( 'NONE', *, *, #53920, .T. ) ;
#35934=CYLINDRICAL_SURFACE ( 'NONE', #34704, 4.999999999999999112 ) ;
#35936=ORIENTED_EDGE ( 'NONE', *, *, #3982, .T. ) ;
#35940=ORIENTED_EDGE ( 'NONE', *, *, #35481, .F. ) ;
#35941=CARTESIAN_POINT ( 'NONE',  ( 36.00000000000000711, -12.16893194857552629, -3.805206332242430101 ) ) ;
#35942=VERTEX_POINT ( 'NONE', #18624 ) ;
#35943=CARTESIAN_POINT ( 'NONE',  ( 35.00000000000000000, 6.265926637539650734, 11.10408318471052347 ) ) ;
#35947=DIRECTION ( 'NONE',  ( 0.000000000000000000, 0.01356324068817998940, -0.9999080150203990547 ) ) ;
#35949=CARTESIAN_POINT ( 'NONE',  ( 22.57855258442565116, 3.026812727784649493, 11.61199400236328749 ) ) ;
#35950=VECTOR ( 'NONE', #59901, 1000.000000000000000 ) ;
#35953=DIRECTION ( 'NONE',  ( 1.000000000000000000, 0.000000000000000000, 0.000000000000000000 ) ) ;
#35954=LINE ( 'NONE', #30989, #19761 ) ;
#35955=FACE_OUTER_BOUND ( 'NONE', #8730, .T. ) ;
#35958=EDGE_CURVE ( 'NONE', #5651, #32797, #50323, .T. ) ;
#35960=ORIENTED_EDGE ( 'NONE', *, *, #58418, .T. ) ;
#35961=VECTOR ( 'NONE', #60605, 1000.000000000000000 ) ;
#35963=ORIENTED_EDGE ( 'NONE', *, *, #4440, .F. ) ;
#35964=DIRECTION ( 'NONE',  ( -1.000000000000000000, 0.000000000000000000, 0.000000000000000000 ) ) ;
#35968=CARTESIAN_POINT ( 'NONE',  ( -35.00000000000000000, 0.000000000000000000, 0.000000000000000000 ) ) ;
#35970=CARTESIAN_POINT ( 'NONE',  ( 47.00000000000000711, 4.705694406421931860E-17, -3.469127814946512892E-15 ) ) ;
#35971=CIRCLE ( 'NONE', #59344, 5.000000000000000000 ) ;
#35974=DIRECTION ( 'NONE',  ( 1.000000000000000000, 0.000000000000000000, 0.000000000000000000 ) ) ;
#35975=CIRCLE ( 'NONE', #922, 12.18649999999999878 ) ;
#35977=CARTESIAN_POINT ( 'NONE',  ( 9.575800908719084958, -13.45729701195359240, -1.072919909436246266 ) ) ;
#35978=FACE_OUTER_BOUND ( 'NONE', #16510, .T. ) ;
#35979=AXIS2_PLACEMENT_3D ( 'NONE', #5928, #27163, #26184 ) ;
#35980=CYLINDRICAL_SURFACE ( 'NONE', #36030, 5.000000000000000888 ) ;
#35982=LINE ( 'NONE', #15704, #62697 ) ;
#35983=EDGE_CURVE ( 'NONE', #25281, #19321, #63800, .T. ) ;
#35984=EDGE_CURVE ( 'NONE', #64903, #19934, #42608, .T. ) ;
#35985=CARTESIAN_POINT ( 'NONE',  ( -29.92777678363736626, -3.750539801530011985, 12.96855624952674724 ) ) ;
#35986=CARTESIAN_POINT ( 'NONE',  ( 35.00000000000000000, 4.705694406421931860E-17, -3.469127814946512892E-15 ) ) ;
#35987=CARTESIAN_POINT ( 'NONE',  ( -37.00000000000000711, -0.9416912585473466990, -12.71517666308949046 ) ) ;
#35988=DIRECTION ( 'NONE',  ( -1.000000000000000000, 0.000000000000000000, 0.000000000000000000 ) ) ;
#35990=CARTESIAN_POINT ( 'NONE',  ( -35.00000000000000000, 0.000000000000000000, 0.000000000000000000 ) ) ;
#35991=DIRECTION ( 'NONE',  ( -1.000000000000000000, -0.000000000000000000, 0.000000000000000000 ) ) ;
#35992=CARTESIAN_POINT ( 'NONE',  ( -35.00000000000000000, 10.32377448871677039, -6.475373545682193033 ) ) ;
#35994=CARTESIAN_POINT ( 'NONE',  ( -14.51082951660905529, 7.864361836847419518, 10.97323765135710261 ) ) ;
#35995=CARTESIAN_POINT ( 'NONE',  ( 19.09840580349259298, -7.043236883969886897, 11.53925104275845470 ) ) ;
#35996=ORIENTED_EDGE ( 'NONE', *, *, #25355, .F. ) ;
#35998=DIRECTION ( 'NONE',  ( -1.000000000000000000, 0.000000000000000000, 0.000000000000000000 ) ) ;
#35999=DIRECTION ( 'NONE',  ( 1.000000000000000000, 0.000000000000000000, 0.000000000000000000 ) ) ;
#36001=ORIENTED_EDGE ( 'NONE', *, *, #51205, .T. ) ;
#36002=CARTESIAN_POINT ( 'NONE',  ( -35.00000000000000000, -9.321877890560388735, -7.146664589318012517 ) ) ;
#36003=DIRECTION ( 'NONE',  ( 1.000000000000000000, 0.000000000000000000, 0.000000000000000000 ) ) ;
#36004=ORIENTED_EDGE ( 'NONE', *, *, #54965, .T. ) ;
#36005=EDGE_CURVE ( 'NONE', #13243, #15906, #9736, .T. ) ;
#36007=VERTEX_POINT ( 'NONE', #4945 ) ;
#36008=ORIENTED_EDGE ( 'NONE', *, *, #7972, .T. ) ;
#36009=EDGE_CURVE ( 'NONE', #6304, #50524, #44753, .T. ) ;
#36010=CIRCLE ( 'NONE', #46630, 12.18649999999999878 ) ;
#36016=DIRECTION ( 'NONE',  ( 0.000000000000000000, -0.01356324068817991828, 0.9999080150203990547 ) ) ;
#36024=EDGE_LOOP ( 'NONE', ( #50668, #37000, #12965, #54704 ) ) ;
#36025=CARTESIAN_POINT ( 'NONE',  ( 35.00000000000000000, -2.905556151562703082, -11.38112321385050052 ) ) ;
#36027=ORIENTED_EDGE ( 'NONE', *, *, #27240, .F. ) ;
#36028=CARTESIAN_POINT ( 'NONE',  ( 35.00000000000000000, -1.738225594540085517, -12.63095688309028475 ) ) ;
#36029=ORIENTED_EDGE ( 'NONE', *, *, #21794, .T. ) ;
#36030=AXIS2_PLACEMENT_3D ( 'NONE', #49997, #34992, #65281 ) ;
#36032=DIRECTION ( 'NONE',  ( 0.000000000000000000, -0.9847383929261599445, 0.1740410799127720953 ) ) ;
#36035=CYLINDRICAL_SURFACE ( 'NONE', #63013, 12.18650000000000055 ) ;
#36037=FACE_OUTER_BOUND ( 'NONE', #51952, .T. ) ;
#36038=DIRECTION ( 'NONE',  ( 1.000000000000000000, -0.000000000000000000, 0.000000000000000000 ) ) ;
#36042=ORIENTED_EDGE ( 'NONE', *, *, #54503, .F. ) ;
#36044=ORIENTED_EDGE ( 'NONE', *, *, #41482, .F. ) ;
#36045=ORIENTED_EDGE ( 'NONE', *, *, #54316, .T. ) ;
#36047=FACE_OUTER_BOUND ( 'NONE', #28764, .T. ) ;
#36049=CARTESIAN_POINT ( 'NONE',  ( 17.41946928281426921, -8.203725127357042624, 8.773628054256990438 ) ) ;
#36051=DIRECTION ( 'NONE',  ( 0.000000000000000000, 0.01356324068817998940, -0.9999080150203989437 ) ) ;
#36052=VECTOR ( 'NONE', #20875, 1000.000000000000000 ) ;
#36053=VECTOR ( 'NONE', #21783, 1000.000000000000000 ) ;
#36054=CARTESIAN_POINT ( 'NONE',  ( 22.88594695219327235, 3.421158645304719137, -11.50198563395279194 ) ) ;
#36056=ORIENTED_EDGE ( 'NONE', *, *, #35958, .T. ) ;
#36059=CARTESIAN_POINT ( 'NONE',  ( -2.788988918599723199, -8.522892352054020293, 10.47550790974846358 ) ) ;
#36061=CARTESIAN_POINT ( 'NONE',  ( 37.00000000000000711, 4.705694406421931860E-17, -3.469127814946512892E-15 ) ) ;
#36064=ADVANCED_FACE ( 'NONE', ( #24556 ), #55473, .T. ) ;
#36065=DIRECTION ( 'NONE',  ( 1.000000000000000000, -0.000000000000000000, -0.000000000000000000 ) ) ;
#36066=CARTESIAN_POINT ( 'NONE',  ( 10.62525021964948913, 0.6055412984861371362, -11.98539912922879758 ) ) ;
#36070=DIRECTION ( 'NONE',  ( 1.000000000000000000, -0.000000000000000000, 0.000000000000000000 ) ) ;
#36073=CARTESIAN_POINT ( 'NONE',  ( 12.27843880161849199, 0.5230167770466689348, -13.48988925457417842 ) ) ;
#36074=CARTESIAN_POINT ( 'NONE',  ( 37.00000000000000711, 4.705694406421931860E-17, -3.469127814946512892E-15 ) ) ;
#36075=ORIENTED_EDGE ( 'NONE', *, *, #23684, .F. ) ;
#36076=CARTESIAN_POINT ( 'NONE',  ( -17.63187738893816814, -5.505153328604047935, -12.32741040139104349 ) ) ;
#36077=DIRECTION ( 'NONE',  ( -1.000000000000000000, 0.000000000000000000, 0.000000000000000000 ) ) ;
#36079=ORIENTED_EDGE ( 'NONE', *, *, #13789, .F. ) ;
#36080=CARTESIAN_POINT ( 'NONE',  ( -35.00000000000000000, 0.000000000000000000, 0.000000000000000000 ) ) ;
#36081=CARTESIAN_POINT ( 'NONE',  ( -15.23343484266066383, 7.971175414668098647, -8.970033181536839706 ) ) ;
#36082=DIRECTION ( 'NONE',  ( 0.000000000000000000, -0.01356324068817998940, 0.9999080150203990547 ) ) ;
#36085=CARTESIAN_POINT ( 'NONE',  ( 47.00000000000000711, 4.705694406421931860E-17, -3.469127814946512892E-15 ) ) ;
#36087=CARTESIAN_POINT ( 'NONE',  ( -36.00000000000000711, -11.39945968423475264, 5.710938531231672499 ) ) ;
#36088=CIRCLE ( 'NONE', #42446, 12.18650000000000055 ) ;
#36090=FACE_OUTER_BOUND ( 'NONE', #18970, .T. ) ;
#36091=VERTEX_POINT ( 'NONE', #60452 ) ;
#36093=DIRECTION ( 'NONE',  ( -1.000000000000000000, 0.000000000000000000, 0.000000000000000000 ) ) ;
#36094=DIRECTION ( 'NONE',  ( -1.000000000000000000, 0.000000000000000000, -0.000000000000000000 ) ) ;
#36096=( BOUNDED_CURVE ( )  B_SPLINE_CURVE ( 3, ( #11790, #32072, #56948, #21694 ),
 .UNSPECIFIED., .F., .F. ) 
 B_SPLINE_CURVE_WITH_KNOTS ( ( 4, 4 ),
 ( 2.698962753596566788, 2.780459056254051209 ),
 .UNSPECIFIED. ) 
 CURVE ( )  GEOMETRIC_REPRESENTATION_ITEM ( )  RATIONAL_B_SPLINE_CURVE ( ( 1.000000000000000000, 0.9994466059659545820, 0.9994466059659545820, 1.000000000000000000 ) ) 
 REPRESENTATION_ITEM ( '' )  );
#36098=CARTESIAN_POINT ( 'NONE',  ( -17.54726996257253191, 25.00000000000000000, 3.865003848717349033 ) ) ;
#36099=ORIENTED_EDGE ( 'NONE', *, *, #27094, .F. ) ;
#36101=ORIENTED_EDGE ( 'NONE', *, *, #26282, .F. ) ;
#36103=AXIS2_PLACEMENT_3D ( 'NONE', #17575, #12550, #43144 ) ;
#36106=CARTESIAN_POINT ( 'NONE',  ( -36.00000000000000711, 9.390600770287994337, 8.624332853796092380 ) ) ;
#36107=AXIS2_PLACEMENT_3D ( 'NONE', #5888, #26147, #41411 ) ;
#36109=CARTESIAN_POINT ( 'NONE',  ( -32.16141091265169649, 25.00000000000000000, 5.384978440493686236 ) ) ;
#36110=CARTESIAN_POINT ( 'NONE',  ( -24.39340877539587993, -9.142083323587534949, 7.776330322708387754 ) ) ;
#36112=ORIENTED_EDGE ( 'NONE', *, *, #15666, .T. ) ;
#36114=CARTESIAN_POINT ( 'NONE',  ( 28.33146005156584479, -12.08694127755678416, 6.025141712200583477 ) ) ;
#36115=ORIENTED_EDGE ( 'NONE', *, *, #1755, .T. ) ;
#36116=AXIS2_PLACEMENT_3D ( 'NONE', #51118, #56083, #26170 ) ;
#36117=CARTESIAN_POINT ( 'NONE',  ( -35.00000000000000000, 11.74226168163341555, 0.3025107581131598611 ) ) ;
#36119=CARTESIAN_POINT ( 'NONE',  ( -37.00000000000000711, 0.000000000000000000, 0.000000000000000000 ) ) ;
#36120=CYLINDRICAL_SURFACE ( 'NONE', #39038, 5.000000000000000888 ) ;
#36121=EDGE_CURVE ( 'NONE', #27224, #65758, #51151, .T. ) ;
#36123=CARTESIAN_POINT ( 'NONE',  ( -35.00000000000000000, 3.916263239775508165, -11.07407352312208459 ) ) ;
#36124=DIRECTION ( 'NONE',  ( -1.000000000000000000, 0.000000000000000000, 0.000000000000000000 ) ) ;
#36127=AXIS2_PLACEMENT_3D ( 'NONE', #65383, #34781, #20505 ) ;
#36128=DIRECTION ( 'NONE',  ( -1.000000000000000000, 0.000000000000000000, -0.000000000000000000 ) ) ;
#36129=CARTESIAN_POINT ( 'NONE',  ( -35.00000000000000000, -11.78977382767499194, 4.245927698352018886 ) ) ;
#36130=CARTESIAN_POINT ( 'NONE',  ( -9.278753422987154664, 10.79879054606790767, -5.236717350350218680 ) ) ;
#36131=DIRECTION ( 'NONE',  ( 1.000000000000000000, 0.000000000000000000, -0.000000000000000000 ) ) ;
#36132=DIRECTION ( 'NONE',  ( 0.000000000000000000, 0.9970832820307041766, 0.07632122047556146038 ) ) ;
#36133=CARTESIAN_POINT ( 'NONE',  ( -35.00000000000000000, -10.70999494708497046, 5.814360711498253842 ) ) ;
#36137=CIRCLE ( 'NONE', #26616, 5.000000000000000888 ) ;
#36138=VECTOR ( 'NONE', #56620, 1000.000000000000000 ) ;
#36139=ORIENTED_EDGE ( 'NONE', *, *, #17851, .F. ) ;
#36140=AXIS2_PLACEMENT_3D ( 'NONE', #48716, #33728, #18475 ) ;
#36141=DIRECTION ( 'NONE',  ( -1.000000000000000000, 0.000000000000000000, 0.000000000000000000 ) ) ;
#36144=ORIENTED_EDGE ( 'NONE', *, *, #33703, .T. ) ;
#36151=ORIENTED_EDGE ( 'NONE', *, *, #22167, .F. ) ;
#36153=DIRECTION ( 'NONE',  ( 0.000000000000000000, -0.8009703041134103030, -0.5987040770935764256 ) ) ;
#36156=AXIS2_PLACEMENT_3D ( 'NONE', #41027, #35377, #61310 ) ;
#36157=EDGE_CURVE ( 'NONE', #12453, #20190, #7616, .T. ) ;
#36160=CARTESIAN_POINT ( 'NONE',  ( -35.00000000000000000, 0.000000000000000000, 0.000000000000000000 ) ) ;
#36162=VECTOR ( 'NONE', #25195, 1000.000000000000000 ) ;
#36164=VERTEX_POINT ( 'NONE', #16557 ) ;
#36168=CIRCLE ( 'NONE', #19198, 12.18650000000000233 ) ;
#36169=DIRECTION ( 'NONE',  ( -1.000000000000000000, 0.000000000000000000, 0.000000000000000000 ) ) ;
#36170=CARTESIAN_POINT ( 'NONE',  ( -35.00000000000000000, -0.7214809346827719683, -11.72397916322013245 ) ) ;
#36171=VERTEX_POINT ( 'NONE', #22524 ) ;
#36172=ORIENTED_EDGE ( 'NONE', *, *, #59381, .F. ) ;
#36173=CARTESIAN_POINT ( 'NONE',  ( -30.18541646480307250, -1.416020129149132112, 11.91616074890920096 ) ) ;
#36175=EDGE_LOOP ( 'NONE', ( #60721, #58135, #8468, #21062 ) ) ;
#36176=AXIS2_PLACEMENT_3D ( 'NONE', #29037, #45300, #19053 ) ;
#36178=CARTESIAN_POINT ( 'NONE',  ( 35.00000000000000000, -11.65554240571056077, 1.456211999474460672 ) ) ;
#36179=DIRECTION ( 'NONE',  ( 0.000000000000000000, 0.01356324068817992175, -0.9999080150203990547 ) ) ;
#36181=FACE_OUTER_BOUND ( 'NONE', #50280, .T. ) ;
#36182=CARTESIAN_POINT ( 'NONE',  ( -11.08973503868622856, -9.548835897016632046, 9.557198817210366570 ) ) ;
#36183=CARTESIAN_POINT ( 'NONE',  ( -5.440603711307418600, -0.9287262547304560023, 11.96401375240336939 ) ) ;
#36184=EDGE_LOOP ( 'NONE', ( #44627, #32670, #39356, #31606 ) ) ;
#36185=AXIS2_PLACEMENT_3D ( 'NONE', #39371, #34392, #54698 ) ;
#36188=CARTESIAN_POINT ( 'NONE',  ( -35.00000000000000000, 0.000000000000000000, 0.000000000000000000 ) ) ;
#36189=DIRECTION ( 'NONE',  ( -1.000000000000000000, 0.000000000000000000, 0.000000000000000000 ) ) ;
#36192=VECTOR ( 'NONE', #21577, 1000.000000000000000 ) ;
#36193=VERTEX_POINT ( 'NONE', #47472 ) ;
#36195=ORIENTED_EDGE ( 'NONE', *, *, #48896, .F. ) ;
#36196=CARTESIAN_POINT ( 'NONE',  ( -2.672122885467072440, -11.33640012973145694, 3.936387307894340548 ) ) ;
#36197=CARTESIAN_POINT ( 'NONE',  ( -35.00000000000000000, 0.000000000000000000, 0.000000000000000000 ) ) ;
#36199=DIRECTION ( 'NONE',  ( 0.000000000000000000, 0.01356324068817998940, -0.9999080150203990547 ) ) ;
#36201=EDGE_LOOP ( 'NONE', ( #59652, #10039, #718, #12958 ) ) ;
#36203=CARTESIAN_POINT ( 'NONE',  ( 3.337809848554626146, 5.204416062760586215, 12.45815437626194289 ) ) ;
#36204=ORIENTED_EDGE ( 'NONE', *, *, #64995, .F. ) ;
#36205=CARTESIAN_POINT ( 'NONE',  ( 35.00000000000000000, 4.705694406421931860E-17, -3.469127814946512892E-15 ) ) ;
#36209=AXIS2_PLACEMENT_3D ( 'NONE', #37103, #26166, #62369 ) ;
#36212=EDGE_CURVE ( 'NONE', #21740, #1650, #52133, .T. ) ;
#36213=AXIS2_PLACEMENT_3D ( 'NONE', #16372, #13339, #1737 ) ;
#36216=CARTESIAN_POINT ( 'NONE',  ( 35.00000000000000000, 4.705694406421931860E-17, -3.469127814946512892E-15 ) ) ;
#36217=ORIENTED_EDGE ( 'NONE', *, *, #33920, .T. ) ;
#36219=DIRECTION ( 'NONE',  ( 0.000000000000000000, -0.8369827122275401710, -0.5472293298355184188 ) ) ;
#36220=CIRCLE ( 'NONE', #39404, 12.75000000000000178 ) ;
#36222=CARTESIAN_POINT ( 'NONE',  ( -29.60265935865812637, -3.677894516095094879, -12.98940028976120509 ) ) ;
#36223=CARTESIAN_POINT ( 'NONE',  ( -3.171556313731246579, 12.42408210250854772, 5.292542471626417111 ) ) ;
#36224=CIRCLE ( 'NONE', #30913, 5.000000000000000000 ) ;
#36226=DIRECTION ( 'NONE',  ( 0.000000000000000000, 0.01356324068817992175, -0.9999080150203990547 ) ) ;
#36227=DIRECTION ( 'NONE',  ( -0.000000000000000000, -1.000000000000000000, -0.000000000000000000 ) ) ;
#36228=CIRCLE ( 'NONE', #27735, 12.74999999999999822 ) ;
#36230=EDGE_CURVE ( 'NONE', #56661, #32997, #63895, .T. ) ;
#36231=ORIENTED_EDGE ( 'NONE', *, *, #3872, .T. ) ;
#36232=DIRECTION ( 'NONE',  ( 0.000000000000000000, 0.4134677391718449280, 0.9105187689795983808 ) ) ;
#36233=AXIS2_PLACEMENT_3D ( 'NONE', #40466, #60767, #1579 ) ;
#36237=CARTESIAN_POINT ( 'NONE',  ( -35.00000000000000000, -11.74614673114904129, -0.01609748574457297438 ) ) ;
#36239=FACE_OUTER_BOUND ( 'NONE', #25401, .T. ) ;
#36240=CIRCLE ( 'NONE', #26708, 5.000000000000000888 ) ;
#36243=VERTEX_POINT ( 'NONE', #13196 ) ;
#36244=DIRECTION ( 'NONE',  ( 0.000000000000000000, -0.01356324068817991828, 0.9999080150203990547 ) ) ;
#36246=DIRECTION ( 'NONE',  ( 1.000000000000000000, 0.000000000000000000, 0.000000000000000000 ) ) ;
#36247=CARTESIAN_POINT ( 'NONE',  ( 25.05309951391468459, -10.77522019223763827, -8.132934882857099979 ) ) ;
#36248=AXIS2_PLACEMENT_3D ( 'NONE', #2083, #41984, #27344 ) ;
#36249=AXIS2_PLACEMENT_3D ( 'NONE', #51067, #25452, #55387 ) ;
#36250=VECTOR ( 'NONE', #63986, 1000.000000000000000 ) ;
#36251=EDGE_CURVE ( 'NONE', #43919, #45722, #3362, .T. ) ;
#36253=EDGE_CURVE ( 'NONE', #5722, #38595, #60679, .T. ) ;
#36254=DIRECTION ( 'NONE',  ( -1.000000000000000000, 0.000000000000000000, 0.000000000000000000 ) ) ;
#36258=EDGE_CURVE ( 'NONE', #44901, #24100, #43721, .T. ) ;
#36259=CIRCLE ( 'NONE', #5492, 12.74999999999999822 ) ;
#36262=CIRCLE ( 'NONE', #34117, 5.000000000000000888 ) ;
#36263=EDGE_CURVE ( 'NONE', #53566, #13432, #40491, .T. ) ;
#36264=ORIENTED_EDGE ( 'NONE', *, *, #56697, .F. ) ;
#36267=DIRECTION ( 'NONE',  ( -1.000000000000000000, -0.000000000000000000, 0.000000000000000000 ) ) ;
#36275=LINE ( 'NONE', #6050, #19583 ) ;
#36277=ORIENTED_EDGE ( 'NONE', *, *, #12308, .F. ) ;
#36280=DIRECTION ( 'NONE',  ( 1.000000000000000000, 0.000000000000000000, 0.000000000000000000 ) ) ;
#36281=EDGE_LOOP ( 'NONE', ( #9990, #2799, #35704, #21152 ) ) ;
#36284=CARTESIAN_POINT ( 'NONE',  ( -35.00000000000000000, -2.968224442958318665, -11.81949347079750012 ) ) ;
#36288=ORIENTED_EDGE ( 'NONE', *, *, #15879, .T. ) ;
#36289=CYLINDRICAL_SURFACE ( 'NONE', #27341, 12.18649999999999878 ) ;
#36290=ORIENTED_EDGE ( 'NONE', *, *, #38376, .T. ) ;
#36291=DIRECTION ( 'NONE',  ( 1.000000000000000000, -0.000000000000000000, -0.000000000000000000 ) ) ;
#36295=AXIS2_PLACEMENT_3D ( 'NONE', #3909, #4220, #64394 ) ;
#36297=AXIS2_PLACEMENT_3D ( 'NONE', #47964, #41974, #21719 ) ;
#36298=DIRECTION ( 'NONE',  ( 0.000000000000000000, -0.01356324068817998940, 0.9999080150203990547 ) ) ;
#36299=VECTOR ( 'NONE', #2082, 1000.000000000000000 ) ;
#36300=LINE ( 'NONE', #57253, #38271 ) ;
#36301=LINE ( 'NONE', #20360, #23992 ) ;
#36303=LINE ( 'NONE', #5085, #46964 ) ;
#36304=EDGE_LOOP ( 'NONE', ( #26741, #4746, #652, #2784 ) ) ;
#36305=CARTESIAN_POINT ( 'NONE',  ( -35.00000000000000000, -11.53507381115581687, -2.216820770815207897 ) ) ;
#36306=( BOUNDED_CURVE ( )  B_SPLINE_CURVE ( 3, ( #47740, #6203, #56400, #17150 ),
 .UNSPECIFIED., .F., .F. ) 
 B_SPLINE_CURVE_WITH_KNOTS ( ( 4, 4 ),
 ( 4.960697898119300397, 4.993371868946114844 ),
 .UNSPECIFIED. ) 
 CURVE ( )  GEOMETRIC_REPRESENTATION_ITEM ( )  RATIONAL_B_SPLINE_CURVE ( ( 1.000000000000000000, 0.9999110362812402286, 0.9999110362812402286, 1.000000000000000000 ) ) 
 REPRESENTATION_ITEM ( '' )  );
#36307=ORIENTED_EDGE ( 'NONE', *, *, #54426, .T. ) ;
#36308=CARTESIAN_POINT ( 'NONE',  ( -37.00000000000000711, 6.946017217729938409, 10.01317267707888981 ) ) ;
#36309=DIRECTION ( 'NONE',  ( -1.000000000000000000, 0.000000000000000000, 0.000000000000000000 ) ) ;
#36313=DIRECTION ( 'NONE',  ( -1.000000000000000000, 0.000000000000000000, 0.000000000000000000 ) ) ;
#36314=DIRECTION ( 'NONE',  ( 0.000000000000000000, -0.01356324068817998940, 0.9999080150203990547 ) ) ;
#36317=AXIS2_PLACEMENT_3D ( 'NONE', #23610, #33580, #42889 ) ;
#36318=CARTESIAN_POINT ( 'NONE',  ( -35.00000000000000000, -5.143145423404362759, 11.66664283989677919 ) ) ;
#36322=CIRCLE ( 'NONE', #29960, 5.000000000000000888 ) ;
#36323=VERTEX_POINT ( 'NONE', #13503 ) ;
#36324=DIRECTION ( 'NONE',  ( 0.000000000000000000, -0.01356324068817998940, 0.9999080150203990547 ) ) ;
#36325=AXIS2_PLACEMENT_3D ( 'NONE', #415, #20684, #30636 ) ;
#36327=DIRECTION ( 'NONE',  ( 0.000000000000000000, 0.5767582926624911233, 0.8169148498130316405 ) ) ;
#36333=CARTESIAN_POINT ( 'NONE',  ( -29.68541646480307250, -1.416020129149132334, 11.91616074890920451 ) ) ;
#36334=EDGE_CURVE ( 'NONE', #2181, #41862, #36262, .T. ) ;
#36335=DIRECTION ( 'NONE',  ( 1.000000000000000000, -0.000000000000000000, 0.000000000000000000 ) ) ;
#36336=CARTESIAN_POINT ( 'NONE',  ( 8.676118928743548508, 5.971998260216028420, 12.11395822404814737 ) ) ;
#36338=CARTESIAN_POINT ( 'NONE',  ( 12.10998784662220551, 10.46621227226785322, -8.526922110106907482 ) ) ;
#36340=AXIS2_PLACEMENT_3D ( 'NONE', #45771, #50766, #20829 ) ;
#36342=EDGE_CURVE ( 'NONE', #49437, #54019, #11812, .T. ) ;
#36343=VECTOR ( 'NONE', #8148, 1000.000000000000000 ) ;
#36344=AXIS2_PLACEMENT_3D ( 'NONE', #37742, #58035, #32722 ) ;
#36345=ORIENTED_EDGE ( 'NONE', *, *, #2287, .F. ) ;
#36347=DIRECTION ( 'NONE',  ( 1.000000000000000000, 0.000000000000000000, 0.000000000000000000 ) ) ;
#36348=DIRECTION ( 'NONE',  ( 0.000000000000000000, -0.01356324068817998940, 0.9999080150203990547 ) ) ;
#36349=VERTEX_POINT ( 'NONE', #10478 ) ;
#36351=DIRECTION ( 'NONE',  ( -1.000000000000000000, 0.000000000000000000, 0.000000000000000000 ) ) ;
#36353=VERTEX_POINT ( 'NONE', #59732 ) ;
#36354=EDGE_CURVE ( 'NONE', #13375, #35130, #56452, .T. ) ;
#36355=DIRECTION ( 'NONE',  ( 0.000000000000000000, -0.4380125133594036657, 0.8989688749565127868 ) ) ;
#36359=ORIENTED_EDGE ( 'NONE', *, *, #33411, .F. ) ;
#36361=CIRCLE ( 'NONE', #60766, 5.000000000000000000 ) ;
#36363=ORIENTED_EDGE ( 'NONE', *, *, #48769, .T. ) ;
#36364=CARTESIAN_POINT ( 'NONE',  ( 36.00000000000000711, -4.237174932027312657, -12.02534193257719686 ) ) ;
#36366=CARTESIAN_POINT ( 'NONE',  ( 36.00000000000000711, -8.830544224263011444, -9.196955404009264257 ) ) ;
#36370=FACE_OUTER_BOUND ( 'NONE', #5436, .T. ) ;
#36371=AXIS2_PLACEMENT_3D ( 'NONE', #65399, #65717, #5234 ) ;
#36373=CARTESIAN_POINT ( 'NONE',  ( -17.80575138031851878, 11.79421038511453901, 2.237023554643799539 ) ) ;
#36375=ORIENTED_EDGE ( 'NONE', *, *, #6159, .F. ) ;
#36378=DIRECTION ( 'NONE',  ( 0.000000000000000000, 0.01356324068817998940, -0.9999080150203990547 ) ) ;
#36379=ORIENTED_EDGE ( 'NONE', *, *, #44826, .F. ) ;
#36382=FACE_OUTER_BOUND ( 'NONE', #12139, .T. ) ;
#36384=DIRECTION ( 'NONE',  ( -1.000000000000000000, 0.000000000000000000, 0.000000000000000000 ) ) ;
#36386=EDGE_CURVE ( 'NONE', #27622, #47144, #64935, .T. ) ;
#36387=FACE_OUTER_BOUND ( 'NONE', #56415, .T. ) ;
#36388=CARTESIAN_POINT ( 'NONE',  ( 10.57504247840390832, 8.113525156875750710, 8.843426623829298450 ) ) ;
#36389=CARTESIAN_POINT ( 'NONE',  ( -18.25006854224444908, -9.443202773001939221, -9.647586298549935435 ) ) ;
#36390=ORIENTED_EDGE ( 'NONE', *, *, #37901, .F. ) ;
#36394=CARTESIAN_POINT ( 'NONE',  ( 35.00000000000000000, -12.01765980939840439, 2.021542716731525413 ) ) ;
#36396=CIRCLE ( 'NONE', #61879, 12.74999999999999822 ) ;
#36397=ORIENTED_EDGE ( 'NONE', *, *, #21882, .T. ) ;
#36398=EDGE_CURVE ( 'NONE', #32962, #58250, #16103, .T. ) ;
#36399=FACE_OUTER_BOUND ( 'NONE', #18510, .T. ) ;
#36400=DIRECTION ( 'NONE',  ( -1.000000000000000000, 0.000000000000000000, 0.000000000000000000 ) ) ;
#36401=LINE ( 'NONE', #56711, #36053 ) ;
#36404=VECTOR ( 'NONE', #26206, 1000.000000000000000 ) ;
#36407=ORIENTED_EDGE ( 'NONE', *, *, #29710, .T. ) ;
#36409=EDGE_CURVE ( 'NONE', #34795, #55862, #20475, .T. ) ;
#36410=CARTESIAN_POINT ( 'NONE',  ( -37.00000000000000711, 11.38112321385055026, -2.905556151562505462 ) ) ;
#36413=AXIS2_PLACEMENT_3D ( 'NONE', #57477, #57814, #36849 ) ;
#36416=CARTESIAN_POINT ( 'NONE',  ( 24.23078042079723815, -1.962945746166874228, -13.35767736023731089 ) ) ;
#36417=CARTESIAN_POINT ( 'NONE',  ( 3.848470891359772494, 5.223518357594018724, -10.80573223417720108 ) ) ;
#36418=AXIS2_PLACEMENT_3D ( 'NONE', #41286, #61570, #30349 ) ;
#36419=CARTESIAN_POINT ( 'NONE',  ( 35.00000000000000000, -10.02106554660713833, -7.882940143791742571 ) ) ;
#36420=ORIENTED_EDGE ( 'NONE', *, *, #57185, .F. ) ;
#36422=CARTESIAN_POINT ( 'NONE',  ( -35.00000000000000000, 0.000000000000000000, 0.000000000000000000 ) ) ;
#36424=EDGE_CURVE ( 'NONE', #57471, #31543, #62239, .T. ) ;
#36425=ADVANCED_FACE ( 'NONE', ( #21111 ), #26436, .T. ) ;
#36426=CARTESIAN_POINT ( 'NONE',  ( -26.40204056389466913, 10.43732693397312694, 5.922310247585463650 ) ) ;
#36428=ORIENTED_EDGE ( 'NONE', *, *, #1738, .T. ) ;
#36429=CARTESIAN_POINT ( 'NONE',  ( -36.00000000000000711, 10.59380114696480391, -7.094637218249241428 ) ) ;
#36433=ADVANCED_FACE ( 'NONE', ( #846 ), #62646, .T. ) ;
#36435=CARTESIAN_POINT ( 'NONE',  ( -16.61479760455914345, 7.633023783503033677, -9.260229731437394918 ) ) ;
#36437=VECTOR ( 'NONE', #24924, 1000.000000000000000 ) ;
#36438=AXIS2_PLACEMENT_3D ( 'NONE', #52819, #7249, #2639 ) ;
#36440=ORIENTED_EDGE ( 'NONE', *, *, #57708, .F. ) ;
#36441=CARTESIAN_POINT ( 'NONE',  ( -35.00000000000000000, 12.70128625845194215, -1.113475361586357515 ) ) ;
#36442=AXIS2_PLACEMENT_3D ( 'NONE', #34041, #19430, #40015 ) ;
#36443=CIRCLE ( 'NONE', #44937, 5.000000000000000888 ) ;
#36448=CYLINDRICAL_SURFACE ( 'NONE', #33285, 5.000000000000000000 ) ;
#36449=DIRECTION ( 'NONE',  ( -1.000000000000000000, 0.000000000000000000, 0.000000000000000000 ) ) ;
#36450=CARTESIAN_POINT ( 'NONE',  ( -35.00000000000000000, 0.000000000000000000, 0.000000000000000000 ) ) ;
#36451=AXIS2_PLACEMENT_3D ( 'NONE', #38276, #33306, #63880 ) ;
#36452=DIRECTION ( 'NONE',  ( -0.000000000000000000, -1.000000000000000000, -0.000000000000000000 ) ) ;
#36454=ORIENTED_EDGE ( 'NONE', *, *, #19970, .F. ) ;
#36456=CARTESIAN_POINT ( 'NONE',  ( 24.54939449645449301, 1.221378253082901821, -11.94324836227821329 ) ) ;
#36458=VERTEX_POINT ( 'NONE', #5529 ) ;
#36461=CARTESIAN_POINT ( 'NONE',  ( 35.00000000000000000, 11.90598845858539789, 4.561791185930283099 ) ) ;
#36467=CARTESIAN_POINT ( 'NONE',  ( -24.80591845283671049, -9.916447262152498610, 6.760652199599259227 ) ) ;
#36468=FACE_BOUND ( 'NONE', #12159, .T. ) ;
#36473=ORIENTED_EDGE ( 'NONE', *, *, #5551, .F. ) ;
#36475=DIRECTION ( 'NONE',  ( -1.000000000000000000, 0.000000000000000000, 0.000000000000000000 ) ) ;
#36477=CARTESIAN_POINT ( 'NONE',  ( 22.36482863261543486, 25.00000000000000000, -0.9234811557364158707 ) ) ;
#36479=CARTESIAN_POINT ( 'NONE',  ( 37.00000000000000711, 4.705694406421931860E-17, -3.469127814946512892E-15 ) ) ;
#36481=VERTEX_POINT ( 'NONE', #36419 ) ;
#36486=AXIS2_PLACEMENT_3D ( 'NONE', #2148, #53691, #18457 ) ;
#36487=DIRECTION ( 'NONE',  ( 1.000000000000000000, 0.000000000000000000, -0.000000000000000000 ) ) ;
#36488=CARTESIAN_POINT ( 'NONE',  ( 37.00000000000000711, -2.250029553613672295, 12.54989509947652770 ) ) ;
#36490=AXIS2_PLACEMENT_3D ( 'NONE', #54947, #24698, #14379 ) ;
#36491=LINE ( 'NONE', #62725, #2206 ) ;
#36492=ADVANCED_FACE ( 'NONE', ( #46085 ), #20801, .T. ) ;
#36494=AXIS2_PLACEMENT_3D ( 'NONE', #26615, #6350, #37823 ) ;
#36496=CARTESIAN_POINT ( 'NONE',  ( 37.00000000000000711, 4.705694406421931860E-17, -3.469127814946512892E-15 ) ) ;
#36503=CARTESIAN_POINT ( 'NONE',  ( -35.00000000000000000, 0.000000000000000000, 0.000000000000000000 ) ) ;
#36507=CYLINDRICAL_SURFACE ( 'NONE', #26858, 5.000000000000000888 ) ;
#36510=EDGE_CURVE ( 'NONE', #37450, #41989, #56501, .T. ) ;
#36511=AXIS2_PLACEMENT_3D ( 'NONE', #16735, #47997, #17060 ) ;
#36515=ORIENTED_EDGE ( 'NONE', *, *, #30815, .F. ) ;
#36516=AXIS2_PLACEMENT_3D ( 'NONE', #4855, #39415, #60045 ) ;
#36517=DIRECTION ( 'NONE',  ( 0.000000000000000000, 0.01356324068817998940, -0.9999080150203990547 ) ) ;
#36521=DIRECTION ( 'NONE',  ( -1.000000000000000000, 0.000000000000000000, 0.000000000000000000 ) ) ;
#36522=CARTESIAN_POINT ( 'NONE',  ( 26.08439714455133185, -11.40113243194250359, 3.743551691817327942 ) ) ;
#36523=DIRECTION ( 'NONE',  ( -1.000000000000000000, 0.000000000000000000, 0.000000000000000000 ) ) ;
#36524=EDGE_CURVE ( 'NONE', #7826, #65529, #47067, .T. ) ;
#36526=EDGE_LOOP ( 'NONE', ( #6424, #26989, #61821, #65569 ) ) ;
#36528=DIRECTION ( 'NONE',  ( 1.000000000000000000, 0.000000000000000000, 0.000000000000000000 ) ) ;
#36530=CARTESIAN_POINT ( 'NONE',  ( 0.3534040366549966450, 0.2453052870633498916, 11.99999999999999112 ) ) ;
#36531=DIRECTION ( 'NONE',  ( 0.000000000000000000, 0.01356324068817998940, -0.9999080150203990547 ) ) ;
#36532=CYLINDRICAL_SURFACE ( 'NONE', #47983, 4.999999999999999112 ) ;
#36534=DIRECTION ( 'NONE',  ( 0.000000000000000000, 0.01356324068817998940, -0.9999080150203989437 ) ) ;
#36536=CARTESIAN_POINT ( 'NONE',  ( -9.565563870443305916, -2.937820479959865061, 11.63604098864692737 ) ) ;
#36537=ORIENTED_EDGE ( 'NONE', *, *, #52170, .T. ) ;
#36540=ORIENTED_EDGE ( 'NONE', *, *, #17502, .F. ) ;
#36541=CARTESIAN_POINT ( 'NONE',  ( 21.74721992753864441, -13.45929105453497776, -1.114420066137331133 ) ) ;
#36543=ORIENTED_EDGE ( 'NONE', *, *, #53865, .F. ) ;
#36546=ORIENTED_EDGE ( 'NONE', *, *, #50179, .F. ) ;
#36547=CARTESIAN_POINT ( 'NONE',  ( 47.00000000000000711, 4.705694406421931860E-17, -3.469127814946512892E-15 ) ) ;
#36551=CARTESIAN_POINT ( 'NONE',  ( 35.00000000000000000, -9.913596905230168232, -8.017674001891750279 ) ) ;
#36552=ORIENTED_EDGE ( 'NONE', *, *, #31510, .F. ) ;
#36555=EDGE_CURVE ( 'NONE', #34975, #19210, #38377, .T. ) ;
#36557=DIRECTION ( 'NONE',  ( -1.000000000000000000, 0.000000000000000000, 0.000000000000000000 ) ) ;
#36558=ORIENTED_EDGE ( 'NONE', *, *, #27900, .F. ) ;
#36559=ORIENTED_EDGE ( 'NONE', *, *, #12308, .T. ) ;
#36561=CARTESIAN_POINT ( 'NONE',  ( -35.00000000000000000, 6.657191900728318679, 9.677500615117924809 ) ) ;
#36562=AXIS2_PLACEMENT_3D ( 'NONE', #12124, #7134, #27414 ) ;
#36566=EDGE_CURVE ( 'NONE', #63705, #49222, #16189, .T. ) ;
#36567=DIRECTION ( 'NONE',  ( 0.000000000000000000, 0.01356324068817998940, -0.9999080150203990547 ) ) ;
#36568=ORIENTED_EDGE ( 'NONE', *, *, #1859, .F. ) ;
#36569=CARTESIAN_POINT ( 'NONE',  ( 16.94767514662584418, 12.18332229639727160, 5.815258616132746639 ) ) ;
#36570=VERTEX_POINT ( 'NONE', #39033 ) ;
#36577=CARTESIAN_POINT ( 'NONE',  ( 29.23580817562944745, 7.598662642114378585, 9.298966629028747377 ) ) ;
#36578=AXIS2_PLACEMENT_3D ( 'NONE', #12514, #13195, #48780 ) ;
#36579=DIRECTION ( 'NONE',  ( 1.000000000000000000, 0.000000000000000000, 0.000000000000000000 ) ) ;
#36582=CARTESIAN_POINT ( 'NONE',  ( -35.00000000000000000, 12.15823808070322798, 0.8294751490779768144 ) ) ;
#36583=ORIENTED_EDGE ( 'NONE', *, *, #51284, .T. ) ;
#36588=CYLINDRICAL_SURFACE ( 'NONE', #15827, 4.000030059823568074 ) ;
#36590=AXIS2_PLACEMENT_3D ( 'NONE', #5811, #50031, #5135 ) ;
#36592=CARTESIAN_POINT ( 'NONE',  ( -35.00000000000000000, 5.273331777780488672, -10.49591321039675229 ) ) ;
#36594=LINE ( 'NONE', #61516, #35352 ) ;
#36596=LINE ( 'NONE', #26291, #63720 ) ;
#36597=LINE ( 'NONE', #21645, #39167 ) ;
#36598=CARTESIAN_POINT ( 'NONE',  ( 35.00000000000000000, 10.62137734850267989, 5.015831474386340361 ) ) ;
#36600=AXIS2_PLACEMENT_3D ( 'NONE', #29042, #49351, #3797 ) ;
#36603=EDGE_CURVE ( 'NONE', #59070, #7715, #59324, .T. ) ;
#36611=VERTEX_POINT ( 'NONE', #28092 ) ;
#36612=ORIENTED_EDGE ( 'NONE', *, *, #18240, .F. ) ;
#36613=CARTESIAN_POINT ( 'NONE',  ( 35.00000000000000000, 9.908974237959730758, 6.307491713048920090 ) ) ;
#36617=ORIENTED_EDGE ( 'NONE', *, *, #52044, .F. ) ;
#36619=DIRECTION ( 'NONE',  ( -1.000000000000000000, -0.000000000000000000, 0.000000000000000000 ) ) ;
#36620=VERTEX_POINT ( 'NONE', #53361 ) ;
#36622=EDGE_CURVE ( 'NONE', #15993, #41767, #45498, .T. ) ;
#36624=CARTESIAN_POINT ( 'NONE',  ( 24.88498457265327346, -1.132774965307099979, 11.94809602833619699 ) ) ;
#36625=ORIENTED_EDGE ( 'NONE', *, *, #24094, .F. ) ;
#36626=DIRECTION ( 'NONE',  ( -1.000000000000000000, -0.000000000000000000, 0.000000000000000000 ) ) ;
#36627=EDGE_CURVE ( 'NONE', #63262, #14422, #34037, .T. ) ;
#36628=B_SPLINE_CURVE_WITH_KNOTS ( 'NONE', 3,
 ( #47766, #22836, #42098, #52446, #62081, #37114, #57416, #43091, #16532, #32452, #46778, #27155, #56788, #63367, #17177, #11846, #53078, #32127 ),
 .UNSPECIFIED., .F., .F.,
 ( 4, 2, 2, 2, 2, 2, 2, 2, 4 ),
 ( 0.004326619632261259271, 0.005066079377112942678, 0.005805539121964627819, 0.006544998866816312960, 0.007284458611667997234, 0.008023918356519681508, 0.008763378101371366649, 0.009502837846223051790, 0.01024229759107473693 ),
 .UNSPECIFIED. ) ;
#36629=ORIENTED_EDGE ( 'NONE', *, *, #64470, .F. ) ;
#36630=AXIS2_PLACEMENT_3D ( 'NONE', #1639, #19705, #39639 ) ;
#36631=FACE_OUTER_BOUND ( 'NONE', #31802, .T. ) ;
#36634=FACE_OUTER_BOUND ( 'NONE', #32610, .T. ) ;
#36635=DIRECTION ( 'NONE',  ( 0.000000000000000000, 0.01356324068818000848, -0.9999080150203990547 ) ) ;
#36636=CARTESIAN_POINT ( 'NONE',  ( 9.746551792753381349, 1.290882055502603931, 11.93221949516759750 ) ) ;
#36637=ADVANCED_FACE ( 'NONE', ( #30037 ), #50005, .T. ) ;
#36638=CARTESIAN_POINT ( 'NONE',  ( -30.18541646480307250, -2.213624975795535299, -13.34140603515871604 ) ) ;
#36639=CARTESIAN_POINT ( 'NONE',  ( 8.500415212161144041, 5.252658130439442630, -10.79141609758813480 ) ) ;
#36640=VERTEX_POINT ( 'NONE', #40673 ) ;
#36642=CIRCLE ( 'NONE', #46245, 4.999999999999999112 ) ;
#36643=VERTEX_POINT ( 'NONE', #25376 ) ;
#36644=FACE_OUTER_BOUND ( 'NONE', #45784, .T. ) ;
#36645=EDGE_CURVE ( 'NONE', #25311, #64820, #35260, .T. ) ;
#36646=CARTESIAN_POINT ( 'NONE',  ( 37.00000000000000711, 11.70009620280413110, 1.039216533672774112 ) ) ;
#36649=FACE_OUTER_BOUND ( 'NONE', #58925, .T. ) ;
#36650=CYLINDRICAL_SURFACE ( 'NONE', #33346, 6.595312090839647645 ) ;
#36652=CIRCLE ( 'NONE', #2699, 5.000000000000000888 ) ;
#36657=ORIENTED_EDGE ( 'NONE', *, *, #32266, .F. ) ;
#36660=DIRECTION ( 'NONE',  ( 0.000000000000000000, 0.01356324068817998940, -0.9999080150203989437 ) ) ;
#36662=ORIENTED_EDGE ( 'NONE', *, *, #18479, .T. ) ;
#36664=VECTOR ( 'NONE', #60959, 1000.000000000000000 ) ;
#36665=CARTESIAN_POINT ( 'NONE',  ( 29.10724821778045168, 10.83570424563273882, 8.063006356801381003 ) ) ;
#36667=DIRECTION ( 'NONE',  ( 1.000000000000000000, 0.000000000000000000, 0.000000000000000000 ) ) ;
#36668=CARTESIAN_POINT ( 'NONE',  ( 9.166623160528491354, 6.959806824555357707, 11.57358056643181676 ) ) ;
#36669=DIRECTION ( 'NONE',  ( -1.000000000000000000, 0.000000000000000000, -0.000000000000000000 ) ) ;
#36672=EDGE_CURVE ( 'NONE', #2417, #57580, #28874, .T. ) ;
#36673=ORIENTED_EDGE ( 'NONE', *, *, #7126, .T. ) ;
#36674=DIRECTION ( 'NONE',  ( 0.000000000000000000, 0.8696919319575202589, 0.4935949184179230231 ) ) ;
#36676=CIRCLE ( 'NONE', #12235, 5.000000000000000000 ) ;
#36677=EDGE_LOOP ( 'NONE', ( #23642, #56149, #24236, #51719 ) ) ;
#36678=DIRECTION ( 'NONE',  ( -0.000000000000000000, -0.000000000000000000, -1.000000000000000000 ) ) ;
#36679=CARTESIAN_POINT ( 'NONE',  ( 3.353434147978485047, 5.295522092567586547, -10.77037561067536053 ) ) ;
#36680=CARTESIAN_POINT ( 'NONE',  ( -7.971178810570282103, 8.542040713314987599, -10.47297027589238816 ) ) ;
#36681=VERTEX_POINT ( 'NONE', #3824 ) ;
#36683=ORIENTED_EDGE ( 'NONE', *, *, #5192, .F. ) ;
#36684=EDGE_CURVE ( 'NONE', #41624, #36171, #3413, .T. ) ;
#36686=ORIENTED_EDGE ( 'NONE', *, *, #49325, .T. ) ;
#36688=AXIS2_PLACEMENT_3D ( 'NONE', #26317, #16667, #7022 ) ;
#36691=ORIENTED_EDGE ( 'NONE', *, *, #34790, .F. ) ;
#36692=CARTESIAN_POINT ( 'NONE',  ( -25.68896891816097039, -10.12442625007511232, 6.443155052333052524 ) ) ;
#36694=DIRECTION ( 'NONE',  ( 0.000000000000000000, -0.7617968321374810614, -0.6478160128812026075 ) ) ;
#36695=CARTESIAN_POINT ( 'NONE',  ( 9.588299228810004848, 6.688210644983048958, 9.969111302884179793 ) ) ;
#36696=ORIENTED_EDGE ( 'NONE', *, *, #13430, .F. ) ;
#36700=CARTESIAN_POINT ( 'NONE',  ( -36.00000000000000711, -3.805206332242558886, 12.16893194857548899 ) ) ;
#36702=VERTEX_POINT ( 'NONE', #4122 ) ;
#36703=DIRECTION ( 'NONE',  ( 1.000000000000000000, 0.000000000000000000, -0.000000000000000000 ) ) ;
#36705=VERTEX_POINT ( 'NONE', #65287 ) ;
#36707=EDGE_LOOP ( 'NONE', ( #35125, #26877, #59276, #13634 ) ) ;
#36709=DIRECTION ( 'NONE',  ( -1.000000000000000000, -0.000000000000000000, 0.000000000000000000 ) ) ;
#36711=VECTOR ( 'NONE', #49833, 1000.000000000000000 ) ;
#36714=CARTESIAN_POINT ( 'NONE',  ( -47.00000000000000711, 0.000000000000000000, 0.000000000000000000 ) ) ;
#36717=ORIENTED_EDGE ( 'NONE', *, *, #25004, .T. ) ;
#36719=FACE_OUTER_BOUND ( 'NONE', #42663, .T. ) ;
#36720=ORIENTED_EDGE ( 'NONE', *, *, #49929, .F. ) ;
#36721=EDGE_CURVE ( 'NONE', #6288, #24332, #40540, .T. ) ;
#36722=EDGE_CURVE ( 'NONE', #18994, #30591, #49068, .T. ) ;
#36724=DIRECTION ( 'NONE',  ( 1.000000000000000000, 0.000000000000000000, 0.000000000000000000 ) ) ;
#36725=CYLINDRICAL_SURFACE ( 'NONE', #63599, 4.999999999999999112 ) ;
#36728=EDGE_CURVE ( 'NONE', #56510, #45342, #4798, .T. ) ;
#36729=DIRECTION ( 'NONE',  ( 0.000000000000000000, 0.9467777615094560284, 0.3218879778916007295 ) ) ;
#36730=CYLINDRICAL_SURFACE ( 'NONE', #47972, 12.18649999999999878 ) ;
#36731=CIRCLE ( 'NONE', #4891, 12.18649999999999878 ) ;
#36732=ADVANCED_FACE ( 'NONE', ( #35672 ), #26049, .T. ) ;
#36733=LINE ( 'NONE', #47382, #38547 ) ;
#36734=EDGE_CURVE ( 'NONE', #45182, #18937, #11389, .T. ) ;
#36736=ORIENTED_EDGE ( 'NONE', *, *, #34401, .F. ) ;
#36737=EDGE_CURVE ( 'NONE', #1560, #16664, #7364, .T. ) ;
#36738=FACE_OUTER_BOUND ( 'NONE', #6194, .T. ) ;
#36739=CARTESIAN_POINT ( 'NONE',  ( -2.952869152607111136, -4.384817011589735358, 11.17020052527586138 ) ) ;
#36742=FACE_OUTER_BOUND ( 'NONE', #64960, .T. ) ;
#36743=CARTESIAN_POINT ( 'NONE',  ( 16.94767514662583352, -12.18332229639725206, 5.815258616132748415 ) ) ;
#36744=CARTESIAN_POINT ( 'NONE',  ( 3.941273214955026472, 6.020113200743838711, -10.38315790873123134 ) ) ;
#36745=DIRECTION ( 'NONE',  ( 0.000000000000000000, 0.01356324068817998940, -0.9999080150203990547 ) ) ;
#36746=ORIENTED_EDGE ( 'NONE', *, *, #50736, .F. ) ;
#36747=CARTESIAN_POINT ( 'NONE',  ( -37.00000000000000711, -10.25474254703948418, -6.584150480049660636 ) ) ;
#36750=DIRECTION ( 'NONE',  ( -1.000000000000000000, -1.836970198721029688E-16, 0.000000000000000000 ) ) ;
#36751=B_SPLINE_CURVE_WITH_KNOTS ( 'NONE', 3,
 ( #34448, #60056, #39101, #9484, #8856, #59729, #45090, #18538, #29149, #23843, #38792, #18840, #3885, #44103, #14794, #59395, #65355, #64685, #34105, #24146, #14156, #29768 ),
 .UNSPECIFIED., .F., .F.,
 ( 4, 2, 2, 2, 2, 2, 2, 2, 2, 2, 4 ),
 ( 0.003235587836267140010, 0.004470998178832687707, 0.005088703350115462640, 0.005706408521398236705, 0.006941818863963784836, 0.008177229206529331232, 0.009412639549094879363, 0.01064804989166042749, 0.01126575506294320156, 0.01188346023422597736, 0.01311887057679152896 ),
 .UNSPECIFIED. ) ;
#36752=EDGE_CURVE ( 'NONE', #33727, #16920, #20380, .T. ) ;
#36753=CARTESIAN_POINT ( 'NONE',  ( 8.957787800376372900, 4.005583820372585535, -12.89440042502234363 ) ) ;
#36754=CARTESIAN_POINT ( 'NONE',  ( -35.00000000000000000, -4.339012074900030491, 10.91536515067646818 ) ) ;
#36755=ORIENTED_EDGE ( 'NONE', *, *, #37931, .F. ) ;
#36756=CARTESIAN_POINT ( 'NONE',  ( -19.47984447937493613, -3.750539801530005768, -12.96855624952674724 ) ) ;
#36757=CYLINDRICAL_SURFACE ( 'NONE', #46050, 4.445031439545090279 ) ;
#36759=VERTEX_POINT ( 'NONE', #35987 ) ;
#36761=CARTESIAN_POINT ( 'NONE',  ( -15.47675659650424329, 7.964312849573895292, -8.976208599246165321 ) ) ;
#36763=EDGE_CURVE ( 'NONE', #50717, #54601, #19345, .T. ) ;
#36764=CYLINDRICAL_SURFACE ( 'NONE', #65724, 4.999999999999999112 ) ;
#36765=VERTEX_POINT ( 'NONE', #16045 ) ;
#36768=AXIS2_PLACEMENT_3D ( 'NONE', #17736, #63583, #8400 ) ;
#36769=CYLINDRICAL_SURFACE ( 'NONE', #18104, 5.000000000000000888 ) ;
#36770=ORIENTED_EDGE ( 'NONE', *, *, #38371, .F. ) ;
#36771=DIRECTION ( 'NONE',  ( 0.000000000000000000, -0.01356324068817998940, 0.9999080150203990547 ) ) ;
#36772=DIRECTION ( 'NONE',  ( 0.000000000000000000, -0.01356324068817998940, 0.9999080150203990547 ) ) ;
#36773=CARTESIAN_POINT ( 'NONE',  ( 35.00000000000000000, 5.814360711498443912, 10.70999494708485678 ) ) ;
#36774=AXIS2_PLACEMENT_3D ( 'NONE', #52642, #7066, #11711 ) ;
#36775=DIRECTION ( 'NONE',  ( -1.000000000000000000, -0.000000000000000000, 0.000000000000000000 ) ) ;
#36776=PLANE ( 'NONE',  #20399 ) ;
#36777=CARTESIAN_POINT ( 'NONE',  ( 35.00000000000000000, 11.73463472867580393, 3.287724142101285274 ) ) ;
#36779=ORIENTED_EDGE ( 'NONE', *, *, #65600, .T. ) ;
#36780=EDGE_CURVE ( 'NONE', #54418, #65236, #17198, .T. ) ;
#36781=EDGE_LOOP ( 'NONE', ( #44747, #40053, #14388, #5286 ) ) ;
#36783=EDGE_LOOP ( 'NONE', ( #5513, #11649, #48251, #38569 ) ) ;
#36785=EDGE_CURVE ( 'NONE', #65370, #32930, #36322, .T. ) ;
#36789=CYLINDRICAL_SURFACE ( 'NONE', #11807, 12.18650000000000055 ) ;
#36793=DIRECTION ( 'NONE',  ( 0.000000000000000000, -0.9796553971857762111, -0.2006870767258790988 ) ) ;
#36794=ORIENTED_EDGE ( 'NONE', *, *, #46641, .F. ) ;
#36795=VERTEX_POINT ( 'NONE', #51657 ) ;
#36796=CARTESIAN_POINT ( 'NONE',  ( 28.67692623539176466, -11.72617184382499644, 6.700251934688060018 ) ) ;
#36798=DIRECTION ( 'NONE',  ( 0.000000000000000000, 0.01356324068817998940, -0.9999080150203989437 ) ) ;
#36800=DIRECTION ( 'NONE',  ( 1.000000000000000000, -0.000000000000000000, 0.000000000000000000 ) ) ;
#36801=ADVANCED_FACE ( 'NONE', ( #6101 ), #16707, .T. ) ;
#36803=DIRECTION ( 'NONE',  ( 0.000000000000000000, -0.01356324068818000328, 0.9999080150203990547 ) ) ;
#36805=EDGE_CURVE ( 'NONE', #28625, #29524, #46644, .T. ) ;
#36806=LINE ( 'NONE', #52107, #411 ) ;
#36807=ORIENTED_EDGE ( 'NONE', *, *, #58622, .T. ) ;
#36808=DIRECTION ( 'NONE',  ( 0.000000000000000000, 0.01356324068817998940, -0.9999080150203990547 ) ) ;
#36809=ORIENTED_EDGE ( 'NONE', *, *, #10181, .F. ) ;
#36810=EDGE_CURVE ( 'NONE', #58284, #33621, #16145, .T. ) ;
#36812=CARTESIAN_POINT ( 'NONE',  ( -1.734723475976807094E-15, -3.469446951953614189E-15, 25.00000000000000000 ) ) ;
#36814=CARTESIAN_POINT ( 'NONE',  ( -35.00000000000000000, 1.113475361586490298, 12.70128625845193326 ) ) ;
#36815=DIRECTION ( 'NONE',  ( 0.000000000000000000, 0.3218879778915972878, -0.9467777615094571386 ) ) ;
#36816=VECTOR ( 'NONE', #52091, 1000.000000000000000 ) ;
#36817=CYLINDRICAL_SURFACE ( 'NONE', #51054, 5.000000000000000888 ) ;
#36818=ORIENTED_EDGE ( 'NONE', *, *, #65487, .F. ) ;
#36819=VERTEX_POINT ( 'NONE', #40999 ) ;
#36820=LINE ( 'NONE', #15222, #62000 ) ;
#36824=CARTESIAN_POINT ( 'NONE',  ( -36.00000000000000711, -9.506317355798310942, -8.496612874013262484 ) ) ;
#36829=LINE ( 'NONE', #5949, #36404 ) ;
#36830=CARTESIAN_POINT ( 'NONE',  ( -37.00000000000000711, 10.54834585426219995, 6.102719229070713070 ) ) ;
#36837=ORIENTED_EDGE ( 'NONE', *, *, #12276, .F. ) ;
#36838=DIRECTION ( 'NONE',  ( 1.000000000000000000, 0.000000000000000000, 0.000000000000000000 ) ) ;
#36840=DIRECTION ( 'NONE',  ( 0.000000000000000000, 0.01356324068817998940, -0.9999080150203990547 ) ) ;
#36841=EDGE_CURVE ( 'NONE', #9063, #65109, #58666, .T. ) ;
#36843=CARTESIAN_POINT ( 'NONE',  ( -37.00000000000000711, 1.463443770872774774, 12.09831040184924866 ) ) ;
#36844=ORIENTED_EDGE ( 'NONE', *, *, #53702, .F. ) ;
#36845=ORIENTED_EDGE ( 'NONE', *, *, #9606, .F. ) ;
#36847=ORIENTED_EDGE ( 'NONE', *, *, #56783, .F. ) ;
#36848=DIRECTION ( 'NONE',  ( -1.000000000000000000, 0.000000000000000000, 0.000000000000000000 ) ) ;
#36849=DIRECTION ( 'NONE',  ( 0.000000000000000000, 0.01356324068817998940, -0.9999080150203990547 ) ) ;
#36850=DIRECTION ( 'NONE',  ( -1.000000000000000000, -0.000000000000000000, 0.000000000000000000 ) ) ;
#36851=AXIS2_PLACEMENT_3D ( 'NONE', #14700, #49361, #59306 ) ;
#36852=CARTESIAN_POINT ( 'NONE',  ( -37.00000000000000711, 8.389074212634413996, -8.839356091079956457 ) ) ;
#36854=CARTESIAN_POINT ( 'NONE',  ( 10.48620311856346454, 8.250315036047107142, -8.713914264323181058 ) ) ;
#36856=EDGE_LOOP ( 'NONE', ( #2783, #38508, #37081, #52623 ) ) ;
#36858=EDGE_CURVE ( 'NONE', #52549, #46634, #60651, .T. ) ;
#36860=VERTEX_POINT ( 'NONE', #21375 ) ;
#36862=CARTESIAN_POINT ( 'NONE',  ( 35.00000000000000000, 4.705694406421931860E-17, -3.469127814946512892E-15 ) ) ;
#36864=CARTESIAN_POINT ( 'NONE',  ( 35.00000000000000000, -1.457575200925456560, 12.66641127287626745 ) ) ;
#36865=DIRECTION ( 'NONE',  ( -1.000000000000000000, -0.000000000000000000, 0.000000000000000000 ) ) ;
#36868=ORIENTED_EDGE ( 'NONE', *, *, #55336, .T. ) ;
#36870=CARTESIAN_POINT ( 'NONE',  ( 47.00000000000000711, 4.705694406421931860E-17, -3.469127814946512892E-15 ) ) ;
#36872=VERTEX_POINT ( 'NONE', #26693 ) ;
#36874=ORIENTED_EDGE ( 'NONE', *, *, #52021, .T. ) ;
#36875=CARTESIAN_POINT ( 'NONE',  ( -37.00000000000000711, 0.000000000000000000, 0.000000000000000000 ) ) ;
#36876=ORIENTED_EDGE ( 'NONE', *, *, #947, .T. ) ;
#36877=ORIENTED_EDGE ( 'NONE', *, *, #57708, .T. ) ;
#36879=VERTEX_POINT ( 'NONE', #37315 ) ;
#36881=EDGE_CURVE ( 'NONE', #40269, #53819, #52824, .T. ) ;
#36882=DIRECTION ( 'NONE',  ( 0.000000000000000000, 0.01356324068817998940, -0.9999080150203990547 ) ) ;
#36884=DIRECTION ( 'NONE',  ( -1.000000000000000000, 0.000000000000000000, 0.000000000000000000 ) ) ;
#36885=DIRECTION ( 'NONE',  ( -1.000000000000000000, 0.000000000000000000, -0.000000000000000000 ) ) ;
#36886=VERTEX_POINT ( 'NONE', #7062 ) ;
#36887=EDGE_CURVE ( 'NONE', #20614, #24790, #18373, .T. ) ;
#36888=DIRECTION ( 'NONE',  ( 0.000000000000000000, -0.2355298848897378061, -0.9718671068226493182 ) ) ;
#36889=( BOUNDED_CURVE ( )  B_SPLINE_CURVE ( 3, ( #12838, #58760, #49106, #18527 ),
 .UNSPECIFIED., .F., .F. ) 
 B_SPLINE_CURVE_WITH_KNOTS ( ( 4, 4 ),
 ( 1.845784941385602673, 1.860835188181379163 ),
 .UNSPECIFIED. ) 
 CURVE ( )  GEOMETRIC_REPRESENTATION_ITEM ( )  RATIONAL_B_SPLINE_CURVE ( ( 1.000000000000000000, 0.9999811242616895024, 0.9999811242616895024, 1.000000000000000000 ) ) 
 REPRESENTATION_ITEM ( '' )  );
#36890=VERTEX_POINT ( 'NONE', #27336 ) ;
#36891=CYLINDRICAL_SURFACE ( 'NONE', #4022, 12.18649999999999878 ) ;
#36893=LINE ( 'NONE', #59973, #16119 ) ;
#36894=FACE_OUTER_BOUND ( 'NONE', #40219, .T. ) ;
#36896=CARTESIAN_POINT ( 'NONE',  ( -32.00000000000000711, 5.510910596163084625E-16, 0.000000000000000000 ) ) ;
#36897=ORIENTED_EDGE ( 'NONE', *, *, #50082, .F. ) ;
#36903=DIRECTION ( 'NONE',  ( 0.000000000000000000, 0.01356324068817998940, -0.9999080150203990547 ) ) ;
#36904=DIRECTION ( 'NONE',  ( 0.000000000000000000, 0.6943713148249588407, -0.7196168960969843154 ) ) ;
#36907=DIRECTION ( 'NONE',  ( 1.000000000000000000, 0.000000000000000000, 0.000000000000000000 ) ) ;
#36908=LINE ( 'NONE', #51580, #58881 ) ;
#36909=LINE ( 'NONE', #41233, #60866 ) ;
#36910=AXIS2_PLACEMENT_3D ( 'NONE', #49101, #2891, #8185 ) ;
#36911=CARTESIAN_POINT ( 'NONE',  ( 26.34661844826604593, 11.53221627053869369, 3.317828791472333005 ) ) ;
#36912=CIRCLE ( 'NONE', #56034, 12.18650000000000055 ) ;
#36917=EDGE_CURVE ( 'NONE', #9409, #50465, #57952, .T. ) ;
#36918=EDGE_LOOP ( 'NONE', ( #41994, #24624, #32906, #40553 ) ) ;
#36920=ORIENTED_EDGE ( 'NONE', *, *, #21862, .F. ) ;
#36923=CARTESIAN_POINT ( 'NONE',  ( -29.58156646296218995, -2.915657712021824111, 13.18682379069277388 ) ) ;
#36924=CYLINDRICAL_SURFACE ( 'NONE', #59437, 5.000000000000000888 ) ;
#36925=ORIENTED_EDGE ( 'NONE', *, *, #17776, .F. ) ;
#36930=CIRCLE ( 'NONE', #8281, 5.000000000000000000 ) ;
#36931=CARTESIAN_POINT ( 'NONE',  ( 21.90174657591892071, 11.97747433400151884, -0.7349207973210698519 ) ) ;
#36934=DIRECTION ( 'NONE',  ( 0.000000000000000000, 0.01356324068817992175, -0.9999080150203990547 ) ) ;
#36936=VERTEX_POINT ( 'NONE', #43606 ) ;
#36937=DIRECTION ( 'NONE',  ( 1.000000000000000000, 0.000000000000000000, 0.000000000000000000 ) ) ;
#36940=CARTESIAN_POINT ( 'NONE',  ( 23.48109318918174182, 2.900249156073090528, 11.64847700441486467 ) ) ;
#36941=ORIENTED_EDGE ( 'NONE', *, *, #25509, .T. ) ;
#36942=DIRECTION ( 'NONE',  ( -0.000000000000000000, -0.000000000000000000, -1.000000000000000000 ) ) ;
#36943=ORIENTED_EDGE ( 'NONE', *, *, #13601, .T. ) ;
#36945=CARTESIAN_POINT ( 'NONE',  ( -17.81734942214415440, -8.644007148549530228, 10.38604278132294922 ) ) ;
#36947=DIRECTION ( 'NONE',  ( 1.000000000000000000, 0.000000000000000000, 0.000000000000000000 ) ) ;
#36951=CARTESIAN_POINT ( 'NONE',  ( 8.821156950359336335, 6.332123185147309208, -10.20069656434953131 ) ) ;
#36952=VERTEX_POINT ( 'NONE', #28331 ) ;
#36953=CARTESIAN_POINT ( 'NONE',  ( 35.00000000000000000, 4.705694406421931860E-17, -3.469127814946512892E-15 ) ) ;
#36954=EDGE_LOOP ( 'NONE', ( #53705, #40430, #16737, #32221 ) ) ;
#36955=CARTESIAN_POINT ( 'NONE',  ( -35.00000000000000000, 7.376655759825023750, -9.700295462048581285 ) ) ;
#36956=DIRECTION ( 'NONE',  ( 0.000000000000000000, -0.6943713148249532896, 0.7196168960969895334 ) ) ;
#36958=ORIENTED_EDGE ( 'NONE', *, *, #45542, .T. ) ;
#36961=DIRECTION ( 'NONE',  ( -1.000000000000000000, 0.000000000000000000, 0.000000000000000000 ) ) ;
#36963=EDGE_LOOP ( 'NONE', ( #19358, #52128, #29403, #44698 ) ) ;
#36964=EDGE_CURVE ( 'NONE', #63113, #8767, #18236, .T. ) ;
#36965=ORIENTED_EDGE ( 'NONE', *, *, #44651, .F. ) ;
#36966=CARTESIAN_POINT ( 'NONE',  ( -10.90165637462999904, -7.508992741355384304, 11.21895841913464587 ) ) ;
#36967=AXIS2_PLACEMENT_3D ( 'NONE', #19136, #53747, #54066 ) ;
#36968=EDGE_LOOP ( 'NONE', ( #29505, #25259, #28530, #59742 ) ) ;
#36969=DIRECTION ( 'NONE',  ( -1.000000000000000000, 0.000000000000000000, 0.000000000000000000 ) ) ;
#36970=LINE ( 'NONE', #6740, #46267 ) ;
#36971=DIRECTION ( 'NONE',  ( -1.000000000000000000, -0.000000000000000000, -0.000000000000000000 ) ) ;
#36972=ORIENTED_EDGE ( 'NONE', *, *, #22692, .T. ) ;
#36976=CIRCLE ( 'NONE', #48691, 12.75000000000000178 ) ;
#36977=ADVANCED_FACE ( 'NONE', ( #37967 ), #32631, .T. ) ;
#36978=CARTESIAN_POINT ( 'NONE',  ( 3.780834652287974773, 8.352030633203074927, 8.616471685210687070 ) ) ;
#36979=CARTESIAN_POINT ( 'NONE',  ( -35.00000000000000000, 0.000000000000000000, 0.000000000000000000 ) ) ;
#36980=CARTESIAN_POINT ( 'NONE',  ( -35.00000000000000000, 11.68758509253248334, -1.171570255487489609 ) ) ;
#36982=CIRCLE ( 'NONE', #34882, 12.75000000000000178 ) ;
#36983=EDGE_CURVE ( 'NONE', #62930, #63438, #35202, .T. ) ;
#36984=DIRECTION ( 'NONE',  ( 1.000000000000000000, 0.000000000000000000, 0.000000000000000000 ) ) ;
#36987=AXIS2_PLACEMENT_3D ( 'NONE', #22848, #39093, #33470 ) ;
#36989=ORIENTED_EDGE ( 'NONE', *, *, #45656, .T. ) ;
#36993=DIRECTION ( 'NONE',  ( 1.000000000000000000, 0.000000000000000000, 0.000000000000000000 ) ) ;
#36998=ORIENTED_EDGE ( 'NONE', *, *, #61568, .T. ) ;
#37000=ORIENTED_EDGE ( 'NONE', *, *, #47801, .F. ) ;
#37001=ORIENTED_EDGE ( 'NONE', *, *, #25131, .T. ) ;
#37002=CARTESIAN_POINT ( 'NONE',  ( 24.82652845881425208, -8.390869743685021476, -8.578654028722157321 ) ) ;
#37003=AXIS2_PLACEMENT_3D ( 'NONE', #38280, #3068, #28979 ) ;
#37004=ORIENTED_EDGE ( 'NONE', *, *, #13358, .F. ) ;
#37005=EDGE_CURVE ( 'NONE', #38749, #34574, #44744, .T. ) ;
#37006=CARTESIAN_POINT ( 'NONE',  ( -26.39842685320601134, -10.43619857301325560, 5.924288189175664243 ) ) ;
#37008=CARTESIAN_POINT ( 'NONE',  ( -35.00000000000000000, -7.215058775251326217, 9.821084925794544063 ) ) ;
#37010=ORIENTED_EDGE ( 'NONE', *, *, #25184, .T. ) ;
#37011=CARTESIAN_POINT ( 'NONE',  ( -4.979813338170842485, -1.249770091004172690, -11.93591655830499931 ) ) ;
#37012=VECTOR ( 'NONE', #63292, 1000.000000000000000 ) ;
#37015=CARTESIAN_POINT ( 'NONE',  ( 36.00000000000000711, -12.63095688309027764, 1.738225594540123708 ) ) ;
#37017=CYLINDRICAL_SURFACE ( 'NONE', #52207, 5.000000000000000888 ) ;
#37018=VERTEX_POINT ( 'NONE', #35522 ) ;
#37019=DIRECTION ( 'NONE',  ( -1.000000000000000000, 0.000000000000000000, 0.000000000000000000 ) ) ;
#37021=CARTESIAN_POINT ( 'NONE',  ( -16.98800322446194855, 2.922502605998049674, 13.17987020110344787 ) ) ;
#37022=CARTESIAN_POINT ( 'NONE',  ( -35.00000000000000000, 10.28547182238008162, 5.672855678558722303 ) ) ;
#37023=AXIS2_PLACEMENT_3D ( 'NONE', #41992, #12063, #21397 ) ;
#37027=DIRECTION ( 'NONE',  ( -1.000000000000000000, -0.000000000000000000, 0.000000000000000000 ) ) ;
#37030=AXIS2_PLACEMENT_3D ( 'NONE', #51975, #6419, #1443 ) ;
#37038=DIRECTION ( 'NONE',  ( 1.000000000000000000, -0.000000000000000000, 0.000000000000000000 ) ) ;
#37040=DIRECTION ( 'NONE',  ( 1.000000000000000000, 0.000000000000000000, 0.000000000000000000 ) ) ;
#37043=EDGE_CURVE ( 'NONE', #60814, #60039, #12905, .T. ) ;
#37044=FACE_OUTER_BOUND ( 'NONE', #49395, .T. ) ;
#37045=FACE_OUTER_BOUND ( 'NONE', #42497, .T. ) ;
#37048=LINE ( 'NONE', #23676, #44642 ) ;
#37050=AXIS2_PLACEMENT_3D ( 'NONE', #56200, #40586, #10639 ) ;
#37051=EDGE_CURVE ( 'NONE', #48033, #23557, #5620, .T. ) ;
#37052=DIRECTION ( 'NONE',  ( 1.000000000000000000, 0.000000000000000000, 0.000000000000000000 ) ) ;
#37053=CIRCLE ( 'NONE', #12660, 5.000000000000000000 ) ;
#37054=DIRECTION ( 'NONE',  ( 1.000000000000000000, 0.000000000000000000, 0.000000000000000000 ) ) ;
#37055=ADVANCED_FACE ( 'NONE', ( #5274 ), #20227, .T. ) ;
#37056=CARTESIAN_POINT ( 'NONE',  ( 8.437200413559441614, 4.218240606060086328, -11.23760835609581399 ) ) ;
#37057=EDGE_CURVE ( 'NONE', #8907, #19699, #14155, .T. ) ;
#37061=FACE_OUTER_BOUND ( 'NONE', #60962, .T. ) ;
#37064=CIRCLE ( 'NONE', #8420, 12.18650000000000055 ) ;
#37066=CARTESIAN_POINT ( 'NONE',  ( -25.68925157440544638, 10.12461928084059259, 6.442855087883957665 ) ) ;
#37067=DIRECTION ( 'NONE',  ( 1.000000000000000000, 0.000000000000000000, 0.000000000000000000 ) ) ;
#37071=DIRECTION ( 'NONE',  ( -1.000000000000000000, 0.000000000000000000, 0.000000000000000000 ) ) ;
#37073=EDGE_CURVE ( 'NONE', #10498, #4335, #27324, .T. ) ;
#37078=DIRECTION ( 'NONE',  ( 0.000000000000000000, 0.01356324068817998940, -0.9999080150203990547 ) ) ;
#37080=LINE ( 'NONE', #3765, #30747 ) ;
#37081=ORIENTED_EDGE ( 'NONE', *, *, #18654, .T. ) ;
#37083=EDGE_CURVE ( 'NONE', #55976, #8578, #17216, .T. ) ;
#37084=FACE_BOUND ( 'NONE', #6575, .T. ) ;
#37085=ORIENTED_EDGE ( 'NONE', *, *, #37204, .T. ) ;
#37086=ADVANCED_FACE ( 'NONE', ( #57796 ), #11558, .T. ) ;
#37088=DIRECTION ( 'NONE',  ( 1.000000000000000000, 0.000000000000000000, -0.000000000000000000 ) ) ;
#37089=CYLINDRICAL_SURFACE ( 'NONE', #3557, 12.18650000000000055 ) ;
#37090=CARTESIAN_POINT ( 'NONE',  ( -3.644870031796809684, -12.49356576308750100, 5.128347001116654980 ) ) ;
#37091=CARTESIAN_POINT ( 'NONE',  ( -9.600257793028196929, 9.184030621591224630, -7.726472095688762920 ) ) ;
#37092=EDGE_CURVE ( 'NONE', #50423, #14292, #3341, .T. ) ;
#37093=DIRECTION ( 'NONE',  ( 0.000000000000000000, -0.1387779952735885280, 0.9903235168508540687 ) ) ;
#37094=CARTESIAN_POINT ( 'NONE',  ( -35.00000000000000000, -10.59380114696474884, 7.094637218249319588 ) ) ;
#37095=ORIENTED_EDGE ( 'NONE', *, *, #3316, .T. ) ;
#37100=DIRECTION ( 'NONE',  ( -1.000000000000000000, 0.000000000000000000, -0.000000000000000000 ) ) ;
#37102=CIRCLE ( 'NONE', #59418, 12.18650000000000055 ) ;
#37103=CARTESIAN_POINT ( 'NONE',  ( 35.00000000000000000, 4.705694406421931860E-17, -3.469127814946512892E-15 ) ) ;
#37104=ORIENTED_EDGE ( 'NONE', *, *, #42650, .T. ) ;
#37106=AXIS2_PLACEMENT_3D ( 'NONE', #59316, #48693, #4112 ) ;
#37108=ORIENTED_EDGE ( 'NONE', *, *, #24767, .T. ) ;
#37109=VERTEX_POINT ( 'NONE', #1612 ) ;
#37112=DIRECTION ( 'NONE',  ( -1.000000000000000000, 0.000000000000000000, 0.000000000000000000 ) ) ;
#37113=DIRECTION ( 'NONE',  ( 0.000000000000000000, -0.01356324068817998940, 0.9999080150203990547 ) ) ;
#37114=CARTESIAN_POINT ( 'NONE',  ( 9.273470328753727898, 2.853023627877379731, 13.19712399426135008 ) ) ;
#37117=EDGE_CURVE ( 'NONE', #7095, #61909, #32804, .T. ) ;
#37119=CARTESIAN_POINT ( 'NONE',  ( 26.17129964821461385, -11.44745868472663197, 3.602463285258928671 ) ) ;
#37120=DIRECTION ( 'NONE',  ( 0.000000000000000000, 0.01356324068817998940, -0.9999080150203990547 ) ) ;
#37122=VERTEX_POINT ( 'NONE', #2254 ) ;
#37123=DIRECTION ( 'NONE',  ( 0.000000000000000000, -0.2006870767258961963, 0.9796553971857727694 ) ) ;
#37124=VERTEX_POINT ( 'NONE', #61772 ) ;
#37125=CYLINDRICAL_SURFACE ( 'NONE', #50215, 5.000000000000000000 ) ;
#37127=CYLINDRICAL_SURFACE ( 'NONE', #64720, 4.999999999999999112 ) ;
#37128=DIRECTION ( 'NONE',  ( 0.000000000000000000, 0.01356324068817991828, -0.9999080150203990547 ) ) ;
#37131=AXIS2_PLACEMENT_3D ( 'NONE', #29270, #14599, #49567 ) ;
#37133=ORIENTED_EDGE ( 'NONE', *, *, #1815, .T. ) ;
#37135=EDGE_CURVE ( 'NONE', #4279, #26831, #44739, .T. ) ;
#37140=DIRECTION ( 'NONE',  ( 1.000000000000000000, 0.000000000000000000, 0.000000000000000000 ) ) ;
#37143=ORIENTED_EDGE ( 'NONE', *, *, #18526, .T. ) ;
#37145=CARTESIAN_POINT ( 'NONE',  ( -35.00000000000000000, 7.146664589318047156, -9.321877890560362090 ) ) ;
#37146=DIRECTION ( 'NONE',  ( 0.000000000000000000, -0.01356324068817998940, 0.9999080150203990547 ) ) ;
#37150=CARTESIAN_POINT ( 'NONE',  ( 9.612870878434209843, -11.96650298090370690, -0.9106810471525499384 ) ) ;
#37151=VERTEX_POINT ( 'NONE', #46812 ) ;
#37154=CARTESIAN_POINT ( 'NONE',  ( -37.00000000000000711, 12.18359334611896472, 0.2661492558803780772 ) ) ;
#37155=CARTESIAN_POINT ( 'NONE',  ( 35.00000000000000000, 9.700295462048766026, 7.376655759824770620 ) ) ;
#37156=CARTESIAN_POINT ( 'NONE',  ( 35.00000000000000000, 4.705694406421931860E-17, -3.469127814946512892E-15 ) ) ;
#37157=DIRECTION ( 'NONE',  ( 1.000000000000000000, 0.000000000000000000, -0.000000000000000000 ) ) ;
#37158=CARTESIAN_POINT ( 'NONE',  ( 35.00000000000000000, -12.38385022362083632, -3.033604067594535714 ) ) ;
#37159=EDGE_CURVE ( 'NONE', #57376, #40209, #11793, .T. ) ;
#37160=AXIS2_PLACEMENT_3D ( 'NONE', #50768, #10508, #10850 ) ;
#37161=EDGE_LOOP ( 'NONE', ( #36876, #39054, #45879, #55072 ) ) ;
#37164=EDGE_CURVE ( 'NONE', #32109, #3960, #42796, .T. ) ;
#37165=ORIENTED_EDGE ( 'NONE', *, *, #535, .F. ) ;
#37168=DIRECTION ( 'NONE',  ( 0.000000000000000000, 0.01356324068817992175, -0.9999080150203990547 ) ) ;
#37171=DIRECTION ( 'NONE',  ( -1.000000000000000000, 0.000000000000000000, 0.000000000000000000 ) ) ;
#37172=EDGE_CURVE ( 'NONE', #26332, #56593, #21557, .T. ) ;
#37174=CARTESIAN_POINT ( 'NONE',  ( -37.00000000000000711, 12.26766708251996363, -3.473736367725128726 ) ) ;
#37175=VERTEX_POINT ( 'NONE', #27186 ) ;
#37176=DIRECTION ( 'NONE',  ( -1.000000000000000000, 0.000000000000000000, 0.000000000000000000 ) ) ;
#37177=AXIS2_PLACEMENT_3D ( 'NONE', #20359, #20035, #10060 ) ;
#37178=ORIENTED_EDGE ( 'NONE', *, *, #17329, .F. ) ;
#37180=FACE_OUTER_BOUND ( 'NONE', #17174, .T. ) ;
#37182=ORIENTED_EDGE ( 'NONE', *, *, #38334, .F. ) ;
#37183=DIRECTION ( 'NONE',  ( 1.000000000000000000, -0.000000000000000000, 0.000000000000000000 ) ) ;
#37186=VERTEX_POINT ( 'NONE', #47480 ) ;
#37187=VERTEX_POINT ( 'NONE', #1919 ) ;
#37188=CYLINDRICAL_SURFACE ( 'NONE', #6680, 5.000000000000000888 ) ;
#37189=ORIENTED_EDGE ( 'NONE', *, *, #58030, .T. ) ;
#37191=ORIENTED_EDGE ( 'NONE', *, *, #358, .F. ) ;
#37193=ORIENTED_EDGE ( 'NONE', *, *, #35711, .F. ) ;
#37195=CARTESIAN_POINT ( 'NONE',  ( 145.1370849898475797, 3.309064568108273190E-14, 0.000000000000000000 ) ) ;
#37198=CIRCLE ( 'NONE', #6413, 5.000000000000000000 ) ;
#37199=CARTESIAN_POINT ( 'NONE',  ( 9.650000913499871658, 11.97776111335499749, -0.7481793053950375194 ) ) ;
#37200=DIRECTION ( 'NONE',  ( -0.6151304903148129277, 0.000000000000000000, -0.7884253166185480888 ) ) ;
#37202=EDGE_LOOP ( 'NONE', ( #40510, #22298, #30566, #63411 ) ) ;
#37203=CARTESIAN_POINT ( 'NONE',  ( 36.00000000000000711, -3.640372113593464576, 12.21925492305365424 ) ) ;
#37204=EDGE_CURVE ( 'NONE', #16407, #1249, #43789, .T. ) ;
#37205=ORIENTED_EDGE ( 'NONE', *, *, #50831, .T. ) ;
#37206=DIRECTION ( 'NONE',  ( 0.000000000000000000, 0.01356324068817992175, -0.9999080150203990547 ) ) ;
#37208=CARTESIAN_POINT ( 'NONE',  ( 35.00000000000000000, -11.65554240571056077, 1.456211999474460672 ) ) ;
#37213=CIRCLE ( 'NONE', #11713, 12.18649999999999878 ) ;
#37215=CARTESIAN_POINT ( 'NONE',  ( 35.00000000000000000, 11.65554240571056788, -1.456211999474385843 ) ) ;
#37216=AXIS2_PLACEMENT_3D ( 'NONE', #52462, #61750, #56802 ) ;
#37224=FACE_OUTER_BOUND ( 'NONE', #31092, .T. ) ;
#37225=CARTESIAN_POINT ( 'NONE',  ( -7.181456785175555524, 25.00000000000000000, -10.45493698471458188 ) ) ;
#37227=DIRECTION ( 'NONE',  ( 0.000000000000000000, -0.01356324068817998940, 0.9999080150203990547 ) ) ;
#37228=CARTESIAN_POINT ( 'NONE',  ( 26.08439714455133185, 11.40113243194252846, 3.743551691817327942 ) ) ;
#37231=AXIS2_PLACEMENT_3D ( 'NONE', #13718, #4087, #3464 ) ;
#37232=DIRECTION ( 'NONE',  ( -1.000000000000000000, -0.000000000000000000, 0.000000000000000000 ) ) ;
#37236=VECTOR ( 'NONE', #28117, 1000.000000000000000 ) ;
#37240=CIRCLE ( 'NONE', #21355, 5.000000000000000888 ) ;
#37241=CIRCLE ( 'NONE', #12792, 5.000000000000000000 ) ;
#37242=VECTOR ( 'NONE', #20503, 1000.000000000000000 ) ;
#37243=ORIENTED_EDGE ( 'NONE', *, *, #60658, .F. ) ;
#37250=CYLINDRICAL_SURFACE ( 'NONE', #50951, 12.75000000000000178 ) ;
#37251=VERTEX_POINT ( 'NONE', #24155 ) ;
#37252=ORIENTED_EDGE ( 'NONE', *, *, #14707, .T. ) ;
#37254=B_SPLINE_CURVE_WITH_KNOTS ( 'NONE', 3,
 ( #34607, #19004, #24980, #19978, #29306, #9325, #49291, #40246, #54261, #24645, #29611, #43949, #24001, #59905, #24308, #44923, #60534, #44573, #14328, #65202, #39270, #59568, #14969, #28644, #35258, #3746 ),
 .UNSPECIFIED., .F., .F.,
 ( 4, 2, 2, 2, 2, 2, 2, 2, 2, 2, 2, 2, 4 ),
 ( 1.852685484479510593E-18, 0.001358278954194288126, 0.002037418431291433164, 0.002716557908388578853, 0.003395697385485724543, 0.004074836862582869798, 0.005433115816777158574, 0.006112255293874302962, 0.006791394770971447351, 0.007470534248068590871, 0.008149673725165736127, 0.009507952679360023168, 0.01086623163355430847 ),
 .UNSPECIFIED. ) ;
#37257=CIRCLE ( 'NONE', #8601, 5.000000000000000888 ) ;
#37258=CARTESIAN_POINT ( 'NONE',  ( 22.05618987420085020, 11.97361567146972483, -0.7978078888370661037 ) ) ;
#37260=LINE ( 'NONE', #43557, #48560 ) ;
#37261=CIRCLE ( 'NONE', #26689, 5.000000000000000000 ) ;
#37262=AXIS2_PLACEMENT_3D ( 'NONE', #11565, #46820, #2263 ) ;
#37263=CARTESIAN_POINT ( 'NONE',  ( -37.00000000000000711, 4.426194442447240363, 11.35427606708807957 ) ) ;
#37266=CARTESIAN_POINT ( 'NONE',  ( 37.00000000000000711, 0.8294751490779324055, -12.15823808070322798 ) ) ;
#37267=CYLINDRICAL_SURFACE ( 'NONE', #6351, 4.999999999999999112 ) ;
#37268=CARTESIAN_POINT ( 'NONE',  ( 22.88594695219327235, 3.421158645304719137, 11.50198563395281148 ) ) ;
#37269=ORIENTED_EDGE ( 'NONE', *, *, #25355, .T. ) ;
#37270=CIRCLE ( 'NONE', #21374, 12.18650000000000055 ) ;
#37272=VERTEX_POINT ( 'NONE', #64699 ) ;
#37274=AXIS2_PLACEMENT_3D ( 'NONE', #23568, #28539, #48844 ) ;
#37275=CARTESIAN_POINT ( 'NONE',  ( -19.18529308429517855, -4.483916446487654639, 12.73508973186750204 ) ) ;
#37277=CARTESIAN_POINT ( 'NONE',  ( -35.00000000000000000, 0.000000000000000000, 0.000000000000000000 ) ) ;
#37279=DIRECTION ( 'NONE',  ( 1.000000000000000000, -0.000000000000000000, 0.000000000000000000 ) ) ;
#37281=DIRECTION ( 'NONE',  ( 1.000000000000000000, -0.000000000000000000, 0.000000000000000000 ) ) ;
#37284=AXIS2_PLACEMENT_3D ( 'NONE', #36561, #46531, #40897 ) ;
#37288=DIRECTION ( 'NONE',  ( 0.000000000000000000, -0.01356324068817998940, 0.9999080150203990547 ) ) ;
#37290=AXIS2_PLACEMENT_3D ( 'NONE', #51007, #35017, #55329 ) ;
#37291=EDGE_LOOP ( 'NONE', ( #56545, #43884, #63490, #5653 ) ) ;
#37292=DIRECTION ( 'NONE',  ( -1.000000000000000000, 0.000000000000000000, 0.000000000000000000 ) ) ;
#37294=DIRECTION ( 'NONE',  ( -1.000000000000000000, 0.000000000000000000, 0.000000000000000000 ) ) ;
#37295=ORIENTED_EDGE ( 'NONE', *, *, #58672, .F. ) ;
#37296=AXIS2_PLACEMENT_3D ( 'NONE', #6749, #46983, #61938 ) ;
#37297=ADVANCED_FACE ( 'NONE', ( #56042 ), #35746, .T. ) ;
#37299=ORIENTED_EDGE ( 'NONE', *, *, #24835, .F. ) ;
#37304=CARTESIAN_POINT ( 'NONE',  ( -3.014567788889948474, -9.061531127596236246, 10.01322194078947447 ) ) ;
#37305=DIRECTION ( 'NONE',  ( 0.000000000000000000, -0.01356324068817992175, 0.9999080150203990547 ) ) ;
#37306=DIRECTION ( 'NONE',  ( 0.000000000000000000, -0.7617968321374810614, -0.6478160128812026075 ) ) ;
#37309=DIRECTION ( 'NONE',  ( 0.000000000000000000, -0.8369827122275286246, -0.5472293298355360713 ) ) ;
#37312=CARTESIAN_POINT ( 'NONE',  ( 27.65241022803075666, 12.51656249166301116, 5.069893477639606516 ) ) ;
#37315=CARTESIAN_POINT ( 'NONE',  ( -18.04458733766117362, 11.34280559204706584, 3.916728392552376370 ) ) ;
#37316=DIRECTION ( 'NONE',  ( -1.000000000000000000, 0.000000000000000000, 0.000000000000000000 ) ) ;
#37317=CARTESIAN_POINT ( 'NONE',  ( -9.044048956294579611, -11.38398270688160530, -3.796001806769629727 ) ) ;
#37318=DIRECTION ( 'NONE',  ( -0.000000000000000000, -1.000000000000000000, -0.000000000000000000 ) ) ;
#37321=ADVANCED_FACE ( 'NONE', ( #55398 ), #9836, .T. ) ;
#37323=DIRECTION ( 'NONE',  ( 0.000000000000000000, 0.3554799084908900619, 0.9346839223284566511 ) ) ;
#37324=CARTESIAN_POINT ( 'NONE',  ( 4.638437190804134858, -10.09537402753981361, 8.963882972395243343 ) ) ;
#37325=CIRCLE ( 'NONE', #44728, 12.75000000000000178 ) ;
#37327=CARTESIAN_POINT ( 'NONE',  ( -37.00000000000000711, -11.01837265713077763, 6.415447294506668285 ) ) ;
#37329=ORIENTED_EDGE ( 'NONE', *, *, #83, .T. ) ;
#37331=CARTESIAN_POINT ( 'NONE',  ( -35.00000000000000000, 1.791059740004591561, -12.05416472667163674 ) ) ;
#37332=ORIENTED_EDGE ( 'NONE', *, *, #50277, .T. ) ;
#37333=LINE ( 'NONE', #62935, #917 ) ;
#37335=ORIENTED_EDGE ( 'NONE', *, *, #25679, .F. ) ;
#37336=EDGE_CURVE ( 'NONE', #37187, #14288, #62782, .T. ) ;
#37338=CARTESIAN_POINT ( 'NONE',  ( 37.00000000000000711, -5.865551165830999558, 11.32068061209301213 ) ) ;
#37339=CIRCLE ( 'NONE', #45850, 4.999999999999999112 ) ;
#37341=DIRECTION ( 'NONE',  ( -1.000000000000000000, 0.000000000000000000, -0.000000000000000000 ) ) ;
#37343=CARTESIAN_POINT ( 'NONE',  ( 35.00000000000000000, -11.53507381115584529, -2.216820770815045805 ) ) ;
#37344=CARTESIAN_POINT ( 'NONE',  ( 35.00000000000000000, 4.705694406421931860E-17, -3.469127814946512892E-15 ) ) ;
#37345=ORIENTED_EDGE ( 'NONE', *, *, #17584, .T. ) ;
#37348=DIRECTION ( 'NONE',  ( -1.000000000000000000, -0.000000000000000000, 0.000000000000000000 ) ) ;
#37349=ORIENTED_EDGE ( 'NONE', *, *, #47798, .F. ) ;
#37354=CARTESIAN_POINT ( 'NONE',  ( 24.17635063625124658, -8.757419633580374452, -8.209409434500527070 ) ) ;
#37355=AXIS2_PLACEMENT_3D ( 'NONE', #45499, #54190, #34545 ) ;
#37356=DIRECTION ( 'NONE',  ( -1.000000000000000000, 0.000000000000000000, 0.000000000000000000 ) ) ;
#37358=AXIS2_PLACEMENT_3D ( 'NONE', #58880, #13294, #52874 ) ;
#37359=ORIENTED_EDGE ( 'NONE', *, *, #35983, .F. ) ;
#37361=DIRECTION ( 'NONE',  ( 0.000000000000000000, -0.6269146997507875074, -0.7790879021242596014 ) ) ;
#37362=CARTESIAN_POINT ( 'NONE',  ( 12.87841448470966377, 11.26304985228344258, -7.445374560091265081 ) ) ;
#37363=VECTOR ( 'NONE', #10400, 1000.000000000000000 ) ;
#37364=ORIENTED_EDGE ( 'NONE', *, *, #28357, .T. ) ;
#37366=ORIENTED_EDGE ( 'NONE', *, *, #48857, .F. ) ;
#37367=LINE ( 'NONE', #17432, #14657 ) ;
#37368=ORIENTED_EDGE ( 'NONE', *, *, #63187, .T. ) ;
#37370=ORIENTED_EDGE ( 'NONE', *, *, #43519, .F. ) ;
#37371=CIRCLE ( 'NONE', #54347, 12.75000000000000178 ) ;
#37372=DIRECTION ( 'NONE',  ( -1.000000000000000000, 0.000000000000000000, 0.000000000000000000 ) ) ;
#37374=CARTESIAN_POINT ( 'NONE',  ( -35.00000000000000000, -0.01609748574453131326, 11.74614673114904129 ) ) ;
#37375=CARTESIAN_POINT ( 'NONE',  ( 37.00000000000000711, 4.705694406421931860E-17, -3.469127814946512892E-15 ) ) ;
#37378=CARTESIAN_POINT ( 'NONE',  ( 35.00000000000000000, -10.91536515067650903, -4.339012074899918581 ) ) ;
#37379=ORIENTED_EDGE ( 'NONE', *, *, #42312, .F. ) ;
#37380=DIRECTION ( 'NONE',  ( 1.000000000000000000, 0.000000000000000000, 0.000000000000000000 ) ) ;
#37381=FACE_OUTER_BOUND ( 'NONE', #7242, .T. ) ;
#37382=ADVANCED_FACE ( 'NONE', ( #22108 ), #7143, .T. ) ;
#37383=AXIS2_PLACEMENT_3D ( 'NONE', #50118, #4574, #566 ) ;
#37384=VECTOR ( 'NONE', #15235, 1000.000000000000000 ) ;
#37385=AXIS2_PLACEMENT_3D ( 'NONE', #37626, #32939, #57923 ) ;
#37387=DIRECTION ( 'NONE',  ( 0.000000000000000000, -0.5987040770935737610, 0.8009703041134120793 ) ) ;
#37389=CARTESIAN_POINT ( 'NONE',  ( -10.95212338237647920, -9.902220863987562183, -9.175839033069911110 ) ) ;
#37390=EDGE_CURVE ( 'NONE', #42435, #38749, #60660, .T. ) ;
#37395=CYLINDRICAL_SURFACE ( 'NONE', #14404, 12.18650000000000055 ) ;
#37398=CIRCLE ( 'NONE', #17245, 5.000000000000000888 ) ;
#37400=DIRECTION ( 'NONE',  ( -0.000000000000000000, -0.000000000000000000, -1.000000000000000000 ) ) ;
#37401=DIRECTION ( 'NONE',  ( 0.000000000000000000, 0.5472293298355215274, -0.8369827122275381726 ) ) ;
#37404=CARTESIAN_POINT ( 'NONE',  ( -35.00000000000000000, 12.18359334611896472, 0.2661492558803780772 ) ) ;
#37405=CARTESIAN_POINT ( 'NONE',  ( 35.00000000000000000, 11.68758509253246558, -1.171570255487653700 ) ) ;
#37407=AXIS2_PLACEMENT_3D ( 'NONE', #21247, #27226, #22232 ) ;
#37409=ORIENTED_EDGE ( 'NONE', *, *, #35275, .T. ) ;
#37411=DIRECTION ( 'NONE',  ( 1.000000000000000000, 0.000000000000000000, -0.000000000000000000 ) ) ;
#37413=VERTEX_POINT ( 'NONE', #27418 ) ;
#37415=ADVANCED_FACE ( 'NONE', ( #42703 ), #1188, .T. ) ;
#37416=DIRECTION ( 'NONE',  ( 0.000000000000000000, -0.01356324068817991828, 0.9999080150203990547 ) ) ;
#37417=ORIENTED_EDGE ( 'NONE', *, *, #12796, .T. ) ;
#37419=AXIS2_PLACEMENT_3D ( 'NONE', #4267, #24539, #44817 ) ;
#37422=DIRECTION ( 'NONE',  ( -0.000000000000000000, -0.000000000000000000, -1.000000000000000000 ) ) ;
#37427=CARTESIAN_POINT ( 'NONE',  ( 10.22080531381022972, 7.430815483004926669, 11.27448495604908452 ) ) ;
#37428=ORIENTED_EDGE ( 'NONE', *, *, #58787, .T. ) ;
#37431=VERTEX_POINT ( 'NONE', #41394 ) ;
#37432=VECTOR ( 'NONE', #23290, 1000.000000000000000 ) ;
#37436=CIRCLE ( 'NONE', #38539, 5.000000000000000888 ) ;
#37437=CARTESIAN_POINT ( 'NONE',  ( -3.857720864536276828, 10.47202569828348651, 5.863983351155762413 ) ) ;
#37440=CARTESIAN_POINT ( 'NONE',  ( -37.00000000000000711, -9.677500615117949678, 6.657191900728284928 ) ) ;
#37443=EDGE_CURVE ( 'NONE', #10928, #38977, #26776, .T. ) ;
#37445=VERTEX_POINT ( 'NONE', #21809 ) ;
#37446=B_SPLINE_CURVE_WITH_KNOTS ( 'NONE', 3,
 ( #45671, #20079, #61607, #50678, #35359, #61957, #36679, #15723, #60639, #5123, #46341, #25390, #127, #60981, #11403, #51986, #10414, #20408 ),
 .UNSPECIFIED., .F., .F.,
 ( 4, 2, 2, 2, 2, 2, 2, 2, 4 ),
 ( 2.453269466693398698E-18, 0.002548279257371096305, 0.003185349071713867563, 0.003822418886056638387, 0.005096558514742179601, 0.006370698143427721248, 0.007644837772113261161, 0.008918977400798800206, 0.01019311702948434012 ),
 .UNSPECIFIED. ) ;
#37447=ORIENTED_EDGE ( 'NONE', *, *, #61380, .T. ) ;
#37448=FACE_OUTER_BOUND ( 'NONE', #41001, .T. ) ;
#37449=EDGE_CURVE ( 'NONE', #46319, #11584, #3574, .T. ) ;
#37450=VERTEX_POINT ( 'NONE', #23099 ) ;
#37451=DIRECTION ( 'NONE',  ( 0.000000000000000000, 0.01356324068817998940, -0.9999080150203990547 ) ) ;
#37453=DIRECTION ( 'NONE',  ( 0.000000000000000000, 0.9246979985058736418, 0.3807014730195186769 ) ) ;
#37455=AXIS2_PLACEMENT_3D ( 'NONE', #61531, #11332, #27275 ) ;
#37459=DIRECTION ( 'NONE',  ( 1.000000000000000000, -0.000000000000000000, 0.000000000000000000 ) ) ;
#37460=ORIENTED_EDGE ( 'NONE', *, *, #53859, .T. ) ;
#37462=EDGE_CURVE ( 'NONE', #9134, #59369, #37736, .T. ) ;
#37463=VERTEX_POINT ( 'NONE', #38048 ) ;
#37465=DIRECTION ( 'NONE',  ( 1.000000000000000000, 0.000000000000000000, 0.000000000000000000 ) ) ;
#37469=ORIENTED_EDGE ( 'NONE', *, *, #15510, .T. ) ;
#37473=( BOUNDED_CURVE ( )  B_SPLINE_CURVE ( 3, ( #52976, #39309, #43646, #34330 ),
 .UNSPECIFIED., .F., .F. ) 
 B_SPLINE_CURVE_WITH_KNOTS ( ( 4, 4 ),
 ( 1.737343023833860078, 1.756906829757061361 ),
 .UNSPECIFIED. ) 
 CURVE ( )  GEOMETRIC_REPRESENTATION_ITEM ( )  RATIONAL_B_SPLINE_CURVE ( ( 1.000000000000000000, 0.9999681050458084641, 0.9999681050458084641, 1.000000000000000000 ) ) 
 REPRESENTATION_ITEM ( '' )  );
#37476=DIRECTION ( 'NONE',  ( -1.000000000000000000, 0.000000000000000000, 0.000000000000000000 ) ) ;
#37477=ADVANCED_FACE ( 'NONE', ( #53371 ), #48708, .T. ) ;
#37481=AXIS2_PLACEMENT_3D ( 'NONE', #34937, #64881, #39625 ) ;
#37485=CARTESIAN_POINT ( 'NONE',  ( 35.00000000000000000, -5.428340790341627198, 10.91072401419415883 ) ) ;
#37488=AXIS2_PLACEMENT_3D ( 'NONE', #57153, #37171, #47819 ) ;
#37490=DIRECTION ( 'NONE',  ( 0.000000000000000000, -0.01356324068817998940, 0.9999080150203990547 ) ) ;
#37491=ORIENTED_EDGE ( 'NONE', *, *, #63581, .T. ) ;
#37492=CIRCLE ( 'NONE', #34309, 5.000000000000000000 ) ;
#37494=VERTEX_POINT ( 'NONE', #54017 ) ;
#37495=CARTESIAN_POINT ( 'NONE',  ( -5.871534791385524699, -0.9854293836816523378, -13.46435699085508908 ) ) ;
#37498=CIRCLE ( 'NONE', #38601, 12.75000000000000178 ) ;
#37499=DIRECTION ( 'NONE',  ( 1.000000000000000000, -0.000000000000000000, 0.000000000000000000 ) ) ;
#37500=CARTESIAN_POINT ( 'NONE',  ( 37.00000000000000711, 12.15823808070323508, 0.8294751490777961811 ) ) ;
#37502=EDGE_CURVE ( 'NONE', #17695, #16904, #1291, .T. ) ;
#37503=EDGE_CURVE ( 'NONE', #23892, #54738, #57546, .T. ) ;
#37507=ORIENTED_EDGE ( 'NONE', *, *, #29695, .F. ) ;
#37509=CARTESIAN_POINT ( 'NONE',  ( 3.423954070241203240, 5.768012864559385555, -12.21298188730038881 ) ) ;
#37510=CARTESIAN_POINT ( 'NONE',  ( 35.00000000000000000, 6.950793414699941941, 10.68873102412834797 ) ) ;
#37511=DIRECTION ( 'NONE',  ( 0.000000000000000000, 0.9987865678893279586, -0.04924826701374244303 ) ) ;
#37516=VERTEX_POINT ( 'NONE', #8457 ) ;
#37518=ADVANCED_FACE ( 'NONE', ( #43042 ), #59330, .T. ) ;
#37519=CARTESIAN_POINT ( 'NONE',  ( -35.00000000000000000, 0.000000000000000000, 0.000000000000000000 ) ) ;
#37521=CARTESIAN_POINT ( 'NONE',  ( 23.30204873196431237, -11.22993834942661273, -7.499434092014816144 ) ) ;
#37522=DIRECTION ( 'NONE',  ( 1.000000000000000000, 0.000000000000000000, 0.000000000000000000 ) ) ;
#37524=ADVANCED_FACE ( 'NONE', ( #18777 ), #58703, .T. ) ;
#37526=ORIENTED_EDGE ( 'NONE', *, *, #4717, .F. ) ;
#37527=PLANE ( 'NONE',  #65135 ) ;
#37530=ORIENTED_EDGE ( 'NONE', *, *, #63274, .F. ) ;
#37532=CARTESIAN_POINT ( 'NONE',  ( 3.291290029914074378, 8.250315036047103590, 10.68561190601527855 ) ) ;
#37536=VECTOR ( 'NONE', #46254, 1000.000000000000000 ) ;
#37538=AXIS2_PLACEMENT_3D ( 'NONE', #8422, #28695, #23733 ) ;
#37540=ORIENTED_EDGE ( 'NONE', *, *, #16395, .T. ) ;
#37542=DIRECTION ( 'NONE',  ( -1.000000000000000000, -1.836970198721029688E-16, 0.000000000000000000 ) ) ;
#37543=AXIS2_PLACEMENT_3D ( 'NONE', #6507, #5877, #47079 ) ;
#37544=AXIS2_PLACEMENT_3D ( 'NONE', #29182, #23877, #28507 ) ;
#37545=CYLINDRICAL_SURFACE ( 'NONE', #29883, 3.309571291727934295 ) ;
#37546=DIRECTION ( 'NONE',  ( -1.000000000000000000, 0.000000000000000000, 0.000000000000000000 ) ) ;
#37547=DIRECTION ( 'NONE',  ( -1.000000000000000000, 0.000000000000000000, 0.000000000000000000 ) ) ;
#37548=DIRECTION ( 'NONE',  ( -1.000000000000000000, 0.000000000000000000, -0.000000000000000000 ) ) ;
#37549=ORIENTED_EDGE ( 'NONE', *, *, #21634, .T. ) ;
#37550=CARTESIAN_POINT ( 'NONE',  ( -36.00000000000000711, -9.733281772932221187, 8.235637554476612721 ) ) ;
#37551=EDGE_CURVE ( 'NONE', #48302, #12489, #25677, .T. ) ;
#37557=VECTOR ( 'NONE', #434, 1000.000000000000000 ) ;
#37558=CYLINDRICAL_SURFACE ( 'NONE', #40327, 5.000000000000000000 ) ;
#37561=EDGE_CURVE ( 'NONE', #22141, #55015, #38724, .T. ) ;
#37563=VERTEX_POINT ( 'NONE', #33721 ) ;
#37564=CARTESIAN_POINT ( 'NONE',  ( -14.37650451283982100, 8.347980080371831590, -8.621445213188774659 ) ) ;
#37565=ADVANCED_FACE ( 'NONE', ( #28736 ), #49052, .T. ) ;
#37566=AXIS2_PLACEMENT_3D ( 'NONE', #29987, #35625, #14034 ) ;
#37570=CIRCLE ( 'NONE', #63047, 5.000000000000000888 ) ;
#37571=CARTESIAN_POINT ( 'NONE',  ( 11.49573924273014391, -13.34169095181821341, -2.066154205673190969 ) ) ;
#37572=EDGE_CURVE ( 'NONE', #57134, #35533, #62837, .T. ) ;
#37575=ORIENTED_EDGE ( 'NONE', *, *, #27493, .F. ) ;
#37578=DIRECTION ( 'NONE',  ( 0.000000000000000000, 0.01356324068817998940, -0.9999080150203990547 ) ) ;
#37579=CARTESIAN_POINT ( 'NONE',  ( -2.952869152607111136, 7.581333670610111319, 11.17020052527586138 ) ) ;
#37580=CIRCLE ( 'NONE', #1467, 12.18650000000000055 ) ;
#37581=CARTESIAN_POINT ( 'NONE',  ( 37.00000000000000711, 6.547236723514018308, -9.752226076388918585 ) ) ;
#37582=ORIENTED_EDGE ( 'NONE', *, *, #4032, .T. ) ;
#37584=CIRCLE ( 'NONE', #53554, 5.000000000000001776 ) ;
#37585=AXIS2_PLACEMENT_3D ( 'NONE', #34169, #18247, #64740 ) ;
#37587=EDGE_CURVE ( 'NONE', #217, #52756, #3398, .T. ) ;
#37592=AXIS2_PLACEMENT_3D ( 'NONE', #46106, #54772, #40097 ) ;
#37593=CARTESIAN_POINT ( 'NONE',  ( 35.00000000000000000, 2.021542716731571154, 12.01765980939839196 ) ) ;
#37594=CARTESIAN_POINT ( 'NONE',  ( -37.00000000000000711, 4.309077947445652867, 10.92721691015457708 ) ) ;
#37596=ORIENTED_EDGE ( 'NONE', *, *, #5870, .F. ) ;
#37597=AXIS2_PLACEMENT_3D ( 'NONE', #4266, #4609, #44815 ) ;
#37598=EDGE_CURVE ( 'NONE', #49577, #61311, #49686, .T. ) ;
#37599=VERTEX_POINT ( 'NONE', #122 ) ;
#37600=ORIENTED_EDGE ( 'NONE', *, *, #57727, .F. ) ;
#37601=DIRECTION ( 'NONE',  ( -1.000000000000000000, 0.000000000000000000, 0.000000000000000000 ) ) ;
#37603=CARTESIAN_POINT ( 'NONE',  ( -27.16196273015727058, 13.32896842526023207, -2.143521441892688895 ) ) ;
#37605=FACE_OUTER_BOUND ( 'NONE', #10256, .T. ) ;
#37607=ORIENTED_EDGE ( 'NONE', *, *, #6400, .F. ) ;
#37609=VECTOR ( 'NONE', #42658, 1000.000000000000000 ) ;
#37610=CARTESIAN_POINT ( 'NONE',  ( 36.00000000000000711, 11.73555825188276280, -4.983891302653623789 ) ) ;
#37614=DIRECTION ( 'NONE',  ( 0.000000000000000000, 0.07632122047555796318, -0.9970832820307045097 ) ) ;
#37615=EDGE_CURVE ( 'NONE', #43482, #42026, #4131, .T. ) ;
#37617=DIRECTION ( 'NONE',  ( -1.000000000000000000, 0.000000000000000000, -0.000000000000000000 ) ) ;
#37619=EDGE_CURVE ( 'NONE', #34726, #44597, #35007, .T. ) ;
#37621=DIRECTION ( 'NONE',  ( 0.000000000000000000, -0.6269146997508042718, -0.7790879021242460567 ) ) ;
#37623=DIRECTION ( 'NONE',  ( 0.000000000000000000, -0.1118654143051685257, -0.9937233664769752339 ) ) ;
#37624=CARTESIAN_POINT ( 'NONE',  ( 24.97632970311352452, -10.66122974065905282, -8.283959357202887119 ) ) ;
#37625=CARTESIAN_POINT ( 'NONE',  ( 35.00000000000000000, -6.891188680298889757, -9.512294188640879611 ) ) ;
#37626=CARTESIAN_POINT ( 'NONE',  ( 37.00000000000000711, -0.7214809346829402781, -11.72397916322012179 ) ) ;
#37628=EDGE_LOOP ( 'NONE', ( #49974, #50961, #64991, #47958 ) ) ;
#37629=FACE_OUTER_BOUND ( 'NONE', #48915, .T. ) ;
#37630=ORIENTED_EDGE ( 'NONE', *, *, #64014, .T. ) ;
#37635=DIRECTION ( 'NONE',  ( 0.000000000000000000, 0.01356324068817998593, -0.9999080150203990547 ) ) ;
#37638=EDGE_CURVE ( 'NONE', #64575, #43456, #60976, .T. ) ;
#37639=VERTEX_POINT ( 'NONE', #45666 ) ;
#37641=DIRECTION ( 'NONE',  ( -1.000000000000000000, -0.000000000000000000, 0.000000000000000000 ) ) ;
#37642=EDGE_CURVE ( 'NONE', #4063, #50233, #24637, .T. ) ;
#37643=ORIENTED_EDGE ( 'NONE', *, *, #45621, .F. ) ;
#37644=CYLINDRICAL_SURFACE ( 'NONE', #30743, 5.000000000000000888 ) ;
#37645=DIRECTION ( 'NONE',  ( 0.000000000000000000, -0.01356324068817998940, 0.9999080150203990547 ) ) ;
#37647=DIRECTION ( 'NONE',  ( 1.000000000000000000, 0.000000000000000000, 0.000000000000000000 ) ) ;
#37648=CARTESIAN_POINT ( 'NONE',  ( -17.81810384895137389, -6.313241100106963266, 10.20918272949938554 ) ) ;
#37649=VERTEX_POINT ( 'NONE', #55318 ) ;
#37651=CIRCLE ( 'NONE', #11124, 5.000000000000000888 ) ;
#37652=EDGE_CURVE ( 'NONE', #19174, #54245, #44666, .T. ) ;
#37654=DIRECTION ( 'NONE',  ( 1.000000000000000000, 0.000000000000000000, -0.000000000000000000 ) ) ;
#37655=DIRECTION ( 'NONE',  ( 1.000000000000000000, -0.000000000000000000, -0.000000000000000000 ) ) ;
#37657=DIRECTION ( 'NONE',  ( 0.4622435816439406930, 0.000000000000000000, -0.8867529933577791290 ) ) ;
#37658=CARTESIAN_POINT ( 'NONE',  ( -35.00000000000000000, 0.000000000000000000, 0.000000000000000000 ) ) ;
#37660=AXIS2_PLACEMENT_3D ( 'NONE', #7444, #37721, #51488 ) ;
#37661=VERTEX_POINT ( 'NONE', #9110 ) ;
#37664=EDGE_CURVE ( 'NONE', #14001, #44564, #13992, .T. ) ;
#37668=LINE ( 'NONE', #57965, #30035 ) ;
#37669=ORIENTED_EDGE ( 'NONE', *, *, #56243, .F. ) ;
#37673=ORIENTED_EDGE ( 'NONE', *, *, #38061, .F. ) ;
#37674=AXIS2_PLACEMENT_3D ( 'NONE', #36862, #26892, #9358 ) ;
#37676=ORIENTED_EDGE ( 'NONE', *, *, #39070, .F. ) ;
#37677=VERTEX_POINT ( 'NONE', #10099 ) ;
#37679=ORIENTED_EDGE ( 'NONE', *, *, #63637, .F. ) ;
#37683=DIRECTION ( 'NONE',  ( 0.000000000000000000, 0.01356324068817991828, -0.9999080150203990547 ) ) ;
#37685=AXIS2_PLACEMENT_3D ( 'NONE', #17774, #46714, #1828 ) ;
#37686=DIRECTION ( 'NONE',  ( -1.000000000000000000, 0.000000000000000000, 0.000000000000000000 ) ) ;
#37689=CARTESIAN_POINT ( 'NONE',  ( 36.00000000000000711, -5.556331110570486231, -11.47561260193575272 ) ) ;
#37690=EDGE_LOOP ( 'NONE', ( #18819, #18285, #13298, #10526 ) ) ;
#37691=CARTESIAN_POINT ( 'NONE',  ( -35.00000000000000000, 11.38112321385055026, -2.905556151562505462 ) ) ;
#37693=ORIENTED_EDGE ( 'NONE', *, *, #64943, .T. ) ;
#37694=AXIS2_PLACEMENT_3D ( 'NONE', #49897, #54882, #19955 ) ;
#37697=CARTESIAN_POINT ( 'NONE',  ( -35.00000000000000000, 10.93004082984018410, 6.564808257521808521 ) ) ;
#37698=CARTESIAN_POINT ( 'NONE',  ( -37.00000000000000711, -12.74068829017553561, -0.4871980014162809458 ) ) ;
#37699=EDGE_CURVE ( 'NONE', #7316, #7009, #17182, .T. ) ;
#37700=AXIS2_PLACEMENT_3D ( 'NONE', #33356, #8745, #3782 ) ;
#37703=DIRECTION ( 'NONE',  ( -1.000000000000000000, -0.000000000000000000, 0.000000000000000000 ) ) ;
#37705=CARTESIAN_POINT ( 'NONE',  ( 12.37428322565249417, 10.69553198490500989, -8.245447885329925342 ) ) ;
#37708=LINE ( 'NONE', #1153, #23187 ) ;
#37709=ORIENTED_EDGE ( 'NONE', *, *, #24387, .F. ) ;
#37710=EDGE_LOOP ( 'NONE', ( #52827, #64193, #62450, #16215 ) ) ;
#37711=DIRECTION ( 'NONE',  ( 0.000000000000000000, 0.01356324068817991828, -0.9999080150203990547 ) ) ;
#37712=CARTESIAN_POINT ( 'NONE',  ( -17.95869421093891916, -11.89647782150295541, 1.606523818316730301 ) ) ;
#37713=DIRECTION ( 'NONE',  ( -1.000000000000000000, 0.000000000000000000, 0.000000000000000000 ) ) ;
#37714=DIRECTION ( 'NONE',  ( 0.000000000000000000, -0.01356324068817998940, 0.9999080150203990547 ) ) ;
#37715=CARTESIAN_POINT ( 'NONE',  ( -36.00000000000000711, -12.26766708251994409, 3.473736367725209551 ) ) ;
#37716=EDGE_CURVE ( 'NONE', #3284, #52011, #60306, .T. ) ;
#37717=CARTESIAN_POINT ( 'NONE',  ( -1.734723475976807094E-15, -3.469446951953614189E-15, 25.00000000000000000 ) ) ;
#37718=CIRCLE ( 'NONE', #13275, 5.000000000000001776 ) ;
#37719=CARTESIAN_POINT ( 'NONE',  ( 37.00000000000000711, 4.237620530777969741, 11.42599468261424356 ) ) ;
#37720=ORIENTED_EDGE ( 'NONE', *, *, #33995, .F. ) ;
#37721=DIRECTION ( 'NONE',  ( 1.000000000000000000, 0.000000000000000000, 0.000000000000000000 ) ) ;
#37722=DIRECTION ( 'NONE',  ( 1.000000000000000000, -0.000000000000000000, 0.000000000000000000 ) ) ;
#37724=ADVANCED_FACE ( 'NONE', ( #54688 ), #9415, .T. ) ;
#37726=CYLINDRICAL_SURFACE ( 'NONE', #56685, 12.74999999999999822 ) ;
#37727=DIRECTION ( 'NONE',  ( 0.000000000000000000, 0.01356324068817998940, -0.9999080150203989437 ) ) ;
#37728=CARTESIAN_POINT ( 'NONE',  ( 17.27839441901508621, -12.20388373500082224, 5.771933972472480967 ) ) ;
#37730=ORIENTED_EDGE ( 'NONE', *, *, #10269, .T. ) ;
#37731=DIRECTION ( 'NONE',  ( 0.000000000000000000, 0.01356324068817998940, -0.9999080150203990547 ) ) ;
#37734=CARTESIAN_POINT ( 'NONE',  ( -17.61481692485065054, -13.12896122980146529, 3.215558237703250111 ) ) ;
#37736=LINE ( 'NONE', #24084, #36250 ) ;
#37737=FACE_OUTER_BOUND ( 'NONE', #60904, .T. ) ;
#37738=ADVANCED_FACE ( 'NONE', ( #4805 ), #25072, .T. ) ;
#37739=ORIENTED_EDGE ( 'NONE', *, *, #20716, .F. ) ;
#37740=CARTESIAN_POINT ( 'NONE',  ( 18.23350676702760609, -7.210796396001341257, 9.602820039526596574 ) ) ;
#37742=CARTESIAN_POINT ( 'NONE',  ( -35.00000000000000000, -6.307491713049102167, 9.908974237959624176 ) ) ;
#37747=DIRECTION ( 'NONE',  ( 1.000000000000000000, 0.000000000000000000, 0.000000000000000000 ) ) ;
#37751=AXIS2_PLACEMENT_3D ( 'NONE', #44492, #14875, #64770 ) ;
#37759=DIRECTION ( 'NONE',  ( -1.000000000000000000, 0.000000000000000000, 0.000000000000000000 ) ) ;
#37762=EDGE_LOOP ( 'NONE', ( #5068, #38550, #28532, #21877 ) ) ;
#37766=LINE ( 'NONE', #1220, #34220 ) ;
#37767=ORIENTED_EDGE ( 'NONE', *, *, #5941, .F. ) ;
#37772=CARTESIAN_POINT ( 'NONE',  ( -4.045856953771468589, 9.480858417917106706, 7.359659509255599197 ) ) ;
#37774=DIRECTION ( 'NONE',  ( -1.000000000000000000, 0.000000000000000000, 0.000000000000000000 ) ) ;
#37775=ORIENTED_EDGE ( 'NONE', *, *, #31166, .F. ) ;
#37778=CARTESIAN_POINT ( 'NONE',  ( 3.924671233276515458, 7.659762911315605827, -11.15143203671860306 ) ) ;
#37783=VERTEX_POINT ( 'NONE', #41006 ) ;
#37787=AXIS2_PLACEMENT_3D ( 'NONE', #52681, #27073, #37361 ) ;
#37791=CARTESIAN_POINT ( 'NONE',  ( 35.00000000000000000, -10.14408668126217350, -5.921969905510321652 ) ) ;
#37792=ORIENTED_EDGE ( 'NONE', *, *, #12684, .T. ) ;
#37793=DIRECTION ( 'NONE',  ( -1.000000000000000000, 0.000000000000000000, -0.000000000000000000 ) ) ;
#37794=EDGE_LOOP ( 'NONE', ( #62611, #41210, #13711, #37861 ) ) ;
#37796=CARTESIAN_POINT ( 'NONE',  ( -8.504635283918430488, -10.07629646921066779, -8.990051544619507951 ) ) ;
#37797=EDGE_CURVE ( 'NONE', #29943, #28034, #34388, .T. ) ;
#37798=CARTESIAN_POINT ( 'NONE',  ( -35.00000000000000000, 1.030638227056741574, -12.14284015767849034 ) ) ;
#37800=ORIENTED_EDGE ( 'NONE', *, *, #11573, .F. ) ;
#37801=ADVANCED_FACE ( 'NONE', ( #41660 ), #31998, .T. ) ;
#37802=ORIENTED_EDGE ( 'NONE', *, *, #5435, .T. ) ;
#37806=CARTESIAN_POINT ( 'NONE',  ( 9.176090415275556467, 6.974186229596638142, 9.772926367110217782 ) ) ;
#37807=DIRECTION ( 'NONE',  ( 1.000000000000000000, 0.000000000000000000, 0.000000000000000000 ) ) ;
#37808=CARTESIAN_POINT ( 'NONE',  ( -37.00000000000000711, 10.59380114696480391, -7.094637218249240540 ) ) ;
#37809=ORIENTED_EDGE ( 'NONE', *, *, #29193, .F. ) ;
#37811=CARTESIAN_POINT ( 'NONE',  ( 18.03946127237285069, 10.01571122672373093, 9.058849096994427086 ) ) ;
#37813=DIRECTION ( 'NONE',  ( 1.000000000000000000, 0.000000000000000000, 0.000000000000000000 ) ) ;
#37814=EDGE_CURVE ( 'NONE', #61800, #59191, #46948, .T. ) ;
#37817=DIRECTION ( 'NONE',  ( -1.000000000000000000, 0.000000000000000000, -0.000000000000000000 ) ) ;
#37818=AXIS2_PLACEMENT_3D ( 'NONE', #43359, #28733, #39036 ) ;
#37819=EDGE_CURVE ( 'NONE', #44068, #40994, #37339, .T. ) ;
#37820=ORIENTED_EDGE ( 'NONE', *, *, #57741, .T. ) ;
#37821=EDGE_CURVE ( 'NONE', #37661, #33997, #11087, .T. ) ;
#37823=DIRECTION ( 'NONE',  ( 0.000000000000000000, 0.8515178078024849828, -0.5243256840888592674 ) ) ;
#37829=DIRECTION ( 'NONE',  ( 0.000000000000000000, -0.9551603052523510717, 0.2960891610144412156 ) ) ;
#37830=DIRECTION ( 'NONE',  ( 0.000000000000000000, -0.9937233664769749009, 0.1118654143051720229 ) ) ;
#37831=CARTESIAN_POINT ( 'NONE',  ( 37.00000000000000711, -2.544412758415763420, 11.91791701451268537 ) ) ;
#37832=ORIENTED_EDGE ( 'NONE', *, *, #32560, .F. ) ;
#37834=ORIENTED_EDGE ( 'NONE', *, *, #18112, .T. ) ;
#37836=VERTEX_POINT ( 'NONE', #47329 ) ;
#37837=DIRECTION ( 'NONE',  ( -0.000000000000000000, -0.000000000000000000, -1.000000000000000000 ) ) ;
#37839=FACE_OUTER_BOUND ( 'NONE', #1232, .T. ) ;
#37844=DIRECTION ( 'NONE',  ( 0.000000000000000000, 0.7196168960969817618, 0.6943713148249616163 ) ) ;
#37845=ORIENTED_EDGE ( 'NONE', *, *, #55196, .T. ) ;
#37846=ORIENTED_EDGE ( 'NONE', *, *, #6747, .F. ) ;
#37848=VERTEX_POINT ( 'NONE', #57636 ) ;
#37852=DIRECTION ( 'NONE',  ( -1.000000000000000000, 0.000000000000000000, 0.000000000000000000 ) ) ;
#37853=ORIENTED_EDGE ( 'NONE', *, *, #14457, .T. ) ;
#37855=LINE ( 'NONE', #21242, #46683 ) ;
#37858=ORIENTED_EDGE ( 'NONE', *, *, #37964, .T. ) ;
#37861=ORIENTED_EDGE ( 'NONE', *, *, #17689, .T. ) ;
#37862=DIRECTION ( 'NONE',  ( 0.000000000000000000, -0.7196168960969719919, -0.6943713148249717193 ) ) ;
#37864=AXIS2_PLACEMENT_3D ( 'NONE', #12616, #2697, #13603 ) ;
#37865=VERTEX_POINT ( 'NONE', #32978 ) ;
#37867=DIRECTION ( 'NONE',  ( 0.000000000000000000, -0.7617968321374811724, -0.6478160128812026075 ) ) ;
#37869=FACE_OUTER_BOUND ( 'NONE', #23456, .T. ) ;
#37870=CYLINDRICAL_SURFACE ( 'NONE', #12522, 5.000000000000000888 ) ;
#37872=DIRECTION ( 'NONE',  ( -1.000000000000000000, 0.000000000000000000, 0.000000000000000000 ) ) ;
#37877=CARTESIAN_POINT ( 'NONE',  ( -35.00000000000000000, 1.791059740004591561, -12.05416472667163674 ) ) ;
#37878=CARTESIAN_POINT ( 'NONE',  ( 47.00000000000000711, 4.705694406421931860E-17, -3.469127814946512892E-15 ) ) ;
#37879=DIRECTION ( 'NONE',  ( 1.000000000000000000, 0.000000000000000000, 0.000000000000000000 ) ) ;
#37882=DIRECTION ( 'NONE',  ( -0.000000000000000000, -1.000000000000000000, -0.000000000000000000 ) ) ;
#37883=EDGE_CURVE ( 'NONE', #14515, #22753, #38970, .T. ) ;
#37884=ORIENTED_EDGE ( 'NONE', *, *, #29284, .T. ) ;
#37886=EDGE_LOOP ( 'NONE', ( #65761, #41412, #65511, #15847 ) ) ;
#37889=CARTESIAN_POINT ( 'NONE',  ( 0.2851083653049530375, -0.4107471485392680810, -13.49374991542258151 ) ) ;
#37892=ORIENTED_EDGE ( 'NONE', *, *, #63979, .T. ) ;
#37894=DIRECTION ( 'NONE',  ( 1.000000000000000000, 0.000000000000000000, 0.000000000000000000 ) ) ;
#37895=CARTESIAN_POINT ( 'NONE',  ( -28.85619398320021745, 3.750539801530000439, 25.00000000000000000 ) ) ;
#37896=CARTESIAN_POINT ( 'NONE',  ( -4.049878455451396242, 11.39499819594600183, 7.250431408498958952 ) ) ;
#37897=EDGE_CURVE ( 'NONE', #52157, #27171, #55435, .T. ) ;
#37899=EDGE_CURVE ( 'NONE', #39860, #8191, #23696, .T. ) ;
#37901=EDGE_CURVE ( 'NONE', #3390, #38662, #16129, .T. ) ;
#37903=CIRCLE ( 'NONE', #28325, 4.999999999999999112 ) ;
#37904=AXIS2_PLACEMENT_3D ( 'NONE', #42912, #23292, #53887 ) ;
#37906=CARTESIAN_POINT ( 'NONE',  ( -9.615673917211060129, 12.77468887473842685, -4.382797285550743105 ) ) ;
#37907=ORIENTED_EDGE ( 'NONE', *, *, #31359, .T. ) ;
#37909=LINE ( 'NONE', #32902, #4582 ) ;
#37910=DIRECTION ( 'NONE',  ( 1.000000000000000000, 0.000000000000000000, -0.000000000000000000 ) ) ;
#37911=FACE_OUTER_BOUND ( 'NONE', #42008, .T. ) ;
#37914=ORIENTED_EDGE ( 'NONE', *, *, #59465, .T. ) ;
#37916=ORIENTED_EDGE ( 'NONE', *, *, #9327, .T. ) ;
#37917=ORIENTED_EDGE ( 'NONE', *, *, #49161, .T. ) ;
#37919=EDGE_CURVE ( 'NONE', #34795, #58896, #24863, .T. ) ;
#37924=CARTESIAN_POINT ( 'NONE',  ( -35.00000000000000000, -7.971186206369537786, 9.217970097227697224 ) ) ;
#37925=VERTEX_POINT ( 'NONE', #9040 ) ;
#37928=CARTESIAN_POINT ( 'NONE',  ( -35.00000000000000000, -10.43555801961479190, 5.391785509270926369 ) ) ;
#37929=ORIENTED_EDGE ( 'NONE', *, *, #21963, .F. ) ;
#37930=VERTEX_POINT ( 'NONE', #14016 ) ;
#37931=EDGE_CURVE ( 'NONE', #46064, #50432, #32063, .T. ) ;
#37933=ORIENTED_EDGE ( 'NONE', *, *, #4853, .F. ) ;
#37934=( NAMED_UNIT ( * ) PLANE_ANGLE_UNIT ( ) SI_UNIT ( $, .RADIAN. ) );
#37935=EDGE_LOOP ( 'NONE', ( #24042, #13387, #37329, #35627 ) ) ;
#37937=DIRECTION ( 'NONE',  ( 0.000000000000000000, 0.01356324068817998940, -0.9999080150203989437 ) ) ;
#37938=CARTESIAN_POINT ( 'NONE',  ( -37.00000000000000711, -4.339012074900030491, 10.91536515067646818 ) ) ;
#37940=CARTESIAN_POINT ( 'NONE',  ( -35.00000000000000000, -6.265926637539413591, -11.10408318471066380 ) ) ;
#37941=CARTESIAN_POINT ( 'NONE',  ( -37.00000000000000711, 12.16632754454237997, -0.7008968033237440443 ) ) ;
#37942=CARTESIAN_POINT ( 'NONE',  ( -27.01437459610461644, -8.723448335974111956, -8.240233560378637634 ) ) ;
#37945=VERTEX_POINT ( 'NONE', #64547 ) ;
#37946=DIRECTION ( 'NONE',  ( -1.000000000000000000, -0.000000000000000000, 0.000000000000000000 ) ) ;
#37947=FACE_OUTER_BOUND ( 'NONE', #46511, .T. ) ;
#37949=CARTESIAN_POINT ( 'NONE',  ( -14.37660149302730694, 8.348016424126690538, 8.621410803000902234 ) ) ;
#37953=VERTEX_POINT ( 'NONE', #59923 ) ;
#37954=EDGE_CURVE ( 'NONE', #22894, #30390, #41658, .T. ) ;
#37955=ORIENTED_EDGE ( 'NONE', *, *, #6392, .F. ) ;
#37956=AXIS2_PLACEMENT_3D ( 'NONE', #22387, #62957, #31396 ) ;
#37958=ORIENTED_EDGE ( 'NONE', *, *, #51801, .F. ) ;
#37959=DIRECTION ( 'NONE',  ( -1.000000000000000000, 0.000000000000000000, 0.000000000000000000 ) ) ;
#37961=CARTESIAN_POINT ( 'NONE',  ( -3.276654955009157710, -12.28508903930122997, 5.608921276358484143 ) ) ;
#37962=CYLINDRICAL_SURFACE ( 'NONE', #55483, 4.999999999999999112 ) ;
#37963=ORIENTED_EDGE ( 'NONE', *, *, #8018, .T. ) ;
#37964=EDGE_CURVE ( 'NONE', #10268, #3168, #50181, .T. ) ;
#37965=CARTESIAN_POINT ( 'NONE',  ( 35.00000000000000000, 11.26103545359850955, -3.340853584269734000 ) ) ;
#37966=DIRECTION ( 'NONE',  ( 0.000000000000000000, 0.01356324068817998940, -0.9999080150203990547 ) ) ;
#37967=FACE_OUTER_BOUND ( 'NONE', #49659, .T. ) ;
#37969=EDGE_CURVE ( 'NONE', #7715, #55405, #7408, .T. ) ;
#37970=CARTESIAN_POINT ( 'NONE',  ( -27.01437459610461644, 25.00000000000000000, -8.240233560378637634 ) ) ;
#37973=AXIS2_PLACEMENT_3D ( 'NONE', #39407, #8177, #28449 ) ;
#37974=ORIENTED_EDGE ( 'NONE', *, *, #9479, .T. ) ;
#37976=CIRCLE ( 'NONE', #19958, 5.000000000000001776 ) ;
#37977=EDGE_LOOP ( 'NONE', ( #50054, #9048, #56915, #20973 ) ) ;
#37978=CARTESIAN_POINT ( 'NONE',  ( -15.95899433880837748, 7.887743777454596206, -9.043566668317041035 ) ) ;
#37980=CARTESIAN_POINT ( 'NONE',  ( -35.00000000000000000, 0.000000000000000000, 0.000000000000000000 ) ) ;
#37981=EDGE_LOOP ( 'NONE', ( #59503, #38273, #46135, #42452 ) ) ;
#37985=ORIENTED_EDGE ( 'NONE', *, *, #1136, .F. ) ;
#37987=ORIENTED_EDGE ( 'NONE', *, *, #18793, .F. ) ;
#37989=EDGE_CURVE ( 'NONE', #44595, #1539, #50279, .T. ) ;
#37991=AXIS2_PLACEMENT_3D ( 'NONE', #9710, #4766, #54944 ) ;
#37993=EDGE_CURVE ( 'NONE', #25258, #63926, #13004, .T. ) ;
#37994=CARTESIAN_POINT ( 'NONE',  ( -25.86628395826706850, -5.139808748864358456, 10.84354029019568522 ) ) ;
#37997=ORIENTED_EDGE ( 'NONE', *, *, #26536, .T. ) ;
#37998=CYLINDRICAL_SURFACE ( 'NONE', #50072, 5.000000000000000888 ) ;
#38001=ORIENTED_EDGE ( 'NONE', *, *, #32366, .F. ) ;
#38002=EDGE_CURVE ( 'NONE', #55842, #35253, #57591, .T. ) ;
#38004=ORIENTED_EDGE ( 'NONE', *, *, #43330, .F. ) ;
#38005=CARTESIAN_POINT ( 'NONE',  ( -4.975205859172452172, -1.416020129149132778, 25.00000000000000000 ) ) ;
#38007=CARTESIAN_POINT ( 'NONE',  ( 35.00000000000000000, 4.705694406421931860E-17, -3.469127814946512892E-15 ) ) ;
#38008=DIRECTION ( 'NONE',  ( 1.000000000000000000, -0.000000000000000000, 0.000000000000000000 ) ) ;
#38009=CARTESIAN_POINT ( 'NONE',  ( -35.00000000000000000, -10.91536515067645041, -4.339012074900068683 ) ) ;
#38013=CARTESIAN_POINT ( 'NONE',  ( 13.00153132360262020, 13.08923778586748732, -3.311356634985274994 ) ) ;
#38016=DIRECTION ( 'NONE',  ( -0.000000000000000000, -0.000000000000000000, -1.000000000000000000 ) ) ;
#38017=ORIENTED_EDGE ( 'NONE', *, *, #28091, .F. ) ;
#38020=FACE_OUTER_BOUND ( 'NONE', #986, .T. ) ;
#38023=AXIS2_PLACEMENT_3D ( 'NONE', #51132, #39494, #39827 ) ;
#38024=DIRECTION ( 'NONE',  ( 0.000000000000000000, -0.6269146997507876184, -0.7790879021242596014 ) ) ;
#38027=EDGE_CURVE ( 'NONE', #21899, #58914, #26813, .T. ) ;
#38028=VERTEX_POINT ( 'NONE', #17619 ) ;
#38031=CARTESIAN_POINT ( 'NONE',  ( 35.00000000000000000, 9.752226076388984310, 6.547236723513913503 ) ) ;
#38032=ADVANCED_FACE ( 'NONE', ( #23245 ), #23585, .T. ) ;
#38033=VECTOR ( 'NONE', #42035, 1000.000000000000000 ) ;
#38035=DIRECTION ( 'NONE',  ( 1.000000000000000000, 0.000000000000000000, -0.000000000000000000 ) ) ;
#38036=( BOUNDED_CURVE ( )  B_SPLINE_CURVE ( 3, ( #23873, #38147, #27864, #23199 ),
 .UNSPECIFIED., .F., .F. ) 
 B_SPLINE_CURVE_WITH_KNOTS ( ( 4, 4 ),
 ( 5.214177674634521864, 5.220361350322005656 ),
 .UNSPECIFIED. ) 
 CURVE ( )  GEOMETRIC_REPRESENTATION_ITEM ( )  RATIONAL_B_SPLINE_CURVE ( ( 1.000000000000000000, 0.9999968135154544413, 0.9999968135154544413, 1.000000000000000000 ) ) 
 REPRESENTATION_ITEM ( '' )  );
#38039=EDGE_CURVE ( 'NONE', #24268, #34288, #8598, .T. ) ;
#38044=DIRECTION ( 'NONE',  ( -1.000000000000000000, 0.000000000000000000, 0.000000000000000000 ) ) ;
#38046=EDGE_CURVE ( 'NONE', #52497, #31515, #18469, .T. ) ;
#38047=CIRCLE ( 'NONE', #11525, 5.000000000000000000 ) ;
#38048=CARTESIAN_POINT ( 'NONE',  ( -35.00000000000000000, 6.018036132182325026, -11.24036214326513949 ) ) ;
#38049=ORIENTED_EDGE ( 'NONE', *, *, #37135, .T. ) ;
#38050=AXIS2_PLACEMENT_3D ( 'NONE', #16191, #5919, #26175 ) ;
#38051=DIRECTION ( 'NONE',  ( 0.000000000000000000, 0.01356324068817991828, -0.9999080150203990547 ) ) ;
#38055=ORIENTED_EDGE ( 'NONE', *, *, #37642, .T. ) ;
#38057=CARTESIAN_POINT ( 'NONE',  ( -19.02967556479663713, 11.99999999999999645, 1.585036030062028271E-15 ) ) ;
#38058=ORIENTED_EDGE ( 'NONE', *, *, #17751, .T. ) ;
#38060=DIRECTION ( 'NONE',  ( 0.000000000000000000, 0.01356324068818000848, -0.9999080150203990547 ) ) ;
#38061=EDGE_CURVE ( 'NONE', #12842, #52828, #16179, .T. ) ;
#38063=CARTESIAN_POINT ( 'NONE',  ( -35.00000000000000000, -6.946017217729864690, -10.01317267707894310 ) ) ;
#38065=EDGE_CURVE ( 'NONE', #42754, #39718, #27755, .T. ) ;
#38068=CIRCLE ( 'NONE', #44473, 12.18650000000000055 ) ;
#38070=AXIS2_PLACEMENT_3D ( 'NONE', #1138, #21417, #61983 ) ;
#38072=DIRECTION ( 'NONE',  ( -1.000000000000000000, -0.000000000000000000, 0.000000000000000000 ) ) ;
#38073=DIRECTION ( 'NONE',  ( 1.000000000000000000, 0.000000000000000000, 0.000000000000000000 ) ) ;
#38075=VERTEX_POINT ( 'NONE', #12939 ) ;
#38076=VECTOR ( 'NONE', #62235, 1000.000000000000000 ) ;
#38077=DIRECTION ( 'NONE',  ( -1.000000000000000000, 0.000000000000000000, 0.000000000000000000 ) ) ;
#38078=ORIENTED_EDGE ( 'NONE', *, *, #35288, .F. ) ;
#38079=LINE ( 'NONE', #43732, #53998 ) ;
#38080=ORIENTED_EDGE ( 'NONE', *, *, #51423, .F. ) ;
#38081=AXIS2_PLACEMENT_3D ( 'NONE', #23833, #49440, #24139 ) ;
#38083=CARTESIAN_POINT ( 'NONE',  ( -26.18480416658880117, 12.06940664534210939, 6.048772596418739766 ) ) ;
#38085=DIRECTION ( 'NONE',  ( -1.000000000000000000, -0.000000000000000000, 0.000000000000000000 ) ) ;
#38088=EDGE_LOOP ( 'NONE', ( #41332, #47272, #14768, #60126 ) ) ;
#38089=CARTESIAN_POINT ( 'NONE',  ( -24.91103398156301907, -10.02593217122324987, 6.596658411782785336 ) ) ;
#38090=CARTESIAN_POINT ( 'NONE',  ( -37.00000000000000711, 2.185196060783882288, 11.54110654723649709 ) ) ;
#38093=ORIENTED_EDGE ( 'NONE', *, *, #140, .T. ) ;
#38096=CARTESIAN_POINT ( 'NONE',  ( -35.00000000000000000, 5.865551165831237590, -11.32068061209289134 ) ) ;
#38100=LINE ( 'NONE', #58409, #26697 ) ;
#38102=VECTOR ( 'NONE', #25285, 1000.000000000000000 ) ;
#38105=ORIENTED_EDGE ( 'NONE', *, *, #4611, .F. ) ;
#38106=DIRECTION ( 'NONE',  ( 0.000000000000000000, 0.7617968321374899432, 0.6478160128811920604 ) ) ;
#38107=CIRCLE ( 'NONE', #50848, 12.18650000000000055 ) ;
#38108=ORIENTED_EDGE ( 'NONE', *, *, #4016, .T. ) ;
#38112=AXIS2_PLACEMENT_3D ( 'NONE', #20779, #46700, #5845 ) ;
#38113=ORIENTED_EDGE ( 'NONE', *, *, #22270, .T. ) ;
#38114=EDGE_CURVE ( 'NONE', #17397, #10044, #33556, .T. ) ;
#38116=VERTEX_POINT ( 'NONE', #8279 ) ;
#38117=CARTESIAN_POINT ( 'NONE',  ( 35.00000000000000000, 9.733281772932159015, -8.235637554476680222 ) ) ;
#38120=DIRECTION ( 'NONE',  ( 1.000000000000000000, 0.000000000000000000, 0.000000000000000000 ) ) ;
#38121=ADVANCED_FACE ( 'NONE', ( #28556 ), #48856, .T. ) ;
#38122=VERTEX_POINT ( 'NONE', #13576 ) ;
#38124=CARTESIAN_POINT ( 'NONE',  ( 36.00000000000000711, 2.527899948230813987, 12.49688848680881037 ) ) ;
#38125=CYLINDRICAL_SURFACE ( 'NONE', #1503, 6.342778212674966554 ) ;
#38127=FACE_OUTER_BOUND ( 'NONE', #24303, .T. ) ;
#38128=EDGE_CURVE ( 'NONE', #15694, #54998, #33865, .T. ) ;
#38131=ORIENTED_EDGE ( 'NONE', *, *, #24242, .F. ) ;
#38132=CARTESIAN_POINT ( 'NONE',  ( 35.00000000000000000, 12.15823808070323508, 0.8294751490777961811 ) ) ;
#38133=DIRECTION ( 'NONE',  ( 1.000000000000000000, 0.000000000000000000, 0.000000000000000000 ) ) ;
#38137=CARTESIAN_POINT ( 'NONE',  ( -17.16501208148281066, 3.058370451741322604, -13.14974288367183597 ) ) ;
#38139=DIRECTION ( 'NONE',  ( 0.000000000000000000, -0.8369827122275401710, -0.5472293298355185298 ) ) ;
#38146=ORIENTED_EDGE ( 'NONE', *, *, #39680, .T. ) ;
#38147=CARTESIAN_POINT ( 'NONE',  ( 17.11285760380283705, -10.50878607827770317, 5.793619504978386736 ) ) ;
#38148=DIRECTION ( 'NONE',  ( -1.000000000000000000, 0.000000000000000000, 0.000000000000000000 ) ) ;
#38149=DIRECTION ( 'NONE',  ( 1.000000000000000000, 0.000000000000000000, 0.000000000000000000 ) ) ;
#38150=CARTESIAN_POINT ( 'NONE',  ( -16.98800322446194855, 2.922502605998049674, 25.00000000000000000 ) ) ;
#38152=CARTESIAN_POINT ( 'NONE',  ( 35.00000000000000000, -11.81949347079744506, 2.968224442958526943 ) ) ;
#38154=ORIENTED_EDGE ( 'NONE', *, *, #24533, .F. ) ;
#38157=ORIENTED_EDGE ( 'NONE', *, *, #15959, .T. ) ;
#38158=CARTESIAN_POINT ( 'NONE',  ( 35.00000000000000000, 4.705694406421931860E-17, -3.469127814946512892E-15 ) ) ;
#38159=CIRCLE ( 'NONE', #48824, 5.000000000000000000 ) ;
#38160=EDGE_CURVE ( 'NONE', #34180, #31078, #60752, .T. ) ;
#38161=LINE ( 'NONE', #51845, #61933 ) ;
#38162=CARTESIAN_POINT ( 'NONE',  ( -35.00000000000000000, 0.000000000000000000, 0.000000000000000000 ) ) ;
#38163=CIRCLE ( 'NONE', #59394, 12.18649999999999878 ) ;
#38164=ORIENTED_EDGE ( 'NONE', *, *, #52964, .F. ) ;
#38165=DIRECTION ( 'NONE',  ( -1.000000000000000000, -0.000000000000000000, -0.000000000000000000 ) ) ;
#38167=DIRECTION ( 'NONE',  ( -1.000000000000000000, 0.000000000000000000, 0.000000000000000000 ) ) ;
#38168=EDGE_LOOP ( 'NONE', ( #43156, #48820, #42594, #57380 ) ) ;
#38171=ORIENTED_EDGE ( 'NONE', *, *, #28283, .T. ) ;
#38172=DIRECTION ( 'NONE',  ( -1.000000000000000000, -0.000000000000000000, 0.000000000000000000 ) ) ;
#38173=VERTEX_POINT ( 'NONE', #24217 ) ;
#38181=CARTESIAN_POINT ( 'NONE',  ( 35.00000000000000000, 0.3025107581131208367, -11.74226168163341555 ) ) ;
#38182=EDGE_CURVE ( 'NONE', #27902, #29107, #8734, .T. ) ;
#38183=ORIENTED_EDGE ( 'NONE', *, *, #48857, .T. ) ;
#38184=CARTESIAN_POINT ( 'NONE',  ( -37.00000000000000711, -12.70128625845193859, 1.113475361586445000 ) ) ;
#38185=ADVANCED_FACE ( 'NONE', ( #55130 ), #35502, .T. ) ;
#38187=EDGE_CURVE ( 'NONE', #33435, #3297, #54415, .T. ) ;
#38190=CARTESIAN_POINT ( 'NONE',  ( 28.69468230381643892, 10.59444862976622304, 5.650893053773811125 ) ) ;
#38191=DIRECTION ( 'NONE',  ( -1.000000000000000000, 0.000000000000000000, -0.000000000000000000 ) ) ;
#38192=CARTESIAN_POINT ( 'NONE',  ( 37.00000000000000711, -12.74921544981110877, 0.1414404973753431438 ) ) ;
#38193=CARTESIAN_POINT ( 'NONE',  ( 3.347841273039249721, -10.61118957148187825, -5.603807266321158664 ) ) ;
#38195=AXIS2_PLACEMENT_3D ( 'NONE', #8209, #34755, #18843 ) ;
#38197=ORIENTED_EDGE ( 'NONE', *, *, #61031, .T. ) ;
#38198=EDGE_CURVE ( 'NONE', #42734, #52495, #9240, .T. ) ;
#38201=ORIENTED_EDGE ( 'NONE', *, *, #32300, .T. ) ;
#38203=CARTESIAN_POINT ( 'NONE',  ( 35.00000000000000000, 11.99999999999999822, 1.469576158976822172E-15 ) ) ;
#38204=CARTESIAN_POINT ( 'NONE',  ( -36.00000000000000711, -0.3137578094508294280, -12.74613886779085625 ) ) ;
#38210=CARTESIAN_POINT ( 'NONE',  ( -36.00000000000000711, -8.366449238204298311, -9.621072037177086145 ) ) ;
#38211=CARTESIAN_POINT ( 'NONE',  ( -35.00000000000000000, 0.000000000000000000, 0.000000000000000000 ) ) ;
#38213=VECTOR ( 'NONE', #36528, 1000.000000000000000 ) ;
#38214=DIRECTION ( 'NONE',  ( 0.000000000000000000, 0.2618041379715635442, -0.9651210252299794456 ) ) ;
#38215=VERTEX_POINT ( 'NONE', #15540 ) ;
#38220=VERTEX_POINT ( 'NONE', #35807 ) ;
#38221=CARTESIAN_POINT ( 'NONE',  ( 10.47216603063722395, 7.645002999120487530, -9.252792978029043880 ) ) ;
#38222=EDGE_LOOP ( 'NONE', ( #710, #45534, #25387, #17814 ) ) ;
#38224=DIRECTION ( 'NONE',  ( 0.000000000000000000, 0.01356324068817998940, -0.9999080150203990547 ) ) ;
#38226=CARTESIAN_POINT ( 'NONE',  ( 35.00000000000000000, 10.92721691015455754, -4.309077947445693724 ) ) ;
#38229=ORIENTED_EDGE ( 'NONE', *, *, #38160, .F. ) ;
#38233=CIRCLE ( 'NONE', #60510, 12.18650000000000055 ) ;
#38235=AXIS2_PLACEMENT_3D ( 'NONE', #44918, #9652, #29947 ) ;
#38236=AXIS2_PLACEMENT_3D ( 'NONE', #23781, #48066, #2524 ) ;
#38238=DIRECTION ( 'NONE',  ( -0.000000000000000000, -1.000000000000000000, -0.000000000000000000 ) ) ;
#38240=EDGE_LOOP ( 'NONE', ( #27139, #61062, #17980, #4809 ) ) ;
#38241=DIRECTION ( 'NONE',  ( 0.000000000000000000, -0.01356324068817991481, 0.9999080150203990547 ) ) ;
#38244=CARTESIAN_POINT ( 'NONE',  ( 37.00000000000000711, 4.705694406421931860E-17, -3.469127814946512892E-15 ) ) ;
#38246=VERTEX_POINT ( 'NONE', #50493 ) ;
#38247=CARTESIAN_POINT ( 'NONE',  ( 0.09505933169495142665, -0.1369491540312669231, 11.99999999999999112 ) ) ;
#38248=EDGE_LOOP ( 'NONE', ( #9894, #35091, #51858, #18626 ) ) ;
#38249=CARTESIAN_POINT ( 'NONE',  ( 9.753977307252423401, 1.283513182606664360, -13.44047255910775185 ) ) ;
#38250=EDGE_LOOP ( 'NONE', ( #51551, #38414 ) ) ;
#38252=AXIS2_PLACEMENT_3D ( 'NONE', #51190, #61797, #25911 ) ;
#38254=CARTESIAN_POINT ( 'NONE',  ( -9.351388602708162523, 25.00000000000000000, -3.665735721005252135 ) ) ;
#38256=EDGE_CURVE ( 'NONE', #2532, #55405, #30506, .T. ) ;
#38257=CARTESIAN_POINT ( 'NONE',  ( 37.00000000000000711, 12.08216339958902630, 1.591260454995109930 ) ) ;
#38259=CARTESIAN_POINT ( 'NONE',  ( -27.74980211595206114, -10.95110850461715657, -4.915186702031700605 ) ) ;
#38260=ORIENTED_EDGE ( 'NONE', *, *, #60422, .T. ) ;
#38261=AXIS2_PLACEMENT_3D ( 'NONE', #50110, #24492, #54108 ) ;
#38263=VERTEX_POINT ( 'NONE', #4619 ) ;
#38264=CARTESIAN_POINT ( 'NONE',  ( 37.00000000000000711, -11.95840593935202811, -2.346765782874394635 ) ) ;
#38265=ADVANCED_FACE ( 'NONE', ( #60781 ), #24885, .F. ) ;
#38267=EDGE_CURVE ( 'NONE', #10044, #11257, #46991, .T. ) ;
#38268=ORIENTED_EDGE ( 'NONE', *, *, #33545, .F. ) ;
#38271=VECTOR ( 'NONE', #11044, 1000.000000000000000 ) ;
#38273=ORIENTED_EDGE ( 'NONE', *, *, #62470, .F. ) ;
#38274=ORIENTED_EDGE ( 'NONE', *, *, #6684, .F. ) ;
#38276=CARTESIAN_POINT ( 'NONE',  ( -28.85619398320021745, 3.750539801530000439, 25.00000000000000000 ) ) ;
#38277=AXIS2_PLACEMENT_3D ( 'NONE', #38999, #59622, #59293 ) ;
#38279=EDGE_CURVE ( 'NONE', #29827, #37187, #35291, .T. ) ;
#38280=CARTESIAN_POINT ( 'NONE',  ( -21.24030193723618609, 25.00000000000000000, -5.230344621181295395 ) ) ;
#38284=CARTESIAN_POINT ( 'NONE',  ( -18.16590544919054295, -5.562395585315481839, 10.63608869936934376 ) ) ;
#38285=ORIENTED_EDGE ( 'NONE', *, *, #558, .T. ) ;
#38286=CARTESIAN_POINT ( 'NONE',  ( 36.00000000000000711, -5.143145423404195782, 11.66664283989685202 ) ) ;
#38289=VECTOR ( 'NONE', #15948, 1000.000000000000000 ) ;
#38290=ADVANCED_FACE ( 'NONE', ( #3957 ), #40831, .T. ) ;
#38294=CARTESIAN_POINT ( 'NONE',  ( -36.00000000000000711, -11.01837265713077763, 6.415447294506668285 ) ) ;
#38299=AXIS2_PLACEMENT_3D ( 'NONE', #28094, #13433, #44341 ) ;
#38300=ORIENTED_EDGE ( 'NONE', *, *, #13658, .T. ) ;
#38301=CARTESIAN_POINT ( 'NONE',  ( 12.68972104065789530, -10.01785652089451695, -6.609210272055840996 ) ) ;
#38304=ORIENTED_EDGE ( 'NONE', *, *, #11209, .F. ) ;
#38305=CARTESIAN_POINT ( 'NONE',  ( -37.00000000000000711, -3.093009498344009955, 11.78745411414838884 ) ) ;
#38307=CARTESIAN_POINT ( 'NONE',  ( -29.92777678363736626, -3.750539801530011985, -11.39883551934752681 ) ) ;
#38308=ORIENTED_EDGE ( 'NONE', *, *, #17950, .F. ) ;
#38309=CIRCLE ( 'NONE', #25709, 5.000000000000001776 ) ;
#38310=DIRECTION ( 'NONE',  ( -1.000000000000000000, 0.000000000000000000, 0.000000000000000000 ) ) ;
#38311=ORIENTED_EDGE ( 'NONE', *, *, #9330, .T. ) ;
#38313=ORIENTED_EDGE ( 'NONE', *, *, #24013, .F. ) ;
#38314=ORIENTED_EDGE ( 'NONE', *, *, #9241, .F. ) ;
#38315=LINE ( 'NONE', #28036, #16398 ) ;
#38317=EDGE_CURVE ( 'NONE', #65390, #20627, #32081, .T. ) ;
#38319=EDGE_LOOP ( 'NONE', ( #58635, #27991 ) ) ;
#38320=DIRECTION ( 'NONE',  ( 0.000000000000000000, 0.7196168960969767658, 0.6943713148249667233 ) ) ;
#38321=CARTESIAN_POINT ( 'NONE',  ( 3.308621013519160492, 3.312703205413596308, 13.09392454462600952 ) ) ;
#38322=CYLINDRICAL_SURFACE ( 'NONE', #3656, 5.225920239717171789 ) ;
#38324=VERTEX_POINT ( 'NONE', #48063 ) ;
#38325=DIRECTION ( 'NONE',  ( 0.000000000000000000, -0.01356324068817991828, 0.9999080150203990547 ) ) ;
#38327=DIRECTION ( 'NONE',  ( 0.000000000000000000, -0.6478160128812002760, 0.7617968321374830598 ) ) ;
#38329=ORIENTED_EDGE ( 'NONE', *, *, #39361, .T. ) ;
#38331=AXIS2_PLACEMENT_3D ( 'NONE', #17473, #37747, #22796 ) ;
#38332=VERTEX_POINT ( 'NONE', #32411 ) ;
#38333=CARTESIAN_POINT ( 'NONE',  ( 37.00000000000000711, -11.07407352312215387, -3.916263239775311433 ) ) ;
#38334=EDGE_CURVE ( 'NONE', #42662, #60382, #42370, .T. ) ;
#38335=VERTEX_POINT ( 'NONE', #17133 ) ;
#38336=DIRECTION ( 'NONE',  ( -1.000000000000000000, 0.000000000000000000, 0.000000000000000000 ) ) ;
#38340=AXIS2_PLACEMENT_3D ( 'NONE', #10100, #35008, #41320 ) ;
#38341=CIRCLE ( 'NONE', #59625, 12.18649999999999878 ) ;
#38342=CYLINDRICAL_SURFACE ( 'NONE', #47381, 4.999999999999999112 ) ;
#38343=CIRCLE ( 'NONE', #1187, 12.18650000000000233 ) ;
#38345=CARTESIAN_POINT ( 'NONE',  ( -6.388056983029618330, -1.618957853436955308, -13.40265429600850311 ) ) ;
#38346=CARTESIAN_POINT ( 'NONE',  ( -35.00000000000000000, -9.493370459201647904, -6.917234959366931335 ) ) ;
#38347=VERTEX_POINT ( 'NONE', #17469 ) ;
#38349=CYLINDRICAL_SURFACE ( 'NONE', #50769, 12.18649999999999878 ) ;
#38350=ORIENTED_EDGE ( 'NONE', *, *, #9606, .T. ) ;
#38351=EDGE_CURVE ( 'NONE', #52499, #53854, #43762, .T. ) ;
#38352=ORIENTED_EDGE ( 'NONE', *, *, #5105, .F. ) ;
#38358=AXIS2_PLACEMENT_3D ( 'NONE', #34794, #19858, #55769 ) ;
#38360=CARTESIAN_POINT ( 'NONE',  ( -35.00000000000000000, 11.17622378668011685, -3.614449339633368119 ) ) ;
#38361=DIRECTION ( 'NONE',  ( 1.000000000000000000, -0.000000000000000000, 0.000000000000000000 ) ) ;
#38362=AXIS2_PLACEMENT_3D ( 'NONE', #45567, #39928, #692 ) ;
#38365=CYLINDRICAL_SURFACE ( 'NONE', #7387, 12.18649999999999878 ) ;
#38366=CIRCLE ( 'NONE', #60624, 12.74999999999999822 ) ;
#38368=DIRECTION ( 'NONE',  ( -0.000000000000000000, -1.000000000000000000, -0.000000000000000000 ) ) ;
#38370=AXIS2_PLACEMENT_3D ( 'NONE', #64123, #18603, #59151 ) ;
#38371=EDGE_CURVE ( 'NONE', #54954, #19174, #53359, .T. ) ;
#38374=EDGE_CURVE ( 'NONE', #20925, #22914, #61840, .T. ) ;
#38376=EDGE_CURVE ( 'NONE', #41890, #52499, #19098, .T. ) ;
#38377=LINE ( 'NONE', #8133, #11868 ) ;
#38378=CIRCLE ( 'NONE', #9705, 5.000000000000001776 ) ;
#38379=AXIS2_PLACEMENT_3D ( 'NONE', #12061, #36003, #31039 ) ;
#38380=VERTEX_POINT ( 'NONE', #18472 ) ;
#38382=LINE ( 'NONE', #23095, #65424 ) ;
#38384=CIRCLE ( 'NONE', #51128, 12.74999999999999822 ) ;
#38386=CARTESIAN_POINT ( 'NONE',  ( -24.90268129027903399, 7.525069038327800719, 9.354736030227490673 ) ) ;
#38387=DIRECTION ( 'NONE',  ( 0.000000000000000000, 0.01356324068817998940, -0.9999080150203989437 ) ) ;
#38389=CARTESIAN_POINT ( 'NONE',  ( -15.27729454824424948, 5.151216734910788908, 25.00000000000000000 ) ) ;
#38392=ORIENTED_EDGE ( 'NONE', *, *, #41941, .F. ) ;
#38393=CARTESIAN_POINT ( 'NONE',  ( -36.00000000000000711, 2.527899948230635907, 12.49688848680885300 ) ) ;
#38394=DIRECTION ( 'NONE',  ( -0.000000000000000000, -0.000000000000000000, -1.000000000000000000 ) ) ;
#38395=ORIENTED_EDGE ( 'NONE', *, *, #31577, .F. ) ;
#38396=ORIENTED_EDGE ( 'NONE', *, *, #43212, .F. ) ;
#38397=B_SPLINE_CURVE_WITH_KNOTS ( 'NONE', 3,
 ( #19255, #29864, #19589, #14558, #55142, #9569, #617, #10905 ),
 .UNSPECIFIED., .F., .F.,
 ( 4, 2, 2, 4 ),
 ( 0.01054950296625598721, 0.01134544828840661213, 0.01214139361055723877, 0.01373328425485848513 ),
 .UNSPECIFIED. ) ;
#38398=CARTESIAN_POINT ( 'NONE',  ( -35.00000000000000000, 0.000000000000000000, 0.000000000000000000 ) ) ;
#38399=VECTOR ( 'NONE', #2205, 1000.000000000000000 ) ;
#38400=AXIS2_PLACEMENT_3D ( 'NONE', #42137, #46182, #10919 ) ;
#38401=EDGE_CURVE ( 'NONE', #40447, #28337, #27915, .T. ) ;
#38403=AXIS2_PLACEMENT_3D ( 'NONE', #6584, #27178, #47790 ) ;
#38404=CARTESIAN_POINT ( 'NONE',  ( -35.00000000000000000, -0.9416912585473466990, -12.71517666308949046 ) ) ;
#38405=EDGE_CURVE ( 'NONE', #64117, #44435, #26859, .T. ) ;
#38406=CARTESIAN_POINT ( 'NONE',  ( -47.00000000000000711, 0.000000000000000000, 0.000000000000000000 ) ) ;
#38407=DIRECTION ( 'NONE',  ( 0.000000000000000000, 0.01356324068817992175, -0.9999080150203990547 ) ) ;
#38409=CARTESIAN_POINT ( 'NONE',  ( -37.00000000000000711, 11.50504120060943158, 4.018060380616439886 ) ) ;
#38410=DIRECTION ( 'NONE',  ( -1.000000000000000000, -0.000000000000000000, 0.000000000000000000 ) ) ;
#38411=DIRECTION ( 'NONE',  ( -1.000000000000000000, -0.000000000000000000, 0.000000000000000000 ) ) ;
#38412=ORIENTED_EDGE ( 'NONE', *, *, #41878, .T. ) ;
#38413=CYLINDRICAL_SURFACE ( 'NONE', #26748, 12.75000000000000178 ) ;
#38414=ORIENTED_EDGE ( 'NONE', *, *, #48633, .T. ) ;
#38415=CARTESIAN_POINT ( 'NONE',  ( -37.00000000000000711, 0.000000000000000000, 0.000000000000000000 ) ) ;
#38416=VECTOR ( 'NONE', #63617, 1000.000000000000000 ) ;
#38421=CARTESIAN_POINT ( 'NONE',  ( -25.68170654058536329, 11.85933282897061503, 6.451667499124866367 ) ) ;
#38423=CARTESIAN_POINT ( 'NONE',  ( -27.45775109278351067, 25.00000000000000000, -8.471355351200609007 ) ) ;
#38424=B_SPLINE_CURVE_WITH_KNOTS ( 'NONE', 3,
 ( #63352, #34074, #48093, #43736, #64017, #54392, #2549, #23130, #17816, #18504, #43395, #3535, #63670, #23809, #13157, #53731, #38756, #8825, #59056, #29114 ),
 .UNSPECIFIED., .F., .F.,
 ( 4, 2, 2, 2, 2, 2, 2, 2, 2, 4 ),
 ( 0.000000000000000000, 0.0008473511760410093376, 0.001694702352082018675, 0.002118377940102530825, 0.002542053528123043842, 0.003389404704164079418, 0.004236755880205114559, 0.005084107056246151002, 0.005931458232287185710, 0.006778809408328222152 ),
 .UNSPECIFIED. ) ;
#38425=DIRECTION ( 'NONE',  ( 0.000000000000000000, -0.9105187689795999351, 0.4134677391718417638 ) ) ;
#38428=ORIENTED_EDGE ( 'NONE', *, *, #11953, .T. ) ;
#38429=DIRECTION ( 'NONE',  ( -1.000000000000000000, -1.836970198721029688E-16, 0.000000000000000000 ) ) ;
#38433=DIRECTION ( 'NONE',  ( 1.000000000000000000, 0.000000000000000000, 0.000000000000000000 ) ) ;
#38434=EDGE_CURVE ( 'NONE', #16649, #54027, #15180, .T. ) ;
#38435=EDGE_LOOP ( 'NONE', ( #27849, #59382, #60424, #8287 ) ) ;
#38436=CARTESIAN_POINT ( 'NONE',  ( -18.25006854224444908, -9.443202773001939221, 25.00000000000000000 ) ) ;
#38440=VECTOR ( 'NONE', #31451, 1000.000000000000000 ) ;
#38441=DIRECTION ( 'NONE',  ( 0.000000000000000000, 0.8169148498130295311, -0.5767582926624942319 ) ) ;
#38442=DIRECTION ( 'NONE',  ( 1.000000000000000000, 0.000000000000000000, 0.000000000000000000 ) ) ;
#38443=VECTOR ( 'NONE', #50013, 1000.000000000000000 ) ;
#38444=DIRECTION ( 'NONE',  ( -1.000000000000000000, -0.000000000000000000, -0.000000000000000000 ) ) ;
#38445=ORIENTED_EDGE ( 'NONE', *, *, #20716, .T. ) ;
#38451=DIRECTION ( 'NONE',  ( 0.000000000000000000, -0.01356324068817991828, 0.9999080150203990547 ) ) ;
#38453=ADVANCED_FACE ( 'NONE', ( #44044 ), #54022, .T. ) ;
#38454=VERTEX_POINT ( 'NONE', #64315 ) ;
#38455=FACE_OUTER_BOUND ( 'NONE', #61911, .T. ) ;
#38460=AXIS2_PLACEMENT_3D ( 'NONE', #11671, #21327, #32593 ) ;
#38464=ORIENTED_EDGE ( 'NONE', *, *, #38746, .F. ) ;
#38468=LINE ( 'NONE', #55310, #45523 ) ;
#38470=AXIS2_PLACEMENT_3D ( 'NONE', #62720, #6893, #1250 ) ;
#38471=DIRECTION ( 'NONE',  ( 1.000000000000000000, 0.000000000000000000, -0.000000000000000000 ) ) ;
#38472=ORIENTED_EDGE ( 'NONE', *, *, #8248, .T. ) ;
#38476=VERTEX_POINT ( 'NONE', #6430 ) ;
#38478=DIRECTION ( 'NONE',  ( 0.000000000000000000, -0.01356324068817998940, 0.9999080150203990547 ) ) ;
#38479=CARTESIAN_POINT ( 'NONE',  ( 18.46655499260420541, -7.261936723394225801, 11.40458322575580752 ) ) ;
#38480=AXIS2_PLACEMENT_3D ( 'NONE', #56232, #10674, #26309 ) ;
#38481=DIRECTION ( 'NONE',  ( -1.000000000000000000, 0.000000000000000000, 0.000000000000000000 ) ) ;
#38483=AXIS2_PLACEMENT_3D ( 'NONE', #34702, #9430, #3842 ) ;
#38484=AXIS2_PLACEMENT_3D ( 'NONE', #39622, #29319, #44278 ) ;
#38486=PLANE ( 'NONE',  #19144 ) ;
#38489=EDGE_CURVE ( 'NONE', #54691, #4335, #30691, .T. ) ;
#38490=DIRECTION ( 'NONE',  ( 0.000000000000000000, -0.01356324068817998940, 0.9999080150203990547 ) ) ;
#38491=CARTESIAN_POINT ( 'NONE',  ( -35.00000000000000000, 11.72397916322013600, -0.7214809346827312231 ) ) ;
#38493=CARTESIAN_POINT ( 'NONE',  ( 35.00000000000000000, -2.772148766916200380, -11.86701198550355585 ) ) ;
#38496=FACE_OUTER_BOUND ( 'NONE', #53766, .T. ) ;
#38497=VERTEX_POINT ( 'NONE', #55979 ) ;
#38498=ORIENTED_EDGE ( 'NONE', *, *, #35820, .T. ) ;
#38499=ORIENTED_EDGE ( 'NONE', *, *, #16749, .F. ) ;
#38503=ORIENTED_EDGE ( 'NONE', *, *, #61127, .F. ) ;
#38504=CARTESIAN_POINT ( 'NONE',  ( 36.00000000000000711, 12.73293890771483916, 0.6593684648219062527 ) ) ;
#38507=LINE ( 'NONE', #52826, #12730 ) ;
#38508=ORIENTED_EDGE ( 'NONE', *, *, #14457, .F. ) ;
#38513=ORIENTED_EDGE ( 'NONE', *, *, #9583, .F. ) ;
#38515=ORIENTED_EDGE ( 'NONE', *, *, #63802, .T. ) ;
#38517=LINE ( 'NONE', #63767, #39457 ) ;
#38518=EDGE_CURVE ( 'NONE', #33298, #53158, #37446, .T. ) ;
#38519=DIRECTION ( 'NONE',  ( -1.000000000000000000, 0.000000000000000000, -0.000000000000000000 ) ) ;
#38521=DIRECTION ( 'NONE',  ( 0.000000000000000000, 0.01356324068817991828, -0.9999080150203990547 ) ) ;
#38525=AXIS2_PLACEMENT_3D ( 'NONE', #55994, #26725, #51018 ) ;
#38528=CYLINDRICAL_SURFACE ( 'NONE', #16391, 4.999999999999999112 ) ;
#38530=DIRECTION ( 'NONE',  ( -1.000000000000000000, 0.000000000000000000, 0.000000000000000000 ) ) ;
#38532=DIRECTION ( 'NONE',  ( 0.000000000000000000, -0.4134677391718386552, -0.9105187689796012673 ) ) ;
#38533=FACE_OUTER_BOUND ( 'NONE', #7111, .T. ) ;
#38535=DIRECTION ( 'NONE',  ( 0.000000000000000000, 0.01356324068817998940, -0.9999080150203990547 ) ) ;
#38537=CARTESIAN_POINT ( 'NONE',  ( -27.16343335735464137, -10.63351257863160626, -8.317934404008965998 ) ) ;
#38539=AXIS2_PLACEMENT_3D ( 'NONE', #62651, #15790, #539 ) ;
#38541=VERTEX_POINT ( 'NONE', #46018 ) ;
#38542=CARTESIAN_POINT ( 'NONE',  ( -37.00000000000000711, 11.74226168163341555, 0.3025107581131598611 ) ) ;
#38544=DIRECTION ( 'NONE',  ( 0.000000000000000000, 0.6745969609292663538, 0.7381862504171949890 ) ) ;
#38546=CARTESIAN_POINT ( 'NONE',  ( 12.52917170697542737, -11.52224091069466638, -7.043940186100077661 ) ) ;
#38547=VECTOR ( 'NONE', #51402, 1000.000000000000000 ) ;
#38550=ORIENTED_EDGE ( 'NONE', *, *, #37819, .T. ) ;
#38551=AXIS2_PLACEMENT_3D ( 'NONE', #29955, #14331, #5031 ) ;
#38553=DIRECTION ( 'NONE',  ( -1.000000000000000000, -0.000000000000000000, 0.000000000000000000 ) ) ;
#38554=DIRECTION ( 'NONE',  ( -1.000000000000000000, 0.000000000000000000, -0.000000000000000000 ) ) ;
#38555=FACE_OUTER_BOUND ( 'NONE', #50747, .T. ) ;
#38556=ADVANCED_FACE ( 'NONE', ( #56299 ), #474, .T. ) ;
#38557=AXIS2_PLACEMENT_3D ( 'NONE', #38491, #59423, #48171 ) ;
#38559=EDGE_LOOP ( 'NONE', ( #45934, #65169, #51933, #33274 ) ) ;
#38562=CARTESIAN_POINT ( 'NONE',  ( -37.00000000000000711, -8.534258022646161734, 8.699265615722952205 ) ) ;
#38563=LINE ( 'NONE', #53867, #31985 ) ;
#38564=AXIS2_PLACEMENT_3D ( 'NONE', #26640, #2030, #22651 ) ;
#38565=ORIENTED_EDGE ( 'NONE', *, *, #58200, .F. ) ;
#38566=ORIENTED_EDGE ( 'NONE', *, *, #61493, .T. ) ;
#38568=EDGE_CURVE ( 'NONE', #37953, #36795, #32114, .T. ) ;
#38569=ORIENTED_EDGE ( 'NONE', *, *, #25038, .F. ) ;
#38575=ADVANCED_FACE ( 'NONE', ( #31035 ), #51346, .T. ) ;
#38576=ORIENTED_EDGE ( 'NONE', *, *, #47300, .T. ) ;
#38578=VECTOR ( 'NONE', #41037, 1000.000000000000000 ) ;
#38582=AXIS2_PLACEMENT_3D ( 'NONE', #10096, #25381, #24395 ) ;
#38583=DIRECTION ( 'NONE',  ( -1.000000000000000000, 0.000000000000000000, 0.000000000000000000 ) ) ;
#38584=AXIS2_PLACEMENT_3D ( 'NONE', #41251, #36267, #6045 ) ;
#38585=EDGE_CURVE ( 'NONE', #31676, #56666, #31090, .T. ) ;
#38586=ORIENTED_EDGE ( 'NONE', *, *, #41270, .F. ) ;
#38587=DIRECTION ( 'NONE',  ( 0.000000000000000000, -0.01356324068817999808, 0.9999080150203990547 ) ) ;
#38589=ORIENTED_EDGE ( 'NONE', *, *, #37638, .T. ) ;
#38591=CARTESIAN_POINT ( 'NONE',  ( 22.05618987420085020, -11.97361567146970529, -0.7978078888370666588 ) ) ;
#38592=DIRECTION ( 'NONE',  ( 0.000000000000000000, -0.01356324068817998940, 0.9999080150203990547 ) ) ;
#38593=VERTEX_POINT ( 'NONE', #7743 ) ;
#38594=AXIS2_PLACEMENT_3D ( 'NONE', #445, #20715, #40989 ) ;
#38595=VERTEX_POINT ( 'NONE', #52956 ) ;
#38597=ORIENTED_EDGE ( 'NONE', *, *, #36510, .F. ) ;
#38599=CARTESIAN_POINT ( 'NONE',  ( 8.938435699493556541, 2.394065638922180828, -13.28818146251820309 ) ) ;
#38600=VERTEX_POINT ( 'NONE', #43293 ) ;
#38601=AXIS2_PLACEMENT_3D ( 'NONE', #61206, #1690, #37227 ) ;
#38606=CARTESIAN_POINT ( 'NONE',  ( 35.00000000000000000, -3.640372113593464576, 12.21925492305365246 ) ) ;
#38608=ORIENTED_EDGE ( 'NONE', *, *, #15156, .T. ) ;
#38609=CARTESIAN_POINT ( 'NONE',  ( 35.00000000000000000, 4.705694406421931860E-17, -3.469127814946512892E-15 ) ) ;
#38610=CIRCLE ( 'NONE', #9932, 12.18650000000000055 ) ;
#38611=VERTEX_POINT ( 'NONE', #38307 ) ;
#38613=CIRCLE ( 'NONE', #15242, 12.18650000000000055 ) ;
#38615=ORIENTED_EDGE ( 'NONE', *, *, #54431, .F. ) ;
#38616=CARTESIAN_POINT ( 'NONE',  ( -16.08885787060327033, 8.362789014594929071, 8.606209290561983138 ) ) ;
#38620=ORIENTED_EDGE ( 'NONE', *, *, #60275, .F. ) ;
#38621=VECTOR ( 'NONE', #65158, 1000.000000000000000 ) ;
#38624=ORIENTED_EDGE ( 'NONE', *, *, #61590, .T. ) ;
#38626=DIRECTION ( 'NONE',  ( 0.000000000000000000, 0.2618041379715563277, -0.9651210252299813330 ) ) ;
#38628=CARTESIAN_POINT ( 'NONE',  ( -2.532614230583026593, 5.020478806276888584, 10.89930238848911337 ) ) ;
#38629=LINE ( 'NONE', #58942, #42685 ) ;
#38630=ORIENTED_EDGE ( 'NONE', *, *, #63463, .T. ) ;
#38632=AXIS2_PLACEMENT_3D ( 'NONE', #17911, #39155, #54140 ) ;
#38633=CARTESIAN_POINT ( 'NONE',  ( -35.00000000000000000, 0.000000000000000000, 0.000000000000000000 ) ) ;
#38634=AXIS2_PLACEMENT_3D ( 'NONE', #16795, #21472, #46732 ) ;
#38638=AXIS2_PLACEMENT_3D ( 'NONE', #36496, #45819, #57117 ) ;
#38639=DIRECTION ( 'NONE',  ( -1.000000000000000000, 0.000000000000000000, 0.000000000000000000 ) ) ;
#38640=CARTESIAN_POINT ( 'NONE',  ( 35.00000000000000000, -2.936739658819788712, 11.37311665002366290 ) ) ;
#38641=CARTESIAN_POINT ( 'NONE',  ( 35.00000000000000000, -11.96656215839371917, -4.400442035670902641 ) ) ;
#38644=AXIS2_PLACEMENT_3D ( 'NONE', #59098, #9177, #24471 ) ;
#38646=EDGE_CURVE ( 'NONE', #27477, #19993, #54454, .T. ) ;
#38648=CARTESIAN_POINT ( 'NONE',  ( 12.56381792447365164, -11.46152505571988556, -3.559530320152763938 ) ) ;
#38650=CARTESIAN_POINT ( 'NONE',  ( 35.00000000000000000, 4.705694406421931860E-17, -3.469127814946512892E-15 ) ) ;
#38651=( BOUNDED_CURVE ( )  B_SPLINE_CURVE ( 3, ( #42692, #36743, #62993, #37728 ),
 .UNSPECIFIED., .F., .F. ) 
 B_SPLINE_CURVE_WITH_KNOTS ( ( 4, 4 ),
 ( 1.123686293514793100, 1.129014759054202566 ),
 .UNSPECIFIED. ) 
 CURVE ( )  GEOMETRIC_REPRESENTATION_ITEM ( )  RATIONAL_B_SPLINE_CURVE ( ( 1.000000000000000000, 0.9999976339559824012, 0.9999976339559824012, 1.000000000000000000 ) ) 
 REPRESENTATION_ITEM ( '' )  );
#38653=DIRECTION ( 'NONE',  ( 1.000000000000000000, 0.000000000000000000, 0.000000000000000000 ) ) ;
#38655=AXIS2_PLACEMENT_3D ( 'NONE', #37791, #17522, #7521 ) ;
#38658=FACE_OUTER_BOUND ( 'NONE', #9136, .T. ) ;
#38659=ADVANCED_FACE ( 'NONE', ( #57300 ), #62929, .T. ) ;
#38660=ORIENTED_EDGE ( 'NONE', *, *, #40026, .F. ) ;
#38661=ORIENTED_EDGE ( 'NONE', *, *, #37615, .T. ) ;
#38662=VERTEX_POINT ( 'NONE', #32003 ) ;
#38663=DIRECTION ( 'NONE',  ( 0.000000000000000000, -0.01356324068817999114, 0.9999080150203989437 ) ) ;
#38665=VECTOR ( 'NONE', #58245, 1000.000000000000000 ) ;
#38668=CARTESIAN_POINT ( 'NONE',  ( -35.00000000000000000, -10.92721691015459307, 4.309077947445612899 ) ) ;
#38669=CARTESIAN_POINT ( 'NONE',  ( -35.00000000000000000, 6.036400161834567513, 10.07641281632180075 ) ) ;
#38670=LINE ( 'NONE', #58974, #34419 ) ;
#38672=ORIENTED_EDGE ( 'NONE', *, *, #35330, .F. ) ;
#38673=FACE_OUTER_BOUND ( 'NONE', #34235, .T. ) ;
#38680=VERTEX_POINT ( 'NONE', #52650 ) ;
#38681=AXIS2_PLACEMENT_3D ( 'NONE', #40104, #562, #10843 ) ;
#38682=DIRECTION ( 'NONE',  ( 0.000000000000000000, 0.9467777615094560284, 0.3218879778916007850 ) ) ;
#38683=CIRCLE ( 'NONE', #37585, 4.999999999999998224 ) ;
#38687=DIRECTION ( 'NONE',  ( 0.000000000000000000, -0.01356324068817998940, 0.9999080150203990547 ) ) ;
#38688=DIRECTION ( 'NONE',  ( 1.000000000000000000, 0.000000000000000000, 0.000000000000000000 ) ) ;
#38690=CARTESIAN_POINT ( 'NONE',  ( -10.90165637462999548, -7.167514722546433070, -11.44751403622255026 ) ) ;
#38692=EDGE_CURVE ( 'NONE', #21953, #21123, #7075, .T. ) ;
#38693=ORIENTED_EDGE ( 'NONE', *, *, #45680, .F. ) ;
#38696=EDGE_CURVE ( 'NONE', #22365, #44, #37668, .T. ) ;
#38700=FACE_OUTER_BOUND ( 'NONE', #34559, .T. ) ;
#38703=VECTOR ( 'NONE', #16258, 1000.000000000000000 ) ;
#38706=EDGE_LOOP ( 'NONE', ( #37447, #41478, #39240, #60485 ) ) ;
#38707=AXIS2_PLACEMENT_3D ( 'NONE', #26631, #37601, #12312 ) ;
#38708=LINE ( 'NONE', #59009, #4232 ) ;
#38712=CARTESIAN_POINT ( 'NONE',  ( 37.00000000000000711, -10.68873102412837639, 6.950793414699901085 ) ) ;
#38716=CARTESIAN_POINT ( 'NONE',  ( -9.572767838435238374, -3.704540188508917087, 12.98284452592227289 ) ) ;
#38718=DIRECTION ( 'NONE',  ( -1.000000000000000000, 0.000000000000000000, -0.000000000000000000 ) ) ;
#38719=AXIS2_PLACEMENT_3D ( 'NONE', #23445, #64975, #29099 ) ;
#38720=DIRECTION ( 'NONE',  ( -1.000000000000000000, 0.000000000000000000, -0.000000000000000000 ) ) ;
#38721=DIRECTION ( 'NONE',  ( 1.000000000000000000, -0.000000000000000000, 0.000000000000000000 ) ) ;
#38723=ADVANCED_FACE ( 'NONE', ( #23355 ), #19693, .T. ) ;
#38724=LINE ( 'NONE', #59025, #32015 ) ;
#38726=AXIS2_PLACEMENT_3D ( 'NONE', #9166, #13496, #59726 ) ;
#38727=ORIENTED_EDGE ( 'NONE', *, *, #7823, .T. ) ;
#38728=CARTESIAN_POINT ( 'NONE',  ( -17.59845147210442917, 3.553096750747292809, 13.02522436870010303 ) ) ;
#38731=CARTESIAN_POINT ( 'NONE',  ( -18.15462106490041094, 3.496563557764767793, -11.48178370015430083 ) ) ;
#38734=CARTESIAN_POINT ( 'NONE',  ( 35.00000000000000000, -11.26103545359853264, 3.340853584269647847 ) ) ;
#38735=ADVANCED_FACE ( 'NONE', ( #29325 ), #14350, .T. ) ;
#38737=AXIS2_PLACEMENT_3D ( 'NONE', #20931, #50563, #29929 ) ;
#38738=ORIENTED_EDGE ( 'NONE', *, *, #45464, .T. ) ;
#38739=CARTESIAN_POINT ( 'NONE',  ( 35.00000000000000000, 4.705694406421931860E-17, -3.469127814946512892E-15 ) ) ;
#38740=AXIS2_PLACEMENT_3D ( 'NONE', #55759, #10191, #50767 ) ;
#38742=CARTESIAN_POINT ( 'NONE',  ( -37.00000000000000711, 0.000000000000000000, 0.000000000000000000 ) ) ;
#38743=CARTESIAN_POINT ( 'NONE',  ( -20.79170840334646542, -12.91784323155722269, -3.921648409140116698 ) ) ;
#38744=FACE_OUTER_BOUND ( 'NONE', #8803, .T. ) ;
#38745=FACE_OUTER_BOUND ( 'NONE', #20706, .T. ) ;
#38746=EDGE_CURVE ( 'NONE', #1560, #10110, #49316, .T. ) ;
#38747=DIRECTION ( 'NONE',  ( 1.000000000000000000, 0.000000000000000000, -0.000000000000000000 ) ) ;
#38748=PLANE ( 'NONE',  #22349 ) ;
#38749=VERTEX_POINT ( 'NONE', #58961 ) ;
#38750=CARTESIAN_POINT ( 'NONE',  ( -35.00000000000000000, 0.7536123767500182424, -11.72195762423409171 ) ) ;
#38751=EDGE_CURVE ( 'NONE', #65741, #19944, #65224, .T. ) ;
#38753=FACE_OUTER_BOUND ( 'NONE', #21148, .T. ) ;
#38754=ORIENTED_EDGE ( 'NONE', *, *, #31472, .F. ) ;
#38755=EDGE_LOOP ( 'NONE', ( #31047, #29581, #32900, #17555 ) ) ;
#38756=CARTESIAN_POINT ( 'NONE',  ( -18.43690493633051730, 6.168852665516345368, 12.01132493851507377 ) ) ;
#38757=EDGE_CURVE ( 'NONE', #46798, #4318, #33658, .T. ) ;
#38759=CARTESIAN_POINT ( 'NONE',  ( -3.161182887995629187, 5.208071662170946858, 10.84703524381376383 ) ) ;
#38761=DIRECTION ( 'NONE',  ( -1.000000000000000000, -0.000000000000000000, -0.000000000000000000 ) ) ;
#38764=LINE ( 'NONE', #17504, #22454 ) ;
#38765=EDGE_CURVE ( 'NONE', #56420, #38541, #5619, .T. ) ;
#38766=ORIENTED_EDGE ( 'NONE', *, *, #55500, .T. ) ;
#38767=CYLINDRICAL_SURFACE ( 'NONE', #41073, 4.999999999999999112 ) ;
#38768=CARTESIAN_POINT ( 'NONE',  ( 35.00000000000000000, 4.705694406421931860E-17, -3.469127814946512892E-15 ) ) ;
#38770=VERTEX_POINT ( 'NONE', #54626 ) ;
#38771=EDGE_CURVE ( 'NONE', #15788, #3402, #14656, .T. ) ;
#38774=ORIENTED_EDGE ( 'NONE', *, *, #34808, .F. ) ;
#38775=FACE_OUTER_BOUND ( 'NONE', #16849, .T. ) ;
#38776=CARTESIAN_POINT ( 'NONE',  ( 35.00000000000000000, 4.237620530777968852, 11.42599468261424178 ) ) ;
#38777=DIRECTION ( 'NONE',  ( 0.000000000000000000, -0.01356324068817992175, 0.9999080150203990547 ) ) ;
#38780=CARTESIAN_POINT ( 'NONE',  ( -35.00000000000000000, -10.14408668126209001, -5.921969905510467314 ) ) ;
#38781=LINE ( 'NONE', #63371, #12059 ) ;
#38782=VERTEX_POINT ( 'NONE', #38974 ) ;
#38783=AXIS2_PLACEMENT_3D ( 'NONE', #14637, #48698, #65512 ) ;
#38784=ORIENTED_EDGE ( 'NONE', *, *, #8928, .F. ) ;
#38786=CARTESIAN_POINT ( 'NONE',  ( -35.00000000000000000, -10.01317267707891467, 6.946017217729903770 ) ) ;
#38788=AXIS2_PLACEMENT_3D ( 'NONE', #30633, #50944, #65548 ) ;
#38789=ADVANCED_FACE ( 'NONE', ( #9346 ), #13691, .T. ) ;
#38791=DIRECTION ( 'NONE',  ( 0.000000000000000000, 0.01356324068817998940, -0.9999080150203990547 ) ) ;
#38792=CARTESIAN_POINT ( 'NONE',  ( -9.620557803072061986, -3.748754942421991920, -11.40376018319986606 ) ) ;
#38793=CARTESIAN_POINT ( 'NONE',  ( 35.00000000000000000, 0.4353888892050056802, 11.73808581813437080 ) ) ;
#38797=CARTESIAN_POINT ( 'NONE',  ( 35.00000000000000000, 4.705694406421931860E-17, -3.469127814946512892E-15 ) ) ;
#38798=CARTESIAN_POINT ( 'NONE',  ( 19.28625800530496903, 6.413918128308424116, 11.87904264843580471 ) ) ;
#38801=CARTESIAN_POINT ( 'NONE',  ( 35.00000000000000000, 1.591260454995240714, -12.08216339958901564 ) ) ;
#38803=AXIS2_PLACEMENT_3D ( 'NONE', #27015, #57276, #17023 ) ;
#38812=DIRECTION ( 'NONE',  ( -1.000000000000000000, 0.000000000000000000, -0.000000000000000000 ) ) ;
#38813=FACE_OUTER_BOUND ( 'NONE', #39051, .T. ) ;
#38814=EDGE_CURVE ( 'NONE', #42534, #10290, #46582, .T. ) ;
#38816=DIRECTION ( 'NONE',  ( -1.000000000000000000, 0.000000000000000000, -0.000000000000000000 ) ) ;
#38817=CYLINDRICAL_SURFACE ( 'NONE', #45848, 5.000000000000000888 ) ;
#38820=DIRECTION ( 'NONE',  ( -1.000000000000000000, 0.000000000000000000, 0.000000000000000000 ) ) ;
#38821=CARTESIAN_POINT ( 'NONE',  ( -37.00000000000000711, 0.000000000000000000, 0.000000000000000000 ) ) ;
#38822=CARTESIAN_POINT ( 'NONE',  ( -37.00000000000000711, -8.366449238204298311, -9.621072037177086145 ) ) ;
#38826=LINE ( 'NONE', #38152, #49098 ) ;
#38827=DIRECTION ( 'NONE',  ( 0.000000000000000000, -0.01356324068817999114, 0.9999080150203989437 ) ) ;
#38828=FACE_OUTER_BOUND ( 'NONE', #50581, .T. ) ;
#38834=EDGE_CURVE ( 'NONE', #43665, #6221, #65050, .T. ) ;
#38836=ADVANCED_FACE ( 'NONE', ( #40266 ), #10339, .T. ) ;
#38837=CIRCLE ( 'NONE', #10156, 4.999999999999999112 ) ;
#38838=DIRECTION ( 'NONE',  ( 1.000000000000000000, -0.000000000000000000, 0.000000000000000000 ) ) ;
#38839=FACE_OUTER_BOUND ( 'NONE', #60408, .T. ) ;
#38840=EDGE_CURVE ( 'NONE', #6120, #46319, #41585, .T. ) ;
#38842=ORIENTED_EDGE ( 'NONE', *, *, #40611, .F. ) ;
#38843=CARTESIAN_POINT ( 'NONE',  ( -35.00000000000000000, 7.474872387601008583, 9.060822531526074641 ) ) ;
#38844=( BOUNDED_CURVE ( )  B_SPLINE_CURVE ( 3, ( #24842, #61071, #35767, #10506 ),
 .UNSPECIFIED., .F., .F. ) 
 B_SPLINE_CURVE_WITH_KNOTS ( ( 4, 4 ),
 ( 4.681958569418493532, 4.712388980384689674 ),
 .UNSPECIFIED. ) 
 CURVE ( )  GEOMETRIC_REPRESENTATION_ITEM ( )  RATIONAL_B_SPLINE_CURVE ( ( 1.000000000000000000, 0.9999228339960630763, 0.9999228339960630763, 1.000000000000000000 ) ) 
 REPRESENTATION_ITEM ( '' )  );
#38846=DIRECTION ( 'NONE',  ( 1.000000000000000000, -0.000000000000000000, -0.000000000000000000 ) ) ;
#38847=ORIENTED_EDGE ( 'NONE', *, *, #21607, .F. ) ;
#38852=ORIENTED_EDGE ( 'NONE', *, *, #3057, .T. ) ;
#38853=ORIENTED_EDGE ( 'NONE', *, *, #46090, .F. ) ;
#38854=DIRECTION ( 'NONE',  ( -1.000000000000000000, 0.000000000000000000, 0.000000000000000000 ) ) ;
#38855=DIRECTION ( 'NONE',  ( 0.000000000000000000, -0.01356324068817998940, 0.9999080150203990547 ) ) ;
#38860=LINE ( 'NONE', #44168, #61958 ) ;
#38863=CARTESIAN_POINT ( 'NONE',  ( -16.29237361052064870, 7.773568625800320042, 9.141951862542200047 ) ) ;
#38864=CARTESIAN_POINT ( 'NONE',  ( 37.00000000000000711, -11.96656215839371917, -4.400442035670902641 ) ) ;
#38865=CARTESIAN_POINT ( 'NONE',  ( -35.00000000000000000, -7.817610399097453922, -8.766823244862070652 ) ) ;
#38866=CYLINDRICAL_SURFACE ( 'NONE', #22209, 12.74999999999999822 ) ;
#38867=FACE_OUTER_BOUND ( 'NONE', #24951, .T. ) ;
#38869=DIRECTION ( 'NONE',  ( 1.000000000000000000, 0.000000000000000000, 0.000000000000000000 ) ) ;
#38870=DIRECTION ( 'NONE',  ( -1.000000000000000000, 0.000000000000000000, -0.000000000000000000 ) ) ;
#38874=CARTESIAN_POINT ( 'NONE',  ( -35.00000000000000000, -8.830544224262881770, -9.196955404009390378 ) ) ;
#38875=AXIS2_PLACEMENT_3D ( 'NONE', #16362, #1727, #12336 ) ;
#38877=CIRCLE ( 'NONE', #49521, 12.74999999999999822 ) ;
#38879=DIRECTION ( 'NONE',  ( -1.000000000000000000, 0.000000000000000000, 0.000000000000000000 ) ) ;
#38880=DIRECTION ( 'NONE',  ( 1.000000000000000000, 0.000000000000000000, 0.000000000000000000 ) ) ;
#38881=CARTESIAN_POINT ( 'NONE',  ( 12.84947240711940530, -12.08188435868343902, -6.035714449063213749 ) ) ;
#38882=DIRECTION ( 'NONE',  ( 1.000000000000000000, -0.000000000000000000, 0.000000000000000000 ) ) ;
#38884=EDGE_LOOP ( 'NONE', ( #10152, #47906, #59104, #50240 ) ) ;
#38885=CYLINDRICAL_SURFACE ( 'NONE', #27146, 13.50000000000000178 ) ;
#38887=ADVANCED_FACE ( 'NONE', ( #35281 ), #45937, .T. ) ;
#38890=AXIS2_PLACEMENT_3D ( 'NONE', #53980, #19056, #3469 ) ;
#38891=DIRECTION ( 'NONE',  ( 1.000000000000000000, -0.000000000000000000, 0.000000000000000000 ) ) ;
#38893=CARTESIAN_POINT ( 'NONE',  ( -18.76908574728738088, 11.99999999999999289, 0.6354707926302536336 ) ) ;
#38894=ORIENTED_EDGE ( 'NONE', *, *, #22840, .T. ) ;
#38896=CARTESIAN_POINT ( 'NONE',  ( -35.00000000000000000, 12.08216339958900676, 1.591260454995285789 ) ) ;
#38899=EDGE_CURVE ( 'NONE', #38611, #47989, #25314, .T. ) ;
#38900=CARTESIAN_POINT ( 'NONE',  ( 6.623202313640009997, -7.527612111493656499, 11.20804235361907253 ) ) ;
#38901=ORIENTED_EDGE ( 'NONE', *, *, #47328, .T. ) ;
#38902=ORIENTED_EDGE ( 'NONE', *, *, #11536, .F. ) ;
#38903=CARTESIAN_POINT ( 'NONE',  ( -27.22222364661110916, 10.76538614228702606, 5.304738902579495097 ) ) ;
#38904=DIRECTION ( 'NONE',  ( 0.000000000000000000, -0.6745969609292717939, -0.7381862504171901040 ) ) ;
#38905=DIRECTION ( 'NONE',  ( 0.000000000000000000, 0.01356324068817998940, -0.9999080150203989437 ) ) ;
#38909=ORIENTED_EDGE ( 'NONE', *, *, #11269, .T. ) ;
#38910=ORIENTED_EDGE ( 'NONE', *, *, #7328, .T. ) ;
#38911=VERTEX_POINT ( 'NONE', #40608 ) ;
#38912=CARTESIAN_POINT ( 'NONE',  ( -35.00000000000000000, 0.000000000000000000, 0.000000000000000000 ) ) ;
#38914=CARTESIAN_POINT ( 'NONE',  ( -28.85619398320021745, 3.750539801530000439, 11.39883551934754280 ) ) ;
#38917=DIRECTION ( 'NONE',  ( -1.000000000000000000, 0.000000000000000000, -0.000000000000000000 ) ) ;
#38918=EDGE_CURVE ( 'NONE', #27953, #54227, #20668, .T. ) ;
#38920=ORIENTED_EDGE ( 'NONE', *, *, #62585, .F. ) ;
#38921=AXIS2_PLACEMENT_3D ( 'NONE', #50596, #60891, #14339 ) ;
#38923=CARTESIAN_POINT ( 'NONE',  ( 21.90174657591892071, -11.97747433400148864, -0.7349207973210698519 ) ) ;
#38924=DIRECTION ( 'NONE',  ( -1.000000000000000000, 0.000000000000000000, 0.000000000000000000 ) ) ;
#38925=ORIENTED_EDGE ( 'NONE', *, *, #33784, .F. ) ;
#38930=CARTESIAN_POINT ( 'NONE',  ( 35.00000000000000000, 4.705694406421931860E-17, -3.469127814946512892E-15 ) ) ;
#38931=ORIENTED_EDGE ( 'NONE', *, *, #59047, .T. ) ;
#38932=ORIENTED_EDGE ( 'NONE', *, *, #62229, .T. ) ;
#38934=DIRECTION ( 'NONE',  ( 0.000000000000000000, -0.01356324068817992001, 0.9999080150203990547 ) ) ;
#38940=DIRECTION ( 'NONE',  ( -1.000000000000000000, 0.000000000000000000, 0.000000000000000000 ) ) ;
#38941=VERTEX_POINT ( 'NONE', #35923 ) ;
#38942=CYLINDRICAL_SURFACE ( 'NONE', #42280, 12.18649999999999878 ) ;
#38944=EDGE_LOOP ( 'NONE', ( #20685, #4650, #7683, #64990 ) ) ;
#38945=CARTESIAN_POINT ( 'NONE',  ( -17.08212596820160556, 7.928502486991608755, 9.008165934404118502 ) ) ;
#38946=DIRECTION ( 'NONE',  ( -1.000000000000000000, 0.000000000000000000, -0.000000000000000000 ) ) ;
#38948=ORIENTED_EDGE ( 'NONE', *, *, #33472, .F. ) ;
#38951=ADVANCED_FACE ( 'NONE', ( #30953 ), #5716, .T. ) ;
#38952=ORIENTED_EDGE ( 'NONE', *, *, #22426, .T. ) ;
#38955=CARTESIAN_POINT ( 'NONE',  ( -29.28424789664604333, 2.973701217869066049, 13.19321996469480318 ) ) ;
#38956=DIRECTION ( 'NONE',  ( 0.1024315404614497965, 0.9947400562552481951, 0.000000000000000000 ) ) ;
#38958=EDGE_LOOP ( 'NONE', ( #51919, #59840, #115, #22720 ) ) ;
#38959=DIRECTION ( 'NONE',  ( -1.000000000000000000, -0.000000000000000000, 0.000000000000000000 ) ) ;
#38960=CIRCLE ( 'NONE', #27272, 12.18650000000000055 ) ;
#38962=EDGE_CURVE ( 'NONE', #19382, #53566, #33266, .T. ) ;
#38967=CARTESIAN_POINT ( 'NONE',  ( 35.00000000000000000, 9.063649021438955344, -8.146229107149434157 ) ) ;
#38970=LINE ( 'NONE', #47637, #36299 ) ;
#38972=CARTESIAN_POINT ( 'NONE',  ( 37.00000000000000711, -10.32377448871663006, 6.475373545682407972 ) ) ;
#38974=CARTESIAN_POINT ( 'NONE',  ( 35.00000000000000000, 9.063649021438955344, -8.146229107149434157 ) ) ;
#38975=DIRECTION ( 'NONE',  ( 0.000000000000000000, 0.01356324068817992175, -0.9999080150203990547 ) ) ;
#38976=ORIENTED_EDGE ( 'NONE', *, *, #19020, .F. ) ;
#38977=VERTEX_POINT ( 'NONE', #26302 ) ;
#38978=EDGE_LOOP ( 'NONE', ( #27579, #16058, #59634, #43991 ) ) ;
#38979=CARTESIAN_POINT ( 'NONE',  ( 36.00000000000000711, 12.74613886779084737, -0.3137578094509725357 ) ) ;
#38980=ORIENTED_EDGE ( 'NONE', *, *, #1424, .F. ) ;
#38984=CARTESIAN_POINT ( 'NONE',  ( 47.00000000000000711, 4.705694406421931860E-17, -3.469127814946512892E-15 ) ) ;
#38985=EDGE_LOOP ( 'NONE', ( #43017, #27744, #37182, #38576 ) ) ;
#38987=AXIS2_PLACEMENT_3D ( 'NONE', #19068, #64592, #55287 ) ;
#38991=ORIENTED_EDGE ( 'NONE', *, *, #947, .F. ) ;
#38993=ORIENTED_EDGE ( 'NONE', *, *, #22358, .F. ) ;
#38994=DIRECTION ( 'NONE',  ( -1.000000000000000000, 0.000000000000000000, -0.000000000000000000 ) ) ;
#38995=VERTEX_POINT ( 'NONE', #17649 ) ;
#38996=CIRCLE ( 'NONE', #47507, 4.999999999999999112 ) ;
#38998=DIRECTION ( 'NONE',  ( 0.000000000000000000, 0.01356324068817998940, -0.9999080150203990547 ) ) ;
#38999=CARTESIAN_POINT ( 'NONE',  ( 35.00000000000000000, 4.705694406421931860E-17, -3.469127814946512892E-15 ) ) ;
#39001=EDGE_CURVE ( 'NONE', #7923, #50600, #23694, .T. ) ;
#39003=AXIS2_PLACEMENT_3D ( 'NONE', #242, #20515, #40800 ) ;
#39004=CARTESIAN_POINT ( 'NONE',  ( -36.00000000000000711, 4.824807283154123105, 11.80185301892982608 ) ) ;
#39005=DIRECTION ( 'NONE',  ( -1.000000000000000000, -1.836970198721029688E-16, -0.000000000000000000 ) ) ;
#39006=ORIENTED_EDGE ( 'NONE', *, *, #27301, .T. ) ;
#39007=CARTESIAN_POINT ( 'NONE',  ( -4.984433189575353751, -1.083073623696802379, 13.45752292036589637 ) ) ;
#39008=ORIENTED_EDGE ( 'NONE', *, *, #23283, .T. ) ;
#39009=ORIENTED_EDGE ( 'NONE', *, *, #36734, .F. ) ;
#39014=DIRECTION ( 'NONE',  ( -1.000000000000000000, -0.000000000000000000, -0.000000000000000000 ) ) ;
#39016=EDGE_CURVE ( 'NONE', #33099, #61338, #56638, .T. ) ;
#39017=CARTESIAN_POINT ( 'NONE',  ( 35.00000000000000000, -11.56998259273180274, -3.827046518385039064 ) ) ;
#39019=EDGE_CURVE ( 'NONE', #29583, #20925, #22646, .T. ) ;
#39020=ADVANCED_FACE ( 'NONE', ( #21659 ), #63494, .T. ) ;
#39021=ORIENTED_EDGE ( 'NONE', *, *, #23826, .F. ) ;
#39022=CARTESIAN_POINT ( 'NONE',  ( 37.00000000000000711, -3.287724142101330571, 11.73463472867579149 ) ) ;
#39024=EDGE_CURVE ( 'NONE', #58596, #5514, #26961, .T. ) ;
#39025=CARTESIAN_POINT ( 'NONE',  ( -35.00000000000000000, 10.42955799785328708, -6.303578524886837009 ) ) ;
#39027=AXIS2_PLACEMENT_3D ( 'NONE', #4421, #55268, #50626 ) ;
#39028=ADVANCED_FACE ( 'NONE', ( #37911 ), #62199, .T. ) ;
#39029=AXIS2_PLACEMENT_3D ( 'NONE', #906, #16202, #31491 ) ;
#39030=( BOUNDED_CURVE ( )  B_SPLINE_CURVE ( 3, ( #19152, #59086, #55050, #59391 ),
 .UNSPECIFIED., .F., .F. ) 
 B_SPLINE_CURVE_WITH_KNOTS ( ( 4, 4 ),
 ( 2.476619846412093651, 2.515060261699084254 ),
 .UNSPECIFIED. ) 
 CURVE ( )  GEOMETRIC_REPRESENTATION_ITEM ( )  RATIONAL_B_SPLINE_CURVE ( ( 1.000000000000000000, 0.9998768649967908484, 0.9998768649967908484, 1.000000000000000000 ) ) 
 REPRESENTATION_ITEM ( '' )  );
#39032=EDGE_CURVE ( 'NONE', #20284, #44987, #51597, .T. ) ;
#39033=CARTESIAN_POINT ( 'NONE',  ( 37.00000000000000711, -0.3137578094510115045, -12.74613886779085092 ) ) ;
#39034=ORIENTED_EDGE ( 'NONE', *, *, #39948, .F. ) ;
#39036=DIRECTION ( 'NONE',  ( 0.000000000000000000, 0.5243256840888503856, 0.8515178078024905339 ) ) ;
#39038=AXIS2_PLACEMENT_3D ( 'NONE', #50789, #5240, #9542 ) ;
#39039=B_SPLINE_CURVE_WITH_KNOTS ( 'NONE', 3,
 ( #57109, #52459, #25867, #20862, #36130, #21184, #56441, #26838, #10888, #31805, #6570, #911, #57429, #41453, #47139, #1591 ),
 .UNSPECIFIED., .F., .F.,
 ( 4, 2, 2, 2, 2, 2, 2, 4 ),
 ( 3.496446946337351263E-18, 0.001151362128401672283, 0.001727043192602508099, 0.002302724256803344131, 0.003454086385205015763, 0.004605448513606687395, 0.006908172770410029792, 0.009210897027213369587 ),
 .UNSPECIFIED. ) ;
#39041=ADVANCED_FACE ( 'NONE', ( #6357 ), #11654, .T. ) ;
#39042=DIRECTION ( 'NONE',  ( -1.000000000000000000, 0.000000000000000000, 0.000000000000000000 ) ) ;
#39044=ORIENTED_EDGE ( 'NONE', *, *, #19413, .F. ) ;
#39045=DIRECTION ( 'NONE',  ( -0.000000000000000000, -0.000000000000000000, -1.000000000000000000 ) ) ;
#39046=CARTESIAN_POINT ( 'NONE',  ( -36.00000000000000711, -2.080187960898653543, 12.57916205664480636 ) ) ;
#39047=CARTESIAN_POINT ( 'NONE',  ( -16.98800322446194855, 2.922502605998049674, -11.63868456991314027 ) ) ;
#39048=ORIENTED_EDGE ( 'NONE', *, *, #56137, .F. ) ;
#39049=CARTESIAN_POINT ( 'NONE',  ( 0.000000000000000000, -1.734723475976807094E-15, -13.50000000000000178 ) ) ;
#39051=EDGE_LOOP ( 'NONE', ( #52621, #37085, #32476, #255 ) ) ;
#39052=ORIENTED_EDGE ( 'NONE', *, *, #42208, .T. ) ;
#39054=ORIENTED_EDGE ( 'NONE', *, *, #11396, .T. ) ;
#39058=LINE ( 'NONE', #13775, #1595 ) ;
#39060=EDGE_LOOP ( 'NONE', ( #57329, #16950, #44496, #20978 ) ) ;
#39063=DIRECTION ( 'NONE',  ( -1.000000000000000000, 0.000000000000000000, 0.000000000000000000 ) ) ;
#39064=ORIENTED_EDGE ( 'NONE', *, *, #19608, .T. ) ;
#39066=LINE ( 'NONE', #59362, #64477 ) ;
#39069=CARTESIAN_POINT ( 'NONE',  ( -24.35620976915924984, 10.90526090019620398, 7.960195681111406962 ) ) ;
#39070=EDGE_CURVE ( 'NONE', #7420, #64126, #6745, .T. ) ;
#39071=CARTESIAN_POINT ( 'NONE',  ( 37.00000000000000711, 4.705694406421931860E-17, -3.469127814946512892E-15 ) ) ;
#39072=DIRECTION ( 'NONE',  ( 0.000000000000000000, -0.9970832820307047317, -0.07632122047555413291 ) ) ;
#39073=CARTESIAN_POINT ( 'NONE',  ( 35.00000000000000000, 12.54989509947654014, 2.250029553613615452 ) ) ;
#39074=ORIENTED_EDGE ( 'NONE', *, *, #34192, .F. ) ;
#39075=AXIS2_PLACEMENT_3D ( 'NONE', #7372, #63237, #19983 ) ;
#39076=ORIENTED_EDGE ( 'NONE', *, *, #34753, .F. ) ;
#39082=CIRCLE ( 'NONE', #35893, 4.999999999999999112 ) ;
#39083=CARTESIAN_POINT ( 'NONE',  ( -35.00000000000000000, 0.000000000000000000, 0.000000000000000000 ) ) ;
#39084=DIRECTION ( 'NONE',  ( -0.000000000000000000, -0.000000000000000000, -1.000000000000000000 ) ) ;
#39087=EDGE_CURVE ( 'NONE', #65435, #27379, #61936, .T. ) ;
#39089=ORIENTED_EDGE ( 'NONE', *, *, #59384, .T. ) ;
#39091=ORIENTED_EDGE ( 'NONE', *, *, #6848, .T. ) ;
#39092=EDGE_CURVE ( 'NONE', #48895, #51071, #54499, .T. ) ;
#39093=DIRECTION ( 'NONE',  ( 1.000000000000000000, -0.000000000000000000, 0.000000000000000000 ) ) ;
#39094=DIRECTION ( 'NONE',  ( 0.000000000000000000, -0.01356324068817999114, 0.9999080150203989437 ) ) ;
#39095=CARTESIAN_POINT ( 'NONE',  ( 29.03457606387295087, 4.854210015632069997, 10.97436308512422265 ) ) ;
#39097=FACE_OUTER_BOUND ( 'NONE', #13233, .T. ) ;
#39098=CARTESIAN_POINT ( 'NONE',  ( -28.25671366997987732, 12.49082151344278735, -5.130654606202838863 ) ) ;
#39100=AXIS2_PLACEMENT_3D ( 'NONE', #40814, #41783, #587 ) ;
#39101=CARTESIAN_POINT ( 'NONE',  ( -10.87579916591577778, -6.848527916712992436, -9.862315760539463128 ) ) ;
#39102=EDGE_CURVE ( 'NONE', #39990, #62542, #47093, .T. ) ;
#39103=CARTESIAN_POINT ( 'NONE',  ( -25.86628395826706850, 5.139808748864376220, 10.84354029019568522 ) ) ;
#39106=EDGE_CURVE ( 'NONE', #60850, #14900, #60854, .T. ) ;
#39108=CARTESIAN_POINT ( 'NONE',  ( 35.00000000000000000, -11.81949347079744506, 2.968224442958526943 ) ) ;
#39109=DIRECTION ( 'NONE',  ( -1.000000000000000000, 0.000000000000000000, -0.000000000000000000 ) ) ;
#39110=ADVANCED_FACE ( 'NONE', ( #3989 ), #13305, .T. ) ;
#39111=AXIS2_PLACEMENT_3D ( 'NONE', #56524, #51559, #57183 ) ;
#39112=EDGE_CURVE ( 'NONE', #36091, #53066, #24779, .T. ) ;
#39115=AXIS2_PLACEMENT_3D ( 'NONE', #61636, #1484, #22385 ) ;
#39117=CARTESIAN_POINT ( 'NONE',  ( 35.00000000000000000, 9.926225166347027340, -6.280308599560179061 ) ) ;
#39122=CIRCLE ( 'NONE', #15765, 12.18650000000000233 ) ;
#39123=CARTESIAN_POINT ( 'NONE',  ( -10.84711731306251714, -4.830322288942776154, -12.61315300571293108 ) ) ;
#39124=CYLINDRICAL_SURFACE ( 'NONE', #5587, 5.000000000000000888 ) ;
#39125=LINE ( 'NONE', #2926, #5239 ) ;
#39127=DIRECTION ( 'NONE',  ( -1.000000000000000000, 0.000000000000000000, -0.000000000000000000 ) ) ;
#39128=CARTESIAN_POINT ( 'NONE',  ( -35.00000000000000000, 10.92721691015462149, -4.309077947445535628 ) ) ;
#39130=ORIENTED_EDGE ( 'NONE', *, *, #25753, .T. ) ;
#39131=DIRECTION ( 'NONE',  ( 1.000000000000000000, -0.000000000000000000, 0.000000000000000000 ) ) ;
#39132=FACE_OUTER_BOUND ( 'NONE', #12810, .T. ) ;
#39135=CARTESIAN_POINT ( 'NONE',  ( -35.00000000000000000, -5.672855678558757830, 10.28547182238005853 ) ) ;
#39136=CARTESIAN_POINT ( 'NONE',  ( -29.61291272822813170, 2.156105836073342275, -11.83797064166018664 ) ) ;
#39138=ORIENTED_EDGE ( 'NONE', *, *, #44975, .T. ) ;
#39139=ORIENTED_EDGE ( 'NONE', *, *, #36398, .T. ) ;
#39140=CARTESIAN_POINT ( 'NONE',  ( -18.17105223446473872, -5.570524445111396439, -10.62960849765157789 ) ) ;
#39141=ORIENTED_EDGE ( 'NONE', *, *, #56234, .T. ) ;
#39144=EDGE_CURVE ( 'NONE', #9770, #27200, #42794, .T. ) ;
#39147=VERTEX_POINT ( 'NONE', #64799 ) ;
#39148=CARTESIAN_POINT ( 'NONE',  ( -35.00000000000000000, 0.000000000000000000, 0.000000000000000000 ) ) ;
#39151=CARTESIAN_POINT ( 'NONE',  ( 24.90165730046861370, -0.3389098318347745220, 13.50162224760967256 ) ) ;
#39152=VERTEX_POINT ( 'NONE', #8009 ) ;
#39155=DIRECTION ( 'NONE',  ( -1.000000000000000000, 0.000000000000000000, 0.000000000000000000 ) ) ;
#39158=ORIENTED_EDGE ( 'NONE', *, *, #15811, .T. ) ;
#39159=CARTESIAN_POINT ( 'NONE',  ( 12.52750123246316072, 0.4973700281276248192, 13.49083477977253764 ) ) ;
#39160=CARTESIAN_POINT ( 'NONE',  ( -37.00000000000000711, 0.000000000000000000, 0.000000000000000000 ) ) ;
#39161=AXIS2_PLACEMENT_3D ( 'NONE', #29255, #18049, #39879 ) ;
#39162=DIRECTION ( 'NONE',  ( 0.000000000000000000, 0.01356324068817998940, -0.9999080150203989437 ) ) ;
#39163=DIRECTION ( 'NONE',  ( 0.000000000000000000, -0.9467777615094536969, -0.3218879778916073908 ) ) ;
#39167=VECTOR ( 'NONE', #26292, 1000.000000000000000 ) ;
#39170=CARTESIAN_POINT ( 'NONE',  ( -17.69949227665007641, 6.590587637064748705, 10.03069147607176426 ) ) ;
#39174=ADVANCED_FACE ( 'NONE', ( #19924 ), #9597, .T. ) ;
#39178=CARTESIAN_POINT ( 'NONE',  ( 35.00000000000000000, -10.80631716521670427, -4.603882218679513194 ) ) ;
#39179=FACE_OUTER_BOUND ( 'NONE', #52679, .T. ) ;
#39180=AXIS2_PLACEMENT_3D ( 'NONE', #45725, #20791, #15777 ) ;
#39182=VERTEX_POINT ( 'NONE', #14582 ) ;
#39185=FACE_OUTER_BOUND ( 'NONE', #43225, .T. ) ;
#39187=CARTESIAN_POINT ( 'NONE',  ( -10.86097166128075386, -8.305831640360002766, 10.65335268811077896 ) ) ;
#39189=VERTEX_POINT ( 'NONE', #35201 ) ;
#39190=CARTESIAN_POINT ( 'NONE',  ( 35.00000000000000000, -12.68495603654572434, -1.286231064351273101 ) ) ;
#39191=CARTESIAN_POINT ( 'NONE',  ( -35.00000000000000000, -0.8294751490780184477, 12.15823808070322443 ) ) ;
#39192=CARTESIAN_POINT ( 'NONE',  ( 9.627852802940182642, 2.216197012197528071, 11.79553571166074555 ) ) ;
#39194=EDGE_CURVE ( 'NONE', #24707, #50839, #26915, .T. ) ;
#39195=AXIS2_PLACEMENT_3D ( 'NONE', #34527, #54826, #14873 ) ;
#39197=FACE_OUTER_BOUND ( 'NONE', #63736, .T. ) ;
#39198=ORIENTED_EDGE ( 'NONE', *, *, #11944, .F. ) ;
#39199=AXIS2_PLACEMENT_3D ( 'NONE', #8353, #3392, #59551 ) ;
#39201=ADVANCED_FACE ( 'NONE', ( #36181 ), #30234, .T. ) ;
#39202=EDGE_LOOP ( 'NONE', ( #21316, #61985, #27349, #38931 ) ) ;
#39206=DIRECTION ( 'NONE',  ( 1.000000000000000000, 0.000000000000000000, 0.000000000000000000 ) ) ;
#39207=AXIS2_PLACEMENT_3D ( 'NONE', #42809, #33162, #28497 ) ;
#39208=ORIENTED_EDGE ( 'NONE', *, *, #16835, .F. ) ;
#39209=EDGE_LOOP ( 'NONE', ( #22955, #2898, #19947, #14521 ) ) ;
#39211=CARTESIAN_POINT ( 'NONE',  ( -27.27855387000350262, 10.59660315834921640, 5.631341004100471892 ) ) ;
#39214=CARTESIAN_POINT ( 'NONE',  ( -35.00000000000000000, 8.258652103341553641, -8.352657516904583801 ) ) ;
#39218=EDGE_LOOP ( 'NONE', ( #44634, #13743, #13553, #14659 ) ) ;
#39219=ORIENTED_EDGE ( 'NONE', *, *, #27374, .F. ) ;
#39220=VECTOR ( 'NONE', #26351, 1000.000000000000000 ) ;
#39221=VERTEX_POINT ( 'NONE', #15578 ) ;
#39223=DIRECTION ( 'NONE',  ( 0.000000000000000000, 0.2960891610144510966, 0.9551603052523478521 ) ) ;
#39225=ORIENTED_EDGE ( 'NONE', *, *, #525, .T. ) ;
#39228=ADVANCED_FACE ( 'NONE', ( #50531 ), #9951, .T. ) ;
#39231=CARTESIAN_POINT ( 'NONE',  ( -35.00000000000000000, 0.000000000000000000, 0.000000000000000000 ) ) ;
#39232=CARTESIAN_POINT ( 'NONE',  ( 35.00000000000000000, 6.657191900728455458, 9.677500615117825333 ) ) ;
#39233=ORIENTED_EDGE ( 'NONE', *, *, #5438, .F. ) ;
#39236=ORIENTED_EDGE ( 'NONE', *, *, #8736, .F. ) ;
#39237=LINE ( 'NONE', #44890, #6157 ) ;
#39239=EDGE_CURVE ( 'NONE', #45342, #27199, #34552, .T. ) ;
#39240=ORIENTED_EDGE ( 'NONE', *, *, #5963, .F. ) ;
#39241=EDGE_LOOP ( 'NONE', ( #27316, #62143, #51593, #58124 ) ) ;
#39246=CARTESIAN_POINT ( 'NONE',  ( -35.00000000000000000, -2.627174906296831480, -11.44858830469743083 ) ) ;
#39251=ORIENTED_EDGE ( 'NONE', *, *, #279, .F. ) ;
#39252=CIRCLE ( 'NONE', #10569, 12.75000000000000178 ) ;
#39254=DIRECTION ( 'NONE',  ( 1.000000000000000000, -0.000000000000000000, 0.000000000000000000 ) ) ;
#39257=CARTESIAN_POINT ( 'NONE',  ( 37.00000000000000711, 10.12742074351896449, -7.745827850123049529 ) ) ;
#39260=EDGE_CURVE ( 'NONE', #42105, #53879, #40870, .T. ) ;
#39262=EDGE_LOOP ( 'NONE', ( #3438, #39747, #7425, #21513 ) ) ;
#39266=CARTESIAN_POINT ( 'NONE',  ( -27.19357181888462094, -12.48377454417556542, 5.138615876886901468 ) ) ;
#39267=LINE ( 'NONE', #30285, #39341 ) ;
#39268=CARTESIAN_POINT ( 'NONE',  ( -30.07167209738885560, 0.1566904097641563520, 13.50094810325072814 ) ) ;
#39270=CARTESIAN_POINT ( 'NONE',  ( 13.26561344960581934, 10.13979182165873993, -6.421342877150610917 ) ) ;
#39272=CIRCLE ( 'NONE', #2115, 12.75000000000000178 ) ;
#39275=ADVANCED_FACE ( 'NONE', ( #25909 ), #46834, .T. ) ;
#39277=EDGE_CURVE ( 'NONE', #39221, #52020, #27523, .T. ) ;
#39280=EDGE_CURVE ( 'NONE', #19066, #24709, #57687, .T. ) ;
#39281=DIRECTION ( 'NONE',  ( -0.9029087107030919768, 0.4298323628305345534, 0.000000000000000000 ) ) ;
#39282=CARTESIAN_POINT ( 'NONE',  ( -37.00000000000000711, -3.614449339633411196, -11.17622378668010441 ) ) ;
#39283=DIRECTION ( 'NONE',  ( -1.000000000000000000, 0.000000000000000000, 0.000000000000000000 ) ) ;
#39284=CIRCLE ( 'NONE', #64763, 4.999999999999999112 ) ;
#39285=EDGE_CURVE ( 'NONE', #14592, #28690, #48146, .T. ) ;
#39286=ORIENTED_EDGE ( 'NONE', *, *, #54731, .T. ) ;
#39287=CARTESIAN_POINT ( 'NONE',  ( 10.35765492805355592, -11.92981863842239498, -1.311496141409351335 ) ) ;
#39289=CARTESIAN_POINT ( 'NONE',  ( -4.989057617119011745, -0.9162120371760335003, 25.00000000000000000 ) ) ;
#39290=LINE ( 'NONE', #3763, #34399 ) ;
#39291=B_SPLINE_CURVE_WITH_KNOTS ( 'NONE', 3,
 ( #31038, #41668, #51350, #2703, #62849, #52878, #60984, #55982, #10417, #25731 ),
 .UNSPECIFIED., .F., .F.,
 ( 4, 2, 2, 2, 4 ),
 ( 4.336808689942017736E-19, 0.0007897640485358541377, 0.001579528097071707842, 0.002369292145607561437, 0.003159056194143415250 ),
 .UNSPECIFIED. ) ;
#39293=ORIENTED_EDGE ( 'NONE', *, *, #44789, .F. ) ;
#39294=ORIENTED_EDGE ( 'NONE', *, *, #41219, .T. ) ;
#39298=VERTEX_POINT ( 'NONE', #61795 ) ;
#39300=CARTESIAN_POINT ( 'NONE',  ( -37.00000000000000711, 0.000000000000000000, 0.000000000000000000 ) ) ;
#39301=AXIS2_PLACEMENT_3D ( 'NONE', #15171, #5552, #30146 ) ;
#39303=CARTESIAN_POINT ( 'NONE',  ( 36.00000000000000711, 7.608228585767871976, 10.23119532541064203 ) ) ;
#39304=ADVANCED_FACE ( 'NONE', ( #32827 ), #42820, .T. ) ;
#39305=ORIENTED_EDGE ( 'NONE', *, *, #50179, .T. ) ;
#39306=DIRECTION ( 'NONE',  ( 1.000000000000000000, 0.000000000000000000, 0.000000000000000000 ) ) ;
#39307=DIRECTION ( 'NONE',  ( 0.000000000000000000, 0.01356324068817998940, -0.9999080150203989437 ) ) ;
#39308=DIRECTION ( 'NONE',  ( 0.000000000000000000, -0.01356324068818000328, 0.9999080150203990547 ) ) ;
#39309=CARTESIAN_POINT ( 'NONE',  ( -27.30970368864378273, -11.82098433594888753, -2.066507538000776467 ) ) ;
#39310=ORIENTED_EDGE ( 'NONE', *, *, #35423, .T. ) ;
#39311=CYLINDRICAL_SURFACE ( 'NONE', #64938, 10.70557198542813815 ) ;
#39312=ORIENTED_EDGE ( 'NONE', *, *, #2130, .F. ) ;
#39314=CIRCLE ( 'NONE', #47827, 12.18650000000000055 ) ;
#39315=VERTEX_POINT ( 'NONE', #56841 ) ;
#39316=CARTESIAN_POINT ( 'NONE',  ( -29.41315789147035886, 0.9355746134413824855, -11.96533147116139162 ) ) ;
#39317=DIRECTION ( 'NONE',  ( -1.000000000000000000, 0.000000000000000000, -0.000000000000000000 ) ) ;
#39318=CARTESIAN_POINT ( 'NONE',  ( -35.00000000000000000, -10.93004082984014147, -6.564808257521884904 ) ) ;
#39319=LINE ( 'NONE', #32673, #60894 ) ;
#39321=DIRECTION ( 'NONE',  ( 0.000000000000000000, 0.01356324068817992175, -0.9999080150203990547 ) ) ;
#39326=CIRCLE ( 'NONE', #10648, 12.18649999999999878 ) ;
#39329=ORIENTED_EDGE ( 'NONE', *, *, #31910, .F. ) ;
#39333=DIRECTION ( 'NONE',  ( 1.000000000000000000, -0.000000000000000000, 0.000000000000000000 ) ) ;
#39334=CARTESIAN_POINT ( 'NONE',  ( -35.00000000000000000, 8.389074212634412220, -8.839356091079954680 ) ) ;
#39338=ADVANCED_FACE ( 'NONE', ( #57480 ), #11905, .T. ) ;
#39340=AXIS2_PLACEMENT_3D ( 'NONE', #23179, #43120, #32484 ) ;
#39341=VECTOR ( 'NONE', #49917, 1000.000000000000000 ) ;
#39342=AXIS2_PLACEMENT_3D ( 'NONE', #27944, #22963, #36355 ) ;
#39343=CARTESIAN_POINT ( 'NONE',  ( -36.00000000000000711, 12.54989509947650994, 2.250029553613800637 ) ) ;
#39344=VERTEX_POINT ( 'NONE', #6938 ) ;
#39349=AXIS2_PLACEMENT_3D ( 'NONE', #35032, #44062, #65318 ) ;
#39350=EDGE_CURVE ( 'NONE', #63989, #34225, #36443, .T. ) ;
#39351=CIRCLE ( 'NONE', #63794, 5.000000000000000000 ) ;
#39352=VECTOR ( 'NONE', #36291, 1000.000000000000000 ) ;
#39354=VECTOR ( 'NONE', #54819, 1000.000000000000000 ) ;
#39356=ORIENTED_EDGE ( 'NONE', *, *, #57670, .F. ) ;
#39357=DIRECTION ( 'NONE',  ( 1.000000000000000000, -0.000000000000000000, 0.000000000000000000 ) ) ;
#39358=DIRECTION ( 'NONE',  ( 0.000000000000000000, 0.8827602140260332186, -0.4698238015817333135 ) ) ;
#39359=CARTESIAN_POINT ( 'NONE',  ( 0.6599377198674351019, -0.1505700908830693296, 12.00187902586435840 ) ) ;
#39360=AXIS2_PLACEMENT_3D ( 'NONE', #33930, #3049, #63858 ) ;
#39361=EDGE_CURVE ( 'NONE', #11586, #42316, #16281, .T. ) ;
#39363=CARTESIAN_POINT ( 'NONE',  ( 37.00000000000000711, 8.766823244861988940, -7.817610399097547180 ) ) ;
#39364=CIRCLE ( 'NONE', #11783, 12.18649999999999878 ) ;
#39367=DIRECTION ( 'NONE',  ( 1.000000000000000000, 0.000000000000000000, 0.000000000000000000 ) ) ;
#39368=CARTESIAN_POINT ( 'NONE',  ( -17.50299937445415566, 2.687489394990541847, -11.69635546961540129 ) ) ;
#39369=ORIENTED_EDGE ( 'NONE', *, *, #36627, .T. ) ;
#39370=CARTESIAN_POINT ( 'NONE',  ( -2.952869152607106251, 25.00000000000000000, 3.755417052241485365 ) ) ;
#39371=CARTESIAN_POINT ( 'NONE',  ( 35.00000000000000000, -2.185196060783960892, -11.54110654723648466 ) ) ;
#39373=ORIENTED_EDGE ( 'NONE', *, *, #3045, .F. ) ;
#39374=CARTESIAN_POINT ( 'NONE',  ( -36.00000000000000711, -12.54989509947649573, -2.250029553613892563 ) ) ;
#39376=CIRCLE ( 'NONE', #10716, 12.18650000000000233 ) ;
#39377=AXIS2_PLACEMENT_3D ( 'NONE', #6199, #31764, #1552 ) ;
#39378=VERTEX_POINT ( 'NONE', #58810 ) ;
#39382=CARTESIAN_POINT ( 'NONE',  ( -36.00000000000000711, 3.033604067594749765, -12.38385022362078836 ) ) ;
#39383=ADVANCED_FACE ( 'NONE', ( #23538 ), #44136, .T. ) ;
#39384=VECTOR ( 'NONE', #29433, 1000.000000000000000 ) ;
#39388=EDGE_CURVE ( 'NONE', #61571, #63912, #21608, .T. ) ;
#39389=CYLINDRICAL_SURFACE ( 'NONE', #42611, 12.75000000000000178 ) ;
#39390=VERTEX_POINT ( 'NONE', #8555 ) ;
#39393=VERTEX_POINT ( 'NONE', #43812 ) ;
#39394=CARTESIAN_POINT ( 'NONE',  ( -26.04781212229947229, 12.02259665859258675, 6.141663214695094020 ) ) ;
#39395=AXIS2_PLACEMENT_3D ( 'NONE', #52181, #25019, #65549 ) ;
#39397=DIRECTION ( 'NONE',  ( 0.000000000000000000, 0.01356324068817998940, -0.9999080150203990547 ) ) ;
#39399=EDGE_CURVE ( 'NONE', #29699, #45790, #48815, .T. ) ;
#39400=CARTESIAN_POINT ( 'NONE',  ( 23.11218445469129890, -3.961089654181102482, 11.33103279473652591 ) ) ;
#39401=DIRECTION ( 'NONE',  ( 0.000000000000000000, 0.6943713148249588407, -0.7196168960969843154 ) ) ;
#39402=LINE ( 'NONE', #49723, #24595 ) ;
#39403=ORIENTED_EDGE ( 'NONE', *, *, #13601, .F. ) ;
#39404=AXIS2_PLACEMENT_3D ( 'NONE', #16095, #12403, #2118 ) ;
#39405=( BOUNDED_CURVE ( )  B_SPLINE_CURVE ( 3, ( #1439, #16396, #46328, #22022 ),
 .UNSPECIFIED., .F., .F. ) 
 B_SPLINE_CURVE_WITH_KNOTS ( ( 4, 4 ),
 ( 5.457079895576344875, 5.508852664714265046 ),
 .UNSPECIFIED. ) 
 CURVE ( )  GEOMETRIC_REPRESENTATION_ITEM ( )  RATIONAL_B_SPLINE_CURVE ( ( 1.000000000000000000, 0.9997766441710536078, 0.9997766441710536078, 1.000000000000000000 ) ) 
 REPRESENTATION_ITEM ( '' )  );
#39407=CARTESIAN_POINT ( 'NONE',  ( 35.00000000000000000, 4.705694406421931860E-17, -3.469127814946512892E-15 ) ) ;
#39409=VECTOR ( 'NONE', #13179, 1000.000000000000000 ) ;
#39415=DIRECTION ( 'NONE',  ( 1.000000000000000000, 0.000000000000000000, 0.000000000000000000 ) ) ;
#39416=ORIENTED_EDGE ( 'NONE', *, *, #10879, .T. ) ;
#39417=B_SPLINE_CURVE_WITH_KNOTS ( 'NONE', 3,
 ( #27193, #17223, #37495, #57801, #12222, #34128, #29169, #63406, #49465, #28187, #53120, #59412, #48475, #18857, #43797, #7911, #39123, #3596, #8540, #48156, #2614, #18209 ),
 .UNSPECIFIED., .F., .F.,
 ( 4, 2, 2, 2, 2, 2, 2, 2, 2, 2, 4 ),
 ( 0.000000000000000000, 0.001318687870781999920, 0.001978031806173001072, 0.002637375741564002007, 0.003956063612346002144, 0.004615407547737001778, 0.005274751483128001413, 0.006593439353909998080, 0.007912127224691993879, 0.009230815095473991413, 0.01054950296625598721 ),
 .UNSPECIFIED. ) ;
#39418=ORIENTED_EDGE ( 'NONE', *, *, #23067, .F. ) ;
#39419=FACE_OUTER_BOUND ( 'NONE', #43521, .T. ) ;
#39420=CARTESIAN_POINT ( 'NONE',  ( -35.00000000000000000, 6.547236723514155976, -9.752226076388824438 ) ) ;
#39427=CARTESIAN_POINT ( 'NONE',  ( -27.45775109278351067, 10.51123867646838583, -8.471355351200609007 ) ) ;
#39428=CARTESIAN_POINT ( 'NONE',  ( 7.266099666122742384, -5.675241298374717580, -12.25103963726659906 ) ) ;
#39429=CARTESIAN_POINT ( 'NONE',  ( 35.00000000000000000, 3.614449339633649227, 11.17622378668002092 ) ) ;
#39434=DIRECTION ( 'NONE',  ( 0.000000000000000000, 0.01356324068818000848, -0.9999080150203990547 ) ) ;
#39436=AXIS2_PLACEMENT_3D ( 'NONE', #16755, #26407, #30415 ) ;
#39441=ORIENTED_EDGE ( 'NONE', *, *, #41482, .T. ) ;
#39443=CARTESIAN_POINT ( 'NONE',  ( 6.361445718264521432, -4.355102044641763648, 11.18181944858514498 ) ) ;
#39446=ORIENTED_EDGE ( 'NONE', *, *, #30941, .F. ) ;
#39447=DIRECTION ( 'NONE',  ( -1.000000000000000000, 0.000000000000000000, 0.000000000000000000 ) ) ;
#39448=CARTESIAN_POINT ( 'NONE',  ( -28.19089594411849475, -12.81260937809825862, -4.263902777033699465 ) ) ;
#39449=CARTESIAN_POINT ( 'NONE',  ( 17.86634709757764838, -9.034895380895633821, 10.05927542744126946 ) ) ;
#39451=CARTESIAN_POINT ( 'NONE',  ( -21.23983773598477498, -7.447593303288433830, 25.00000000000000000 ) ) ;
#39452=CARTESIAN_POINT ( 'NONE',  ( -8.384530407289302545, -9.055240063205157952, -10.03793618941832655 ) ) ;
#39453=EDGE_CURVE ( 'NONE', #48767, #48483, #40720, .T. ) ;
#39457=VECTOR ( 'NONE', #58837, 1000.000000000000000 ) ;
#39462=CARTESIAN_POINT ( 'NONE',  ( -35.00000000000000000, -14.99999999999998757, 0.000000000000000000 ) ) ;
#39463=EDGE_CURVE ( 'NONE', #65264, #41230, #63916, .T. ) ;
#39465=CARTESIAN_POINT ( 'NONE',  ( -27.31188777422505609, -8.574970748528183861, -8.395320217058435119 ) ) ;
#39466=AXIS2_PLACEMENT_3D ( 'NONE', #17274, #6653, #1980 ) ;
#39467=EDGE_LOOP ( 'NONE', ( #29279, #26412, #58748, #2153 ) ) ;
#39468=ADVANCED_FACE ( 'NONE', ( #12892 ), #53802, .T. ) ;
#39471=ORIENTED_EDGE ( 'NONE', *, *, #13403, .F. ) ;
#39472=VECTOR ( 'NONE', #1854, 1000.000000000000000 ) ;
#39474=AXIS2_PLACEMENT_3D ( 'NONE', #5168, #60690, #18255 ) ;
#39481=CARTESIAN_POINT ( 'NONE',  ( 24.68094058364964027, 0.8458801819018304524, 13.47910264936496105 ) ) ;
#39483=ORIENTED_EDGE ( 'NONE', *, *, #29801, .T. ) ;
#39484=ORIENTED_EDGE ( 'NONE', *, *, #41490, .F. ) ;
#39486=CARTESIAN_POINT ( 'NONE',  ( -35.00000000000000000, -11.47758908105692655, -2.497432891016966749 ) ) ;
#39487=ORIENTED_EDGE ( 'NONE', *, *, #56007, .T. ) ;
#39488=CARTESIAN_POINT ( 'NONE',  ( 6.722269201495262081, -7.162924562234429970, -9.635873505962649688 ) ) ;
#39491=CARTESIAN_POINT ( 'NONE',  ( -19.47984447937493613, -3.750539801530005768, -11.39883551934754102 ) ) ;
#39492=FACE_OUTER_BOUND ( 'NONE', #14878, .T. ) ;
#39493=CARTESIAN_POINT ( 'NONE',  ( -7.181456785175555524, 8.540743096806467705, -10.45493698471458188 ) ) ;
#39494=DIRECTION ( 'NONE',  ( 1.000000000000000000, -0.000000000000000000, 0.000000000000000000 ) ) ;
#39495=VECTOR ( 'NONE', #55309, 1000.000000000000000 ) ;
#39496=EDGE_CURVE ( 'NONE', #62930, #52024, #28843, .T. ) ;
#39498=ORIENTED_EDGE ( 'NONE', *, *, #16135, .F. ) ;
#39500=CARTESIAN_POINT ( 'NONE',  ( -18.06060982367787204, 5.590226830146772130, 10.62101905373911315 ) ) ;
#39501=AXIS2_PLACEMENT_3D ( 'NONE', #51934, #46601, #47921 ) ;
#39502=EDGE_CURVE ( 'NONE', #14915, #5644, #62874, .T. ) ;
#39504=CARTESIAN_POINT ( 'NONE',  ( 37.00000000000000711, 11.59605747147793942, 5.300372733891518529 ) ) ;
#39506=CARTESIAN_POINT ( 'NONE',  ( 24.06471749115019776, -2.481826756221663821, 13.27386424782494601 ) ) ;
#39509=CARTESIAN_POINT ( 'NONE',  ( -35.00000000000000000, -11.54110654723650420, 2.185196060783841432 ) ) ;
#39512=CARTESIAN_POINT ( 'NONE',  ( 35.00000000000000000, -2.220215194441986561, -11.98254675519227597 ) ) ;
#39513=CIRCLE ( 'NONE', #54400, 5.000000000000000888 ) ;
#39514=EDGE_LOOP ( 'NONE', ( #351, #38513, #41967, #57395 ) ) ;
#39515=DIRECTION ( 'NONE',  ( 0.000000000000000000, -0.01356324068817991828, 0.9999080150203990547 ) ) ;
#39519=DIRECTION ( 'NONE',  ( 0.000000000000000000, -0.7790879021242442803, 0.6269146997508066033 ) ) ;
#39520=ORIENTED_EDGE ( 'NONE', *, *, #56934, .F. ) ;
#39523=VECTOR ( 'NONE', #22890, 1000.000000000000000 ) ;
#39524=DIRECTION ( 'NONE',  ( -1.000000000000000000, 0.000000000000000000, 0.000000000000000000 ) ) ;
#39525=FACE_OUTER_BOUND ( 'NONE', #22293, .T. ) ;
#39526=EDGE_CURVE ( 'NONE', #1051, #40174, #63744, .T. ) ;
#39527=VECTOR ( 'NONE', #9339, 1000.000000000000000 ) ;
#39529=EDGE_CURVE ( 'NONE', #1056, #3801, #38826, .T. ) ;
#39535=EDGE_CURVE ( 'NONE', #29592, #64891, #12042, .T. ) ;
#39537=AXIS2_PLACEMENT_3D ( 'NONE', #58137, #12553, #32832 ) ;
#39538=DIRECTION ( 'NONE',  ( 0.000000000000000000, 0.01356324068818000328, -0.9999080150203990547 ) ) ;
#39539=AXIS2_PLACEMENT_3D ( 'NONE', #10494, #63250, #30457 ) ;
#39541=VERTEX_POINT ( 'NONE', #30470 ) ;
#39543=CARTESIAN_POINT ( 'NONE',  ( -35.00000000000000000, -11.68758509253249223, 1.171570255487406786 ) ) ;
#39544=CARTESIAN_POINT ( 'NONE',  ( -36.00000000000000711, 11.90598845858533750, 4.561791185930457182 ) ) ;
#39549=AXIS2_PLACEMENT_3D ( 'NONE', #34883, #9974, #40550 ) ;
#39550=DIRECTION ( 'NONE',  ( 0.000000000000000000, 0.7381862504171974315, -0.6745969609292639113 ) ) ;
#39551=DIRECTION ( 'NONE',  ( -1.000000000000000000, 0.000000000000000000, 0.000000000000000000 ) ) ;
#39554=ORIENTED_EDGE ( 'NONE', *, *, #32185, .T. ) ;
#39555=ORIENTED_EDGE ( 'NONE', *, *, #44421, .T. ) ;
#39556=CARTESIAN_POINT ( 'NONE',  ( 35.00000000000000000, -6.564808257521689505, 10.93004082984025160 ) ) ;
#39558=VERTEX_POINT ( 'NONE', #19848 ) ;
#39559=DIRECTION ( 'NONE',  ( 0.000000000000000000, 0.01356324068817992175, -0.9999080150203990547 ) ) ;
#39560=FACE_BOUND ( 'NONE', #41708, .T. ) ;
#39561=ORIENTED_EDGE ( 'NONE', *, *, #42927, .T. ) ;
#39562=CARTESIAN_POINT ( 'NONE',  ( 37.00000000000000711, 4.561791185930414549, -11.90598845858535704 ) ) ;
#39563=CARTESIAN_POINT ( 'NONE',  ( 37.00000000000000711, -4.339012074899872395, 10.91536515067652324 ) ) ;
#39564=EDGE_CURVE ( 'NONE', #40351, #40103, #25483, .T. ) ;
#39565=CARTESIAN_POINT ( 'NONE',  ( 3.663040366865097486, -11.05188025280430786, 4.676643728192003913 ) ) ;
#39566=EDGE_LOOP ( 'NONE', ( #53127, #52852, #30563, #55948 ) ) ;
#39567=VERTEX_POINT ( 'NONE', #50452 ) ;
#39568=CARTESIAN_POINT ( 'NONE',  ( -35.00000000000000000, 0.000000000000000000, 0.000000000000000000 ) ) ;
#39569=EDGE_CURVE ( 'NONE', #17690, #24391, #386, .T. ) ;
#39570=ORIENTED_EDGE ( 'NONE', *, *, #46028, .T. ) ;
#39571=CARTESIAN_POINT ( 'NONE',  ( 10.66646312117316420, 7.972760762573107840, 10.89565866104123515 ) ) ;
#39572=ORIENTED_EDGE ( 'NONE', *, *, #42402, .T. ) ;
#39574=AXIS2_PLACEMENT_3D ( 'NONE', #30244, #50540, #65784 ) ;
#39575=VERTEX_POINT ( 'NONE', #56067 ) ;
#39576=VERTEX_POINT ( 'NONE', #49783 ) ;
#39577=EDGE_CURVE ( 'NONE', #1393, #20343, #51236, .T. ) ;
#39578=CARTESIAN_POINT ( 'NONE',  ( 37.00000000000000711, 4.705694406421931860E-17, -3.469127814946512892E-15 ) ) ;
#39581=VECTOR ( 'NONE', #13372, 1000.000000000000000 ) ;
#39582=DIRECTION ( 'NONE',  ( -1.000000000000000000, 0.000000000000000000, 0.000000000000000000 ) ) ;
#39583=CYLINDRICAL_SURFACE ( 'NONE', #537, 4.999999999999999112 ) ;
#39584=ORIENTED_EDGE ( 'NONE', *, *, #44146, .T. ) ;
#39585=ADVANCED_FACE ( 'NONE', ( #60401 ), #5216, .T. ) ;
#39588=DIRECTION ( 'NONE',  ( 0.000000000000000000, -0.01356324068818000328, 0.9999080150203990547 ) ) ;
#39589=CARTESIAN_POINT ( 'NONE',  ( -18.25006854224444908, -9.443202773001939221, -9.647586298549935435 ) ) ;
#39593=CIRCLE ( 'NONE', #32166, 12.18649999999999878 ) ;
#39597=CIRCLE ( 'NONE', #19432, 4.999999999999999112 ) ;
#39598=ORIENTED_EDGE ( 'NONE', *, *, #26930, .F. ) ;
#39602=CARTESIAN_POINT ( 'NONE',  ( -19.12534438730314434, -13.43125637399242756, -1.404165056817866297 ) ) ;
#39606=VERTEX_POINT ( 'NONE', #55087 ) ;
#39608=CARTESIAN_POINT ( 'NONE',  ( 35.00000000000000000, -2.696588552979144460, -12.46157735505188313 ) ) ;
#39611=DIRECTION ( 'NONE',  ( 0.000000000000000000, 0.01356324068817998940, -0.9999080150203990547 ) ) ;
#39612=( BOUNDED_CURVE ( )  B_SPLINE_CURVE ( 3, ( #8489, #64344, #18812, #13791 ),
 .UNSPECIFIED., .F., .F. ) 
 B_SPLINE_CURVE_WITH_KNOTS ( ( 4, 4 ),
 ( 2.655715767958479745, 2.751510998045912704 ),
 .UNSPECIFIED. ) 
 CURVE ( )  GEOMETRIC_REPRESENTATION_ITEM ( )  RATIONAL_B_SPLINE_CURVE ( ( 1.000000000000000000, 0.9992354190151078175, 0.9992354190151078175, 1.000000000000000000 ) ) 
 REPRESENTATION_ITEM ( '' )  );
#39613=DIRECTION ( 'NONE',  ( 1.000000000000000000, 0.000000000000000000, 0.000000000000000000 ) ) ;
#39615=DIRECTION ( 'NONE',  ( 0.000000000000000000, -0.01356324068817999114, 0.9999080150203989437 ) ) ;
#39616=FACE_OUTER_BOUND ( 'NONE', #39218, .T. ) ;
#39618=VECTOR ( 'NONE', #11829, 1000.000000000000000 ) ;
#39619=CIRCLE ( 'NONE', #10965, 12.18650000000000055 ) ;
#39620=AXIS2_PLACEMENT_3D ( 'NONE', #50203, #45511, #45198 ) ;
#39621=ORIENTED_EDGE ( 'NONE', *, *, #34488, .T. ) ;
#39622=CARTESIAN_POINT ( 'NONE',  ( -35.00000000000000000, 0.000000000000000000, 0.000000000000000000 ) ) ;
#39623=ORIENTED_EDGE ( 'NONE', *, *, #43704, .T. ) ;
#39625=DIRECTION ( 'NONE',  ( 0.000000000000000000, -0.5243256840888622650, -0.8515178078024832065 ) ) ;
#39627=CIRCLE ( 'NONE', #16292, 12.18650000000000055 ) ;
#39628=CARTESIAN_POINT ( 'NONE',  ( -37.00000000000000711, -6.946017217729864690, -10.01317267707894310 ) ) ;
#39629=ORIENTED_EDGE ( 'NONE', *, *, #55988, .F. ) ;
#39630=EDGE_CURVE ( 'NONE', #11130, #42300, #38844, .T. ) ;
#39631=AXIS2_PLACEMENT_3D ( 'NONE', #60457, #9925, #14881 ) ;
#39634=CARTESIAN_POINT ( 'NONE',  ( 29.73654696047771751, -7.541957041131760242, 9.346911106860231300 ) ) ;
#39636=AXIS2_PLACEMENT_3D ( 'NONE', #10930, #62129, #51834 ) ;
#39637=CARTESIAN_POINT ( 'NONE',  ( 36.00000000000000711, -4.074242145636093326, -12.08151691381188719 ) ) ;
#39638=EDGE_LOOP ( 'NONE', ( #37095, #2163, #42393, #34171 ) ) ;
#39639=DIRECTION ( 'NONE',  ( 0.000000000000000000, 0.01356324068817998940, -0.9999080150203990547 ) ) ;
#39640=CYLINDRICAL_SURFACE ( 'NONE', #63384, 4.999999999999999112 ) ;
#39642=CYLINDRICAL_SURFACE ( 'NONE', #34372, 12.18649999999999878 ) ;
#39643=ORIENTED_EDGE ( 'NONE', *, *, #32637, .F. ) ;
#39644=DIRECTION ( 'NONE',  ( 1.000000000000000000, 0.000000000000000000, 0.000000000000000000 ) ) ;
#39645=VECTOR ( 'NONE', #10972, 1000.000000000000000 ) ;
#39647=DIRECTION ( 'NONE',  ( 0.000000000000000000, 0.4935949184179200810, -0.8696919319575219243 ) ) ;
#39649=ORIENTED_EDGE ( 'NONE', *, *, #9714, .T. ) ;
#39650=CARTESIAN_POINT ( 'NONE',  ( -37.00000000000000711, -11.90598845858530730, -4.561791185930540671 ) ) ;
#39651=ORIENTED_EDGE ( 'NONE', *, *, #54912, .T. ) ;
#39652=DIRECTION ( 'NONE',  ( 0.000000000000000000, -0.01356324068817998940, 0.9999080150203990547 ) ) ;
#39653=ORIENTED_EDGE ( 'NONE', *, *, #25305, .T. ) ;
#39655=CARTESIAN_POINT ( 'NONE',  ( 12.61303456006366552, -11.71602035781408269, -2.601723401083803289 ) ) ;
#39656=EDGE_CURVE ( 'NONE', #8671, #4651, #240, .T. ) ;
#39657=CARTESIAN_POINT ( 'NONE',  ( 35.00000000000000000, 4.705694406421931860E-17, -3.469127814946512892E-15 ) ) ;
#39659=AXIS2_PLACEMENT_3D ( 'NONE', #45735, #10814, #15786 ) ;
#39663=DIRECTION ( 'NONE',  ( -1.000000000000000000, 0.000000000000000000, 0.000000000000000000 ) ) ;
#39667=CARTESIAN_POINT ( 'NONE',  ( 11.12460659294225351, -13.44996865318204904, -1.166173210671453742 ) ) ;
#39668=ORIENTED_EDGE ( 'NONE', *, *, #21216, .F. ) ;
#39669=EDGE_CURVE ( 'NONE', #44514, #58860, #24671, .T. ) ;
#39670=CIRCLE ( 'NONE', #58833, 4.999999999999999112 ) ;
#39671=ORIENTED_EDGE ( 'NONE', *, *, #553, .F. ) ;
#39676=CARTESIAN_POINT ( 'NONE',  ( -35.00000000000000000, 0.000000000000000000, 0.000000000000000000 ) ) ;
#39677=CARTESIAN_POINT ( 'NONE',  ( -35.00000000000000000, 4.339012074900111315, -10.91536515067643620 ) ) ;
#39678=VECTOR ( 'NONE', #55401, 1000.000000000000000 ) ;
#39680=EDGE_CURVE ( 'NONE', #29332, #11288, #36306, .T. ) ;
#39685=DIRECTION ( 'NONE',  ( 0.000000000000000000, 0.01356324068817999808, -0.9999080150203990547 ) ) ;
#39691=EDGE_CURVE ( 'NONE', #52755, #55501, #1669, .T. ) ;
#39693=CIRCLE ( 'NONE', #36516, 5.000000000000000888 ) ;
#39695=ORIENTED_EDGE ( 'NONE', *, *, #18915, .F. ) ;
#39696=DIRECTION ( 'NONE',  ( 1.000000000000000000, 0.000000000000000000, 0.000000000000000000 ) ) ;
#39698=FACE_OUTER_BOUND ( 'NONE', #49830, .T. ) ;
#39699=CARTESIAN_POINT ( 'NONE',  ( 37.00000000000000711, 4.705694406421931860E-17, -3.469127814946512892E-15 ) ) ;
#39701=ORIENTED_EDGE ( 'NONE', *, *, #14104, .T. ) ;
#39704=CARTESIAN_POINT ( 'NONE',  ( -18.31776534785701216, 3.837936424772297794, -11.37033739218235695 ) ) ;
#39706=CARTESIAN_POINT ( 'NONE',  ( 8.815713299111846979, 2.649613430600505914, 13.23998980317660035 ) ) ;
#39709=EDGE_CURVE ( 'NONE', #32907, #3342, #16166, .T. ) ;
#39710=EDGE_CURVE ( 'NONE', #64727, #8331, #60746, .T. ) ;
#39711=AXIS2_PLACEMENT_3D ( 'NONE', #46747, #41091, #61370 ) ;
#39712=AXIS2_PLACEMENT_3D ( 'NONE', #29200, #3934, #24198 ) ;
#39715=DIRECTION ( 'NONE',  ( 1.000000000000000000, -0.000000000000000000, -0.000000000000000000 ) ) ;
#39716=EDGE_CURVE ( 'NONE', #12670, #19302, #56539, .T. ) ;
#39718=VERTEX_POINT ( 'NONE', #31460 ) ;
#39720=DIRECTION ( 'NONE',  ( -1.000000000000000000, 0.000000000000000000, 0.000000000000000000 ) ) ;
#39721=DIRECTION ( 'NONE',  ( 0.000000000000000000, 0.01356324068817992175, -0.9999080150203990547 ) ) ;
#39722=CARTESIAN_POINT ( 'NONE',  ( -36.00000000000000711, -1.457575200925635528, 12.66641127287625501 ) ) ;
#39729=EDGE_LOOP ( 'NONE', ( #37104, #40330, #52468, #5227 ) ) ;
#39730=FACE_OUTER_BOUND ( 'NONE', #12824, .T. ) ;
#39732=VERTEX_POINT ( 'NONE', #21493 ) ;
#39733=VERTEX_POINT ( 'NONE', #56762 ) ;
#39734=DIRECTION ( 'NONE',  ( 0.000000000000000000, -0.9847383929261636082, 0.1740410799127514174 ) ) ;
#39736=ADVANCED_FACE ( 'NONE', ( #16507 ), #36776, .T. ) ;
#39737=AXIS2_PLACEMENT_3D ( 'NONE', #63119, #38838, #58140 ) ;
#39738=CARTESIAN_POINT ( 'NONE',  ( -47.00000000000000711, 0.000000000000000000, 0.000000000000000000 ) ) ;
#39740=CARTESIAN_POINT ( 'NONE',  ( -35.00000000000000000, 0.000000000000000000, 0.000000000000000000 ) ) ;
#39741=DIRECTION ( 'NONE',  ( -1.000000000000000000, 0.000000000000000000, 0.000000000000000000 ) ) ;
#39743=ORIENTED_EDGE ( 'NONE', *, *, #22590, .F. ) ;
#39744=CARTESIAN_POINT ( 'NONE',  ( -36.00000000000000711, -5.710938531231627202, -11.39945968423477751 ) ) ;
#39746=VECTOR ( 'NONE', #43634, 1000.000000000000000 ) ;
#39747=ORIENTED_EDGE ( 'NONE', *, *, #41222, .T. ) ;
#39750=DIRECTION ( 'NONE',  ( 0.000000000000000000, 0.01356324068817991828, -0.9999080150203990547 ) ) ;
#39753=CARTESIAN_POINT ( 'NONE',  ( -35.00000000000000000, -10.92721691015459307, 4.309077947445612899 ) ) ;
#39754=AXIS2_PLACEMENT_3D ( 'NONE', #29600, #44562, #14625 ) ;
#39755=CARTESIAN_POINT ( 'NONE',  ( 47.00000000000000711, 4.705694406421931860E-17, -3.469127814946512892E-15 ) ) ;
#39756=ORIENTED_EDGE ( 'NONE', *, *, #59260, .F. ) ;
#39761=DIRECTION ( 'NONE',  ( -1.000000000000000000, 0.000000000000000000, 0.000000000000000000 ) ) ;
#39763=DIRECTION ( 'NONE',  ( -1.000000000000000000, 0.000000000000000000, 0.000000000000000000 ) ) ;
#39766=CARTESIAN_POINT ( 'NONE',  ( 3.862716043132853105, -11.00608440648994346, -7.819365458621474474 ) ) ;
#39767=FACE_OUTER_BOUND ( 'NONE', #8398, .T. ) ;
#39770=CARTESIAN_POINT ( 'NONE',  ( -37.00000000000000711, 0.000000000000000000, 0.000000000000000000 ) ) ;
#39771=ORIENTED_EDGE ( 'NONE', *, *, #57163, .T. ) ;
#39776=VECTOR ( 'NONE', #46753, 1000.000000000000000 ) ;
#39777=ADVANCED_FACE ( 'NONE', ( #42386 ), #19702, .T. ) ;
#39779=CARTESIAN_POINT ( 'NONE',  ( -27.45775109278351067, -11.83395752356219255, -1.989333891161980894 ) ) ;
#39781=CARTESIAN_POINT ( 'NONE',  ( -37.00000000000000711, 0.000000000000000000, 0.000000000000000000 ) ) ;
#39785=FACE_OUTER_BOUND ( 'NONE', #14408, .T. ) ;
#39786=CARTESIAN_POINT ( 'NONE',  ( -27.69083675036838343, -10.87160676531835257, -8.024211436650034557 ) ) ;
#39788=ADVANCED_FACE ( 'NONE', ( #53722 ), #63661, .T. ) ;
#39790=CARTESIAN_POINT ( 'NONE',  ( 19.28625800530496903, 25.00000000000000000, 11.87904264843580471 ) ) ;
#39791=CARTESIAN_POINT ( 'NONE',  ( -14.11589373245165469, 8.250315036047107142, 8.713914264323175729 ) ) ;
#39792=CIRCLE ( 'NONE', #46175, 12.75000000000000178 ) ;
#39793=DIRECTION ( 'NONE',  ( 0.000000000000000000, -0.9999080150203992767, -0.01356324068816951341 ) ) ;
#39794=ORIENTED_EDGE ( 'NONE', *, *, #7215, .F. ) ;
#39797=( BOUNDED_CURVE ( )  B_SPLINE_CURVE ( 3, ( #57854, #62805, #36569, #11298 ),
 .UNSPECIFIED., .F., .F. ) 
 B_SPLINE_CURVE_WITH_KNOTS ( ( 4, 4 ),
 ( 5.154170548125383888, 5.159499013664793132 ),
 .UNSPECIFIED. ) 
 CURVE ( )  GEOMETRIC_REPRESENTATION_ITEM ( )  RATIONAL_B_SPLINE_CURVE ( ( 1.000000000000000000, 0.9999976339559824012, 0.9999976339559824012, 1.000000000000000000 ) ) 
 REPRESENTATION_ITEM ( '' )  );
#39798=DIRECTION ( 'NONE',  ( -1.000000000000000000, -1.836970198721029688E-16, -0.000000000000000000 ) ) ;
#39799=CARTESIAN_POINT ( 'NONE',  ( 35.00000000000000000, -2.627174906296994905, -11.44858830469739530 ) ) ;
#39800=CARTESIAN_POINT ( 'NONE',  ( -35.00000000000000000, 0.000000000000000000, 0.000000000000000000 ) ) ;
#39801=DIRECTION ( 'NONE',  ( -1.000000000000000000, -0.000000000000000000, 0.000000000000000000 ) ) ;
#39802=DIRECTION ( 'NONE',  ( 1.000000000000000000, 0.000000000000000000, 0.000000000000000000 ) ) ;
#39803=FACE_OUTER_BOUND ( 'NONE', #23607, .T. ) ;
#39804=ORIENTED_EDGE ( 'NONE', *, *, #51398, .F. ) ;
#39807=CARTESIAN_POINT ( 'NONE',  ( -18.50195596262152620, -5.100756500577913854, -10.86505773444920564 ) ) ;
#39810=DIRECTION ( 'NONE',  ( -1.000000000000000000, -0.000000000000000000, 0.000000000000000000 ) ) ;
#39811=CARTESIAN_POINT ( 'NONE',  ( -37.00000000000000711, 9.733281772932279807, -8.235637554476541666 ) ) ;
#39812=ORIENTED_EDGE ( 'NONE', *, *, #46604, .T. ) ;
#39813=FACE_OUTER_BOUND ( 'NONE', #29758, .T. ) ;
#39815=CARTESIAN_POINT ( 'NONE',  ( 23.96381627259500746, -3.708881761758332729, 12.98433744281732061 ) ) ;
#39816=ORIENTED_EDGE ( 'NONE', *, *, #17117, .F. ) ;
#39817=VERTEX_POINT ( 'NONE', #38409 ) ;
#39819=EDGE_CURVE ( 'NONE', #22363, #57005, #54408, .T. ) ;
#39820=ORIENTED_EDGE ( 'NONE', *, *, #23283, .F. ) ;
#39821=CARTESIAN_POINT ( 'NONE',  ( 6.810356414152409776, -6.143480531804472733, -10.31617154035105521 ) ) ;
#39822=ORIENTED_EDGE ( 'NONE', *, *, #22076, .F. ) ;
#39826=CARTESIAN_POINT ( 'NONE',  ( 35.00000000000000000, 6.280308599560279426, 9.926225166346956286 ) ) ;
#39827=DIRECTION ( 'NONE',  ( 0.000000000000000000, 0.01356324068817998940, -0.9999080150203990547 ) ) ;
#39828=CARTESIAN_POINT ( 'NONE',  ( 36.00000000000000711, -8.624332853795991127, 9.390600770288079602 ) ) ;
#39829=VERTEX_POINT ( 'NONE', #7485 ) ;
#39832=CARTESIAN_POINT ( 'NONE',  ( -35.00000000000000000, 11.95840593935201213, 2.346765782874477679 ) ) ;
#39833=DIRECTION ( 'NONE',  ( 0.000000000000000000, 0.01356324068817992175, -0.9999080150203990547 ) ) ;
#39834=CARTESIAN_POINT ( 'NONE',  ( 12.89950770217806664, 12.24699127810561627, -5.693691681728255460 ) ) ;
#39835=CARTESIAN_POINT ( 'NONE',  ( 24.40116933105910846, -0.3707949922271567278, 13.49969628832376856 ) ) ;
#39837=DIRECTION ( 'NONE',  ( 1.000000000000000000, -0.000000000000000000, -0.000000000000000000 ) ) ;
#39838=CARTESIAN_POINT ( 'NONE',  ( -30.18541646480307250, -1.416020129149132334, 25.00000000000000000 ) ) ;
#39839=CIRCLE ( 'NONE', #30264, 5.000000000000000888 ) ;
#39840=EDGE_CURVE ( 'NONE', #32947, #13249, #19781, .T. ) ;
#39841=EDGE_LOOP ( 'NONE', ( #12470, #53964, #57945, #8099 ) ) ;
#39842=CARTESIAN_POINT ( 'NONE',  ( -18.43828812910839687, 6.163775148567135709, -10.29989178887608503 ) ) ;
#39843=EDGE_CURVE ( 'NONE', #45163, #38116, #42684, .T. ) ;
#39844=ORIENTED_EDGE ( 'NONE', *, *, #28296, .F. ) ;
#39846=DIRECTION ( 'NONE',  ( 0.000000000000000000, 0.7196168960969767658, 0.6943713148249667233 ) ) ;
#39847=LINE ( 'NONE', #35165, #51590 ) ;
#39848=DIRECTION ( 'NONE',  ( 1.000000000000000000, 0.000000000000000000, -0.000000000000000000 ) ) ;
#39850=CARTESIAN_POINT ( 'NONE',  ( 35.00000000000000000, 10.49591321039688019, 5.273331777780226659 ) ) ;
#39851=ORIENTED_EDGE ( 'NONE', *, *, #2976, .F. ) ;
#39856=DIRECTION ( 'NONE',  ( 1.000000000000000000, -0.000000000000000000, 0.000000000000000000 ) ) ;
#39857=EDGE_CURVE ( 'NONE', #38941, #38782, #65006, .T. ) ;
#39858=DIRECTION ( 'NONE',  ( 0.000000000000000000, -0.01356324068817998940, 0.9999080150203990547 ) ) ;
#39859=AXIS2_PLACEMENT_3D ( 'NONE', #50905, #26285, #36244 ) ;
#39860=VERTEX_POINT ( 'NONE', #43385 ) ;
#39861=EDGE_CURVE ( 'NONE', #34161, #56661, #44601, .T. ) ;
#39862=DIRECTION ( 'NONE',  ( 0.000000000000000000, 0.8989688749565173387, 0.4380125133593943398 ) ) ;
#39863=ORIENTED_EDGE ( 'NONE', *, *, #17377, .F. ) ;
#39864=DIRECTION ( 'NONE',  ( 0.000000000000000000, -0.2960891610144577579, -0.9551603052523459647 ) ) ;
#39865=DIRECTION ( 'NONE',  ( 1.000000000000000000, 0.000000000000000000, 0.000000000000000000 ) ) ;
#39869=ORIENTED_EDGE ( 'NONE', *, *, #2595, .F. ) ;
#39872=EDGE_CURVE ( 'NONE', #49136, #19519, #24676, .T. ) ;
#39874=CARTESIAN_POINT ( 'NONE',  ( 35.00000000000000000, 6.303578524887091916, 10.42955799785312720 ) ) ;
#39876=DIRECTION ( 'NONE',  ( -0.000000000000000000, -1.000000000000000000, -0.000000000000000000 ) ) ;
#39877=DIRECTION ( 'NONE',  ( 0.000000000000000000, 0.01356324068817992175, -0.9999080150203990547 ) ) ;
#39879=DIRECTION ( 'NONE',  ( 0.000000000000000000, 0.9999080150203989437, 0.01356324068818338426 ) ) ;
#39881=ORIENTED_EDGE ( 'NONE', *, *, #23571, .T. ) ;
#39883=EDGE_LOOP ( 'NONE', ( #20877, #52656, #32928, #6797 ) ) ;
#39885=CARTESIAN_POINT ( 'NONE',  ( 36.00000000000000711, -9.076753354953932984, 8.954052073409695112 ) ) ;
#39886=AXIS2_PLACEMENT_3D ( 'NONE', #57443, #25878, #52470 ) ;
#39887=LINE ( 'NONE', #34564, #37432 ) ;
#39888=ORIENTED_EDGE ( 'NONE', *, *, #28396, .F. ) ;
#39889=DIRECTION ( 'NONE',  ( 0.000000000000000000, -1.000000000000000000, 0.000000000000000000 ) ) ;
#39890=ORIENTED_EDGE ( 'NONE', *, *, #4853, .T. ) ;
#39891=CARTESIAN_POINT ( 'NONE',  ( 36.00000000000000711, -12.74921544981110877, 0.1414404973753431438 ) ) ;
#39892=CARTESIAN_POINT ( 'NONE',  ( 35.00000000000000000, 5.636262487437473823, 10.80478261802175233 ) ) ;
#39894=VERTEX_POINT ( 'NONE', #30625 ) ;
#39897=ORIENTED_EDGE ( 'NONE', *, *, #25177, .T. ) ;
#39898=DIRECTION ( 'NONE',  ( 0.000000000000000000, 0.9937233664769765662, -0.1118654143051580896 ) ) ;
#39899=ORIENTED_EDGE ( 'NONE', *, *, #49877, .F. ) ;
#39900=ORIENTED_EDGE ( 'NONE', *, *, #43176, .F. ) ;
#39901=ORIENTED_EDGE ( 'NONE', *, *, #47893, .F. ) ;
#39902=DIRECTION ( 'NONE',  ( 1.000000000000000000, -0.000000000000000000, 0.000000000000000000 ) ) ;
#39903=LINE ( 'NONE', #29282, #65515 ) ;
#39904=EDGE_CURVE ( 'NONE', #28963, #62960, #45629, .T. ) ;
#39906=DIRECTION ( 'NONE',  ( 1.000000000000000000, 0.000000000000000000, 0.000000000000000000 ) ) ;
#39907=EDGE_LOOP ( 'NONE', ( #41299, #12150, #58909, #32493 ) ) ;
#39909=DIRECTION ( 'NONE',  ( -1.000000000000000000, 0.000000000000000000, 0.000000000000000000 ) ) ;
#39910=CIRCLE ( 'NONE', #13336, 12.18649999999999878 ) ;
#39911=ORIENTED_EDGE ( 'NONE', *, *, #8692, .T. ) ;
#39912=CARTESIAN_POINT ( 'NONE',  ( 35.00000000000000000, 4.705694406421931860E-17, -3.469127814946512892E-15 ) ) ;
#39913=DIRECTION ( 'NONE',  ( 0.000000000000000000, -0.01356324068817991828, 0.9999080150203990547 ) ) ;
#39914=VERTEX_POINT ( 'NONE', #55602 ) ;
#39915=CARTESIAN_POINT ( 'NONE',  ( -27.75615700819353293, 12.49246195788914093, -5.125355884365527359 ) ) ;
#39921=ORIENTED_EDGE ( 'NONE', *, *, #12857, .F. ) ;
#39923=ORIENTED_EDGE ( 'NONE', *, *, #9747, .F. ) ;
#39928=DIRECTION ( 'NONE',  ( -1.000000000000000000, 0.000000000000000000, -0.000000000000000000 ) ) ;
#39931=ORIENTED_EDGE ( 'NONE', *, *, #30362, .F. ) ;
#39932=DIRECTION ( 'NONE',  ( 1.000000000000000000, 0.000000000000000000, 0.000000000000000000 ) ) ;
#39937=EDGE_CURVE ( 'NONE', #22527, #26195, #6659, .T. ) ;
#39941=DIRECTION ( 'NONE',  ( -1.000000000000000000, -0.000000000000000000, 0.000000000000000000 ) ) ;
#39942=DIRECTION ( 'NONE',  ( -1.000000000000000000, 0.000000000000000000, 0.000000000000000000 ) ) ;
#39943=ADVANCED_FACE ( 'NONE', ( #60565 ), #50613, .T. ) ;
#39944=B_SPLINE_CURVE_WITH_KNOTS ( 'NONE', 3,
 ( #52676, #1140, #37354, #57325, #1488, #16441, #62612, #21764, #42014, #42652, #62295, #52353, #7101, #6792, #22065, #42321, #57666, #18073, #23385, #34001, #23731, #18419 ),
 .UNSPECIFIED., .F., .F.,
 ( 4, 2, 2, 2, 2, 2, 2, 2, 2, 2, 4 ),
 ( 4.249187360970369464E-18, 0.001238599178509041483, 0.002477198357018077328, 0.003715797535527113390, 0.004954396714036149452, 0.005573696303290667266, 0.006192995892545185947, 0.006812295481799704629, 0.007431595071054223310, 0.008670194249563258071, 0.009908793428072295434 ),
 .UNSPECIFIED. ) ;
#39945=CIRCLE ( 'NONE', #46327, 5.000000000000000888 ) ;
#39946=EDGE_LOOP ( 'NONE', ( #42921, #6040, #23137, #40030 ) ) ;
#39947=CARTESIAN_POINT ( 'NONE',  ( 11.81877095885896267, -11.76046328181930889, -2.390220360951764711 ) ) ;
#39948=EDGE_CURVE ( 'NONE', #34038, #50294, #1342, .T. ) ;
#39951=CYLINDRICAL_SURFACE ( 'NONE', #35266, 4.999999999999999112 ) ;
#39953=CARTESIAN_POINT ( 'NONE',  ( -21.23983773598477498, -7.447593303288433830, 25.00000000000000000 ) ) ;
#39954=EDGE_CURVE ( 'NONE', #9287, #45349, #1046, .T. ) ;
#39956=ORIENTED_EDGE ( 'NONE', *, *, #60954, .F. ) ;
#39957=VERTEX_POINT ( 'NONE', #25653 ) ;
#39963=CARTESIAN_POINT ( 'NONE',  ( 37.00000000000000711, 0.2661492558803343900, -12.18359334611896827 ) ) ;
#39964=LINE ( 'NONE', #39303, #14190 ) ;
#39966=DIRECTION ( 'NONE',  ( 1.000000000000000000, 0.000000000000000000, 0.000000000000000000 ) ) ;
#39968=DIRECTION ( 'NONE',  ( 0.000000000000000000, 0.01356324068817992175, -0.9999080150203990547 ) ) ;
#39969=LINE ( 'NONE', #19714, #55354 ) ;
#39971=CARTESIAN_POINT ( 'NONE',  ( -35.00000000000000000, 0.3025107581132838175, -11.74226168163341377 ) ) ;
#39972=ORIENTED_EDGE ( 'NONE', *, *, #16527, .F. ) ;
#39974=EDGE_LOOP ( 'NONE', ( #62127, #17222, #45961, #32283 ) ) ;
#39977=DIRECTION ( 'NONE',  ( 1.000000000000000000, 0.000000000000000000, 0.000000000000000000 ) ) ;
#39978=LINE ( 'NONE', #5401, #30172 ) ;
#39983=DIRECTION ( 'NONE',  ( 0.000000000000000000, 0.9467777615094583599, 0.3218879778915939571 ) ) ;
#39984=DIRECTION ( 'NONE',  ( 1.000000000000000000, 0.000000000000000000, -0.000000000000000000 ) ) ;
#39985=CARTESIAN_POINT ( 'NONE',  ( -35.00000000000000000, 0.000000000000000000, 0.000000000000000000 ) ) ;
#39986=ORIENTED_EDGE ( 'NONE', *, *, #51600, .F. ) ;
#39989=CARTESIAN_POINT ( 'NONE',  ( 13.39780866403243564, -12.21976414386113241, -5.755504928417656707 ) ) ;
#39990=VERTEX_POINT ( 'NONE', #46590 ) ;
#39992=ORIENTED_EDGE ( 'NONE', *, *, #58012, .F. ) ;
#39993=EDGE_CURVE ( 'NONE', #42493, #14627, #2429, .T. ) ;
#39996=DIRECTION ( 'NONE',  ( 0.000000000000000000, 0.01356324068817992175, -0.9999080150203990547 ) ) ;
#39997=DIRECTION ( 'NONE',  ( -0.000000000000000000, -1.000000000000000000, -0.000000000000000000 ) ) ;
#39999=EDGE_CURVE ( 'NONE', #42172, #33099, #46279, .T. ) ;
#40001=DIRECTION ( 'NONE',  ( 0.000000000000000000, 0.01356324068817992175, -0.9999080150203990547 ) ) ;
#40003=ORIENTED_EDGE ( 'NONE', *, *, #42539, .T. ) ;
#40007=EDGE_CURVE ( 'NONE', #7090, #15788, #13042, .T. ) ;
#40008=ORIENTED_EDGE ( 'NONE', *, *, #10255, .F. ) ;
#40009=DIRECTION ( 'NONE',  ( 1.000000000000000000, 0.000000000000000000, -0.000000000000000000 ) ) ;
#40010=DIRECTION ( 'NONE',  ( -1.000000000000000000, -0.000000000000000000, 0.000000000000000000 ) ) ;
#40012=EDGE_LOOP ( 'NONE', ( #25757, #48495, #40727, #23314 ) ) ;
#40015=DIRECTION ( 'NONE',  ( 0.000000000000000000, 0.01356324068817998940, -0.9999080150203990547 ) ) ;
#40016=EDGE_CURVE ( 'NONE', #61800, #39558, #6052, .T. ) ;
#40018=CARTESIAN_POINT ( 'NONE',  ( -37.00000000000000711, -7.499679039484122178, 9.040300684349668714 ) ) ;
#40019=CARTESIAN_POINT ( 'NONE',  ( 35.00000000000000000, 7.376655759824880754, -9.700295462048687867 ) ) ;
#40021=AXIS2_PLACEMENT_3D ( 'NONE', #12747, #33698, #53001 ) ;
#40024=DIRECTION ( 'NONE',  ( 1.000000000000000000, 0.000000000000000000, 0.000000000000000000 ) ) ;
#40025=EDGE_LOOP ( 'NONE', ( #60922, #30838, #34935, #56814 ) ) ;
#40026=EDGE_CURVE ( 'NONE', #51803, #22718, #23643, .T. ) ;
#40027=CARTESIAN_POINT ( 'NONE',  ( 11.12897774696030417, 0.3461397579055390250, 13.49616809366566983 ) ) ;
#40028=DIRECTION ( 'NONE',  ( 1.000000000000000000, -0.000000000000000000, 0.000000000000000000 ) ) ;
#40029=ORIENTED_EDGE ( 'NONE', *, *, #19601, .F. ) ;
#40030=ORIENTED_EDGE ( 'NONE', *, *, #42456, .T. ) ;
#40031=AXIS2_PLACEMENT_3D ( 'NONE', #42177, #62464, #27896 ) ;
#40032=VERTEX_POINT ( 'NONE', #16982 ) ;
#40033=ORIENTED_EDGE ( 'NONE', *, *, #56308, .T. ) ;
#40034=CARTESIAN_POINT ( 'NONE',  ( -37.00000000000000711, 8.699265615722982403, 8.534258022646129760 ) ) ;
#40036=DIRECTION ( 'NONE',  ( -1.000000000000000000, 0.000000000000000000, -0.000000000000000000 ) ) ;
#40037=CARTESIAN_POINT ( 'NONE',  ( -10.95212338237647920, -9.902220863987562183, 9.175839033069923545 ) ) ;
#40039=CARTESIAN_POINT ( 'NONE',  ( 23.48125385833485268, 2.900065688388548057, -13.18851851003229925 ) ) ;
#40040=CARTESIAN_POINT ( 'NONE',  ( -29.43980975494970309, -3.641506875706030488, 25.00000000000000000 ) ) ;
#40042=DIRECTION ( 'NONE',  ( 0.000000000000000000, 0.01356324068817998940, -0.9999080150203990547 ) ) ;
#40043=ORIENTED_EDGE ( 'NONE', *, *, #46912, .T. ) ;
#40044=DIRECTION ( 'NONE',  ( 1.000000000000000000, 0.000000000000000000, 0.000000000000000000 ) ) ;
#40050=ADVANCED_FACE ( 'NONE', ( #57235 ), #2713, .T. ) ;
#40052=CARTESIAN_POINT ( 'NONE',  ( -37.00000000000000711, 0.01609748574461371262, -11.74614673114903951 ) ) ;
#40053=ORIENTED_EDGE ( 'NONE', *, *, #32866, .F. ) ;
#40055=ORIENTED_EDGE ( 'NONE', *, *, #58339, .F. ) ;
#40059=ADVANCED_FACE ( 'NONE', ( #21669 ), #11990, .T. ) ;
#40060=CARTESIAN_POINT ( 'NONE',  ( 35.00000000000000000, 7.718225330433935660, 9.430788938293964918 ) ) ;
#40062=CARTESIAN_POINT ( 'NONE',  ( 17.70424766539830941, -7.192594383037563155, 9.609139074359166699 ) ) ;
#40064=AXIS2_PLACEMENT_3D ( 'NONE', #43320, #3119, #13396 ) ;
#40069=ADVANCED_FACE ( 'NONE', ( #62205 ), #21975, .T. ) ;
#40070=DIRECTION ( 'NONE',  ( -1.000000000000000000, -0.000000000000000000, 0.000000000000000000 ) ) ;
#40071=EDGE_CURVE ( 'NONE', #37494, #35347, #196, .T. ) ;
#40072=LINE ( 'NONE', #189, #35045 ) ;
#40073=CIRCLE ( 'NONE', #12493, 5.000000000000000888 ) ;
#40074=DIRECTION ( 'NONE',  ( -1.000000000000000000, 0.000000000000000000, -0.000000000000000000 ) ) ;
#40075=ADVANCED_FACE ( 'NONE', ( #1710 ), #58556, .T. ) ;
#40076=CARTESIAN_POINT ( 'NONE',  ( 5.590291635455702846, -9.340929066271097980, 7.541605757018187361 ) ) ;
#40077=CARTESIAN_POINT ( 'NONE',  ( -35.00000000000000000, 0.000000000000000000, 0.000000000000000000 ) ) ;
#40078=AXIS2_PLACEMENT_3D ( 'NONE', #58386, #59696, #54717 ) ;
#40079=CARTESIAN_POINT ( 'NONE',  ( 5.741342436335442834, -9.898584468105083189, -9.185852332820985566 ) ) ;
#40080=CARTESIAN_POINT ( 'NONE',  ( -35.00000000000000000, -11.95840593935199792, -2.346765782874564277 ) ) ;
#40084=CARTESIAN_POINT ( 'NONE',  ( 35.00000000000000000, -5.644643009979139592, -10.30098186818248074 ) ) ;
#40086=EDGE_CURVE ( 'NONE', #18084, #4318, #6996, .T. ) ;
#40089=CARTESIAN_POINT ( 'NONE',  ( 35.00000000000000000, 4.705694406421931860E-17, -3.469127814946512892E-15 ) ) ;
#40094=ORIENTED_EDGE ( 'NONE', *, *, #24511, .F. ) ;
#40095=CARTESIAN_POINT ( 'NONE',  ( 35.00000000000000000, 1.456211999474505969, 11.65554240571055011 ) ) ;
#40096=DIRECTION ( 'NONE',  ( -1.000000000000000000, 0.000000000000000000, 0.000000000000000000 ) ) ;
#40097=DIRECTION ( 'NONE',  ( 0.000000000000000000, -0.9346839223284501008, 0.3554799084909072149 ) ) ;
#40098=LINE ( 'NONE', #39790, #22222 ) ;
#40099=ORIENTED_EDGE ( 'NONE', *, *, #22358, .T. ) ;
#40100=CARTESIAN_POINT ( 'NONE',  ( -35.00000000000000000, 8.146229107149400406, 9.063649021438985542 ) ) ;
#40103=VERTEX_POINT ( 'NONE', #57569 ) ;
#40104=CARTESIAN_POINT ( 'NONE',  ( 6.361445718264521432, -4.355102044641763648, 25.00000000000000000 ) ) ;
#40107=CARTESIAN_POINT ( 'NONE',  ( -14.65039111264524863, 8.403879406532434260, -10.56534429714927370 ) ) ;
#40110=CARTESIAN_POINT ( 'NONE',  ( -30.18541646480307250, -0.9627431840302674848, -11.97002451358074815 ) ) ;
#40111=CYLINDRICAL_SURFACE ( 'NONE', #50994, 12.18650000000000055 ) ;
#40112=AXIS2_PLACEMENT_3D ( 'NONE', #17760, #31713, #56703 ) ;
#40116=VERTEX_POINT ( 'NONE', #52257 ) ;
#40117=CIRCLE ( 'NONE', #10408, 12.18650000000000233 ) ;
#40120=CARTESIAN_POINT ( 'NONE',  ( 47.00000000000000711, 4.705694406421931860E-17, -3.469127814946512892E-15 ) ) ;
#40121=ORIENTED_EDGE ( 'NONE', *, *, #25308, .T. ) ;
#40122=CARTESIAN_POINT ( 'NONE',  ( 17.27839441901508621, -10.52068335315807524, 5.771933972472480967 ) ) ;
#40123=EDGE_CURVE ( 'NONE', #23816, #38680, #62522, .T. ) ;
#40124=LINE ( 'NONE', #54797, #4034 ) ;
#40125=DIRECTION ( 'NONE',  ( 1.000000000000000000, 0.000000000000000000, 0.000000000000000000 ) ) ;
#40126=ORIENTED_EDGE ( 'NONE', *, *, #12755, .F. ) ;
#40127=ORIENTED_EDGE ( 'NONE', *, *, #55847, .T. ) ;
#40128=DIRECTION ( 'NONE',  ( 1.000000000000000000, 0.000000000000000000, -0.000000000000000000 ) ) ;
#40129=ORIENTED_EDGE ( 'NONE', *, *, #30941, .T. ) ;
#40131=VERTEX_POINT ( 'NONE', #47271 ) ;
#40133=DIRECTION ( 'NONE',  ( -1.000000000000000000, 0.000000000000000000, 0.000000000000000000 ) ) ;
#40135=EDGE_CURVE ( 'NONE', #5900, #61338, #52888, .T. ) ;
#40137=CARTESIAN_POINT ( 'NONE',  ( 37.00000000000000711, 4.705694406421931860E-17, -3.469127814946512892E-15 ) ) ;
#40138=ORIENTED_EDGE ( 'NONE', *, *, #41045, .T. ) ;
#40140=CARTESIAN_POINT ( 'NONE',  ( -37.00000000000000711, 0.000000000000000000, 0.000000000000000000 ) ) ;
#40142=CARTESIAN_POINT ( 'NONE',  ( -27.27855387000350262, 12.26939275170278343, 5.631341004100471892 ) ) ;
#40144=CARTESIAN_POINT ( 'NONE',  ( 22.85977700535744006, -4.208561018118428088, 12.82933600296545684 ) ) ;
#40146=DIRECTION ( 'NONE',  ( 0.000000000000000000, 0.4698238015817302604, 0.8827602140260348840 ) ) ;
#40147=CARTESIAN_POINT ( 'NONE',  ( -4.590058209962335489, 6.612760447609789871, 25.00000000000000000 ) ) ;
#40151=VERTEX_POINT ( 'NONE', #3697 ) ;
#40152=CARTESIAN_POINT ( 'NONE',  ( -15.52346636470029040, 8.464258284448757053, -8.506501996115177988 ) ) ;
#40153=AXIS2_PLACEMENT_3D ( 'NONE', #12290, #6674, #26945 ) ;
#40154=CIRCLE ( 'NONE', #3031, 5.000000000000000888 ) ;
#40155=ORIENTED_EDGE ( 'NONE', *, *, #4180, .F. ) ;
#40158=CARTESIAN_POINT ( 'NONE',  ( -18.08686583997275221, 5.151216734910927464, -12.47858029384662970 ) ) ;
#40159=CIRCLE ( 'NONE', #59318, 12.18650000000000055 ) ;
#40162=VERTEX_POINT ( 'NONE', #23627 ) ;
#40163=FACE_OUTER_BOUND ( 'NONE', #34678, .T. ) ;
#40165=CARTESIAN_POINT ( 'NONE',  ( 8.937200413559443390, 4.246084004433933856, 11.22641390959094565 ) ) ;
#40166=VECTOR ( 'NONE', #20202, 1000.000000000000000 ) ;
#40168=EDGE_CURVE ( 'NONE', #57837, #52191, #39887, .T. ) ;
#40169=CARTESIAN_POINT ( 'NONE',  ( -17.57573412780800126, -9.333560918461788702, 7.571049167956692472 ) ) ;
#40173=FACE_OUTER_BOUND ( 'NONE', #57940, .T. ) ;
#40174=VERTEX_POINT ( 'NONE', #43899 ) ;
#40178=DIRECTION ( 'NONE',  ( 1.000000000000000000, -0.000000000000000000, 0.000000000000000000 ) ) ;
#40179=EDGE_CURVE ( 'NONE', #48583, #65768, #53402, .T. ) ;
#40181=VERTEX_POINT ( 'NONE', #53884 ) ;
#40182=ORIENTED_EDGE ( 'NONE', *, *, #35510, .F. ) ;
#40183=ORIENTED_EDGE ( 'NONE', *, *, #18904, .F. ) ;
#40184=CARTESIAN_POINT ( 'NONE',  ( 35.00000000000000000, 10.64792938439763859, 5.927257550915197015 ) ) ;
#40186=CARTESIAN_POINT ( 'NONE',  ( 8.937200413559443390, 4.476360154859203355, 25.00000000000000000 ) ) ;
#40188=CIRCLE ( 'NONE', #26433, 5.000000000000000000 ) ;
#40190=CARTESIAN_POINT ( 'NONE',  ( 35.00000000000000000, -11.54110654723647400, 2.185196060784003524 ) ) ;
#40191=CYLINDRICAL_SURFACE ( 'NONE', #54127, 5.000000000000000888 ) ;
#40195=ORIENTED_EDGE ( 'NONE', *, *, #442, .F. ) ;
#40197=CIRCLE ( 'NONE', #65674, 4.999999999999999112 ) ;
#40198=CYLINDRICAL_SURFACE ( 'NONE', #34257, 5.000000000000001776 ) ;
#40199=VERTEX_POINT ( 'NONE', #18317 ) ;
#40200=FACE_BOUND ( 'NONE', #22153, .T. ) ;
#40202=EDGE_LOOP ( 'NONE', ( #62079, #13932, #10239, #11995 ) ) ;
#40203=CIRCLE ( 'NONE', #24167, 5.000000000000001776 ) ;
#40204=DIRECTION ( 'NONE',  ( 0.000000000000000000, 0.01356324068817998940, -0.9999080150203990547 ) ) ;
#40208=CARTESIAN_POINT ( 'NONE',  ( 3.848792418524904502, -10.99609134338280825, 4.807220403714089763 ) ) ;
#40209=VERTEX_POINT ( 'NONE', #54861 ) ;
#40211=AXIS2_PLACEMENT_3D ( 'NONE', #21936, #61496, #51563 ) ;
#40214=EDGE_LOOP ( 'NONE', ( #39021, #38049, #48723, #48118 ) ) ;
#40215=LINE ( 'NONE', #29921, #20976 ) ;
#40217=EDGE_LOOP ( 'NONE', ( #58652, #62622, #64085, #20414 ) ) ;
#40218=CIRCLE ( 'NONE', #26454, 12.75000000000000178 ) ;
#40219=EDGE_LOOP ( 'NONE', ( #41746, #18050, #1573, #17130 ) ) ;
#40224=EDGE_CURVE ( 'NONE', #60956, #52121, #14080, .T. ) ;
#40226=ORIENTED_EDGE ( 'NONE', *, *, #24942, .T. ) ;
#40227=CARTESIAN_POINT ( 'NONE',  ( 35.00000000000000000, 4.426194442447407340, 11.35427606708800852 ) ) ;
#40228=VERTEX_POINT ( 'NONE', #55179 ) ;
#40229=DIRECTION ( 'NONE',  ( 1.000000000000000000, -0.000000000000000000, 0.000000000000000000 ) ) ;
#40230=CARTESIAN_POINT ( 'NONE',  ( -18.21154635310088565, -5.491257917030544888, -12.33504523915716966 ) ) ;
#40231=EDGE_CURVE ( 'NONE', #27273, #47988, #57632, .T. ) ;
#40232=ORIENTED_EDGE ( 'NONE', *, *, #31540, .F. ) ;
#40234=CARTESIAN_POINT ( 'NONE',  ( 26.08439714455133185, 11.40113243194252846, 3.743551691817327942 ) ) ;
#40236=AXIS2_PLACEMENT_3D ( 'NONE', #25530, #40493, #34829 ) ;
#40237=EDGE_LOOP ( 'NONE', ( #61543, #58069, #5839, #4881 ) ) ;
#40239=EDGE_CURVE ( 'NONE', #9384, #36860, #65153, .T. ) ;
#40240=AXIS2_PLACEMENT_3D ( 'NONE', #25773, #20119, #61656 ) ;
#40241=VERTEX_POINT ( 'NONE', #18656 ) ;
#40242=CARTESIAN_POINT ( 'NONE',  ( -25.54417658651491863, -7.498517398407823720, 11.22596262356930197 ) ) ;
#40245=DIRECTION ( 'NONE',  ( 1.000000000000000000, 0.000000000000000000, -0.000000000000000000 ) ) ;
#40246=CARTESIAN_POINT ( 'NONE',  ( 12.19101310789403136, 11.82374128125938739, -2.055631940355953091 ) ) ;
#40247=ORIENTED_EDGE ( 'NONE', *, *, #21650, .T. ) ;
#40248=DIRECTION ( 'NONE',  ( 1.000000000000000000, 0.000000000000000000, 0.000000000000000000 ) ) ;
#40249=DIRECTION ( 'NONE',  ( -1.000000000000000000, 0.000000000000000000, 0.000000000000000000 ) ) ;
#40251=DIRECTION ( 'NONE',  ( 0.000000000000000000, 0.9937233664769756780, -0.1118654143051653060 ) ) ;
#40253=AXIS2_PLACEMENT_3D ( 'NONE', #11483, #5548, #25152 ) ;
#40254=VECTOR ( 'NONE', #16881, 1000.000000000000000 ) ;
#40258=CARTESIAN_POINT ( 'NONE',  ( -7.181456785175555524, -5.890186129966251904, -10.45493698471458188 ) ) ;
#40261=ORIENTED_EDGE ( 'NONE', *, *, #40778, .T. ) ;
#40263=ORIENTED_EDGE ( 'NONE', *, *, #28309, .T. ) ;
#40264=DIRECTION ( 'NONE',  ( 0.000000000000000000, -0.01356324068817998940, 0.9999080150203990547 ) ) ;
#40266=FACE_OUTER_BOUND ( 'NONE', #39202, .T. ) ;
#40269=VERTEX_POINT ( 'NONE', #38914 ) ;
#40270=ORIENTED_EDGE ( 'NONE', *, *, #10709, .F. ) ;
#40271=LINE ( 'NONE', #55600, #46119 ) ;
#40273=ADVANCED_FACE ( 'NONE', ( #8322 ), #48902, .T. ) ;
#40274=EDGE_LOOP ( 'NONE', ( #11786, #15751, #60845, #49259 ) ) ;
#40277=LINE ( 'NONE', #54637, #4986 ) ;
#40278=DIRECTION ( 'NONE',  ( 0.000000000000000000, -0.01356324068817998940, 0.9999080150203990547 ) ) ;
#40279=VERTEX_POINT ( 'NONE', #8653 ) ;
#40281=AXIS2_PLACEMENT_3D ( 'NONE', #61576, #4442, #4782 ) ;
#40282=EDGE_CURVE ( 'NONE', #58319, #3877, #51270, .T. ) ;
#40284=DIRECTION ( 'NONE',  ( -1.000000000000000000, -1.836970198721029688E-16, 0.000000000000000000 ) ) ;
#40287=DIRECTION ( 'NONE',  ( 1.000000000000000000, 0.000000000000000000, 0.000000000000000000 ) ) ;
#40288=ADVANCED_FACE ( 'NONE', ( #59518 ), #34869, .T. ) ;
#40289=ORIENTED_EDGE ( 'NONE', *, *, #41972, .F. ) ;
#40291=ORIENTED_EDGE ( 'NONE', *, *, #525, .F. ) ;
#40292=CARTESIAN_POINT ( 'NONE',  ( -27.01437459610461644, -8.723448335974111956, -8.240233560378637634 ) ) ;
#40293=CARTESIAN_POINT ( 'NONE',  ( 12.93934141822999528, -9.509120055689606943, -7.322759090511362423 ) ) ;
#40295=DIRECTION ( 'NONE',  ( -1.000000000000000000, 0.000000000000000000, 0.000000000000000000 ) ) ;
#40299=CARTESIAN_POINT ( 'NONE',  ( 12.47628546223243617, 0.000000000000000000, 11.99999999999999645 ) ) ;
#40302=DIRECTION ( 'NONE',  ( -1.000000000000000000, 0.000000000000000000, 0.000000000000000000 ) ) ;
#40303=CARTESIAN_POINT ( 'NONE',  ( 4.225017978203527313, -10.87119238259119314, 8.008815562465079196 ) ) ;
#40304=VERTEX_POINT ( 'NONE', #4984 ) ;
#40306=ORIENTED_EDGE ( 'NONE', *, *, #4712, .T. ) ;
#40307=CARTESIAN_POINT ( 'NONE',  ( 9.687175622948608122, -13.48729812737142986, -0.5854820436212360146 ) ) ;
#40308=ORIENTED_EDGE ( 'NONE', *, *, #8534, .T. ) ;
#40309=ADVANCED_FACE ( 'NONE', ( #35212 ), #40198, .T. ) ;
#40310=EDGE_LOOP ( 'NONE', ( #22741, #9946, #10249, #17049 ) ) ;
#40316=CARTESIAN_POINT ( 'NONE',  ( 35.00000000000000000, 4.705694406421931860E-17, -3.469127814946512892E-15 ) ) ;
#40318=DIRECTION ( 'NONE',  ( 0.000000000000000000, -0.01356324068817999114, 0.9999080150203989437 ) ) ;
#40323=LINE ( 'NONE', #4793, #56869 ) ;
#40325=ORIENTED_EDGE ( 'NONE', *, *, #40392, .F. ) ;
#40326=CIRCLE ( 'NONE', #47797, 12.75000000000000178 ) ;
#40327=AXIS2_PLACEMENT_3D ( 'NONE', #11946, #47863, #28237 ) ;
#40329=DIRECTION ( 'NONE',  ( 1.000000000000000000, 0.000000000000000000, 0.000000000000000000 ) ) ;
#40330=ORIENTED_EDGE ( 'NONE', *, *, #32319, .T. ) ;
#40331=LINE ( 'NONE', #15405, #6478 ) ;
#40333=CYLINDRICAL_SURFACE ( 'NONE', #7791, 12.18649999999999878 ) ;
#40334=AXIS2_PLACEMENT_3D ( 'NONE', #28510, #48818, #6940 ) ;
#40335=EDGE_CURVE ( 'NONE', #32047, #54583, #62920, .T. ) ;
#40336=EDGE_CURVE ( 'NONE', #54640, #44205, #10907, .T. ) ;
#40338=CARTESIAN_POINT ( 'NONE',  ( -37.00000000000000711, 0.000000000000000000, 0.000000000000000000 ) ) ;
#40339=CIRCLE ( 'NONE', #48875, 5.000000000000000000 ) ;
#40343=DIRECTION ( 'NONE',  ( -1.000000000000000000, 0.000000000000000000, 0.000000000000000000 ) ) ;
#40345=CARTESIAN_POINT ( 'NONE',  ( -37.00000000000000711, 2.968224442958403486, 11.81949347079748058 ) ) ;
#40346=FACE_OUTER_BOUND ( 'NONE', #10002, .T. ) ;
#40348=ADVANCED_FACE ( 'NONE', ( #324 ), #20602, .T. ) ;
#40351=VERTEX_POINT ( 'NONE', #61157 ) ;
#40352=ADVANCED_FACE ( 'NONE', ( #10942 ), #15588, .T. ) ;
#40353=VERTEX_POINT ( 'NONE', #25920 ) ;
#40354=CARTESIAN_POINT ( 'NONE',  ( 37.00000000000000711, 4.705694406421931860E-17, -3.469127814946512892E-15 ) ) ;
#40356=CARTESIAN_POINT ( 'NONE',  ( 35.00000000000000000, 5.672855678558685888, -10.28547182238010116 ) ) ;
#40359=CARTESIAN_POINT ( 'NONE',  ( -18.04208054618453616, 11.95114819866064693, 1.265206980359397271 ) ) ;
#40361=EDGE_LOOP ( 'NONE', ( #61364, #19459, #57030, #55629 ) ) ;
#40362=DIRECTION ( 'NONE',  ( 0.6147887355352468219, -0.7886918350401329603, 0.000000000000000000 ) ) ;
#40363=EDGE_CURVE ( 'NONE', #10842, #43145, #17434, .T. ) ;
#40365=CARTESIAN_POINT ( 'NONE',  ( 35.00000000000000000, 4.705694406421931860E-17, -3.469127814946512892E-15 ) ) ;
#40366=ORIENTED_EDGE ( 'NONE', *, *, #19104, .F. ) ;
#40368=CARTESIAN_POINT ( 'NONE',  ( 35.00000000000000000, -1.591260454995155671, 12.08216339958901742 ) ) ;
#40370=DIRECTION ( 'NONE',  ( -1.000000000000000000, 0.000000000000000000, -0.000000000000000000 ) ) ;
#40373=VECTOR ( 'NONE', #24092, 1000.000000000000000 ) ;
#40376=ORIENTED_EDGE ( 'NONE', *, *, #29067, .F. ) ;
#40377=( BOUNDED_CURVE ( )  B_SPLINE_CURVE ( 3, ( #26489, #12181, #42414, #62709 ),
 .UNSPECIFIED., .F., .F. ) 
 B_SPLINE_CURVE_WITH_KNOTS ( ( 4, 4 ),
 ( 4.670929601778163409, 4.712388980384690562 ),
 .UNSPECIFIED. ) 
 CURVE ( )  GEOMETRIC_REPRESENTATION_ITEM ( )  RATIONAL_B_SPLINE_CURVE ( ( 1.000000000000000000, 0.9998567651231480280, 0.9998567651231480280, 1.000000000000000000 ) ) 
 REPRESENTATION_ITEM ( '' )  );
#40378=ORIENTED_EDGE ( 'NONE', *, *, #13054, .T. ) ;
#40379=CARTESIAN_POINT ( 'NONE',  ( -35.00000000000000000, 3.827046518385245122, -11.56998259273173701 ) ) ;
#40380=ORIENTED_EDGE ( 'NONE', *, *, #39112, .T. ) ;
#40381=EDGE_CURVE ( 'NONE', #55675, #9403, #50274, .T. ) ;
#40382=EDGE_CURVE ( 'NONE', #12941, #49613, #40666, .T. ) ;
#40383=VERTEX_POINT ( 'NONE', #21911 ) ;
#40384=DIRECTION ( 'NONE',  ( 1.000000000000000000, 0.000000000000000000, 0.000000000000000000 ) ) ;
#40392=EDGE_CURVE ( 'NONE', #55347, #55842, #21589, .T. ) ;
#40393=CARTESIAN_POINT ( 'NONE',  ( 27.72497957433742855, -12.75711206765212324, 4.419907683352735539 ) ) ;
#40395=ORIENTED_EDGE ( 'NONE', *, *, #7551, .F. ) ;
#40396=ORIENTED_EDGE ( 'NONE', *, *, #16723, .T. ) ;
#40398=DIRECTION ( 'NONE',  ( 0.000000000000000000, -0.01356324068817998940, 0.9999080150203990547 ) ) ;
#40400=VECTOR ( 'NONE', #61725, 1000.000000000000000 ) ;
#40401=DIRECTION ( 'NONE',  ( 0.000000000000000000, -0.01356324068817992175, 0.9999080150203990547 ) ) ;
#40402=CARTESIAN_POINT ( 'NONE',  ( 6.716177905018834160, -7.149925761153411941, 9.639490146783378677 ) ) ;
#40403=FACE_OUTER_BOUND ( 'NONE', #39060, .T. ) ;
#40405=FACE_OUTER_BOUND ( 'NONE', #2895, .T. ) ;
#40409=EDGE_LOOP ( 'NONE', ( #8975, #55803 ) ) ;
#40411=CARTESIAN_POINT ( 'NONE',  ( -14.11589373245165469, 8.250315036047107142, 8.713914264323175729 ) ) ;
#40412=DIRECTION ( 'NONE',  ( 0.000000000000000000, -1.000000000000000000, 0.000000000000000000 ) ) ;
#40413=AXIS2_PLACEMENT_3D ( 'NONE', #30046, #60307, #5120 ) ;
#40414=ADVANCED_FACE ( 'NONE', ( #37180 ), #42482, .T. ) ;
#40415=CIRCLE ( 'NONE', #25576, 5.000000000000000888 ) ;
#40416=CARTESIAN_POINT ( 'NONE',  ( 37.00000000000000711, 4.705694406421931860E-17, -3.469127814946512892E-15 ) ) ;
#40417=ADVANCED_FACE ( 'NONE', ( #32836 ), #62781, .T. ) ;
#40424=ORIENTED_EDGE ( 'NONE', *, *, #8120, .F. ) ;
#40428=ADVANCED_FACE ( 'NONE', ( #48185 ), #32510, .F. ) ;
#40430=ORIENTED_EDGE ( 'NONE', *, *, #11214, .T. ) ;
#40433=CIRCLE ( 'NONE', #52141, 12.74999999999999822 ) ;
#40435=ORIENTED_EDGE ( 'NONE', *, *, #11464, .F. ) ;
#40436=AXIS2_PLACEMENT_3D ( 'NONE', #41062, #52628, #7368 ) ;
#40437=CARTESIAN_POINT ( 'NONE',  ( 0.09505933169494876211, -0.1369491540312630928, -11.99999999999999112 ) ) ;
#40439=DIRECTION ( 'NONE',  ( 0.000000000000000000, 0.01356324068817991828, -0.9999080150203990547 ) ) ;
#40440=CARTESIAN_POINT ( 'NONE',  ( -17.98378524109403287, 7.072918058914841488, -11.50120456127047142 ) ) ;
#40441=LINE ( 'NONE', #14825, #63762 ) ;
#40443=CIRCLE ( 'NONE', #34082, 12.18649999999999700 ) ;
#40445=DIRECTION ( 'NONE',  ( 0.000000000000000000, 0.000000000000000000, -1.000000000000000000 ) ) ;
#40446=EDGE_CURVE ( 'NONE', #41793, #13375, #43152, .T. ) ;
#40447=VERTEX_POINT ( 'NONE', #22568 ) ;
#40448=DIRECTION ( 'NONE',  ( 0.000000000000000000, -0.8827602140260367714, 0.4698238015817268742 ) ) ;
#40451=EDGE_CURVE ( 'NONE', #52651, #34584, #38161, .T. ) ;
#40452=DIRECTION ( 'NONE',  ( 0.000000000000000000, -0.01356324068817999114, 0.9999080150203989437 ) ) ;
#40453=FACE_OUTER_BOUND ( 'NONE', #1388, .T. ) ;
#40454=ORIENTED_EDGE ( 'NONE', *, *, #5789, .F. ) ;
#40455=AXIS2_PLACEMENT_3D ( 'NONE', #57918, #26991, #42574 ) ;
#40457=CARTESIAN_POINT ( 'NONE',  ( 35.00000000000000000, 11.72397916322012179, -0.7214809346829029746 ) ) ;
#40460=ORIENTED_EDGE ( 'NONE', *, *, #25701, .T. ) ;
#40463=ORIENTED_EDGE ( 'NONE', *, *, #31827, .T. ) ;
#40464=DIRECTION ( 'NONE',  ( 1.000000000000000000, -0.000000000000000000, -0.000000000000000000 ) ) ;
#40466=CARTESIAN_POINT ( 'NONE',  ( 37.00000000000000711, 11.65554240571056788, -1.456211999474385843 ) ) ;
#40469=AXIS2_PLACEMENT_3D ( 'NONE', #25725, #4474, #14730 ) ;
#40471=CARTESIAN_POINT ( 'NONE',  ( -35.00000000000000000, 11.61175578952786047, 1.771820996347196697 ) ) ;
#40478=DIRECTION ( 'NONE',  ( -0.000000000000000000, -0.000000000000000000, -1.000000000000000000 ) ) ;
#40479=CARTESIAN_POINT ( 'NONE',  ( -37.00000000000000711, 2.544412758416015219, -11.91791701451263741 ) ) ;
#40480=CARTESIAN_POINT ( 'NONE',  ( 9.963898962030125261, 13.44886489065879331, -1.176091836301444760 ) ) ;
#40481=CARTESIAN_POINT ( 'NONE',  ( -19.69476066079020171, -4.201994156881551312, 12.82938989607585789 ) ) ;
#40483=LINE ( 'NONE', #23918, #6872 ) ;
#40485=CARTESIAN_POINT ( 'NONE',  ( -11.40165637462999904, -7.508992741355383416, 25.00000000000000000 ) ) ;
#40486=AXIS2_PLACEMENT_3D ( 'NONE', #40052, #19128, #9145 ) ;
#40488=VERTEX_POINT ( 'NONE', #43822 ) ;
#40489=DIRECTION ( 'NONE',  ( 0.000000000000000000, 0.01356324068817991828, -0.9999080150203990547 ) ) ;
#40490=EDGE_CURVE ( 'NONE', #8767, #44513, #65070, .T. ) ;
#40491=CIRCLE ( 'NONE', #15051, 5.000000000000000888 ) ;
#40493=DIRECTION ( 'NONE',  ( -1.000000000000000000, 0.000000000000000000, 0.000000000000000000 ) ) ;
#40495=DIRECTION ( 'NONE',  ( 0.000000000000000000, -0.01356324068817998940, 0.9999080150203990547 ) ) ;
#40499=B_SPLINE_CURVE_WITH_KNOTS ( 'NONE', 3,
 ( #37994, #31685, #11416, #26720, #51997, #27687, #11106, #6777, #21749, #1470, #32348, #6440, #47995, #56990, #47013, #51682, #16733, #61970, #36692, #41679, #57309, #37006, #27051, #31380, #12069, #17404 ),
 .UNSPECIFIED., .F., .F.,
 ( 4, 2, 2, 2, 2, 2, 2, 2, 2, 2, 2, 2, 4 ),
 ( 7.806255641895631925E-18, 0.001111772592860239871, 0.002223545185720471936, 0.003335317778580703784, 0.004447090371440936066, 0.005002976667871053724, 0.005558862964301172251, 0.006114749260731289909, 0.006670635557161407568, 0.007226521853591526094, 0.007782408150021643753, 0.008338294446451760544, 0.008894180742881879070 ),
 .UNSPECIFIED. ) ;
#40502=CIRCLE ( 'NONE', #20387, 5.000000000000001776 ) ;
#40506=CARTESIAN_POINT ( 'NONE',  ( -37.00000000000000711, -5.814360711498210321, -10.70999494708499000 ) ) ;
#40510=ORIENTED_EDGE ( 'NONE', *, *, #26860, .F. ) ;
#40511=AXIS2_PLACEMENT_3D ( 'NONE', #9595, #10586, #19922 ) ;
#40514=DIRECTION ( 'NONE',  ( 0.000000000000000000, 0.01356324068817998940, -0.9999080150203989437 ) ) ;
#40515=CARTESIAN_POINT ( 'NONE',  ( -35.00000000000000000, -4.339012074900030491, 10.91536515067646818 ) ) ;
#40516=AXIS2_PLACEMENT_3D ( 'NONE', #5550, #26144, #25474 ) ;
#40517=VECTOR ( 'NONE', #25681, 1000.000000000000000 ) ;
#40518=VECTOR ( 'NONE', #34383, 1000.000000000000000 ) ;
#40520=ORIENTED_EDGE ( 'NONE', *, *, #30588, .T. ) ;
#40521=CARTESIAN_POINT ( 'NONE',  ( -30.04163406560897442, 0.3900926402758986278, 12.00202977223371192 ) ) ;
#40522=ORIENTED_EDGE ( 'NONE', *, *, #6237, .F. ) ;
#40523=CARTESIAN_POINT ( 'NONE',  ( 35.00000000000000000, 4.705694406421931860E-17, -3.469127814946512892E-15 ) ) ;
#40525=CARTESIAN_POINT ( 'NONE',  ( 37.00000000000000711, -3.473736367725341889, -12.26766708251990501 ) ) ;
#40531=EDGE_CURVE ( 'NONE', #36171, #56420, #23212, .T. ) ;
#40533=ORIENTED_EDGE ( 'NONE', *, *, #16035, .T. ) ;
#40536=EDGE_CURVE ( 'NONE', #54366, #43796, #42289, .T. ) ;
#40539=EDGE_LOOP ( 'NONE', ( #22996, #27190, #42120, #37845 ) ) ;
#40540=CIRCLE ( 'NONE', #10823, 5.000000000000000888 ) ;
#40541=DIRECTION ( 'NONE',  ( 0.000000000000000000, 0.9651210252299803338, 0.2618041379715598249 ) ) ;
#40542=ORIENTED_EDGE ( 'NONE', *, *, #45132, .T. ) ;
#40543=CARTESIAN_POINT ( 'NONE',  ( 26.34661844826604593, 11.53221627053869369, 3.317828791472333005 ) ) ;
#40544=CARTESIAN_POINT ( 'NONE',  ( 5.046549821695511362, -9.819109663588886150, -9.265868187600728945 ) ) ;
#40545=DIRECTION ( 'NONE',  ( 0.000000000000000000, 0.01356324068817992175, -0.9999080150203990547 ) ) ;
#40547=VERTEX_POINT ( 'NONE', #43474 ) ;
#40548=AXIS2_PLACEMENT_3D ( 'NONE', #19943, #14932, #56169 ) ;
#40549=ORIENTED_EDGE ( 'NONE', *, *, #32438, .F. ) ;
#40550=DIRECTION ( 'NONE',  ( 0.000000000000000000, -0.01356324068817998940, 0.9999080150203990547 ) ) ;
#40551=VERTEX_POINT ( 'NONE', #44786 ) ;
#40553=ORIENTED_EDGE ( 'NONE', *, *, #42067, .T. ) ;
#40555=VERTEX_POINT ( 'NONE', #64729 ) ;
#40556=VERTEX_POINT ( 'NONE', #34489 ) ;
#40557=CARTESIAN_POINT ( 'NONE',  ( -37.00000000000000711, 0.000000000000000000, 0.000000000000000000 ) ) ;
#40558=ADVANCED_FACE ( 'NONE', ( #38839 ), #63753, .F. ) ;
#40562=CARTESIAN_POINT ( 'NONE',  ( 35.00000000000000000, -7.474872387601069867, -9.060822531526026680 ) ) ;
#40563=ORIENTED_EDGE ( 'NONE', *, *, #62896, .T. ) ;
#40565=AXIS2_PLACEMENT_3D ( 'NONE', #15618, #31570, #65273 ) ;
#40567=CARTESIAN_POINT ( 'NONE',  ( -36.00000000000000711, 12.74613886779085448, -0.3137578094507843529 ) ) ;
#40571=LINE ( 'NONE', #46240, #27558 ) ;
#40576=CIRCLE ( 'NONE', #18291, 5.000000000000000888 ) ;
#40577=AXIS2_PLACEMENT_3D ( 'NONE', #59804, #61108, #64762 ) ;
#40578=VERTEX_POINT ( 'NONE', #4242 ) ;
#40579=DIRECTION ( 'NONE',  ( -1.000000000000000000, 0.000000000000000000, 0.000000000000000000 ) ) ;
#40581=ORIENTED_EDGE ( 'NONE', *, *, #65767, .T. ) ;
#40582=DIRECTION ( 'NONE',  ( 0.000000000000000000, -0.3554799084909036067, -0.9346839223284515441 ) ) ;
#40583=DIRECTION ( 'NONE',  ( 0.6442147435043042991, 0.000000000000000000, 0.7648446667472313942 ) ) ;
#40584=CARTESIAN_POINT ( 'NONE',  ( -35.00000000000000000, -6.950793414699719008, -10.68873102412850074 ) ) ;
#40586=DIRECTION ( 'NONE',  ( 1.000000000000000000, 0.000000000000000000, 0.000000000000000000 ) ) ;
#40587=ORIENTED_EDGE ( 'NONE', *, *, #23042, .T. ) ;
#40588=DIRECTION ( 'NONE',  ( -0.7886918350401376232, 0.6147887355352408267, 0.000000000000000000 ) ) ;
#40590=DIRECTION ( 'NONE',  ( -1.000000000000000000, 0.000000000000000000, 0.000000000000000000 ) ) ;
#40591=CARTESIAN_POINT ( 'NONE',  ( -47.00000000000000711, 0.000000000000000000, 0.000000000000000000 ) ) ;
#40592=AXIS2_PLACEMENT_3D ( 'NONE', #15339, #35613, #30310 ) ;
#40596=LINE ( 'NONE', #45581, #43381 ) ;
#40601=B_SPLINE_CURVE_WITH_KNOTS ( 'NONE', 3,
 ( #65044, #19176, #49769, #44763, #39448, #59749, #35097, #9847, #14178, #34468, #60075, #9189, #39786, #30139 ),
 .UNSPECIFIED., .F., .F.,
 ( 4, 2, 2, 2, 2, 2, 4 ),
 ( 0.000000000000000000, 0.001836665365673664872, 0.002754998048510496657, 0.003673330731347328876, 0.004591663414184160227, 0.005509996097020991579, 0.007346661462694656017 ),
 .UNSPECIFIED. ) ;
#40602=EDGE_CURVE ( 'NONE', #14759, #45661, #48142, .T. ) ;
#40603=ORIENTED_EDGE ( 'NONE', *, *, #65740, .F. ) ;
#40606=DIRECTION ( 'NONE',  ( 0.000000000000000000, 0.5243256840888503856, 0.8515178078024905339 ) ) ;
#40608=CARTESIAN_POINT ( 'NONE',  ( -37.00000000000000711, -5.865551165831157654, 11.32068061209293219 ) ) ;
#40610=ORIENTED_EDGE ( 'NONE', *, *, #38489, .F. ) ;
#40611=EDGE_CURVE ( 'NONE', #22391, #27971, #6693, .T. ) ;
#40612=VECTOR ( 'NONE', #7013, 1000.000000000000000 ) ;
#40613=ORIENTED_EDGE ( 'NONE', *, *, #28170, .F. ) ;
#40614=VERTEX_POINT ( 'NONE', #18885 ) ;
#40616=CIRCLE ( 'NONE', #46990, 5.000000000000000000 ) ;
#40617=CARTESIAN_POINT ( 'NONE',  ( 36.00000000000000711, 12.08151691381189963, -4.074242145636052470 ) ) ;
#40618=AXIS2_PLACEMENT_3D ( 'NONE', #20741, #61292, #16060 ) ;
#40619=ORIENTED_EDGE ( 'NONE', *, *, #24512, .F. ) ;
#40620=CARTESIAN_POINT ( 'NONE',  ( -35.00000000000000000, -10.30098186818253758, 5.644643009979033899 ) ) ;
#40622=DIRECTION ( 'NONE',  ( 1.000000000000000000, 0.000000000000000000, 0.000000000000000000 ) ) ;
#40626=DIRECTION ( 'NONE',  ( 1.000000000000000000, -0.000000000000000000, 0.000000000000000000 ) ) ;
#40628=CARTESIAN_POINT ( 'NONE',  ( 35.00000000000000000, -11.59605747147790211, -5.300372733891605570 ) ) ;
#40630=CARTESIAN_POINT ( 'NONE',  ( -47.00000000000000711, 0.000000000000000000, 0.000000000000000000 ) ) ;
#40631=VERTEX_POINT ( 'NONE', #59438 ) ;
#40633=CARTESIAN_POINT ( 'NONE',  ( 13.41123448928980366, -10.79486891117419134, -5.246219947578315335 ) ) ;
#40636=AXIS2_PLACEMENT_3D ( 'NONE', #36178, #27204, #41171 ) ;
#40637=DIRECTION ( 'NONE',  ( -0.000000000000000000, -1.000000000000000000, -0.000000000000000000 ) ) ;
#40640=DIRECTION ( 'NONE',  ( 0.000000000000000000, -0.01356324068818001369, 0.9999080150203990547 ) ) ;
#40642=CARTESIAN_POINT ( 'NONE',  ( 6.993057411323677641, -4.515497414218242689, 12.72858834154033758 ) ) ;
#40644=DIRECTION ( 'NONE',  ( -1.000000000000000000, 0.000000000000000000, 0.000000000000000000 ) ) ;
#40645=CIRCLE ( 'NONE', #14058, 5.000000000000000888 ) ;
#40647=DIRECTION ( 'NONE',  ( -0.000000000000000000, -1.000000000000000000, -0.000000000000000000 ) ) ;
#40650=DIRECTION ( 'NONE',  ( -1.000000000000000000, 0.000000000000000000, 0.000000000000000000 ) ) ;
#40655=CARTESIAN_POINT ( 'NONE',  ( -36.00000000000000711, -12.31350058095525846, 3.307597835713200762 ) ) ;
#40656=EDGE_CURVE ( 'NONE', #38263, #39189, #23692, .T. ) ;
#40657=CYLINDRICAL_SURFACE ( 'NONE', #7510, 12.18649999999999878 ) ;
#40659=DIRECTION ( 'NONE',  ( -1.000000000000000000, 0.000000000000000000, 0.000000000000000000 ) ) ;
#40660=EDGE_LOOP ( 'NONE', ( #43626, #60732, #7619, #50882 ) ) ;
#40663=CARTESIAN_POINT ( 'NONE',  ( -2.822269947909834986, 4.599275498345582136, 11.08601571419042031 ) ) ;
#40664=VERTEX_POINT ( 'NONE', #20178 ) ;
#40665=VECTOR ( 'NONE', #22280, 1000.000000000000000 ) ;
#40666=CIRCLE ( 'NONE', #339, 4.999999999999999112 ) ;
#40668=CIRCLE ( 'NONE', #2430, 12.75000000000000178 ) ;
#40669=EDGE_CURVE ( 'NONE', #61654, #21666, #2481, .T. ) ;
#40671=ADVANCED_FACE ( 'NONE', ( #24852 ), #19857, .T. ) ;
#40672=VECTOR ( 'NONE', #34988, 1000.000000000000000 ) ;
#40673=CARTESIAN_POINT ( 'NONE',  ( -35.00000000000000000, -12.26766708251994231, 3.473736367725209551 ) ) ;
#40676=ORIENTED_EDGE ( 'NONE', *, *, #28526, .F. ) ;
#40681=AXIS2_PLACEMENT_3D ( 'NONE', #33510, #22887, #53479 ) ;
#40684=CARTESIAN_POINT ( 'NONE',  ( -35.00000000000000000, 3.704519465651306742, 11.60979404548636218 ) ) ;
#40685=ORIENTED_EDGE ( 'NONE', *, *, #31160, .F. ) ;
#40686=DIRECTION ( 'NONE',  ( 0.000000000000000000, -0.01356324068817998940, 0.9999080150203990547 ) ) ;
#40689=CIRCLE ( 'NONE', #12019, 5.000000000000000000 ) ;
#40693=DIRECTION ( 'NONE',  ( -1.000000000000000000, 0.000000000000000000, 0.000000000000000000 ) ) ;
#40694=ORIENTED_EDGE ( 'NONE', *, *, #41164, .T. ) ;
#40696=ORIENTED_EDGE ( 'NONE', *, *, #32069, .T. ) ;
#40698=ORIENTED_EDGE ( 'NONE', *, *, #3875, .T. ) ;
#40700=CARTESIAN_POINT ( 'NONE',  ( 47.00000000000000711, 4.705694406421931860E-17, -3.469127814946512892E-15 ) ) ;
#40703=CARTESIAN_POINT ( 'NONE',  ( 6.511148368283224741, -4.283242813471564325, 11.20980722696366882 ) ) ;
#40706=CARTESIAN_POINT ( 'NONE',  ( 24.54370396021021605, 1.234610750962751080, -13.44821043565675467 ) ) ;
#40707=FACE_OUTER_BOUND ( 'NONE', #9326, .T. ) ;
#40708=ORIENTED_EDGE ( 'NONE', *, *, #6637, .T. ) ;
#40709=DIRECTION ( 'NONE',  ( -1.000000000000000000, -1.836970198721029688E-16, 0.000000000000000000 ) ) ;
#40710=VERTEX_POINT ( 'NONE', #35468 ) ;
#40712=CARTESIAN_POINT ( 'NONE',  ( 37.00000000000000711, 1.791059740004421919, -12.05416472667166339 ) ) ;
#40714=CIRCLE ( 'NONE', #16327, 12.74999999999999822 ) ;
#40718=AXIS2_PLACEMENT_3D ( 'NONE', #6755, #11084, #6106 ) ;
#40719=DIRECTION ( 'NONE',  ( 0.000000000000000000, -0.01356324068817999114, 0.9999080150203989437 ) ) ;
#40720=CIRCLE ( 'NONE', #57726, 5.000000000000000888 ) ;
#40722=DIRECTION ( 'NONE',  ( -1.000000000000000000, 0.000000000000000000, 0.000000000000000000 ) ) ;
#40724=ORIENTED_EDGE ( 'NONE', *, *, #11374, .F. ) ;
#40725=EDGE_LOOP ( 'NONE', ( #31903, #10947, #30669, #54385 ) ) ;
#40726=CARTESIAN_POINT ( 'NONE',  ( -35.00000000000000000, 0.000000000000000000, 0.000000000000000000 ) ) ;
#40727=ORIENTED_EDGE ( 'NONE', *, *, #25308, .F. ) ;
#40729=VERTEX_POINT ( 'NONE', #51113 ) ;
#40730=CIRCLE ( 'NONE', #57694, 12.18649999999999878 ) ;
#40731=CYLINDRICAL_SURFACE ( 'NONE', #20042, 12.18649999999999878 ) ;
#40745=DIRECTION ( 'NONE',  ( -1.000000000000000000, -0.000000000000000000, 0.000000000000000000 ) ) ;
#40746=CARTESIAN_POINT ( 'NONE',  ( 6.550563172034069126, -7.779754947801418297, 9.145170272292368452 ) ) ;
#40747=VECTOR ( 'NONE', #36937, 1000.000000000000000 ) ;
#40749=CARTESIAN_POINT ( 'NONE',  ( 3.426183256940671829, -10.95277051985667605, 4.917698437020844082 ) ) ;
#40753=CARTESIAN_POINT ( 'NONE',  ( 3.415098594035642421, 3.602609866107200354, -11.44847010818049604 ) ) ;
#40760=DIRECTION ( 'NONE',  ( 1.000000000000000000, 0.000000000000000000, 0.000000000000000000 ) ) ;
#40762=DIRECTION ( 'NONE',  ( 0.000000000000000000, 0.01356324068817998940, -0.9999080150203990547 ) ) ;
#40764=CIRCLE ( 'NONE', #49297, 12.18650000000000233 ) ;
#40765=CARTESIAN_POINT ( 'NONE',  ( 0.2851083653049504285, -0.4107471485392698018, 25.00000000000000000 ) ) ;
#40766=CARTESIAN_POINT ( 'NONE',  ( -37.00000000000000711, -12.08151691381193160, 4.074242145635959211 ) ) ;
#40767=CIRCLE ( 'NONE', #18490, 5.000000000000000888 ) ;
#40768=ORIENTED_EDGE ( 'NONE', *, *, #46011, .T. ) ;
#40772=CIRCLE ( 'NONE', #52471, 12.74999999999999822 ) ;
#40774=ORIENTED_EDGE ( 'NONE', *, *, #65343, .F. ) ;
#40778=EDGE_CURVE ( 'NONE', #48808, #19993, #31776, .T. ) ;
#40779=AXIS2_PLACEMENT_3D ( 'NONE', #11366, #1076, #30655 ) ;
#40780=CARTESIAN_POINT ( 'NONE',  ( -35.00000000000000000, -7.146664589317976102, 9.321877890560418933 ) ) ;
#40781=VERTEX_POINT ( 'NONE', #36461 ) ;
#40782=FACE_OUTER_BOUND ( 'NONE', #47814, .T. ) ;
#40783=ADVANCED_FACE ( 'NONE', ( #6537 ), #22144, .T. ) ;
#40785=EDGE_CURVE ( 'NONE', #60941, #51695, #50646, .T. ) ;
#40786=ORIENTED_EDGE ( 'NONE', *, *, #24683, .F. ) ;
#40788=CYLINDRICAL_SURFACE ( 'NONE', #11055, 12.75000000000000178 ) ;
#40789=CARTESIAN_POINT ( 'NONE',  ( -9.130651553988846203, 12.72949299159512115, -4.509469149381835962 ) ) ;
#40791=FACE_OUTER_BOUND ( 'NONE', #45898, .T. ) ;
#40795=CARTESIAN_POINT ( 'NONE',  ( -27.78468958554971380, 25.00000000000000000, 8.565911087387465983 ) ) ;
#40797=VERTEX_POINT ( 'NONE', #32113 ) ;
#40798=CARTESIAN_POINT ( 'NONE',  ( 35.00000000000000000, 8.352657516904789858, 8.258652103341336925 ) ) ;
#40799=VERTEX_POINT ( 'NONE', #22480 ) ;
#40800=DIRECTION ( 'NONE',  ( 0.000000000000000000, 0.01356324068818000328, -0.9999080150203990547 ) ) ;
#40802=VECTOR ( 'NONE', #3061, 1000.000000000000000 ) ;
#40805=DIRECTION ( 'NONE',  ( 1.000000000000000000, 0.000000000000000000, 0.000000000000000000 ) ) ;
#40808=EDGE_LOOP ( 'NONE', ( #50648, #22907, #8942, #19088 ) ) ;
#40809=ORIENTED_EDGE ( 'NONE', *, *, #34251, .F. ) ;
#40814=CARTESIAN_POINT ( 'NONE',  ( 35.00000000000000000, 4.705694406421931860E-17, -3.469127814946512892E-15 ) ) ;
#40821=VERTEX_POINT ( 'NONE', #57401 ) ;
#40823=CARTESIAN_POINT ( 'NONE',  ( 22.64108410429532370, 10.50347544506924891, -5.812766615855110786 ) ) ;
#40826=AXIS2_PLACEMENT_3D ( 'NONE', #55643, #29682, #40001 ) ;
#40827=CARTESIAN_POINT ( 'NONE',  ( -19.55186598411636467, -3.901828651817480953, 12.92480312515320229 ) ) ;
#40828=DIRECTION ( 'NONE',  ( 1.000000000000000000, 0.000000000000000000, 0.000000000000000000 ) ) ;
#40829=DIRECTION ( 'NONE',  ( -0.000000000000000000, -0.000000000000000000, -1.000000000000000000 ) ) ;
#40830=EDGE_CURVE ( 'NONE', #35611, #51290, #2202, .T. ) ;
#40831=CYLINDRICAL_SURFACE ( 'NONE', #52280, 12.18649999999999878 ) ;
#40832=AXIS2_PLACEMENT_3D ( 'NONE', #14507, #9518, #64403 ) ;
#40833=AXIS2_PLACEMENT_3D ( 'NONE', #15620, #35891, #46548 ) ;
#40835=DIRECTION ( 'NONE',  ( 1.000000000000000000, 0.000000000000000000, 0.000000000000000000 ) ) ;
#40836=VERTEX_POINT ( 'NONE', #62694 ) ;
#40837=CARTESIAN_POINT ( 'NONE',  ( -2.747351760715558200, -5.743695276321967746, 10.56617162187726322 ) ) ;
#40838=CARTESIAN_POINT ( 'NONE',  ( -35.00000000000000000, -5.814360711498210321, -10.70999494708499000 ) ) ;
#40839=AXIS2_PLACEMENT_3D ( 'NONE', #26742, #16099, #32040 ) ;
#40842=CYLINDRICAL_SURFACE ( 'NONE', #48805, 12.18649999999999878 ) ;
#40843=EDGE_CURVE ( 'NONE', #29123, #22816, #10934, .T. ) ;
#40847=DIRECTION ( 'NONE',  ( 1.000000000000000000, 0.000000000000000000, 0.000000000000000000 ) ) ;
#40851=CARTESIAN_POINT ( 'NONE',  ( -17.39032955383490275, -6.043477806738668079, 10.36841493105847611 ) ) ;
#40853=VERTEX_POINT ( 'NONE', #3538 ) ;
#40857=FACE_OUTER_BOUND ( 'NONE', #3966, .T. ) ;
#40858=DIRECTION ( 'NONE',  ( -1.000000000000000000, 0.000000000000000000, 0.000000000000000000 ) ) ;
#40859=CYLINDRICAL_SURFACE ( 'NONE', #16071, 4.999999999999999112 ) ;
#40860=EDGE_CURVE ( 'NONE', #34948, #5010, #62973, .T. ) ;
#40862=EDGE_LOOP ( 'NONE', ( #4483, #30147, #9762, #19879 ) ) ;
#40864=EDGE_CURVE ( 'NONE', #5514, #44, #5666, .T. ) ;
#40866=CARTESIAN_POINT ( 'NONE',  ( -35.00000000000000000, -7.376655759824951808, 9.700295462048636352 ) ) ;
#40870=LINE ( 'NONE', #51189, #49199 ) ;
#40871=EDGE_CURVE ( 'NONE', #2584, #64575, #15741, .T. ) ;
#40876=CIRCLE ( 'NONE', #12193, 4.999999999999999112 ) ;
#40877=CARTESIAN_POINT ( 'NONE',  ( -9.289599981290024289, -10.79669820059283758, -5.251390403865245027 ) ) ;
#40878=EDGE_LOOP ( 'NONE', ( #48390, #53818, #64968, #3334 ) ) ;
#40880=AXIS2_PLACEMENT_3D ( 'NONE', #16741, #48002, #7093 ) ;
#40881=DIRECTION ( 'NONE',  ( 0.000000000000000000, -0.01356324068817991828, 0.9999080150203990547 ) ) ;
#40882=ORIENTED_EDGE ( 'NONE', *, *, #17117, .T. ) ;
#40886=CARTESIAN_POINT ( 'NONE',  ( 4.915077328917121235, -9.915524164001334739, -9.162427078388006407 ) ) ;
#40887=CARTESIAN_POINT ( 'NONE',  ( -36.00000000000000711, 0.9416912585474430664, 12.71517666308948513 ) ) ;
#40889=EDGE_LOOP ( 'NONE', ( #64043, #22674, #20721, #36989 ) ) ;
#40890=ORIENTED_EDGE ( 'NONE', *, *, #29562, .T. ) ;
#40894=ORIENTED_EDGE ( 'NONE', *, *, #6684, .T. ) ;
#40895=ORIENTED_EDGE ( 'NONE', *, *, #47258, .T. ) ;
#40896=ORIENTED_EDGE ( 'NONE', *, *, #45180, .T. ) ;
#40897=DIRECTION ( 'NONE',  ( 0.000000000000000000, 0.9847383929261624980, -0.1740410799127578012 ) ) ;
#40898=DIRECTION ( 'NONE',  ( 0.000000000000000000, 0.6478160128811947249, -0.7617968321374877227 ) ) ;
#40900=EDGE_CURVE ( 'NONE', #6695, #18713, #13467, .T. ) ;
#40903=EDGE_LOOP ( 'NONE', ( #4476, #47133, #11316, #18429 ) ) ;
#40904=CARTESIAN_POINT ( 'NONE',  ( -35.00000000000000000, 10.30098186818257666, -5.644643009978957515 ) ) ;
#40906=ORIENTED_EDGE ( 'NONE', *, *, #9030, .F. ) ;
#40907=DIRECTION ( 'NONE',  ( -1.000000000000000000, 0.000000000000000000, 0.000000000000000000 ) ) ;
#40908=DIRECTION ( 'NONE',  ( -1.000000000000000000, -0.000000000000000000, 0.000000000000000000 ) ) ;
#40909=DIRECTION ( 'NONE',  ( 1.000000000000000000, -0.000000000000000000, 0.000000000000000000 ) ) ;
#40910=CARTESIAN_POINT ( 'NONE',  ( -18.49080574448724690, -13.49999999999999822, -2.827202046691532642E-15 ) ) ;
#40911=CARTESIAN_POINT ( 'NONE',  ( 37.00000000000000711, 10.64792938439763859, 5.927257550915197015 ) ) ;
#40914=ADVANCED_FACE ( 'NONE', ( #28129 ), #34420, .T. ) ;
#40917=VERTEX_POINT ( 'NONE', #8828 ) ;
#40918=CARTESIAN_POINT ( 'NONE',  ( 35.00000000000000000, -11.72195762423410414, -0.7536123767498126291 ) ) ;
#40923=ADVANCED_FACE ( 'NONE', ( #2876 ), #43739, .T. ) ;
#40924=EDGE_CURVE ( 'NONE', #11428, #16086, #54053, .T. ) ;
#40925=ORIENTED_EDGE ( 'NONE', *, *, #59979, .F. ) ;
#40926=DIRECTION ( 'NONE',  ( -1.000000000000000000, 0.000000000000000000, 0.000000000000000000 ) ) ;
#40927=DIRECTION ( 'NONE',  ( 1.000000000000000000, 0.000000000000000000, 0.000000000000000000 ) ) ;
#40935=CARTESIAN_POINT ( 'NONE',  ( 35.00000000000000000, 4.705694406421931860E-17, -3.469127814946512892E-15 ) ) ;
#40936=ADVANCED_FACE ( 'NONE', ( #55356 ), #30078, .T. ) ;
#40938=EDGE_LOOP ( 'NONE', ( #46370, #29453, #42050, #61142 ) ) ;
#40940=ORIENTED_EDGE ( 'NONE', *, *, #11683, .F. ) ;
#40942=DIRECTION ( 'NONE',  ( 0.000000000000000000, 0.01356324068817999114, -0.9999080150203990547 ) ) ;
#40943=CARTESIAN_POINT ( 'NONE',  ( -35.00000000000000000, 11.13736569743281457, -4.946702696913053643 ) ) ;
#40946=ORIENTED_EDGE ( 'NONE', *, *, #41792, .F. ) ;
#40948=CARTESIAN_POINT ( 'NONE',  ( 29.66301245255163366, -8.641839016897280956, 8.340436526386785232 ) ) ;
#40949=CARTESIAN_POINT ( 'NONE',  ( -21.17861794710831091, -11.44571409049744481, -3.604945070120774808 ) ) ;
#40951=DIRECTION ( 'NONE',  ( 1.000000000000000000, 0.000000000000000000, -0.000000000000000000 ) ) ;
#40952=CARTESIAN_POINT ( 'NONE',  ( 37.00000000000000711, 11.66664283989686979, 5.143145423404151373 ) ) ;
#40954=AXIS2_PLACEMENT_3D ( 'NONE', #6910, #12861, #53107 ) ;
#40955=CARTESIAN_POINT ( 'NONE',  ( -37.00000000000000711, 8.258652103341553641, -8.352657516904583801 ) ) ;
#40957=FACE_OUTER_BOUND ( 'NONE', #44911, .T. ) ;
#40958=ORIENTED_EDGE ( 'NONE', *, *, #46028, .F. ) ;
#40960=ORIENTED_EDGE ( 'NONE', *, *, #16703, .F. ) ;
#40965=DIRECTION ( 'NONE',  ( -1.000000000000000000, 0.000000000000000000, 0.000000000000000000 ) ) ;
#40967=DIRECTION ( 'NONE',  ( 0.000000000000000000, -0.2355298848897378061, -0.9718671068226493182 ) ) ;
#40968=DIRECTION ( 'NONE',  ( -1.000000000000000000, -0.000000000000000000, 0.000000000000000000 ) ) ;
#40972=CARTESIAN_POINT ( 'NONE',  ( 6.601852703653428911, -8.834089529978390587, 10.21601470017478341 ) ) ;
#40975=EDGE_CURVE ( 'NONE', #37151, #29673, #26909, .T. ) ;
#40977=ORIENTED_EDGE ( 'NONE', *, *, #9075, .T. ) ;
#40978=CARTESIAN_POINT ( 'NONE',  ( 12.37382948190224141, -10.69513828756983287, -8.245931121816388654 ) ) ;
#40979=ORIENTED_EDGE ( 'NONE', *, *, #47258, .F. ) ;
#40981=VERTEX_POINT ( 'NONE', #46051 ) ;
#40982=CARTESIAN_POINT ( 'NONE',  ( -35.00000000000000000, 2.865935305911801123, -12.42372387097879383 ) ) ;
#40984=CARTESIAN_POINT ( 'NONE',  ( 35.00000000000000000, -8.927548052240835474, 8.295159312811946961 ) ) ;
#40986=CARTESIAN_POINT ( 'NONE',  ( 36.00000000000000711, 10.93004082984027825, 6.564808257521646873 ) ) ;
#40987=ADVANCED_FACE ( 'NONE', ( #30723 ), #36035, .T. ) ;
#40988=ORIENTED_EDGE ( 'NONE', *, *, #21806, .F. ) ;
#40989=DIRECTION ( 'NONE',  ( 0.000000000000000000, 0.01356324068817992522, -0.9999080150203990547 ) ) ;
#40992=CYLINDRICAL_SURFACE ( 'NONE', #12211, 5.000000000000000888 ) ;
#40993=CARTESIAN_POINT ( 'NONE',  ( -18.39456087108311522, -4.498649229773558744, 12.72900479644374094 ) ) ;
#40994=VERTEX_POINT ( 'NONE', #25104 ) ;
#40996=VECTOR ( 'NONE', #45663, 1000.000000000000000 ) ;
#40997=CARTESIAN_POINT ( 'NONE',  ( 36.00000000000000711, -10.02106554660714011, -7.882940143791743459 ) ) ;
#40998=CARTESIAN_POINT ( 'NONE',  ( -36.00000000000000711, -11.59605747147783106, -5.300372733891766330 ) ) ;
#40999=CARTESIAN_POINT ( 'NONE',  ( 37.00000000000000711, -11.05394794832825767, 5.130401251914841865 ) ) ;
#41001=EDGE_LOOP ( 'NONE', ( #7583, #8897, #60983, #11680 ) ) ;
#41002=CARTESIAN_POINT ( 'NONE',  ( -35.00000000000000000, 0.000000000000000000, 0.000000000000000000 ) ) ;
#41006=CARTESIAN_POINT ( 'NONE',  ( -35.00000000000000000, -4.074242145635921908, -12.08151691381194404 ) ) ;
#41007=CARTESIAN_POINT ( 'NONE',  ( 17.94443053578330094, -10.27027613361345004, 8.791042504289096726 ) ) ;
#41012=EDGE_LOOP ( 'NONE', ( #8021, #63519, #42922, #2622 ) ) ;
#41015=ORIENTED_EDGE ( 'NONE', *, *, #44334, .T. ) ;
#41016=ORIENTED_EDGE ( 'NONE', *, *, #701, .T. ) ;
#41017=ORIENTED_EDGE ( 'NONE', *, *, #40135, .T. ) ;
#41019=ORIENTED_EDGE ( 'NONE', *, *, #62711, .F. ) ;
#41020=CARTESIAN_POINT ( 'NONE',  ( 37.00000000000000711, 11.13736569743274352, -4.946702696913214403 ) ) ;
#41021=CARTESIAN_POINT ( 'NONE',  ( 35.00000000000000000, 3.614449339633649227, 11.17622378668002092 ) ) ;
#41022=LINE ( 'NONE', #61304, #46071 ) ;
#41026=DIRECTION ( 'NONE',  ( 0.000000000000000000, 0.01356324068817998940, -0.9999080150203990547 ) ) ;
#41027=CARTESIAN_POINT ( 'NONE',  ( -37.00000000000000711, 0.000000000000000000, 0.000000000000000000 ) ) ;
#41028=ORIENTED_EDGE ( 'NONE', *, *, #35035, .T. ) ;
#41029=CARTESIAN_POINT ( 'NONE',  ( -35.00000000000000000, 7.379373053629018742, -10.39746860227882586 ) ) ;
#41032=EDGE_LOOP ( 'NONE', ( #15547, #7571, #8195, #19622 ) ) ;
#41033=ORIENTED_EDGE ( 'NONE', *, *, #10570, .T. ) ;
#41034=AXIS2_PLACEMENT_3D ( 'NONE', #59956, #44973, #34648 ) ;
#41037=DIRECTION ( 'NONE',  ( -0.000000000000000000, -1.000000000000000000, -0.000000000000000000 ) ) ;
#41042=ORIENTED_EDGE ( 'NONE', *, *, #63405, .T. ) ;
#41043=ADVANCED_FACE ( 'NONE', ( #19467 ), #35043, .T. ) ;
#41045=EDGE_CURVE ( 'NONE', #65334, #50289, #22695, .T. ) ;
#41047=ORIENTED_EDGE ( 'NONE', *, *, #1449, .T. ) ;
#41048=EDGE_CURVE ( 'NONE', #18977, #6781, #64062, .T. ) ;
#41049=EDGE_LOOP ( 'NONE', ( #59213, #37332, #16578, #5988 ) ) ;
#41055=CARTESIAN_POINT ( 'NONE',  ( -7.184946476706033813, -1.341365231991552998, -11.92630736377528500 ) ) ;
#41056=ADVANCED_FACE ( 'NONE', ( #45372 ), #20767, .T. ) ;
#41057=CARTESIAN_POINT ( 'NONE',  ( 35.00000000000000000, 4.705694406421931860E-17, -3.469127814946512892E-15 ) ) ;
#41059=VERTEX_POINT ( 'NONE', #25760 ) ;
#41060=CARTESIAN_POINT ( 'NONE',  ( 37.00000000000000711, -9.557269938331499404, 7.561043153948067364 ) ) ;
#41062=CARTESIAN_POINT ( 'NONE',  ( -35.00000000000000000, 0.000000000000000000, 0.000000000000000000 ) ) ;
#41063=CARTESIAN_POINT ( 'NONE',  ( 6.802398627868447178, -6.309174925604525086, 10.20958905146123286 ) ) ;
#41064=EDGE_CURVE ( 'NONE', #37494, #42367, #35710, .T. ) ;
#41065=CYLINDRICAL_SURFACE ( 'NONE', #16073, 5.000000000000000888 ) ;
#41068=CARTESIAN_POINT ( 'NONE',  ( 8.929416320216105873, 2.411192301257917059, -11.75776610390553323 ) ) ;
#41069=EDGE_LOOP ( 'NONE', ( #40396, #61186, #6723, #40768 ) ) ;
#41072=CARTESIAN_POINT ( 'NONE',  ( 145.1370849898475797, 3.309064568108273190E-14, 0.000000000000000000 ) ) ;
#41073=AXIS2_PLACEMENT_3D ( 'NONE', #27798, #48100, #54059 ) ;
#41076=CYLINDRICAL_SURFACE ( 'NONE', #42540, 4.999999999999999112 ) ;
#41077=ORIENTED_EDGE ( 'NONE', *, *, #59094, .T. ) ;
#41078=CARTESIAN_POINT ( 'NONE',  ( -18.07060594675151322, -4.850101347397025364, -12.59940754866924983 ) ) ;
#41079=CARTESIAN_POINT ( 'NONE',  ( -27.66223155157100422, -11.89179406365635217, -6.414297969418397471 ) ) ;
#41081=VERTEX_POINT ( 'NONE', #4507 ) ;
#41082=FACE_OUTER_BOUND ( 'NONE', #1549, .T. ) ;
#41083=FACE_OUTER_BOUND ( 'NONE', #16925, .T. ) ;
#41085=DIRECTION ( 'NONE',  ( 0.000000000000000000, 0.01356324068817998940, -0.9999080150203989437 ) ) ;
#41086=ORIENTED_EDGE ( 'NONE', *, *, #19134, .T. ) ;
#41087=CARTESIAN_POINT ( 'NONE',  ( 35.00000000000000000, -6.265926637539568134, -11.10408318471057321 ) ) ;
#41088=ADVANCED_FACE ( 'NONE', ( #35389 ), #55696, .T. ) ;
#41091=DIRECTION ( 'NONE',  ( -1.000000000000000000, -0.000000000000000000, 0.000000000000000000 ) ) ;
#41093=CYLINDRICAL_SURFACE ( 'NONE', #7800, 12.74999999999999822 ) ;
#41096=DIRECTION ( 'NONE',  ( 0.9946347501772865307, 0.000000000000000000, -0.1034490876700550205 ) ) ;
#41098=ORIENTED_EDGE ( 'NONE', *, *, #42829, .T. ) ;
#41099=DIRECTION ( 'NONE',  ( 1.000000000000000000, 0.000000000000000000, -0.000000000000000000 ) ) ;
#41100=ORIENTED_EDGE ( 'NONE', *, *, #62194, .F. ) ;
#41101=DIRECTION ( 'NONE',  ( 0.000000000000000000, -0.9551603052523448545, 0.2960891610144612551 ) ) ;
#41103=ADVANCED_FACE ( 'NONE', ( #11125 ), #56694, .T. ) ;
#41106=DIRECTION ( 'NONE',  ( -0.000000000000000000, -1.000000000000000000, -0.000000000000000000 ) ) ;
#41107=CARTESIAN_POINT ( 'NONE',  ( 37.00000000000000711, -10.91536515067650903, -4.339012074899918581 ) ) ;
#41108=ADVANCED_FACE ( 'NONE', ( #41697 ), #41358, .T. ) ;
#41109=FACE_BOUND ( 'NONE', #32849, .T. ) ;
#41112=CARTESIAN_POINT ( 'NONE',  ( 26.08439714455133185, -12.97057518889163674, 3.743551691817328386 ) ) ;
#41113=EDGE_CURVE ( 'NONE', #39990, #38220, #31399, .T. ) ;
#41114=ORIENTED_EDGE ( 'NONE', *, *, #16654, .T. ) ;
#41116=AXIS2_PLACEMENT_3D ( 'NONE', #2967, #8581, #43491 ) ;
#41117=DIRECTION ( 'NONE',  ( 0.000000000000000000, 0.7381862504171975425, -0.6745969609292638003 ) ) ;
#41120=CARTESIAN_POINT ( 'NONE',  ( 9.612882454814815958, 13.47023598955341583, -0.9106303824545893821 ) ) ;
#41121=LINE ( 'NONE', #61404, #14704 ) ;
#41122=CIRCLE ( 'NONE', #11413, 4.999999999999998224 ) ;
#41123=EDGE_CURVE ( 'NONE', #31517, #36643, #51381, .T. ) ;
#41125=ORIENTED_EDGE ( 'NONE', *, *, #1605, .T. ) ;
#41126=CARTESIAN_POINT ( 'NONE',  ( -37.00000000000000711, -12.31350058095525846, 3.307597835713201651 ) ) ;
#41127=EDGE_CURVE ( 'NONE', #3400, #23545, #47087, .T. ) ;
#41128=CARTESIAN_POINT ( 'NONE',  ( -37.00000000000000711, -11.54110654723650420, 2.185196060783841432 ) ) ;
#41129=CARTESIAN_POINT ( 'NONE',  ( 35.00000000000000000, 8.830544224263075392, 9.196955404009196755 ) ) ;
#41133=DIRECTION ( 'NONE',  ( 0.000000000000000000, 0.5987040770935622147, -0.8009703041134207391 ) ) ;
#41136=ORIENTED_EDGE ( 'NONE', *, *, #58352, .F. ) ;
#41137=CARTESIAN_POINT ( 'NONE',  ( -37.00000000000000711, -6.891188680298757419, -9.512294188640973758 ) ) ;
#41139=VERTEX_POINT ( 'NONE', #42016 ) ;
#41145=ORIENTED_EDGE ( 'NONE', *, *, #53370, .T. ) ;
#41147=DIRECTION ( 'NONE',  ( 0.000000000000000000, 0.01356324068817999808, -0.9999080150203990547 ) ) ;
#41148=CARTESIAN_POINT ( 'NONE',  ( 37.00000000000000711, 10.54834585426228877, 6.102719229070555862 ) ) ;
#41150=VECTOR ( 'NONE', #49094, 1000.000000000000000 ) ;
#41151=CARTESIAN_POINT ( 'NONE',  ( 8.937200413559443390, 4.476360154859203355, -12.73625532737111143 ) ) ;
#41153=VECTOR ( 'NONE', #7620, 1000.000000000000000 ) ;
#41157=ORIENTED_EDGE ( 'NONE', *, *, #2299, .F. ) ;
#41158=DIRECTION ( 'NONE',  ( 0.000000000000000000, 0.01356324068817998940, -0.9999080150203989437 ) ) ;
#41160=AXIS2_PLACEMENT_3D ( 'NONE', #21854, #22158, #16535 ) ;
#41161=CARTESIAN_POINT ( 'NONE',  ( -35.00000000000000000, 0.000000000000000000, 0.000000000000000000 ) ) ;
#41162=CARTESIAN_POINT ( 'NONE',  ( -8.766550606785775912, -2.870938393825745116, 11.65238521198515187 ) ) ;
#41163=ADVANCED_FACE ( 'NONE', ( #52678 ), #7103, .T. ) ;
#41164=EDGE_CURVE ( 'NONE', #19811, #15014, #12039, .T. ) ;
#41167=VERTEX_POINT ( 'NONE', #52986 ) ;
#41168=CARTESIAN_POINT ( 'NONE',  ( 37.00000000000000711, -8.052525312709825300, 8.551552972817161091 ) ) ;
#41171=DIRECTION ( 'NONE',  ( 0.000000000000000000, 0.01356324068817992175, -0.9999080150203990547 ) ) ;
#41172=DIRECTION ( 'NONE',  ( -0.000000000000000000, -0.000000000000000000, -1.000000000000000000 ) ) ;
#41175=CARTESIAN_POINT ( 'NONE',  ( -6.533703001908491181, -1.140004534245788737, 11.94583671674990555 ) ) ;
#41179=ORIENTED_EDGE ( 'NONE', *, *, #60221, .T. ) ;
#41180=B_SPLINE_CURVE_WITH_KNOTS ( 'NONE', 3,
 ( #53325, #7769, #43651, #23062, #8098, #8414, #22739, #28367, #33680, #58656, #28688, #18070, #33362, #49003 ),
 .UNSPECIFIED., .F., .F.,
 ( 4, 2, 2, 2, 2, 2, 4 ),
 ( 1.301042606982605321E-18, 0.002148955746805324314, 0.003223433620207984303, 0.004297911493610643424, 0.006446867240415959932, 0.007521345113818616451, 0.008595822987221272971 ),
 .UNSPECIFIED. ) ;
#41183=CARTESIAN_POINT ( 'NONE',  ( 18.06777465640019997, 8.467087186347326266, 10.54078692479376045 ) ) ;
#41185=VERTEX_POINT ( 'NONE', #18745 ) ;
#41187=VERTEX_POINT ( 'NONE', #49348 ) ;
#41188=DIRECTION ( 'NONE',  ( -1.000000000000000000, -0.000000000000000000, -0.000000000000000000 ) ) ;
#41192=VERTEX_POINT ( 'NONE', #13719 ) ;
#41193=ORIENTED_EDGE ( 'NONE', *, *, #65168, .F. ) ;
#41194=CYLINDRICAL_SURFACE ( 'NONE', #4544, 12.18650000000000055 ) ;
#41195=B_SPLINE_CURVE_WITH_KNOTS ( 'NONE', 3,
 ( #20633, #62168, #31260, #56533, #55874, #25950, #61834, #5334, #16622, #41212, #41881, #56876, #36223, #21617, #55550, #10976 ),
 .UNSPECIFIED., .F., .F.,
 ( 4, 2, 2, 2, 2, 2, 2, 4 ),
 ( 2.163628596297127287E-17, 0.002218008919589290178, 0.003327013379383922907, 0.004436017839178555203, 0.005545022298973183161, 0.006654026758767811987, 0.007763031218562439946, 0.008872035678357067037 ),
 .UNSPECIFIED. ) ;
#41196=EDGE_CURVE ( 'NONE', #37677, #56356, #63283, .T. ) ;
#41197=ORIENTED_EDGE ( 'NONE', *, *, #21400, .F. ) ;
#41198=CARTESIAN_POINT ( 'NONE',  ( -37.00000000000000711, -11.47561260193580956, 5.556331110570369880 ) ) ;
#41199=ORIENTED_EDGE ( 'NONE', *, *, #31435, .T. ) ;
#41201=ORIENTED_EDGE ( 'NONE', *, *, #22422, .F. ) ;
#41202=DIRECTION ( 'NONE',  ( 0.000000000000000000, -0.01356324068817998940, 0.9999080150203990547 ) ) ;
#41205=CARTESIAN_POINT ( 'NONE',  ( 9.612870878434209843, 11.96650298090372289, -0.9106810471525464967 ) ) ;
#41206=DIRECTION ( 'NONE',  ( 0.000000000000000000, 0.01356324068817992175, -0.9999080150203990547 ) ) ;
#41207=EDGE_LOOP ( 'NONE', ( #51123, #13807, #51168, #13793 ) ) ;
#41208=LINE ( 'NONE', #40227, #3612 ) ;
#41209=AXIS2_PLACEMENT_3D ( 'NONE', #38633, #31983, #52633 ) ;
#41210=ORIENTED_EDGE ( 'NONE', *, *, #34680, .F. ) ;
#41211=DIRECTION ( 'NONE',  ( -1.000000000000000000, 0.000000000000000000, 0.000000000000000000 ) ) ;
#41212=CARTESIAN_POINT ( 'NONE',  ( -3.491752571392269910, 11.78957267686408095, 6.587477860936952645 ) ) ;
#41216=CARTESIAN_POINT ( 'NONE',  ( 28.45979645211560438, 10.25197200398427810, 6.251877464400086737 ) ) ;
#41218=AXIS2_PLACEMENT_3D ( 'NONE', #31644, #61265, #51955 ) ;
#41219=EDGE_CURVE ( 'NONE', #31308, #45530, #14165, .T. ) ;
#41220=ORIENTED_EDGE ( 'NONE', *, *, #37598, .T. ) ;
#41221=DIRECTION ( 'NONE',  ( 0.000000000000000000, -0.9903235168508535136, -0.1387779952735919697 ) ) ;
#41222=EDGE_CURVE ( 'NONE', #29123, #14422, #21946, .T. ) ;
#41223=ORIENTED_EDGE ( 'NONE', *, *, #38160, .T. ) ;
#41224=CARTESIAN_POINT ( 'NONE',  ( -24.38941346611472483, -9.755923631413494945, 9.333302870830756603 ) ) ;
#41227=EDGE_CURVE ( 'NONE', #13636, #23085, #18435, .T. ) ;
#41228=CARTESIAN_POINT ( 'NONE',  ( 35.00000000000000000, -8.389074212634222150, 8.839356091080130540 ) ) ;
#41229=CARTESIAN_POINT ( 'NONE',  ( 35.00000000000000000, 11.66953048682399441, -3.511814412392164186 ) ) ;
#41230=VERTEX_POINT ( 'NONE', #48671 ) ;
#41231=FACE_OUTER_BOUND ( 'NONE', #1487, .T. ) ;
#41233=CARTESIAN_POINT ( 'NONE',  ( 35.00000000000000000, 8.927548052240892318, -8.295159312811890118 ) ) ;
#41234=CARTESIAN_POINT ( 'NONE',  ( 23.89564968379661281, -11.31614867562879034, -7.366089092235777791 ) ) ;
#41236=CYLINDRICAL_SURFACE ( 'NONE', #15928, 6.595312090839647645 ) ;
#41243=EDGE_CURVE ( 'NONE', #54635, #50600, #39319, .T. ) ;
#41245=EDGE_CURVE ( 'NONE', #15906, #27211, #55582, .T. ) ;
#41246=VECTOR ( 'NONE', #47882, 1000.000000000000000 ) ;
#41251=CARTESIAN_POINT ( 'NONE',  ( -35.00000000000000000, 0.000000000000000000, 0.000000000000000000 ) ) ;
#41252=AXIS2_PLACEMENT_3D ( 'NONE', #28627, #22675, #43255 ) ;
#41254=VERTEX_POINT ( 'NONE', #63946 ) ;
#41255=EDGE_CURVE ( 'NONE', #45626, #56247, #43894, .T. ) ;
#41257=AXIS2_PLACEMENT_3D ( 'NONE', #28881, #8930, #3952 ) ;
#41258=EDGE_LOOP ( 'NONE', ( #65800, #38183, #31697, #37997 ) ) ;
#41260=DIRECTION ( 'NONE',  ( -1.000000000000000000, -0.000000000000000000, 0.000000000000000000 ) ) ;
#41261=ORIENTED_EDGE ( 'NONE', *, *, #21400, .T. ) ;
#41262=DIRECTION ( 'NONE',  ( 1.000000000000000000, 0.000000000000000000, 0.000000000000000000 ) ) ;
#41263=CARTESIAN_POINT ( 'NONE',  ( 37.00000000000000711, 4.705694406421931860E-17, -3.469127814946512892E-15 ) ) ;
#41264=ORIENTED_EDGE ( 'NONE', *, *, #24030, .T. ) ;
#41267=DIRECTION ( 'NONE',  ( -1.000000000000000000, 0.000000000000000000, 0.000000000000000000 ) ) ;
#41268=ORIENTED_EDGE ( 'NONE', *, *, #17408, .T. ) ;
#41269=CARTESIAN_POINT ( 'NONE',  ( 145.1370849898475797, 3.309064568108273190E-14, 0.000000000000000000 ) ) ;
#41270=EDGE_CURVE ( 'NONE', #50979, #52347, #15217, .T. ) ;
#41271=ORIENTED_EDGE ( 'NONE', *, *, #24901, .F. ) ;
#41273=ORIENTED_EDGE ( 'NONE', *, *, #7929, .T. ) ;
#41278=DIRECTION ( 'NONE',  ( 0.000000000000000000, 0.01356324068817992175, -0.9999080150203990547 ) ) ;
#41279=AXIS2_PLACEMENT_3D ( 'NONE', #57202, #41892, #21948 ) ;
#41283=CARTESIAN_POINT ( 'NONE',  ( 35.00000000000000000, 7.215058775251253387, -9.821084925794595577 ) ) ;
#41284=CARTESIAN_POINT ( 'NONE',  ( 5.329935900150571726, -10.23194172168328464, 8.808226182152964157 ) ) ;
#41285=VERTEX_POINT ( 'NONE', #29352 ) ;
#41286=CARTESIAN_POINT ( 'NONE',  ( 37.00000000000000711, 8.052525312709883920, -8.551552972817113130 ) ) ;
#41287=ORIENTED_EDGE ( 'NONE', *, *, #32541, .F. ) ;
#41288=CIRCLE ( 'NONE', #957, 12.74999999999999822 ) ;
#41290=CARTESIAN_POINT ( 'NONE',  ( 35.00000000000000000, 12.01765980939841683, -2.021542716731445921 ) ) ;
#41291=ORIENTED_EDGE ( 'NONE', *, *, #50736, .T. ) ;
#41297=EDGE_CURVE ( 'NONE', #24621, #33199, #3582, .T. ) ;
#41298=CARTESIAN_POINT ( 'NONE',  ( 29.03457606387295087, -7.862146963512102182, 10.97436308512422265 ) ) ;
#41299=ORIENTED_EDGE ( 'NONE', *, *, #10363, .T. ) ;
#41300=CYLINDRICAL_SURFACE ( 'NONE', #5680, 12.74999999999999822 ) ;
#41301=ADVANCED_FACE ( 'NONE', ( #30341 ), #59959, .T. ) ;
#41302=CIRCLE ( 'NONE', #52993, 4.999999999999999112 ) ;
#41304=CARTESIAN_POINT ( 'NONE',  ( 35.00000000000000000, 10.54834585426228877, 6.102719229070555862 ) ) ;
#41305=DIRECTION ( 'NONE',  ( -1.000000000000000000, 0.000000000000000000, -0.000000000000000000 ) ) ;
#41307=ORIENTED_EDGE ( 'NONE', *, *, #22336, .T. ) ;
#41308=CIRCLE ( 'NONE', #65688, 12.75000000000000178 ) ;
#41312=DIRECTION ( 'NONE',  ( 1.000000000000000000, 0.000000000000000000, 0.000000000000000000 ) ) ;
#41313=CARTESIAN_POINT ( 'NONE',  ( 9.384597055785796726, 7.262755914012919867, 11.38454852282039198 ) ) ;
#41314=DIRECTION ( 'NONE',  ( 1.000000000000000000, 0.000000000000000000, 0.000000000000000000 ) ) ;
#41315=CARTESIAN_POINT ( 'NONE',  ( 37.00000000000000711, 8.146229107149528303, 9.063649021438866527 ) ) ;
#41318=ORIENTED_EDGE ( 'NONE', *, *, #39577, .F. ) ;
#41319=CARTESIAN_POINT ( 'NONE',  ( 35.00000000000000000, -11.73808581813437613, 0.4353888892049613824 ) ) ;
#41320=DIRECTION ( 'NONE',  ( 0.000000000000000000, -0.01356324068817998940, 0.9999080150203990547 ) ) ;
#41321=ADVANCED_FACE ( 'NONE', ( #65560 ), #10365, .T. ) ;
#41326=DIRECTION ( 'NONE',  ( 0.000000000000000000, -0.3218879778915842427, 0.9467777615094616905 ) ) ;
#41331=CYLINDRICAL_SURFACE ( 'NONE', #37023, 5.000000000000000888 ) ;
#41332=ORIENTED_EDGE ( 'NONE', *, *, #53491, .F. ) ;
#41333=ORIENTED_EDGE ( 'NONE', *, *, #48663, .T. ) ;
#41334=CIRCLE ( 'NONE', #43426, 5.000000000000001776 ) ;
#41337=ORIENTED_EDGE ( 'NONE', *, *, #64696, .F. ) ;
#41340=LINE ( 'NONE', #11733, #48224 ) ;
#41346=DIRECTION ( 'NONE',  ( 1.000000000000000000, -0.000000000000000000, 0.000000000000000000 ) ) ;
#41348=ORIENTED_EDGE ( 'NONE', *, *, #60490, .T. ) ;
#41350=ADVANCED_FACE ( 'NONE', ( #60929 ), #34340, .T. ) ;
#41351=ORIENTED_EDGE ( 'NONE', *, *, #41113, .T. ) ;
#41352=CARTESIAN_POINT ( 'NONE',  ( -35.00000000000000000, 8.927548052241016663, -8.295159312811756891 ) ) ;
#41354=ORIENTED_EDGE ( 'NONE', *, *, #49689, .F. ) ;
#41357=EDGE_CURVE ( 'NONE', #23545, #21056, #40714, .T. ) ;
#41358=CYLINDRICAL_SURFACE ( 'NONE', #54545, 12.18649999999999878 ) ;
#41361=CARTESIAN_POINT ( 'NONE',  ( -20.73885153823040639, 11.61492743593955801, -3.067692064997443957 ) ) ;
#41364=ORIENTED_EDGE ( 'NONE', *, *, #209, .F. ) ;
#41365=LINE ( 'NONE', #9461, #56070 ) ;
#41369=DIRECTION ( 'NONE',  ( 0.000000000000000000, -0.01356324068817998940, 0.9999080150203990547 ) ) ;
#41371=DIRECTION ( 'NONE',  ( 0.000000000000000000, -0.01356324068817998940, 0.9999080150203990547 ) ) ;
#41374=CARTESIAN_POINT ( 'NONE',  ( -8.891032880924177206, 25.00000000000000000, -3.860857758255646921 ) ) ;
#41376=AXIS2_PLACEMENT_3D ( 'NONE', #1253, #36131, #51141 ) ;
#41378=AXIS2_PLACEMENT_3D ( 'NONE', #62394, #13422, #19416 ) ;
#41380=CARTESIAN_POINT ( 'NONE',  ( -37.00000000000000711, 0.000000000000000000, 0.000000000000000000 ) ) ;
#41383=CARTESIAN_POINT ( 'NONE',  ( 6.147033604836291687, -8.616929040695943343, 8.360196263819061002 ) ) ;
#41384=DIRECTION ( 'NONE',  ( 0.000000000000000000, 0.8989688749565172277, 0.4380125133593943398 ) ) ;
#41385=AXIS2_PLACEMENT_3D ( 'NONE', #39543, #65139, #28922 ) ;
#41386=CARTESIAN_POINT ( 'NONE',  ( -35.00000000000000000, 10.99909370905157324, 5.246972444134057056 ) ) ;
#41389=ORIENTED_EDGE ( 'NONE', *, *, #49, .T. ) ;
#41391=DIRECTION ( 'NONE',  ( 0.000000000000000000, 0.01356324068817298112, -0.9999080150203990547 ) ) ;
#41394=CARTESIAN_POINT ( 'NONE',  ( -28.85619398320021745, 3.750539801530000439, 12.96855624952675612 ) ) ;
#41395=DIRECTION ( 'NONE',  ( -1.000000000000000000, 0.000000000000000000, 0.000000000000000000 ) ) ;
#41396=EDGE_CURVE ( 'NONE', #58893, #8992, #39978, .T. ) ;
#41399=CARTESIAN_POINT ( 'NONE',  ( -35.00000000000000000, 0.000000000000000000, 0.000000000000000000 ) ) ;
#41406=DIRECTION ( 'NONE',  ( 0.000000000000000000, 0.01356324068817998940, -0.9999080150203990547 ) ) ;
#41409=AXIS2_PLACEMENT_3D ( 'NONE', #61034, #45726, #4534 ) ;
#41410=EDGE_CURVE ( 'NONE', #60081, #64143, #55621, .T. ) ;
#41411=DIRECTION ( 'NONE',  ( 0.000000000000000000, -0.01356324068817991828, 0.9999080150203990547 ) ) ;
#41412=ORIENTED_EDGE ( 'NONE', *, *, #45939, .F. ) ;
#41413=LINE ( 'NONE', #42382, #23784 ) ;
#41416=DIRECTION ( 'NONE',  ( -1.000000000000000000, 0.000000000000000000, 0.000000000000000000 ) ) ;
#41417=DIRECTION ( 'NONE',  ( 0.000000000000000000, 0.6745969609292609137, 0.7381862504172000961 ) ) ;
#41420=ORIENTED_EDGE ( 'NONE', *, *, #14337, .T. ) ;
#41421=ADVANCED_FACE ( 'NONE', ( #30982 ), #53507, .T. ) ;
#41422=ORIENTED_EDGE ( 'NONE', *, *, #65610, .T. ) ;
#41423=CARTESIAN_POINT ( 'NONE',  ( 35.00000000000000000, -10.80478261802177897, 5.636262487437428526 ) ) ;
#41424=ORIENTED_EDGE ( 'NONE', *, *, #14604, .T. ) ;
#41425=CYLINDRICAL_SURFACE ( 'NONE', #24145, 5.000000000000000888 ) ;
#41426=AXIS2_PLACEMENT_3D ( 'NONE', #29483, #65386, #54464 ) ;
#41427=CARTESIAN_POINT ( 'NONE',  ( -17.97314397134535469, 4.332534348537287805, 11.19277487034911012 ) ) ;
#41429=CARTESIAN_POINT ( 'NONE',  ( 35.00000000000000000, -2.936739658819788712, 11.37311665002366290 ) ) ;
#41430=AXIS2_PLACEMENT_3D ( 'NONE', #13221, #23197, #43457 ) ;
#41432=CARTESIAN_POINT ( 'NONE',  ( 35.00000000000000000, -10.39746860227895731, -7.379373053628834889 ) ) ;
#41433=CARTESIAN_POINT ( 'NONE',  ( -24.62662350575228487, -9.678819843908897269, 7.096674636486683063 ) ) ;
#41437=CARTESIAN_POINT ( 'NONE',  ( 27.76677820897042182, -12.45056549256346479, 5.221417433310395317 ) ) ;
#41438=ORIENTED_EDGE ( 'NONE', *, *, #61923, .F. ) ;
#41439=CIRCLE ( 'NONE', #64789, 12.74999999999999822 ) ;
#41440=CARTESIAN_POINT ( 'NONE',  ( 23.20859878307385316, -9.989936526681711726, -6.655393916305755830 ) ) ;
#41445=CARTESIAN_POINT ( 'NONE',  ( 26.25871678826176847, -11.49115831596997062, 3.460539353551115305 ) ) ;
#41447=CIRCLE ( 'NONE', #38277, 12.74999999999999822 ) ;
#41448=ORIENTED_EDGE ( 'NONE', *, *, #2492, .T. ) ;
#41449=DIRECTION ( 'NONE',  ( -1.000000000000000000, 0.000000000000000000, 0.000000000000000000 ) ) ;
#41450=AXIS2_PLACEMENT_3D ( 'NONE', #2185, #41416, #62055 ) ;
#41451=DIRECTION ( 'NONE',  ( 1.000000000000000000, 0.000000000000000000, -0.000000000000000000 ) ) ;
#41452=DIRECTION ( 'NONE',  ( 1.000000000000000000, -0.000000000000000000, -0.000000000000000000 ) ) ;
#41453=CARTESIAN_POINT ( 'NONE',  ( -7.962338368258669696, 7.023910026709175192, -9.755115923264007449 ) ) ;
#41454=CARTESIAN_POINT ( 'NONE',  ( -37.00000000000000711, -0.7214809346827719683, -11.72397916322013245 ) ) ;
#41455=FACE_OUTER_BOUND ( 'NONE', #17510, .T. ) ;
#41456=ORIENTED_EDGE ( 'NONE', *, *, #41882, .F. ) ;
#41457=EDGE_CURVE ( 'NONE', #33917, #48302, #12569, .T. ) ;
#41458=AXIS2_PLACEMENT_3D ( 'NONE', #40089, #8870, #34461 ) ;
#41462=LINE ( 'NONE', #278, #19517 ) ;
#41463=EDGE_LOOP ( 'NONE', ( #12230, #65481, #21779, #54870 ) ) ;
#41467=DIRECTION ( 'NONE',  ( -1.000000000000000000, -1.836970198721029688E-16, -0.000000000000000000 ) ) ;
#41470=FACE_OUTER_BOUND ( 'NONE', #3346, .T. ) ;
#41471=DIRECTION ( 'NONE',  ( 0.000000000000000000, -0.2006870767258961963, 0.9796553971857727694 ) ) ;
#41473=CIRCLE ( 'NONE', #43570, 5.000000000000001776 ) ;
#41475=CIRCLE ( 'NONE', #30844, 12.18650000000000055 ) ;
#41477=DIRECTION ( 'NONE',  ( 0.000000000000000000, -0.01356324068817999114, 0.9999080150203989437 ) ) ;
#41478=ORIENTED_EDGE ( 'NONE', *, *, #53310, .F. ) ;
#41479=EDGE_CURVE ( 'NONE', #37563, #10290, #54602, .T. ) ;
#41480=CARTESIAN_POINT ( 'NONE',  ( 47.00000000000000711, 4.705694406421931860E-17, -3.469127814946512892E-15 ) ) ;
#41481=ORIENTED_EDGE ( 'NONE', *, *, #15589, .T. ) ;
#41482=EDGE_CURVE ( 'NONE', #2029, #39221, #64115, .T. ) ;
#41487=CARTESIAN_POINT ( 'NONE',  ( 26.83852350919729801, -11.22119259825004711, 4.265317526618762400 ) ) ;
#41488=CARTESIAN_POINT ( 'NONE',  ( -9.068975030232913070, -3.147254398582626678, 11.58080990864780979 ) ) ;
#41489=EDGE_LOOP ( 'NONE', ( #7133, #2953, #60712, #33418 ) ) ;
#41490=EDGE_CURVE ( 'NONE', #49219, #47265, #16007, .T. ) ;
#41491=ORIENTED_EDGE ( 'NONE', *, *, #43907, .F. ) ;
#41493=ORIENTED_EDGE ( 'NONE', *, *, #39535, .T. ) ;
#41498=CARTESIAN_POINT ( 'NONE',  ( 37.00000000000000711, -4.237620530777882699, -11.42599468261428086 ) ) ;
#41499=CARTESIAN_POINT ( 'NONE',  ( -35.00000000000000000, -11.98254675519229906, 2.220215194441857331 ) ) ;
#41501=CARTESIAN_POINT ( 'NONE',  ( 35.00000000000000000, -3.340853584269612764, -11.26103545359855040 ) ) ;
#41504=AXIS2_PLACEMENT_3D ( 'NONE', #5882, #26140, #31757 ) ;
#41506=ORIENTED_EDGE ( 'NONE', *, *, #46094, .T. ) ;
#41507=CARTESIAN_POINT ( 'NONE',  ( 21.75117853020661585, -12.54259235896871694, -4.997187019246493556 ) ) ;
#41508=AXIS2_PLACEMENT_3D ( 'NONE', #13123, #29706, #48709 ) ;
#41509=DIRECTION ( 'NONE',  ( 0.000000000000000000, -0.6478160128812003871, 0.7617968321374831708 ) ) ;
#41510=AXIS2_PLACEMENT_3D ( 'NONE', #28839, #18219, #13224 ) ;
#41511=ORIENTED_EDGE ( 'NONE', *, *, #49286, .F. ) ;
#41513=DIRECTION ( 'NONE',  ( 0.000000000000000000, -0.7790879021242440583, 0.6269146997508067143 ) ) ;
#41516=DIRECTION ( 'NONE',  ( 0.2227494284590502138, 0.000000000000000000, 0.9748757316300199482 ) ) ;
#41518=AXIS2_PLACEMENT_3D ( 'NONE', #23399, #48026, #24063 ) ;
#41519=DIRECTION ( 'NONE',  ( 1.000000000000000000, 0.000000000000000000, 0.000000000000000000 ) ) ;
#41521=VERTEX_POINT ( 'NONE', #42495 ) ;
#41522=ADVANCED_FACE ( 'NONE', ( #48510 ), #32522, .F. ) ;
#41523=DIRECTION ( 'NONE',  ( 0.000000000000000000, -0.01356324068817991828, 0.9999080150203990547 ) ) ;
#41524=ORIENTED_EDGE ( 'NONE', *, *, #37502, .T. ) ;
#41525=CARTESIAN_POINT ( 'NONE',  ( -35.00000000000000000, 0.01609748574461371262, -11.74614673114903951 ) ) ;
#41528=ORIENTED_EDGE ( 'NONE', *, *, #29081, .F. ) ;
#41530=CARTESIAN_POINT ( 'NONE',  ( 37.00000000000000711, -4.237174932027311769, -12.02534193257719686 ) ) ;
#41533=DIRECTION ( 'NONE',  ( 0.000000000000000000, -0.9467777615094604693, -0.3218879778915876289 ) ) ;
#41535=PLANE ( 'NONE',  #62465 ) ;
#41536=ORIENTED_EDGE ( 'NONE', *, *, #39630, .T. ) ;
#41538=CARTESIAN_POINT ( 'NONE',  ( 35.00000000000000000, 4.018060380616396365, -11.50504120060944757 ) ) ;
#41539=( BOUNDED_CURVE ( )  B_SPLINE_CURVE ( 3, ( #16031, #15394, #15699, #35977 ),
 .UNSPECIFIED., .F., .F. ) 
 B_SPLINE_CURVE_WITH_KNOTS ( ( 4, 4 ),
 ( 4.755771627453653672, 4.791948434006704005 ),
 .UNSPECIFIED. ) 
 CURVE ( )  GEOMETRIC_REPRESENTATION_ITEM ( )  RATIONAL_B_SPLINE_CURVE ( ( 1.000000000000000000, 0.9998909395293115177, 0.9998909395293115177, 1.000000000000000000 ) ) 
 REPRESENTATION_ITEM ( '' )  );
#41540=ORIENTED_EDGE ( 'NONE', *, *, #26702, .F. ) ;
#41543=VECTOR ( 'NONE', #23287, 1000.000000000000000 ) ;
#41544=FACE_OUTER_BOUND ( 'NONE', #49998, .T. ) ;
#41547=AXIS2_PLACEMENT_3D ( 'NONE', #26828, #47129, #18523 ) ;
#41550=ORIENTED_EDGE ( 'NONE', *, *, #44115, .F. ) ;
#41551=CARTESIAN_POINT ( 'NONE',  ( 35.00000000000000000, 4.705694406421931860E-17, -3.469127814946512892E-15 ) ) ;
#41552=CIRCLE ( 'NONE', #12886, 4.999999999999999112 ) ;
#41553=ORIENTED_EDGE ( 'NONE', *, *, #22585, .T. ) ;
#41559=VECTOR ( 'NONE', #43295, 1000.000000000000000 ) ;
#41562=EDGE_CURVE ( 'NONE', #48679, #46698, #3633, .T. ) ;
#41563=DIRECTION ( 'NONE',  ( -1.000000000000000000, 0.000000000000000000, 0.000000000000000000 ) ) ;
#41565=CARTESIAN_POINT ( 'NONE',  ( 21.47693580707085559, 11.78067291942578443, -2.319680692362900754 ) ) ;
#41566=DIRECTION ( 'NONE',  ( 1.000000000000000000, 0.000000000000000000, 0.000000000000000000 ) ) ;
#41567=AXIS2_PLACEMENT_3D ( 'NONE', #9941, #4647, #39538 ) ;
#41570=EDGE_CURVE ( 'NONE', #19519, #64188, #438, .T. ) ;
#41571=DIRECTION ( 'NONE',  ( -0.000000000000000000, -1.000000000000000000, -0.000000000000000000 ) ) ;
#41573=ADVANCED_FACE ( 'NONE', ( #27892 ), #58154, .T. ) ;
#41574=DIRECTION ( 'NONE',  ( 0.000000000000000000, 0.01356324068817992175, -0.9999080150203990547 ) ) ;
#41576=CARTESIAN_POINT ( 'NONE',  ( 36.00000000000000711, 10.84030624090615724, 6.711949091238026632 ) ) ;
#41578=AXIS2_PLACEMENT_3D ( 'NONE', #35779, #25840, #42087 ) ;
#41579=AXIS2_PLACEMENT_3D ( 'NONE', #21564, #11888, #47486 ) ;
#41580=EDGE_LOOP ( 'NONE', ( #8403, #59332, #27075, #53379 ) ) ;
#41582=ORIENTED_EDGE ( 'NONE', *, *, #62290, .T. ) ;
#41585=LINE ( 'NONE', #31295, #6699 ) ;
#41587=VECTOR ( 'NONE', #21415, 1000.000000000000000 ) ;
#41589=EDGE_LOOP ( 'NONE', ( #41536, #19262, #31010, #8798 ) ) ;
#41590=EDGE_CURVE ( 'NONE', #3801, #58474, #38683, .T. ) ;
#41591=AXIS2_PLACEMENT_3D ( 'NONE', #3213, #23481, #59380 ) ;
#41593=EDGE_LOOP ( 'NONE', ( #21820, #20966, #47733, #65137 ) ) ;
#41595=EDGE_CURVE ( 'NONE', #58998, #29569, #31225, .T. ) ;
#41597=ORIENTED_EDGE ( 'NONE', *, *, #22409, .F. ) ;
#41598=EDGE_CURVE ( 'NONE', #62046, #53449, #23560, .T. ) ;
#41600=EDGE_CURVE ( 'NONE', #416, #29168, #8912, .T. ) ;
#41601=CIRCLE ( 'NONE', #55420, 5.000000000000000000 ) ;
#41602=FACE_OUTER_BOUND ( 'NONE', #12829, .T. ) ;
#41603=EDGE_LOOP ( 'NONE', ( #48099, #50936, #36397, #5258 ) ) ;
#41610=ORIENTED_EDGE ( 'NONE', *, *, #6068, .F. ) ;
#41614=DIRECTION ( 'NONE',  ( 1.000000000000000000, 0.000000000000000000, 0.000000000000000000 ) ) ;
#41615=AXIS2_PLACEMENT_3D ( 'NONE', #3639, #13879, #39162 ) ;
#41617=AXIS2_PLACEMENT_3D ( 'NONE', #48394, #2842, #63317 ) ;
#41618=CARTESIAN_POINT ( 'NONE',  ( 37.00000000000000711, 4.705694406421931860E-17, -3.469127814946512892E-15 ) ) ;
#41619=CARTESIAN_POINT ( 'NONE',  ( -30.09739282105660862, -2.991438519309432387, -13.18809029152657608 ) ) ;
#41620=CARTESIAN_POINT ( 'NONE',  ( 8.538029044866334516, 5.442243673389044467, -10.69694707505074760 ) ) ;
#41621=CARTESIAN_POINT ( 'NONE',  ( -18.58686583997247155, 5.151216734910867068, -12.47858029384659417 ) ) ;
#41624=VERTEX_POINT ( 'NONE', #59143 ) ;
#41626=CYLINDRICAL_SURFACE ( 'NONE', #36213, 12.75000000000000178 ) ;
#41627=ORIENTED_EDGE ( 'NONE', *, *, #25875, .T. ) ;
#41630=CARTESIAN_POINT ( 'NONE',  ( -47.00000000000000711, 0.000000000000000000, 0.000000000000000000 ) ) ;
#41632=AXIS2_PLACEMENT_3D ( 'NONE', #14055, #24362, #34345 ) ;
#41633=DIRECTION ( 'NONE',  ( 1.000000000000000000, 0.000000000000000000, 0.000000000000000000 ) ) ;
#41634=EDGE_CURVE ( 'NONE', #36481, #48679, #12084, .T. ) ;
#41635=ORIENTED_EDGE ( 'NONE', *, *, #36721, .T. ) ;
#41636=CARTESIAN_POINT ( 'NONE',  ( -17.13740638563841756, -7.345997652321633709, -9.495308414869118252 ) ) ;
#41638=ORIENTED_EDGE ( 'NONE', *, *, #26045, .T. ) ;
#41639=CYLINDRICAL_SURFACE ( 'NONE', #32772, 5.000000000000000888 ) ;
#41641=DIRECTION ( 'NONE',  ( -1.000000000000000000, 0.000000000000000000, 0.000000000000000000 ) ) ;
#41642=DIRECTION ( 'NONE',  ( -1.000000000000000000, 0.000000000000000000, -0.000000000000000000 ) ) ;
#41643=ORIENTED_EDGE ( 'NONE', *, *, #4053, .T. ) ;
#41644=ADVANCED_FACE ( 'NONE', ( #33839 ), #8577, .T. ) ;
#41647=CARTESIAN_POINT ( 'NONE',  ( 27.37598419994968069, 12.63452493104432506, 4.764905059084485472 ) ) ;
#41648=CYLINDRICAL_SURFACE ( 'NONE', #25629, 12.74999999999999822 ) ;
#41651=EDGE_CURVE ( 'NONE', #23831, #6864, #45032, .T. ) ;
#41652=DIRECTION ( 'NONE',  ( 0.000000000000000000, -0.9551603052523510717, 0.2960891610144412156 ) ) ;
#41654=CARTESIAN_POINT ( 'NONE',  ( -35.00000000000000000, 10.70999494708501132, -5.814360711498173018 ) ) ;
#41655=AXIS2_PLACEMENT_3D ( 'NONE', #17976, #41923, #53571 ) ;
#41657=VECTOR ( 'NONE', #2066, 1000.000000000000000 ) ;
#41658=CIRCLE ( 'NONE', #18342, 5.000000000000001776 ) ;
#41659=ORIENTED_EDGE ( 'NONE', *, *, #42803, .T. ) ;
#41660=FACE_OUTER_BOUND ( 'NONE', #25733, .T. ) ;
#41662=ORIENTED_EDGE ( 'NONE', *, *, #60447, .F. ) ;
#41665=CARTESIAN_POINT ( 'NONE',  ( -9.734731986197230569, 12.56932029542845974, -4.929511566481978413 ) ) ;
#41668=CARTESIAN_POINT ( 'NONE',  ( -17.50255050041978677, 2.687144849813047909, 11.69642965478562324 ) ) ;
#41671=LINE ( 'NONE', #7393, #6242 ) ;
#41673=VERTEX_POINT ( 'NONE', #3632 ) ;
#41675=EDGE_CURVE ( 'NONE', #65264, #40614, #13873, .T. ) ;
#41676=DIRECTION ( 'NONE',  ( 1.000000000000000000, 0.000000000000000000, 0.000000000000000000 ) ) ;
#41677=ORIENTED_EDGE ( 'NONE', *, *, #58148, .F. ) ;
#41678=ADVANCED_FACE ( 'NONE', ( #54479 ), #8911, .T. ) ;
#41679=CARTESIAN_POINT ( 'NONE',  ( -25.95039640524091951, -10.26692734564517195, 6.213570374660478457 ) ) ;
#41681=DIRECTION ( 'NONE',  ( -1.000000000000000000, 0.000000000000000000, 0.000000000000000000 ) ) ;
#41683=EDGE_LOOP ( 'NONE', ( #3324, #27289, #42972, #12794, #24325, #14594 ) ) ;
#41688=DIRECTION ( 'NONE',  ( 1.000000000000000000, 0.000000000000000000, 0.000000000000000000 ) ) ;
#41691=CARTESIAN_POINT ( 'NONE',  ( -28.12644806133159392, 10.04153257883247363, -6.577776757711345290 ) ) ;
#41692=ORIENTED_EDGE ( 'NONE', *, *, #6714, .T. ) ;
#41694=VERTEX_POINT ( 'NONE', #59835 ) ;
#41696=DIRECTION ( 'NONE',  ( -1.000000000000000000, 0.000000000000000000, 0.000000000000000000 ) ) ;
#41697=FACE_OUTER_BOUND ( 'NONE', #63320, .T. ) ;
#41700=ADVANCED_FACE ( 'NONE', ( #46181 ), #301, .T. ) ;
#41701=FACE_OUTER_BOUND ( 'NONE', #24746, .T. ) ;
#41703=ORIENTED_EDGE ( 'NONE', *, *, #38696, .T. ) ;
#41704=CIRCLE ( 'NONE', #30025, 5.000000000000000888 ) ;
#41707=ORIENTED_EDGE ( 'NONE', *, *, #41064, .T. ) ;
#41708=EDGE_LOOP ( 'NONE', ( #10453, #58174, #51392, #10954 ) ) ;
#41709=LINE ( 'NONE', #62311, #25351 ) ;
#41710=VECTOR ( 'NONE', #41260, 1000.000000000000000 ) ;
#41713=CARTESIAN_POINT ( 'NONE',  ( -47.00000000000000711, 0.000000000000000000, 0.000000000000000000 ) ) ;
#41714=DIRECTION ( 'NONE',  ( 0.000000000000000000, 0.2355298848897516562, 0.9718671068226458765 ) ) ;
#41715=CARTESIAN_POINT ( 'NONE',  ( -9.862567555648398709, -3.268643206080108499, -11.54748364193017451 ) ) ;
#41717=DIRECTION ( 'NONE',  ( 1.000000000000000000, 0.000000000000000000, 0.000000000000000000 ) ) ;
#41719=ORIENTED_EDGE ( 'NONE', *, *, #40086, .F. ) ;
#41720=DIRECTION ( 'NONE',  ( 1.000000000000000000, -0.000000000000000000, -0.000000000000000000 ) ) ;
#41721=CARTESIAN_POINT ( 'NONE',  ( -3.384821952288626257, -5.980207314672072449, 10.44102928066339331 ) ) ;
#41722=AXIS2_PLACEMENT_3D ( 'NONE', #2149, #32064, #22777 ) ;
#41723=EDGE_CURVE ( 'NONE', #1524, #54137, #34395, .T. ) ;
#41726=DIRECTION ( 'NONE',  ( -1.000000000000000000, 0.000000000000000000, -0.000000000000000000 ) ) ;
#41732=EDGE_LOOP ( 'NONE', ( #23304, #33609, #17016, #23505, #39483, #30893 ) ) ;
#41733=CARTESIAN_POINT ( 'NONE',  ( -19.02967556479664069, -11.99999999999998934, 9.262893081595934602E-16 ) ) ;
#41734=DIRECTION ( 'NONE',  ( 0.000000000000000000, -0.01356324068817999114, 0.9999080150203989437 ) ) ;
#41737=ADVANCED_FACE ( 'NONE', ( #60807 ), #19910, .T. ) ;
#41738=AXIS2_PLACEMENT_3D ( 'NONE', #25035, #45306, #40302 ) ;
#41739=CARTESIAN_POINT ( 'NONE',  ( 35.00000000000000000, 4.705694406421931860E-17, -3.469127814946512892E-15 ) ) ;
#41744=DIRECTION ( 'NONE',  ( 1.000000000000000000, 0.000000000000000000, 0.000000000000000000 ) ) ;
#41746=ORIENTED_EDGE ( 'NONE', *, *, #63719, .T. ) ;
#41748=CYLINDRICAL_SURFACE ( 'NONE', #48054, 4.999999999999999112 ) ;
#41750=AXIS2_PLACEMENT_3D ( 'NONE', #56772, #27454, #21155 ) ;
#41751=CARTESIAN_POINT ( 'NONE',  ( 35.00000000000000000, 6.547236723514018308, -9.752226076388918585 ) ) ;
#41752=ORIENTED_EDGE ( 'NONE', *, *, #61961, .F. ) ;
#41753=CARTESIAN_POINT ( 'NONE',  ( 35.00000000000000000, 9.430788938294046631, -7.718225330433843290 ) ) ;
#41754=EDGE_CURVE ( 'NONE', #32750, #9298, #62029, .T. ) ;
#41755=DIRECTION ( 'NONE',  ( 0.000000000000000000, -0.01356324068817991828, 0.9999080150203990547 ) ) ;
#41758=CARTESIAN_POINT ( 'NONE',  ( 36.00000000000000711, 4.237174932027401475, 12.02534193257715600 ) ) ;
#41759=DIRECTION ( 'NONE',  ( 0.000000000000000000, 0.01356324068817998940, -0.9999080150203990547 ) ) ;
#41761=DIRECTION ( 'NONE',  ( -1.000000000000000000, -0.000000000000000000, 0.000000000000000000 ) ) ;
#41762=DIRECTION ( 'NONE',  ( 0.000000000000000000, 0.01356324068818000848, -0.9999080150203990547 ) ) ;
#41764=ORIENTED_EDGE ( 'NONE', *, *, #53920, .F. ) ;
#41765=VERTEX_POINT ( 'NONE', #19602 ) ;
#41767=VERTEX_POINT ( 'NONE', #60146 ) ;
#41770=CIRCLE ( 'NONE', #30044, 12.75000000000000178 ) ;
#41771=CARTESIAN_POINT ( 'NONE',  ( 36.00000000000000711, 11.47561260193577048, -5.556331110570448928 ) ) ;
#41773=ORIENTED_EDGE ( 'NONE', *, *, #30998, .F. ) ;
#41776=CARTESIAN_POINT ( 'NONE',  ( -35.00000000000000000, -8.839356091079983102, -8.389074212634382022 ) ) ;
#41777=B_SPLINE_CURVE_WITH_KNOTS ( 'NONE', 3,
 ( #43127, #12877, #27850, #17876, #18559, #33156, #8877, #17556 ),
 .UNSPECIFIED., .F., .F.,
 ( 4, 2, 2, 4 ),
 ( 2.453269466693398698E-18, 0.001774887840461971235, 0.002662331760692956528, 0.003549775680923942470 ),
 .UNSPECIFIED. ) ;
#41779=AXIS2_PLACEMENT_3D ( 'NONE', #38609, #3385, #18681 ) ;
#41780=ORIENTED_EDGE ( 'NONE', *, *, #1005, .T. ) ;
#41783=DIRECTION ( 'NONE',  ( 1.000000000000000000, -0.000000000000000000, 0.000000000000000000 ) ) ;
#41785=CARTESIAN_POINT ( 'NONE',  ( -35.00000000000000000, 4.732539170486427693, -11.23004253107759176 ) ) ;
#41786=DIRECTION ( 'NONE',  ( 1.000000000000000000, 0.000000000000000000, 0.000000000000000000 ) ) ;
#41788=CARTESIAN_POINT ( 'NONE',  ( 9.575800908719084958, 13.45729701195361372, -1.072919909436246266 ) ) ;
#41792=EDGE_CURVE ( 'NONE', #55068, #18977, #49294, .T. ) ;
#41793=VERTEX_POINT ( 'NONE', #62753 ) ;
#41794=CARTESIAN_POINT ( 'NONE',  ( -35.00000000000000000, 8.366449238204365813, 9.621072037177025749 ) ) ;
#41798=VECTOR ( 'NONE', #30599, 1000.000000000000000 ) ;
#41799=CARTESIAN_POINT ( 'NONE',  ( 37.00000000000000711, 0.1414404973753909112, 12.74921544981110522 ) ) ;
#41801=DIRECTION ( 'NONE',  ( 1.000000000000000000, 0.000000000000000000, -0.000000000000000000 ) ) ;
#41805=CIRCLE ( 'NONE', #11006, 5.000000000000000888 ) ;
#41806=ORIENTED_EDGE ( 'NONE', *, *, #15964, .F. ) ;
#41807=EDGE_CURVE ( 'NONE', #44942, #9046, #51420, .T. ) ;
#41808=LINE ( 'NONE', #21539, #14174 ) ;
#41810=DIRECTION ( 'NONE',  ( 1.000000000000000000, 0.000000000000000000, 0.000000000000000000 ) ) ;
#41811=CARTESIAN_POINT ( 'NONE',  ( -35.00000000000000000, -5.015831474386382105, 10.62137734850266391 ) ) ;
#41814=DIRECTION ( 'NONE',  ( 1.000000000000000000, 0.000000000000000000, -0.000000000000000000 ) ) ;
#41815=EDGE_CURVE ( 'NONE', #20113, #44262, #33363, .T. ) ;
#41816=VERTEX_POINT ( 'NONE', #6271 ) ;
#41821=CYLINDRICAL_SURFACE ( 'NONE', #62508, 11.99999999999998579 ) ;
#41822=CIRCLE ( 'NONE', #17387, 5.000000000000000888 ) ;
#41826=ORIENTED_EDGE ( 'NONE', *, *, #13626, .T. ) ;
#41827=AXIS2_PLACEMENT_3D ( 'NONE', #44394, #24797, #54737 ) ;
#41829=ORIENTED_EDGE ( 'NONE', *, *, #15979, .F. ) ;
#41830=DIRECTION ( 'NONE',  ( 0.000000000000000000, 0.01356324068817998940, -0.9999080150203990547 ) ) ;
#41832=DIRECTION ( 'NONE',  ( -1.000000000000000000, 0.000000000000000000, -0.000000000000000000 ) ) ;
#41834=CARTESIAN_POINT ( 'NONE',  ( -8.109707593773686440, -2.369880750454201213, 11.76635280190479982 ) ) ;
#41835=AXIS2_PLACEMENT_3D ( 'NONE', #9391, #50973, #44994 ) ;
#41838=DIRECTION ( 'NONE',  ( 1.000000000000000000, 0.000000000000000000, 0.000000000000000000 ) ) ;
#41839=VERTEX_POINT ( 'NONE', #37154 ) ;
#41840=CARTESIAN_POINT ( 'NONE',  ( 35.00000000000000000, 4.705694406421931860E-17, -3.469127814946512892E-15 ) ) ;
#41842=FACE_OUTER_BOUND ( 'NONE', #25984, .T. ) ;
#41843=DIRECTION ( 'NONE',  ( 0.000000000000000000, -0.4698238015817237656, -0.8827602140260383257 ) ) ;
#41847=ORIENTED_EDGE ( 'NONE', *, *, #57607, .F. ) ;
#41849=EDGE_CURVE ( 'NONE', #43631, #15685, #65205, .T. ) ;
#41851=ORIENTED_EDGE ( 'NONE', *, *, #50688, .T. ) ;
#41853=ADVANCED_FACE ( 'NONE', ( #11248 ), #52794, .T. ) ;
#41854=CARTESIAN_POINT ( 'NONE',  ( 16.78263030916553689, 12.17295508002146320, 5.836879698929895888 ) ) ;
#41856=VERTEX_POINT ( 'NONE', #31207 ) ;
#41860=DIRECTION ( 'NONE',  ( -0.000000000000000000, -1.000000000000000000, -0.000000000000000000 ) ) ;
#41861=ORIENTED_EDGE ( 'NONE', *, *, #47374, .F. ) ;
#41862=VERTEX_POINT ( 'NONE', #51511 ) ;
#41864=ORIENTED_EDGE ( 'NONE', *, *, #28091, .T. ) ;
#41865=DIRECTION ( 'NONE',  ( -1.000000000000000000, 0.000000000000000000, -0.000000000000000000 ) ) ;
#41866=ORIENTED_EDGE ( 'NONE', *, *, #43343, .T. ) ;
#41867=CIRCLE ( 'NONE', #51434, 5.000000000000000888 ) ;
#41872=EDGE_CURVE ( 'NONE', #26911, #36952, #55673, .T. ) ;
#41874=CARTESIAN_POINT ( 'NONE',  ( 9.687175622948609899, 11.98570860552671391, -0.5854820436212360146 ) ) ;
#41875=DIRECTION ( 'NONE',  ( 1.000000000000000000, 0.000000000000000000, 0.000000000000000000 ) ) ;
#41876=ORIENTED_EDGE ( 'NONE', *, *, #13754, .F. ) ;
#41878=EDGE_CURVE ( 'NONE', #19477, #5474, #5958, .T. ) ;
#41879=ORIENTED_EDGE ( 'NONE', *, *, #37083, .F. ) ;
#41880=DIRECTION ( 'NONE',  ( 1.000000000000000000, -0.000000000000000000, 0.000000000000000000 ) ) ;
#41881=CARTESIAN_POINT ( 'NONE',  ( -3.438323251045651396, 11.96547819944141544, 6.261536211207373803 ) ) ;
#41882=EDGE_CURVE ( 'NONE', #18732, #34279, #1617, .T. ) ;
#41886=CARTESIAN_POINT ( 'NONE',  ( -35.00000000000000000, 0.000000000000000000, 0.000000000000000000 ) ) ;
#41887=VERTEX_POINT ( 'NONE', #21210 ) ;
#41889=CARTESIAN_POINT ( 'NONE',  ( -35.00000000000000000, -3.340853584269456888, -11.26103545359859304 ) ) ;
#41890=VERTEX_POINT ( 'NONE', #46818 ) ;
#41892=DIRECTION ( 'NONE',  ( -1.000000000000000000, 0.000000000000000000, 0.000000000000000000 ) ) ;
#41893=CARTESIAN_POINT ( 'NONE',  ( -35.00000000000000000, 0.000000000000000000, 0.000000000000000000 ) ) ;
#41895=CARTESIAN_POINT ( 'NONE',  ( -35.00000000000000000, 9.217970097227725645, 7.971186206369506699 ) ) ;
#41899=DIRECTION ( 'NONE',  ( 0.000000000000000000, 0.01356324068817998940, -0.9999080150203990547 ) ) ;
#41900=CARTESIAN_POINT ( 'NONE',  ( -10.90165637463012516, -7.508992741355087652, 9.360289953322833867 ) ) ;
#41901=DIRECTION ( 'NONE',  ( -1.000000000000000000, 0.000000000000000000, 0.000000000000000000 ) ) ;
#41903=EDGE_CURVE ( 'NONE', #38263, #50140, #65252, .T. ) ;
#41904=DIRECTION ( 'NONE',  ( -0.000000000000000000, -0.000000000000000000, -1.000000000000000000 ) ) ;
#41905=CIRCLE ( 'NONE', #13245, 5.000000000000000000 ) ;
#41908=CARTESIAN_POINT ( 'NONE',  ( 35.00000000000000000, -11.61175578952786758, -1.771820996347120092 ) ) ;
#41909=CARTESIAN_POINT ( 'NONE',  ( -21.17861794710831091, -11.44571409049744481, -3.604945070120774808 ) ) ;
#41911=ORIENTED_EDGE ( 'NONE', *, *, #2552, .F. ) ;
#41915=DIRECTION ( 'NONE',  ( 1.000000000000000000, 0.000000000000000000, 0.000000000000000000 ) ) ;
#41917=ORIENTED_EDGE ( 'NONE', *, *, #3587, .T. ) ;
#41918=VERTEX_POINT ( 'NONE', #57138 ) ;
#41919=ORIENTED_EDGE ( 'NONE', *, *, #7126, .F. ) ;
#41921=EDGE_CURVE ( 'NONE', #42603, #58929, #35482, .T. ) ;
#41922=AXIS2_PLACEMENT_3D ( 'NONE', #9400, #25055, #30028 ) ;
#41923=DIRECTION ( 'NONE',  ( 1.000000000000000000, -0.000000000000000000, 0.000000000000000000 ) ) ;
#41924=EDGE_LOOP ( 'NONE', ( #38154, #65455, #36568, #1949 ) ) ;
#41925=CYLINDRICAL_SURFACE ( 'NONE', #57048, 12.18649999999999878 ) ;
#41926=DIRECTION ( 'NONE',  ( 0.000000000000000000, -0.01356324068817998940, 0.9999080150203990547 ) ) ;
#41927=ORIENTED_EDGE ( 'NONE', *, *, #65265, .T. ) ;
#41928=( BOUNDED_CURVE ( )  B_SPLINE_CURVE ( 3, ( #61508, #56547, #60530, #10315 ),
 .UNSPECIFIED., .F., .F. ) 
 B_SPLINE_CURVE_WITH_KNOTS ( ( 4, 4 ),
 ( 0.6002665644134519418, 0.6265323918907089729 ),
 .UNSPECIFIED. ) 
 CURVE ( )  GEOMETRIC_REPRESENTATION_ITEM ( )  RATIONAL_B_SPLINE_CURVE ( ( 1.000000000000000000, 0.9999425096852141426, 0.9999425096852141426, 1.000000000000000000 ) ) 
 REPRESENTATION_ITEM ( '' )  );
#41929=LINE ( 'NONE', #16665, #40747 ) ;
#41931=FACE_OUTER_BOUND ( 'NONE', #3268, .T. ) ;
#41932=ORIENTED_EDGE ( 'NONE', *, *, #26617, .T. ) ;
#41933=CYLINDRICAL_SURFACE ( 'NONE', #38460, 5.000000000000000888 ) ;
#41939=CARTESIAN_POINT ( 'NONE',  ( 35.00000000000000000, 12.18632975068352664, 0.06441628369840225743 ) ) ;
#41941=EDGE_CURVE ( 'NONE', #47639, #34574, #26595, .T. ) ;
#41945=VERTEX_POINT ( 'NONE', #26869 ) ;
#41946=DIRECTION ( 'NONE',  ( 1.000000000000000000, 0.000000000000000000, 0.000000000000000000 ) ) ;
#41948=ORIENTED_EDGE ( 'NONE', *, *, #65060, .F. ) ;
#41950=EDGE_CURVE ( 'NONE', #57314, #54998, #39417, .T. ) ;
#41953=EDGE_LOOP ( 'NONE', ( #14243, #57810, #19366, #12437 ) ) ;
#41954=DIRECTION ( 'NONE',  ( 1.000000000000000000, 0.000000000000000000, -0.000000000000000000 ) ) ;
#41956=FACE_OUTER_BOUND ( 'NONE', #30104, .T. ) ;
#41959=EDGE_LOOP ( 'NONE', ( #15573, #16745, #9852, #38727 ) ) ;
#41960=DIRECTION ( 'NONE',  ( 0.000000000000000000, -0.01356324068817998940, 0.9999080150203990547 ) ) ;
#41961=ORIENTED_EDGE ( 'NONE', *, *, #46621, .F. ) ;
#41963=CARTESIAN_POINT ( 'NONE',  ( -37.00000000000000711, 11.86701198550360203, -2.772148766915989881 ) ) ;
#41965=LINE ( 'NONE', #17026, #9493 ) ;
#41967=ORIENTED_EDGE ( 'NONE', *, *, #14517, .F. ) ;
#41970=EDGE_CURVE ( 'NONE', #36702, #4408, #22540, .T. ) ;
#41972=EDGE_CURVE ( 'NONE', #8982, #15694, #41777, .T. ) ;
#41973=CARTESIAN_POINT ( 'NONE',  ( 29.20591975386996708, 10.31637300579003558, 8.717626168519132079 ) ) ;
#41974=DIRECTION ( 'NONE',  ( -1.000000000000000000, 0.000000000000000000, -0.000000000000000000 ) ) ;
#41975=EDGE_CURVE ( 'NONE', #34540, #1249, #48175, .T. ) ;
#41976=CARTESIAN_POINT ( 'NONE',  ( 35.00000000000000000, 4.705694406421931860E-17, -3.469127814946512892E-15 ) ) ;
#41978=DIRECTION ( 'NONE',  ( 1.000000000000000000, 0.000000000000000000, 0.000000000000000000 ) ) ;
#41979=PRODUCT_DEFINITION_FORMATION_WITH_SPECIFIED_SOURCE ( 'ANY', '', #54612, .NOT_KNOWN. ) ;
#41980=LINE ( 'NONE', #46986, #22979 ) ;
#41981=DIRECTION ( 'NONE',  ( -1.000000000000000000, 0.000000000000000000, 0.000000000000000000 ) ) ;
#41982=ORIENTED_EDGE ( 'NONE', *, *, #52708, .F. ) ;
#41984=DIRECTION ( 'NONE',  ( -1.000000000000000000, 0.000000000000000000, 0.000000000000000000 ) ) ;
#41985=AXIS2_PLACEMENT_3D ( 'NONE', #3967, #19900, #33879 ) ;
#41986=ORIENTED_EDGE ( 'NONE', *, *, #30332, .T. ) ;
#41989=VERTEX_POINT ( 'NONE', #13213 ) ;
#41991=VERTEX_POINT ( 'NONE', #33498 ) ;
#41992=CARTESIAN_POINT ( 'NONE',  ( -35.00000000000000000, -4.041347439435779343, -11.02904044024213270 ) ) ;
#41994=ORIENTED_EDGE ( 'NONE', *, *, #41457, .T. ) ;
#41995=AXIS2_PLACEMENT_3D ( 'NONE', #3863, #64022, #39072 ) ;
#41998=ORIENTED_EDGE ( 'NONE', *, *, #27172, .F. ) ;
#41999=DIRECTION ( 'NONE',  ( 0.000000000000000000, -0.01356324068817998940, 0.9999080150203990547 ) ) ;
#42001=CARTESIAN_POINT ( 'NONE',  ( 35.00000000000000000, 2.080187960898561172, -12.57916205664482234 ) ) ;
#42004=CYLINDRICAL_SURFACE ( 'NONE', #8683, 2.809571291727933851 ) ;
#42007=DIRECTION ( 'NONE',  ( 1.000000000000000000, 0.000000000000000000, 0.000000000000000000 ) ) ;
#42008=EDGE_LOOP ( 'NONE', ( #8352, #31773, #30568, #51601 ) ) ;
#42010=ORIENTED_EDGE ( 'NONE', *, *, #28898, .F. ) ;
#42011=CARTESIAN_POINT ( 'NONE',  ( -35.00000000000000000, -0.1652884326465054177, 12.18537902504609072 ) ) ;
#42014=CARTESIAN_POINT ( 'NONE',  ( 22.05006909623952183, -10.53419554220477217, -5.760554779199603459 ) ) ;
#42016=CARTESIAN_POINT ( 'NONE',  ( 35.00000000000000000, 10.80478261802181628, -5.636262487437359248 ) ) ;
#42017=VECTOR ( 'NONE', #17539, 1000.000000000000000 ) ;
#42019=CARTESIAN_POINT ( 'NONE',  ( 36.00000000000000711, -1.457575200925455672, 12.66641127287626745 ) ) ;
#42020=ADVANCED_FACE ( 'NONE', ( #45110 ), #61058, .T. ) ;
#42021=DIRECTION ( 'NONE',  ( 1.000000000000000000, 0.000000000000000000, 0.000000000000000000 ) ) ;
#42025=DIRECTION ( 'NONE',  ( 0.000000000000000000, -0.01356324068818000328, 0.9999080150203990547 ) ) ;
#42026=VERTEX_POINT ( 'NONE', #10493 ) ;
#42029=EDGE_CURVE ( 'NONE', #28743, #34193, #43997, .T. ) ;
#42030=ORIENTED_EDGE ( 'NONE', *, *, #14483, .T. ) ;
#42033=CARTESIAN_POINT ( 'NONE',  ( -37.00000000000000711, 12.17626345777664376, -0.4993900848166082374 ) ) ;
#42035=DIRECTION ( 'NONE',  ( 1.000000000000000000, 0.000000000000000000, 0.000000000000000000 ) ) ;
#42036=DIRECTION ( 'NONE',  ( 0.000000000000000000, -0.01356324068817998940, 0.9999080150203990547 ) ) ;
#42037=CYLINDRICAL_SURFACE ( 'NONE', #33375, 12.18650000000000055 ) ;
#42038=CIRCLE ( 'NONE', #54824, 5.000000000000000888 ) ;
#42039=ORIENTED_EDGE ( 'NONE', *, *, #36212, .T. ) ;
#42040=CARTESIAN_POINT ( 'NONE',  ( -27.78468958554971380, 25.00000000000000000, 8.565911087387465983 ) ) ;
#42041=CARTESIAN_POINT ( 'NONE',  ( -3.386646625484277529, -11.12986073946647991, 4.506218457162742830 ) ) ;
#42042=EDGE_CURVE ( 'NONE', #11684, #47167, #15322, .T. ) ;
#42043=CIRCLE ( 'NONE', #44050, 12.74999999999999822 ) ;
#42047=DIRECTION ( 'NONE',  ( 0.000000000000000000, 0.01356324068817992175, -0.9999080150203990547 ) ) ;
#42049=CARTESIAN_POINT ( 'NONE',  ( 35.00000000000000000, -11.73463472867578083, -3.287724142101374092 ) ) ;
#42050=ORIENTED_EDGE ( 'NONE', *, *, #44652, .T. ) ;
#42052=LINE ( 'NONE', #48050, #17663 ) ;
#42055=CARTESIAN_POINT ( 'NONE',  ( -26.56896637191177035, 10.48260233735502922, 5.841271018688308558 ) ) ;
#42056=DIRECTION ( 'NONE',  ( -1.000000000000000000, 0.000000000000000000, 0.000000000000000000 ) ) ;
#42058=DIRECTION ( 'NONE',  ( 1.000000000000000000, 0.000000000000000000, -0.000000000000000000 ) ) ;
#42059=DIRECTION ( 'NONE',  ( -0.000000000000000000, -0.000000000000000000, -1.000000000000000000 ) ) ;
#42061=ORIENTED_EDGE ( 'NONE', *, *, #47336, .T. ) ;
#42063=FACE_OUTER_BOUND ( 'NONE', #52192, .T. ) ;
#42064=DIRECTION ( 'NONE',  ( -1.000000000000000000, -0.000000000000000000, 0.000000000000000000 ) ) ;
#42066=CARTESIAN_POINT ( 'NONE',  ( -37.00000000000000711, 0.000000000000000000, 0.000000000000000000 ) ) ;
#42067=EDGE_CURVE ( 'NONE', #62829, #33917, #45084, .T. ) ;
#42069=CARTESIAN_POINT ( 'NONE',  ( -35.00000000000000000, 11.73808581813437968, -0.4353888892048790038 ) ) ;
#42071=DIRECTION ( 'NONE',  ( -0.000000000000000000, -1.000000000000000000, -0.000000000000000000 ) ) ;
#42072=EDGE_CURVE ( 'NONE', #36819, #17286, #52511, .T. ) ;
#42073=CARTESIAN_POINT ( 'NONE',  ( 35.00000000000000000, -11.35427606708803161, 4.426194442447358490 ) ) ;
#42080=EDGE_LOOP ( 'NONE', ( #6635, #54138, #26664, #48458 ) ) ;
#42081=ORIENTED_EDGE ( 'NONE', *, *, #47823, .F. ) ;
#42082=CARTESIAN_POINT ( 'NONE',  ( 23.20059726473823503, 3.175887350242510898, -11.57493929936777377 ) ) ;
#42085=CARTESIAN_POINT ( 'NONE',  ( -35.00000000000000000, 11.68758509253248334, -1.171570255487489609 ) ) ;
#42087=DIRECTION ( 'NONE',  ( 0.000000000000000000, 0.01356324068817991481, -0.9999080150203990547 ) ) ;
#42088=VERTEX_POINT ( 'NONE', #4559 ) ;
#42089=CARTESIAN_POINT ( 'NONE',  ( -25.54417658651491863, -4.240019242199836391, 11.22596262356930197 ) ) ;
#42092=ORIENTED_EDGE ( 'NONE', *, *, #14672, .T. ) ;
#42094=EDGE_CURVE ( 'NONE', #56806, #45280, #20650, .T. ) ;
#42096=CYLINDRICAL_SURFACE ( 'NONE', #10431, 12.18649999999999878 ) ;
#42098=CARTESIAN_POINT ( 'NONE',  ( 8.958004941509509322, 4.004350268857352013, 12.89476050860881173 ) ) ;
#42099=ADVANCED_FACE ( 'NONE', ( #39785 ), #9846, .T. ) ;
#42104=CYLINDRICAL_SURFACE ( 'NONE', #39029, 5.000000000000001776 ) ;
#42105=VERTEX_POINT ( 'NONE', #218 ) ;
#42106=DIRECTION ( 'NONE',  ( 1.000000000000000000, 0.000000000000000000, 0.000000000000000000 ) ) ;
#42107=CARTESIAN_POINT ( 'NONE',  ( -37.00000000000000711, 11.98254675519231860, -2.220215194441768514 ) ) ;
#42108=CARTESIAN_POINT ( 'NONE',  ( -37.00000000000000711, 12.68495603654572079, 1.286231064351357256 ) ) ;
#42109=DIRECTION ( 'NONE',  ( 0.000000000000000000, -0.01356324068817991828, 0.9999080150203990547 ) ) ;
#42113=EDGE_CURVE ( 'NONE', #27370, #31676, #34768, .T. ) ;
#42114=ORIENTED_EDGE ( 'NONE', *, *, #40843, .T. ) ;
#42119=( BOUNDED_CURVE ( )  B_SPLINE_CURVE ( 3, ( #49852, #4301, #24575, #29879 ),
 .UNSPECIFIED., .F., .F. ) 
 B_SPLINE_CURVE_WITH_KNOTS ( ( 4, 4 ),
 ( 5.652045941182875843, 5.686890868700008816 ),
 .UNSPECIFIED. ) 
 CURVE ( )  GEOMETRIC_REPRESENTATION_ITEM ( )  RATIONAL_B_SPLINE_CURVE ( ( 1.000000000000000000, 0.9998988218115538729, 0.9998988218115538729, 1.000000000000000000 ) ) 
 REPRESENTATION_ITEM ( '' )  );
#42120=ORIENTED_EDGE ( 'NONE', *, *, #41598, .T. ) ;
#42125=ORIENTED_EDGE ( 'NONE', *, *, #29208, .T. ) ;
#42126=CYLINDRICAL_SURFACE ( 'NONE', #20786, 12.75000000000000178 ) ;
#42127=LINE ( 'NONE', #20878, #25779 ) ;
#42131=CARTESIAN_POINT ( 'NONE',  ( -36.00000000000000711, 4.074242145636004508, 12.08151691381191917 ) ) ;
#42132=FACE_OUTER_BOUND ( 'NONE', #3716, .T. ) ;
#42133=VERTEX_POINT ( 'NONE', #5544 ) ;
#42135=VERTEX_POINT ( 'NONE', #15804 ) ;
#42136=DIRECTION ( 'NONE',  ( 0.000000000000000000, 0.01356324068817998940, -0.9999080150203990547 ) ) ;
#42137=CARTESIAN_POINT ( 'NONE',  ( -35.00000000000000000, -9.040300684349640292, -7.499679039484155041 ) ) ;
#42140=CARTESIAN_POINT ( 'NONE',  ( -6.407494522312451757, -1.624111497457272790, 11.88968263856500940 ) ) ;
#42142=ORIENTED_EDGE ( 'NONE', *, *, #57044, .T. ) ;
#42145=EDGE_CURVE ( 'NONE', #44513, #23007, #29144, .T. ) ;
#42146=CARTESIAN_POINT ( 'NONE',  ( 1.577070743587938306, 1.421807588298878322, 11.92044867579712886 ) ) ;
#42147=CARTESIAN_POINT ( 'NONE',  ( 0.2851083653049504285, -0.4107471485392698018, 11.99296822225285730 ) ) ;
#42148=CARTESIAN_POINT ( 'NONE',  ( 21.90174657591892071, -13.47998113580522528, -0.7349207973210680755 ) ) ;
#42149=DIRECTION ( 'NONE',  ( 0.000000000000000000, -0.9999080150203990547, -0.01356324068816951688 ) ) ;
#42150=DIRECTION ( 'NONE',  ( -1.000000000000000000, 0.000000000000000000, 0.000000000000000000 ) ) ;
#42152=DIRECTION ( 'NONE',  ( -1.000000000000000000, 0.000000000000000000, -0.000000000000000000 ) ) ;
#42153=VERTEX_POINT ( 'NONE', #61692 ) ;
#42160=ADVANCED_FACE ( 'NONE', ( #31755 ), #31117, .T. ) ;
#42165=DIRECTION ( 'NONE',  ( -1.000000000000000000, -0.000000000000000000, -0.000000000000000000 ) ) ;
#42169=CARTESIAN_POINT ( 'NONE',  ( -17.19056858472900728, 2.658600115333384917, -11.70257571668042296 ) ) ;
#42170=ORIENTED_EDGE ( 'NONE', *, *, #12140, .F. ) ;
#42171=EDGE_CURVE ( 'NONE', #12997, #34948, #63116, .T. ) ;
#42172=VERTEX_POINT ( 'NONE', #16154 ) ;
#42174=ORIENTED_EDGE ( 'NONE', *, *, #63248, .F. ) ;
#42177=CARTESIAN_POINT ( 'NONE',  ( -37.00000000000000711, -5.391785509270885512, -10.43555801961481677 ) ) ;
#42178=DIRECTION ( 'NONE',  ( -1.000000000000000000, 0.000000000000000000, 0.000000000000000000 ) ) ;
#42180=FACE_OUTER_BOUND ( 'NONE', #37935, .T. ) ;
#42183=CARTESIAN_POINT ( 'NONE',  ( -35.00000000000000000, -7.110831038798204773, -9.896810808925470937 ) ) ;
#42184=ORIENTED_EDGE ( 'NONE', *, *, #52480, .T. ) ;
#42185=CARTESIAN_POINT ( 'NONE',  ( -35.00000000000000000, 7.474872387601008583, 9.060822531526074641 ) ) ;
#42190=CARTESIAN_POINT ( 'NONE',  ( 35.00000000000000000, -4.983891302653661093, -11.73555825188274504 ) ) ;
#42191=ADVANCED_FACE ( 'NONE', ( #41082 ), #61360, .T. ) ;
#42192=VECTOR ( 'NONE', #32284, 1000.000000000000000 ) ;
#42193=ORIENTED_EDGE ( 'NONE', *, *, #21455, .T. ) ;
#42197=DIRECTION ( 'NONE',  ( 0.000000000000000000, -0.01356324068817991828, 0.9999080150203990547 ) ) ;
#42199=FACE_OUTER_BOUND ( 'NONE', #35870, .T. ) ;
#42201=EDGE_LOOP ( 'NONE', ( #21560, #25605, #14509, #58583 ) ) ;
#42202=CARTESIAN_POINT ( 'NONE',  ( 35.00000000000000000, -8.766823244861932096, 7.817610399097601359 ) ) ;
#42205=AXIS2_PLACEMENT_3D ( 'NONE', #14462, #20123, #4852 ) ;
#42206=CARTESIAN_POINT ( 'NONE',  ( -3.649648704207571814, 12.48837185217044166, 5.141182941002472973 ) ) ;
#42207=B_SPLINE_CURVE_WITH_KNOTS ( 'NONE', 3,
 ( #44820, #10224, #55460, #45810, #25193, #49821, #30502, #50799, #39834, #9550, #34818, #60439, #5252, #35803, #35150, #19570, #25518, #54817, #45466, #15212, #65734, #20203, #24881, #40480, #60777, #64758 ),
 .UNSPECIFIED., .F., .F.,
 ( 4, 2, 2, 2, 2, 2, 2, 2, 2, 2, 2, 2, 4 ),
 ( 3.004629197474318463E-18, 0.001181670535257466504, 0.001772505802886197371, 0.002363341070514927804, 0.003545011605772387803, 0.004726682141029846934, 0.005317517408658578235, 0.005908352676287307800, 0.007090023211544771269, 0.007680858479173503436, 0.008271693746802234737, 0.008862529014430967772, 0.009453364282059699072 ),
 .UNSPECIFIED. ) ;
#42208=EDGE_CURVE ( 'NONE', #20627, #27642, #4075, .T. ) ;
#42210=CARTESIAN_POINT ( 'NONE',  ( -37.00000000000000711, 0.000000000000000000, 0.000000000000000000 ) ) ;
#42214=ORIENTED_EDGE ( 'NONE', *, *, #17491, .F. ) ;
#42216=ORIENTED_EDGE ( 'NONE', *, *, #65428, .T. ) ;
#42217=CARTESIAN_POINT ( 'NONE',  ( -37.00000000000000711, 8.573591947375437172, -8.029056188533592930 ) ) ;
#42218=LINE ( 'NONE', #3016, #35338 ) ;
#42219=CARTESIAN_POINT ( 'NONE',  ( -29.68541646480307250, -1.792450633335325616, 13.38582821403480771 ) ) ;
#42220=FACE_OUTER_BOUND ( 'NONE', #17388, .T. ) ;
#42223=ORIENTED_EDGE ( 'NONE', *, *, #12115, .T. ) ;
#42224=ORIENTED_EDGE ( 'NONE', *, *, #56280, .F. ) ;
#42225=CYLINDRICAL_SURFACE ( 'NONE', #48273, 4.999999999999999112 ) ;
#42226=CIRCLE ( 'NONE', #12479, 12.75000000000000178 ) ;
#42227=DIRECTION ( 'NONE',  ( -1.000000000000000000, -0.000000000000000000, 0.000000000000000000 ) ) ;
#42231=CYLINDRICAL_SURFACE ( 'NONE', #27883, 5.000000000000000000 ) ;
#42232=AXIS2_PLACEMENT_3D ( 'NONE', #12502, #63699, #53757 ) ;
#42233=ORIENTED_EDGE ( 'NONE', *, *, #8004, .F. ) ;
#42238=CIRCLE ( 'NONE', #18924, 4.999999999999999112 ) ;
#42242=DIRECTION ( 'NONE',  ( 0.000000000000000000, 0.01356324068817992175, -0.9999080150203990547 ) ) ;
#42246=LINE ( 'NONE', #41939, #30445 ) ;
#42247=DIRECTION ( 'NONE',  ( 0.000000000000000000, -0.01356324068817992175, 0.9999080150203990547 ) ) ;
#42248=CARTESIAN_POINT ( 'NONE',  ( 24.90079489126681977, -10.54408982692481977, -8.432554294912243620 ) ) ;
#42249=DIRECTION ( 'NONE',  ( 0.000000000000000000, 0.01356324068818000848, -0.9999080150203990547 ) ) ;
#42250=DIRECTION ( 'NONE',  ( 0.000000000000000000, 0.01356324068817998940, -0.9999080150203990547 ) ) ;
#42254=ORIENTED_EDGE ( 'NONE', *, *, #58754, .F. ) ;
#42259=CARTESIAN_POINT ( 'NONE',  ( 22.61491127797214062, 25.00000000000000000, 9.376349503825034404 ) ) ;
#42260=DIRECTION ( 'NONE',  ( -1.000000000000000000, 0.000000000000000000, 0.000000000000000000 ) ) ;
#42262=ORIENTED_EDGE ( 'NONE', *, *, #18101, .T. ) ;
#42263=EDGE_LOOP ( 'NONE', ( #36290, #28717, #55261, #45030 ) ) ;
#42265=AXIS2_PLACEMENT_3D ( 'NONE', #58404, #47448, #62707 ) ;
#42268=CARTESIAN_POINT ( 'NONE',  ( 35.00000000000000000, 4.705694406421931860E-17, -3.469127814946512892E-15 ) ) ;
#42269=CARTESIAN_POINT ( 'NONE',  ( -35.00000000000000000, -2.968224442958318665, -11.81949347079750012 ) ) ;
#42270=FACE_OUTER_BOUND ( 'NONE', #15463, .T. ) ;
#42274=AXIS2_PLACEMENT_3D ( 'NONE', #50481, #4924, #64749 ) ;
#42275=EDGE_CURVE ( 'NONE', #3924, #43734, #21301, .T. ) ;
#42276=AXIS2_PLACEMENT_3D ( 'NONE', #9447, #15104, #45694 ) ;
#42278=DIRECTION ( 'NONE',  ( 0.000000000000000000, 0.9718671068226466536, -0.2355298848897482422 ) ) ;
#42279=CARTESIAN_POINT ( 'NONE',  ( 37.00000000000000711, 12.18632975068352664, 0.06441628369840225743 ) ) ;
#42280=AXIS2_PLACEMENT_3D ( 'NONE', #59230, #20289, #19317 ) ;
#42283=LINE ( 'NONE', #58954, #34301 ) ;
#42284=AXIS2_PLACEMENT_3D ( 'NONE', #38865, #38530, #8593 ) ;
#42285=ADVANCED_FACE ( 'NONE', ( #53380 ), #7470, .T. ) ;
#42287=CARTESIAN_POINT ( 'NONE',  ( 35.00000000000000000, 1.039216533672905785, -11.70009620280412221 ) ) ;
#42288=CARTESIAN_POINT ( 'NONE',  ( 3.711556079772022176, -10.52777116167494675, 8.451878016623856738 ) ) ;
#42289=( BOUNDED_CURVE ( )  B_SPLINE_CURVE ( 3, ( #23549, #24510, #19544, #33826 ),
 .UNSPECIFIED., .F., .F. ) 
 B_SPLINE_CURVE_WITH_KNOTS ( ( 4, 4 ),
 ( 3.747275043436211650, 3.808054268073822524 ),
 .UNSPECIFIED. ) 
 CURVE ( )  GEOMETRIC_REPRESENTATION_ITEM ( )  RATIONAL_B_SPLINE_CURVE ( ( 1.000000000000000000, 0.9996921808454459768, 0.9996921808454459768, 1.000000000000000000 ) ) 
 REPRESENTATION_ITEM ( '' )  );
#42290=ORIENTED_EDGE ( 'NONE', *, *, #44484, .T. ) ;
#42295=CARTESIAN_POINT ( 'NONE',  ( -35.00000000000000000, 7.718225330433806874, 9.430788938294076829 ) ) ;
#42298=LINE ( 'NONE', #17053, #43377 ) ;
#42299=VERTEX_POINT ( 'NONE', #43370 ) ;
#42300=VERTEX_POINT ( 'NONE', #39049 ) ;
#42301=DIRECTION ( 'NONE',  ( 1.000000000000000000, 0.000000000000000000, 0.000000000000000000 ) ) ;
#42302=CIRCLE ( 'NONE', #3104, 5.000000000000000000 ) ;
#42304=EDGE_LOOP ( 'NONE', ( #1667, #13739, #58819, #43372 ) ) ;
#42305=FACE_OUTER_BOUND ( 'NONE', #26379, .T. ) ;
#42307=CYLINDRICAL_SURFACE ( 'NONE', #55652, 4.999999999999999112 ) ;
#42312=EDGE_CURVE ( 'NONE', #12370, #1280, #18123, .T. ) ;
#42315=CARTESIAN_POINT ( 'NONE',  ( -25.60894296954852223, 10.48177738153426830, 5.844539321404759846 ) ) ;
#42316=VERTEX_POINT ( 'NONE', #23434 ) ;
#42318=VERTEX_POINT ( 'NONE', #32414 ) ;
#42320=ORIENTED_EDGE ( 'NONE', *, *, #2793, .F. ) ;
#42321=CARTESIAN_POINT ( 'NONE',  ( 21.46003464439880659, -11.46841712088275322, -3.538095200798918594 ) ) ;
#42322=CARTESIAN_POINT ( 'NONE',  ( -35.00000000000000000, 10.43555801961483098, -5.391785509270847321 ) ) ;
#42323=CIRCLE ( 'NONE', #49758, 4.999999999999999112 ) ;
#42324=CARTESIAN_POINT ( 'NONE',  ( 35.00000000000000000, -11.16627499335657703, -3.645068577059991988 ) ) ;
#42325=VERTEX_POINT ( 'NONE', #13129 ) ;
#42327=CARTESIAN_POINT ( 'NONE',  ( 35.00000000000000000, 10.75351884295727345, -4.725891942574794058 ) ) ;
#42328=LINE ( 'NONE', #28064, #24650 ) ;
#42329=EDGE_CURVE ( 'NONE', #33526, #57232, #52069, .T. ) ;
#42330=ORIENTED_EDGE ( 'NONE', *, *, #53517, .T. ) ;
#42331=CIRCLE ( 'NONE', #9397, 12.18649999999999878 ) ;
#42335=EDGE_CURVE ( 'NONE', #42786, #24439, #15970, .T. ) ;
#42338=DIRECTION ( 'NONE',  ( -1.000000000000000000, 0.000000000000000000, 0.000000000000000000 ) ) ;
#42341=CARTESIAN_POINT ( 'NONE',  ( 35.00000000000000000, -1.903127969211267700, -11.59095880812007628 ) ) ;
#42343=FACE_OUTER_BOUND ( 'NONE', #9223, .T. ) ;
#42345=VERTEX_POINT ( 'NONE', #59033 ) ;
#42347=EDGE_CURVE ( 'NONE', #21730, #46798, #55207, .T. ) ;
#42349=EDGE_CURVE ( 'NONE', #44279, #2026, #17033, .T. ) ;
#42350=DIRECTION ( 'NONE',  ( 1.000000000000000000, -0.000000000000000000, 0.000000000000000000 ) ) ;
#42351=CIRCLE ( 'NONE', #46609, 12.18650000000000233 ) ;
#42352=CARTESIAN_POINT ( 'NONE',  ( -47.00000000000000711, 0.000000000000000000, 0.000000000000000000 ) ) ;
#42355=CARTESIAN_POINT ( 'NONE',  ( 11.12233887262441279, 0.3490535524848530358, -11.99560895363750923 ) ) ;
#42357=DIRECTION ( 'NONE',  ( 0.000000000000000000, 0.9970832820307041766, 0.07632122047556143263 ) ) ;
#42359=CARTESIAN_POINT ( 'NONE',  ( 35.00000000000000000, 1.591260454995240714, -12.08216339958901564 ) ) ;
#42360=ADVANCED_FACE ( 'NONE', ( #60642 ), #59673, .T. ) ;
#42362=CIRCLE ( 'NONE', #60428, 5.000000000000000888 ) ;
#42363=ADVANCED_FACE ( 'NONE', ( #20411 ), #29397, .T. ) ;
#42364=CARTESIAN_POINT ( 'NONE',  ( -36.00000000000000711, -6.950793414699719008, -10.68873102412850074 ) ) ;
#42365=CARTESIAN_POINT ( 'NONE',  ( 35.00000000000000000, 4.705694406421931860E-17, -3.469127814946512892E-15 ) ) ;
#42366=AXIS2_PLACEMENT_3D ( 'NONE', #3005, #18295, #63813 ) ;
#42367=VERTEX_POINT ( 'NONE', #4481 ) ;
#42368=DIRECTION ( 'NONE',  ( 0.000000000000000000, 0.01356324068817998940, -0.9999080150203990547 ) ) ;
#42369=CARTESIAN_POINT ( 'NONE',  ( -35.00000000000000000, 0.000000000000000000, 0.000000000000000000 ) ) ;
#42370=LINE ( 'NONE', #57715, #59716 ) ;
#42372=ORIENTED_EDGE ( 'NONE', *, *, #4121, .F. ) ;
#42373=CARTESIAN_POINT ( 'NONE',  ( -37.00000000000000711, 0.000000000000000000, 0.000000000000000000 ) ) ;
#42376=CIRCLE ( 'NONE', #53038, 12.74999999999999822 ) ;
#42377=CARTESIAN_POINT ( 'NONE',  ( -35.00000000000000000, 11.29812557209476864, 3.213188559034282132 ) ) ;
#42378=VERTEX_POINT ( 'NONE', #45674 ) ;
#42379=DIRECTION ( 'NONE',  ( -1.000000000000000000, -0.000000000000000000, -0.000000000000000000 ) ) ;
#42381=VERTEX_POINT ( 'NONE', #40345 ) ;
#42382=CARTESIAN_POINT ( 'NONE',  ( -35.00000000000000000, 6.102719229070827645, -10.54834585426213422 ) ) ;
#42383=DIRECTION ( 'NONE',  ( 1.000000000000000000, -0.000000000000000000, 0.000000000000000000 ) ) ;
#42386=FACE_OUTER_BOUND ( 'NONE', #64661, .T. ) ;
#42387=EDGE_CURVE ( 'NONE', #11516, #48650, #49396, .T. ) ;
#42388=DIRECTION ( 'NONE',  ( 0.000000000000000000, 0.5472293298355273006, -0.8369827122275343978 ) ) ;
#42389=DIRECTION ( 'NONE',  ( -1.000000000000000000, 0.000000000000000000, 0.000000000000000000 ) ) ;
#42392=EDGE_CURVE ( 'NONE', #49156, #40383, #35016, .T. ) ;
#42393=ORIENTED_EDGE ( 'NONE', *, *, #49302, .T. ) ;
#42394=DIRECTION ( 'NONE',  ( 0.000000000000000000, 0.1387779952735818945, -0.9903235168508549569 ) ) ;
#42395=EDGE_LOOP ( 'NONE', ( #19472, #65193, #49375, #43832 ) ) ;
#42400=AXIS2_PLACEMENT_3D ( 'NONE', #21876, #38120, #2245 ) ;
#42401=DIRECTION ( 'NONE',  ( -1.000000000000000000, -0.000000000000000000, -0.000000000000000000 ) ) ;
#42402=EDGE_CURVE ( 'NONE', #43073, #32242, #15083, .T. ) ;
#42404=VERTEX_POINT ( 'NONE', #25079 ) ;
#42405=CARTESIAN_POINT ( 'NONE',  ( -24.89073217517900360, -5.758728772039412469, 10.56290472577202522 ) ) ;
#42407=CARTESIAN_POINT ( 'NONE',  ( 0.2851083653049530375, -0.4107471485392680810, -13.49374991542258151 ) ) ;
#42409=ORIENTED_EDGE ( 'NONE', *, *, #28085, .T. ) ;
#42410=ADVANCED_FACE ( 'NONE', ( #44354 ), #19101, .T. ) ;
#42412=EDGE_LOOP ( 'NONE', ( #63143, #53487, #12307, #23695, #46815, #48897 ) ) ;
#42413=DIRECTION ( 'NONE',  ( 1.000000000000000000, 0.000000000000000000, 0.000000000000000000 ) ) ;
#42414=CARTESIAN_POINT ( 'NONE',  ( 12.49336350054390365, 0.1658493928153598473, 11.99999999999999645 ) ) ;
#42415=FACE_OUTER_BOUND ( 'NONE', #12740, .T. ) ;
#42416=AXIS2_PLACEMENT_3D ( 'NONE', #29898, #30236, #50851 ) ;
#42417=DIRECTION ( 'NONE',  ( 1.000000000000000000, 0.000000000000000000, 0.000000000000000000 ) ) ;
#42418=DIRECTION ( 'NONE',  ( 1.000000000000000000, -0.000000000000000000, -0.000000000000000000 ) ) ;
#42419=CARTESIAN_POINT ( 'NONE',  ( 35.00000000000000000, 4.705694406421931860E-17, -3.469127814946512892E-15 ) ) ;
#42423=ORIENTED_EDGE ( 'NONE', *, *, #29284, .F. ) ;
#42424=FACE_OUTER_BOUND ( 'NONE', #8871, .T. ) ;
#42425=CARTESIAN_POINT ( 'NONE',  ( -9.129631415690074192, -12.73028175706349430, -4.506864653171657409 ) ) ;
#42430=ORIENTED_EDGE ( 'NONE', *, *, #16819, .T. ) ;
#42431=EDGE_CURVE ( 'NONE', #16656, #57717, #4463, .T. ) ;
#42433=CARTESIAN_POINT ( 'NONE',  ( -2.952869152607107139, 12.96714474214482138, 3.755417052241487585 ) ) ;
#42434=EDGE_CURVE ( 'NONE', #57088, #61909, #45247, .T. ) ;
#42435=VERTEX_POINT ( 'NONE', #32571 ) ;
#42437=DIRECTION ( 'NONE',  ( -1.000000000000000000, -0.000000000000000000, 0.000000000000000000 ) ) ;
#42445=LINE ( 'NONE', #57793, #62472 ) ;
#42446=AXIS2_PLACEMENT_3D ( 'NONE', #42210, #16963, #7300 ) ;
#42447=CIRCLE ( 'NONE', #13788, 5.000000000000000888 ) ;
#42448=CARTESIAN_POINT ( 'NONE',  ( -35.00000000000000000, 0.000000000000000000, 0.000000000000000000 ) ) ;
#42449=CARTESIAN_POINT ( 'NONE',  ( -35.00000000000000000, 0.000000000000000000, 0.000000000000000000 ) ) ;
#42452=ORIENTED_EDGE ( 'NONE', *, *, #14596, .T. ) ;
#42453=CARTESIAN_POINT ( 'NONE',  ( -37.00000000000000711, -1.771820996347237331, 11.61175578952785692 ) ) ;
#42455=CARTESIAN_POINT ( 'NONE',  ( -35.00000000000000000, 0.000000000000000000, 0.000000000000000000 ) ) ;
#42456=EDGE_CURVE ( 'NONE', #5624, #35473, #36, .T. ) ;
#42460=AXIS2_PLACEMENT_3D ( 'NONE', #34148, #19850, #29184 ) ;
#42463=VERTEX_POINT ( 'NONE', #31369 ) ;
#42464=CARTESIAN_POINT ( 'NONE',  ( -35.00000000000000000, 0.000000000000000000, 0.000000000000000000 ) ) ;
#42466=AXIS2_PLACEMENT_3D ( 'NONE', #44769, #3604, #34774 ) ;
#42467=CARTESIAN_POINT ( 'NONE',  ( 3.243709820962341617, 4.721130720727682473, 11.04021256742971069 ) ) ;
#42470=CARTESIAN_POINT ( 'NONE',  ( 35.00000000000000000, 4.705694406421931860E-17, -3.469127814946512892E-15 ) ) ;
#42471=DIRECTION ( 'NONE',  ( -1.000000000000000000, 0.000000000000000000, -0.000000000000000000 ) ) ;
#42473=CARTESIAN_POINT ( 'NONE',  ( -37.00000000000000711, 10.80631716521666874, 4.603882218679588689 ) ) ;
#42474=ORIENTED_EDGE ( 'NONE', *, *, #25581, .T. ) ;
#42475=ORIENTED_EDGE ( 'NONE', *, *, #63768, .F. ) ;
#42477=AXIS2_PLACEMENT_3D ( 'NONE', #59066, #13474, #33757 ) ;
#42478=ORIENTED_EDGE ( 'NONE', *, *, #23791, .T. ) ;
#42480=EDGE_CURVE ( 'NONE', #33417, #49413, #45705, .T. ) ;
#42481=CARTESIAN_POINT ( 'NONE',  ( 24.16730227909621220, -10.72488973065076223, -8.203994665790906637 ) ) ;
#42482=CYLINDRICAL_SURFACE ( 'NONE', #64015, 4.999999999999999112 ) ;
#42484=CARTESIAN_POINT ( 'NONE',  ( -35.00000000000000000, 0.000000000000000000, 0.000000000000000000 ) ) ;
#42486=AXIS2_PLACEMENT_3D ( 'NONE', #50300, #43643, #59607 ) ;
#42490=ORIENTED_EDGE ( 'NONE', *, *, #17201, .F. ) ;
#42491=EDGE_LOOP ( 'NONE', ( #56482, #33681, #49079, #14578 ) ) ;
#42492=EDGE_CURVE ( 'NONE', #58003, #14898, #39291, .T. ) ;
#42493=VERTEX_POINT ( 'NONE', #477 ) ;
#42494=ORIENTED_EDGE ( 'NONE', *, *, #57016, .F. ) ;
#42495=CARTESIAN_POINT ( 'NONE',  ( 25.05309951391468459, -10.77522019223763827, -8.132934882857099979 ) ) ;
#42496=ORIENTED_EDGE ( 'NONE', *, *, #19598, .T. ) ;
#42497=EDGE_LOOP ( 'NONE', ( #41911, #41268, #29276, #696 ) ) ;
#42498=PLANE ( 'NONE',  #32000 ) ;
#42500=AXIS2_PLACEMENT_3D ( 'NONE', #42449, #37817, #62748 ) ;
#42502=CIRCLE ( 'NONE', #51034, 5.000000000000000888 ) ;
#42503=CIRCLE ( 'NONE', #22338, 12.75000000000000178 ) ;
#42505=CARTESIAN_POINT ( 'NONE',  ( -35.00000000000000000, 3.645068577060182946, -11.16627499335651130 ) ) ;
#42506=CARTESIAN_POINT ( 'NONE',  ( -37.00000000000000711, 12.05416472667165806, 1.791059740004466994 ) ) ;
#42507=ORIENTED_EDGE ( 'NONE', *, *, #35778, .F. ) ;
#42509=CARTESIAN_POINT ( 'NONE',  ( -35.00000000000000000, 0.4993900848167411310, 12.17626345777664021 ) ) ;
#42511=DIRECTION ( 'NONE',  ( -1.000000000000000000, 0.000000000000000000, 0.000000000000000000 ) ) ;
#42517=DIRECTION ( 'NONE',  ( 0.000000000000000000, 0.1740410799127543318, 0.9847383929261630531 ) ) ;
#42524=CARTESIAN_POINT ( 'NONE',  ( 9.575800908719084958, -13.45729701195359240, -1.072919909436246266 ) ) ;
#42528=DIRECTION ( 'NONE',  ( -1.000000000000000000, 0.000000000000000000, 0.000000000000000000 ) ) ;
#42529=DIRECTION ( 'NONE',  ( 0.000000000000000000, 0.3218879778915904044, -0.9467777615094594701 ) ) ;
#42530=CIRCLE ( 'NONE', #2217, 5.000000000000000000 ) ;
#42532=DIRECTION ( 'NONE',  ( 0.000000000000000000, -0.01356324068817999114, 0.9999080150203989437 ) ) ;
#42533=DIRECTION ( 'NONE',  ( -1.000000000000000000, 0.000000000000000000, -0.000000000000000000 ) ) ;
#42534=VERTEX_POINT ( 'NONE', #53559 ) ;
#42536=CIRCLE ( 'NONE', #27650, 5.000000000000001776 ) ;
#42537=FACE_OUTER_BOUND ( 'NONE', #59493, .T. ) ;
#42538=ADVANCED_FACE ( 'NONE', ( #24250 ), #8639, .T. ) ;
#42539=EDGE_CURVE ( 'NONE', #49728, #57334, #10659, .T. ) ;
#42540=AXIS2_PLACEMENT_3D ( 'NONE', #60378, #55399, #45747 ) ;
#42541=AXIS2_PLACEMENT_3D ( 'NONE', #59480, #34830, #3962 ) ;
#42543=ORIENTED_EDGE ( 'NONE', *, *, #54505, .F. ) ;
#42546=VECTOR ( 'NONE', #33034, 1000.000000000000000 ) ;
#42547=LINE ( 'NONE', #58890, #40665 ) ;
#42549=DIRECTION ( 'NONE',  ( 1.000000000000000000, 0.000000000000000000, 0.000000000000000000 ) ) ;
#42550=ORIENTED_EDGE ( 'NONE', *, *, #52846, .T. ) ;
#42551=ORIENTED_EDGE ( 'NONE', *, *, #39453, .T. ) ;
#42552=ORIENTED_EDGE ( 'NONE', *, *, #50573, .T. ) ;
#42554=AXIS2_PLACEMENT_3D ( 'NONE', #21590, #16596, #57164 ) ;
#42556=AXIS2_PLACEMENT_3D ( 'NONE', #7353, #27636, #63219 ) ;
#42557=CARTESIAN_POINT ( 'NONE',  ( -27.45775109278350712, 13.35262336282554152, -1.989333891161978674 ) ) ;
#42558=ORIENTED_EDGE ( 'NONE', *, *, #64051, .T. ) ;
#42559=CYLINDRICAL_SURFACE ( 'NONE', #32566, 12.18650000000000055 ) ;
#42564=CARTESIAN_POINT ( 'NONE',  ( 35.00000000000000000, 1.030638227056565048, -12.14284015767850278 ) ) ;
#42565=CARTESIAN_POINT ( 'NONE',  ( 35.00000000000000000, -11.68758509253247091, 1.171570255487570655 ) ) ;
#42566=ORIENTED_EDGE ( 'NONE', *, *, #7281, .F. ) ;
#42570=VERTEX_POINT ( 'NONE', #63491 ) ;
#42572=CIRCLE ( 'NONE', #55366, 5.000000000000000000 ) ;
#42573=CARTESIAN_POINT ( 'NONE',  ( -35.00000000000000000, 0.000000000000000000, 0.000000000000000000 ) ) ;
#42574=DIRECTION ( 'NONE',  ( 0.000000000000000000, 0.01356324068817998940, -0.9999080150203990547 ) ) ;
#42576=LINE ( 'NONE', #1726, #58092 ) ;
#42578=DIRECTION ( 'NONE',  ( -1.000000000000000000, 0.000000000000000000, 0.000000000000000000 ) ) ;
#42579=CARTESIAN_POINT ( 'NONE',  ( -29.92777678363736626, -3.750539801530011985, -12.96855624952674724 ) ) ;
#42580=CARTESIAN_POINT ( 'NONE',  ( 6.432001473550251092, -8.074322192336737203, -8.885343091696837448 ) ) ;
#42581=ORIENTED_EDGE ( 'NONE', *, *, #50672, .T. ) ;
#42582=FACE_OUTER_BOUND ( 'NONE', #44575, .T. ) ;
#42583=VECTOR ( 'NONE', #4344, 1000.000000000000000 ) ;
#42587=AXIS2_PLACEMENT_3D ( 'NONE', #47415, #37411, #62346 ) ;
#42588=ORIENTED_EDGE ( 'NONE', *, *, #53900, .T. ) ;
#42591=CARTESIAN_POINT ( 'NONE',  ( -35.00000000000000000, 8.352657516904674395, 8.258652103341463047 ) ) ;
#42592=ORIENTED_EDGE ( 'NONE', *, *, #17599, .F. ) ;
#42593=AXIS2_PLACEMENT_3D ( 'NONE', #40765, #34761, #55063 ) ;
#42594=ORIENTED_EDGE ( 'NONE', *, *, #8566, .T. ) ;
#42596=EDGE_CURVE ( 'NONE', #49507, #55512, #19276, .T. ) ;
#42597=ORIENTED_EDGE ( 'NONE', *, *, #3335, .T. ) ;
#42600=ADVANCED_FACE ( 'NONE', ( #12970 ), #23276, .T. ) ;
#42601=CARTESIAN_POINT ( 'NONE',  ( 35.00000000000000000, -11.73808581813437613, 0.4353888892049613824 ) ) ;
#42602=DIRECTION ( 'NONE',  ( 0.000000000000000000, 0.01356324068817992175, -0.9999080150203990547 ) ) ;
#42603=VERTEX_POINT ( 'NONE', #13302 ) ;
#42606=AXIS2_PLACEMENT_3D ( 'NONE', #24318, #9333, #14338 ) ;
#42607=EDGE_CURVE ( 'NONE', #1074, #63071, #11705, .T. ) ;
#42608=CIRCLE ( 'NONE', #31986, 4.999999999999999112 ) ;
#42610=FACE_OUTER_BOUND ( 'NONE', #16271, .T. ) ;
#42611=AXIS2_PLACEMENT_3D ( 'NONE', #33742, #54045, #8480 ) ;
#42614=FACE_OUTER_BOUND ( 'NONE', #16465, .T. ) ;
#42615=EDGE_CURVE ( 'NONE', #37563, #43734, #54211, .T. ) ;
#42618=AXIS2_PLACEMENT_3D ( 'NONE', #13803, #65011, #59715 ) ;
#42622=AXIS2_PLACEMENT_3D ( 'NONE', #13876, #33842, #54144 ) ;
#42624=CARTESIAN_POINT ( 'NONE',  ( 35.00000000000000000, -5.636262487437393887, -10.80478261802180207 ) ) ;
#42626=VERTEX_POINT ( 'NONE', #54849 ) ;
#42627=CIRCLE ( 'NONE', #46892, 5.000000000000000000 ) ;
#42629=DIRECTION ( 'NONE',  ( 0.000000000000000000, 0.01356324068817998940, -0.9999080150203990547 ) ) ;
#42630=ORIENTED_EDGE ( 'NONE', *, *, #5938, .T. ) ;
#42633=EDGE_LOOP ( 'NONE', ( #50436, #37820, #15057, #41420 ) ) ;
#42636=ORIENTED_EDGE ( 'NONE', *, *, #26045, .F. ) ;
#42637=DIRECTION ( 'NONE',  ( 0.000000000000000000, 0.4698238015817365332, 0.8827602140260315533 ) ) ;
#42639=FACE_OUTER_BOUND ( 'NONE', #45613, .T. ) ;
#42642=CARTESIAN_POINT ( 'NONE',  ( 35.00000000000000000, 4.705694406421931860E-17, -3.469127814946512892E-15 ) ) ;
#42645=CARTESIAN_POINT ( 'NONE',  ( 37.00000000000000711, 6.018036132182163378, -11.24036214326523009 ) ) ;
#42647=DIRECTION ( 'NONE',  ( 0.000000000000000000, -0.01356324068818000328, 0.9999080150203990547 ) ) ;
#42648=ORIENTED_EDGE ( 'NONE', *, *, #23485, .T. ) ;
#42649=DIRECTION ( 'NONE',  ( 0.000000000000000000, 0.8515178078024886466, -0.5243256840888532722 ) ) ;
#42650=EDGE_CURVE ( 'NONE', #21734, #55560, #3347, .T. ) ;
#42651=ORIENTED_EDGE ( 'NONE', *, *, #48613, .T. ) ;
#42652=CARTESIAN_POINT ( 'NONE',  ( 21.83529864932240017, -10.79899791687600619, -5.236407238049663349 ) ) ;
#42653=DIRECTION ( 'NONE',  ( 0.000000000000000000, 0.01356324068817992175, -0.9999080150203990547 ) ) ;
#42654=DIRECTION ( 'NONE',  ( 1.000000000000000000, 0.000000000000000000, 0.000000000000000000 ) ) ;
#42655=EDGE_CURVE ( 'NONE', #20112, #48583, #34024, .T. ) ;
#42657=ORIENTED_EDGE ( 'NONE', *, *, #39861, .F. ) ;
#42658=DIRECTION ( 'NONE',  ( 1.000000000000000000, 0.000000000000000000, -0.000000000000000000 ) ) ;
#42660=CARTESIAN_POINT ( 'NONE',  ( 13.17631928000994712, 11.70382209058883483, -6.731835258288742629 ) ) ;
#42662=VERTEX_POINT ( 'NONE', #14902 ) ;
#42663=EDGE_LOOP ( 'NONE', ( #31347, #15439, #39651, #1354 ) ) ;
#42664=CARTESIAN_POINT ( 'NONE',  ( -37.00000000000000711, -6.564808257521847601, 10.93004082984016634 ) ) ;
#42665=ORIENTED_EDGE ( 'NONE', *, *, #7835, .F. ) ;
#42666=CIRCLE ( 'NONE', #5541, 12.75000000000000178 ) ;
#42669=CYLINDRICAL_SURFACE ( 'NONE', #55102, 5.594511299047803199 ) ;
#42670=DIRECTION ( 'NONE',  ( -1.000000000000000000, -1.836970198721029688E-16, 0.000000000000000000 ) ) ;
#42671=CARTESIAN_POINT ( 'NONE',  ( -37.00000000000000711, -7.474872387600942858, -9.060822531526127932 ) ) ;
#42674=CYLINDRICAL_SURFACE ( 'NONE', #16111, 4.999999999999999112 ) ;
#42675=EDGE_CURVE ( 'NONE', #32268, #57074, #19920, .T. ) ;
#42677=CIRCLE ( 'NONE', #61773, 5.000000000000000888 ) ;
#42678=EDGE_CURVE ( 'NONE', #8992, #60025, #20212, .T. ) ;
#42679=EDGE_CURVE ( 'NONE', #59695, #62587, #51037, .T. ) ;
#42680=ORIENTED_EDGE ( 'NONE', *, *, #9463, .T. ) ;
#42681=CARTESIAN_POINT ( 'NONE',  ( -36.00000000000000711, 4.561791185930588632, -11.90598845858528776 ) ) ;
#42682=EDGE_CURVE ( 'NONE', #4661, #51925, #53170, .T. ) ;
#42684=CIRCLE ( 'NONE', #31029, 5.000000000000000888 ) ;
#42685=VECTOR ( 'NONE', #8368, 1000.000000000000000 ) ;
#42688=VECTOR ( 'NONE', #16796, 1000.000000000000000 ) ;
#42692=CARTESIAN_POINT ( 'NONE',  ( 16.78263030916553333, -12.17295508002144011, 5.836879698929882565 ) ) ;
#42694=CARTESIAN_POINT ( 'NONE',  ( 8.957021277343063304, 4.012943098840286105, -11.31181617744290158 ) ) ;
#42695=ORIENTED_EDGE ( 'NONE', *, *, #29079, .F. ) ;
#42696=DIRECTION ( 'NONE',  ( 1.000000000000000000, -0.000000000000000000, 0.000000000000000000 ) ) ;
#42698=DIRECTION ( 'NONE',  ( 0.000000000000000000, -1.000000000000000000, 0.000000000000000000 ) ) ;
#42701=AXIS2_PLACEMENT_3D ( 'NONE', #38650, #43622, #3431 ) ;
#42703=FACE_OUTER_BOUND ( 'NONE', #129, .T. ) ;
#42705=AXIS2_PLACEMENT_3D ( 'NONE', #15992, #56585, #11026 ) ;
#42706=VERTEX_POINT ( 'NONE', #44862 ) ;
#42707=CARTESIAN_POINT ( 'NONE',  ( 19.21195920369069299, -2.638879775956874507, 11.74464917922519547 ) ) ;
#42708=CARTESIAN_POINT ( 'NONE',  ( -17.32245137130363943, 3.212379320876176170, 13.11341242674679286 ) ) ;
#42710=CIRCLE ( 'NONE', #50204, 5.000000000000000000 ) ;
#42716=ORIENTED_EDGE ( 'NONE', *, *, #38039, .T. ) ;
#42719=DIRECTION ( 'NONE',  ( -1.000000000000000000, -0.000000000000000000, 0.000000000000000000 ) ) ;
#42723=CARTESIAN_POINT ( 'NONE',  ( -37.00000000000000711, 0.000000000000000000, 0.000000000000000000 ) ) ;
#42725=PLANE ( 'NONE',  #56324 ) ;
#42726=DIRECTION ( 'NONE',  ( 0.000000000000000000, -0.1740410799127471153, -0.9847383929261642743 ) ) ;
#42728=CARTESIAN_POINT ( 'NONE',  ( -2.532614230583023041, 12.88560382747354005, 4.026315189028235153 ) ) ;
#42729=ORIENTED_EDGE ( 'NONE', *, *, #37899, .F. ) ;
#42731=ORIENTED_EDGE ( 'NONE', *, *, #33430, .T. ) ;
#42732=CIRCLE ( 'NONE', #44892, 12.18649999999999878 ) ;
#42734=VERTEX_POINT ( 'NONE', #10261 ) ;
#42735=VECTOR ( 'NONE', #14591, 1000.000000000000000 ) ;
#42736=VERTEX_POINT ( 'NONE', #40184 ) ;
#42740=CIRCLE ( 'NONE', #7735, 12.74999999999999822 ) ;
#42741=CARTESIAN_POINT ( 'NONE',  ( -3.386137662399145487, 11.13011477932007232, 4.505408349134588875 ) ) ;
#42742=EDGE_CURVE ( 'NONE', #12098, #14609, #7478, .T. ) ;
#42743=VECTOR ( 'NONE', #31366, 1000.000000000000000 ) ;
#42746=ORIENTED_EDGE ( 'NONE', *, *, #7307, .T. ) ;
#42747=CARTESIAN_POINT ( 'NONE',  ( -35.00000000000000000, -9.908974237959601084, -6.307491713049132365 ) ) ;
#42748=ADVANCED_FACE ( 'NONE', ( #34855 ), #15894, .T. ) ;
#42749=CARTESIAN_POINT ( 'NONE',  ( 2.740575968810160301, 2.123581467810721435, -13.35090380385353548 ) ) ;
#42750=ORIENTED_EDGE ( 'NONE', *, *, #13296, .T. ) ;
#42751=ORIENTED_EDGE ( 'NONE', *, *, #33129, .F. ) ;
#42752=CARTESIAN_POINT ( 'NONE',  ( -1.734723475976807094E-15, -3.469446951953614189E-15, -11.99999999999998934 ) ) ;
#42754=VERTEX_POINT ( 'NONE', #312 ) ;
#42755=AXIS2_PLACEMENT_3D ( 'NONE', #57356, #18701, #37727 ) ;
#42756=CARTESIAN_POINT ( 'NONE',  ( 35.00000000000000000, 4.705694406421931860E-17, -3.469127814946512892E-15 ) ) ;
#42759=CARTESIAN_POINT ( 'NONE',  ( -47.00000000000000711, 0.000000000000000000, 0.000000000000000000 ) ) ;
#42760=AXIS2_PLACEMENT_3D ( 'NONE', #8007, #48566, #33588 ) ;
#42761=DIRECTION ( 'NONE',  ( 1.000000000000000000, 0.000000000000000000, 0.000000000000000000 ) ) ;
#42763=EDGE_CURVE ( 'NONE', #13765, #46293, #65141, .T. ) ;
#42765=ORIENTED_EDGE ( 'NONE', *, *, #55495, .T. ) ;
#42766=FACE_OUTER_BOUND ( 'NONE', #63014, .T. ) ;
#42767=ADVANCED_FACE ( 'NONE', ( #35840 ), #50198, .T. ) ;
#42768=VERTEX_POINT ( 'NONE', #7235 ) ;
#42771=EDGE_CURVE ( 'NONE', #26553, #36879, #46830, .T. ) ;
#42772=CARTESIAN_POINT ( 'NONE',  ( -8.902713192980971968, -10.71502374161934057, -8.218914786477059309 ) ) ;
#42778=CARTESIAN_POINT ( 'NONE',  ( -36.00000000000000711, -10.49626516989265923, -7.238157050195740183 ) ) ;
#42779=VERTEX_POINT ( 'NONE', #32822 ) ;
#42780=CARTESIAN_POINT ( 'NONE',  ( 35.00000000000000000, -10.30098186818245409, 5.644643009979177783 ) ) ;
#42781=EDGE_CURVE ( 'NONE', #5722, #5002, #6612, .T. ) ;
#42786=VERTEX_POINT ( 'NONE', #22205 ) ;
#42787=AXIS2_PLACEMENT_3D ( 'NONE', #64174, #19615, #39877 ) ;
#42790=AXIS2_PLACEMENT_3D ( 'NONE', #49420, #13786, #64020 ) ;
#42791=FACE_OUTER_BOUND ( 'NONE', #35276, .T. ) ;
#42792=DIRECTION ( 'NONE',  ( -1.000000000000000000, -1.836970198721029688E-16, -0.000000000000000000 ) ) ;
#42793=ADVANCED_FACE ( 'NONE', ( #1626 ), #21900, .T. ) ;
#42794=CIRCLE ( 'NONE', #51329, 5.000000000000000000 ) ;
#42795=EDGE_CURVE ( 'NONE', #60735, #39298, #63775, .T. ) ;
#42796=LINE ( 'NONE', #57458, #28804 ) ;
#42801=AXIS2_PLACEMENT_3D ( 'NONE', #23328, #18015, #58601 ) ;
#42803=EDGE_CURVE ( 'NONE', #9125, #51886, #1937, .T. ) ;
#42804=VERTEX_POINT ( 'NONE', #953 ) ;
#42807=CARTESIAN_POINT ( 'NONE',  ( -37.00000000000000711, -11.65554240571058031, 1.456211999474302798 ) ) ;
#42808=CIRCLE ( 'NONE', #5684, 12.74999999999999822 ) ;
#42809=CARTESIAN_POINT ( 'NONE',  ( 37.00000000000000711, -11.38112321385048631, 2.905556151562744382 ) ) ;
#42811=AXIS2_PLACEMENT_3D ( 'NONE', #7576, #38148, #28196 ) ;
#42812=EDGE_LOOP ( 'NONE', ( #54588, #12907, #7023, #25664 ) ) ;
#42813=ORIENTED_EDGE ( 'NONE', *, *, #46514, .T. ) ;
#42814=CARTESIAN_POINT ( 'NONE',  ( 37.00000000000000711, -11.74614673114903596, -0.01609748574441245694 ) ) ;
#42818=CARTESIAN_POINT ( 'NONE',  ( -35.00000000000000000, -7.110831038798204773, -9.896810808925470937 ) ) ;
#42819=CARTESIAN_POINT ( 'NONE',  ( -35.00000000000000000, -12.54989509947649751, -2.250029553613891675 ) ) ;
#42820=CYLINDRICAL_SURFACE ( 'NONE', #65106, 12.18649999999999878 ) ;
#42821=VECTOR ( 'NONE', #48599, 1000.000000000000000 ) ;
#42823=ORIENTED_EDGE ( 'NONE', *, *, #50243, .T. ) ;
#42826=ORIENTED_EDGE ( 'NONE', *, *, #36983, .F. ) ;
#42827=CARTESIAN_POINT ( 'NONE',  ( 21.44662240950248133, -13.04912158988539339, -3.483575318819825739 ) ) ;
#42828=DIRECTION ( 'NONE',  ( -1.000000000000000000, -0.000000000000000000, -0.000000000000000000 ) ) ;
#42829=EDGE_CURVE ( 'NONE', #38497, #56049, #32921, .T. ) ;
#42830=AXIS2_PLACEMENT_3D ( 'NONE', #14157, #13817, #34106 ) ;
#42831=CYLINDRICAL_SURFACE ( 'NONE', #47908, 12.18650000000000055 ) ;
#42832=VERTEX_POINT ( 'NONE', #21222 ) ;
#42833=DIRECTION ( 'NONE',  ( -0.4531421102008652557, 0.000000000000000000, -0.8914382917301156839 ) ) ;
#42836=ORIENTED_EDGE ( 'NONE', *, *, #51284, .F. ) ;
#42837=ORIENTED_EDGE ( 'NONE', *, *, #5809, .F. ) ;
#42839=VERTEX_POINT ( 'NONE', #11260 ) ;
#42841=CIRCLE ( 'NONE', #4662, 12.18650000000000055 ) ;
#42842=DIRECTION ( 'NONE',  ( -1.000000000000000000, -0.000000000000000000, 0.000000000000000000 ) ) ;
#42845=ORIENTED_EDGE ( 'NONE', *, *, #9463, .F. ) ;
#42846=VERTEX_POINT ( 'NONE', #13530 ) ;
#42847=FACE_OUTER_BOUND ( 'NONE', #60952, .T. ) ;
#42850=CARTESIAN_POINT ( 'NONE',  ( -20.15450366670237869, -11.80221610452082714, -2.191204727034115507 ) ) ;
#42852=DIRECTION ( 'NONE',  ( 1.000000000000000000, 0.000000000000000000, 0.000000000000000000 ) ) ;
#42853=DIRECTION ( 'NONE',  ( 0.000000000000000000, -0.5472293298355330737, 0.8369827122275305120 ) ) ;
#42854=ORIENTED_EDGE ( 'NONE', *, *, #21009, .T. ) ;
#42858=B_SPLINE_CURVE_WITH_KNOTS ( 'NONE', 3,
 ( #44172, #13569, #13890, #33857, #28549, #49510, #8592, #48850 ),
 .UNSPECIFIED., .F., .F.,
 ( 4, 2, 2, 4 ),
 ( 0.000000000000000000, 0.002114292923455004559, 0.003171439385182506839, 0.004228585846910009986 ),
 .UNSPECIFIED. ) ;
#42860=EDGE_CURVE ( 'NONE', #16579, #40797, #28195, .T. ) ;
#42861=DIRECTION ( 'NONE',  ( 1.000000000000000000, -0.000000000000000000, 0.000000000000000000 ) ) ;
#42863=DIRECTION ( 'NONE',  ( 1.000000000000000000, 0.000000000000000000, -0.000000000000000000 ) ) ;
#42866=CIRCLE ( 'NONE', #22707, 12.74999999999999822 ) ;
#42867=ORIENTED_EDGE ( 'NONE', *, *, #40924, .T. ) ;
#42868=CARTESIAN_POINT ( 'NONE',  ( -37.00000000000000711, -5.556331110570327247, -11.47561260193582910 ) ) ;
#42869=AXIS2_PLACEMENT_3D ( 'NONE', #59605, #14363, #40278 ) ;
#42873=CIRCLE ( 'NONE', #21675, 5.000000000000000888 ) ;
#42874=CYLINDRICAL_SURFACE ( 'NONE', #3813, 12.18649999999999878 ) ;
#42879=LINE ( 'NONE', #17295, #49293 ) ;
#42880=CARTESIAN_POINT ( 'NONE',  ( -47.00000000000000711, 0.000000000000000000, 0.000000000000000000 ) ) ;
#42881=CARTESIAN_POINT ( 'NONE',  ( 35.00000000000000000, 9.240395740215630482, -7.251710744571611578 ) ) ;
#42884=EDGE_CURVE ( 'NONE', #4710, #20776, #59121, .T. ) ;
#42885=DIRECTION ( 'NONE',  ( 0.000000000000000000, 0.01356324068817992175, -0.9999080150203990547 ) ) ;
#42886=EDGE_LOOP ( 'NONE', ( #21743, #64396, #49959, #49292 ) ) ;
#42888=EDGE_CURVE ( 'NONE', #1051, #63114, #21356, .T. ) ;
#42889=DIRECTION ( 'NONE',  ( 0.000000000000000000, 0.01356324068817998940, -0.9999080150203990547 ) ) ;
#42892=ORIENTED_EDGE ( 'NONE', *, *, #61134, .T. ) ;
#42893=LINE ( 'NONE', #63180, #34977 ) ;
#42896=ORIENTED_EDGE ( 'NONE', *, *, #13505, .F. ) ;
#42900=LINE ( 'NONE', #53216, #338 ) ;
#42901=CARTESIAN_POINT ( 'NONE',  ( -37.00000000000000711, -11.70009620280410978, -1.039216533673027243 ) ) ;
#42903=ORIENTED_EDGE ( 'NONE', *, *, #4375, .F. ) ;
#42905=ORIENTED_EDGE ( 'NONE', *, *, #8273, .F. ) ;
#42906=ORIENTED_EDGE ( 'NONE', *, *, #31364, .F. ) ;
#42909=CARTESIAN_POINT ( 'NONE',  ( -19.47984447937493613, -1.416020129149132334, 25.00000000000000000 ) ) ;
#42912=CARTESIAN_POINT ( 'NONE',  ( -35.00000000000000000, 0.4353888892048373149, 11.73808581813438323 ) ) ;
#42916=CARTESIAN_POINT ( 'NONE',  ( -35.00000000000000000, -10.07641281632181673, 6.036400161834530209 ) ) ;
#42919=DIRECTION ( 'NONE',  ( 0.000000000000000000, 0.01356324068817998940, -0.9999080150203990547 ) ) ;
#42921=ORIENTED_EDGE ( 'NONE', *, *, #8111, .T. ) ;
#42922=ORIENTED_EDGE ( 'NONE', *, *, #42492, .F. ) ;
#42923=LINE ( 'NONE', #17337, #22523 ) ;
#42924=ORIENTED_EDGE ( 'NONE', *, *, #59806, .F. ) ;
#42925=CARTESIAN_POINT ( 'NONE',  ( -20.31672697212907508, 11.54175897114123117, -3.341373981289996298 ) ) ;
#42926=ORIENTED_EDGE ( 'NONE', *, *, #10363, .F. ) ;
#42927=EDGE_CURVE ( 'NONE', #136, #14909, #35087, .T. ) ;
#42932=DIRECTION ( 'NONE',  ( -1.000000000000000000, 0.000000000000000000, 0.000000000000000000 ) ) ;
#42933=FACE_OUTER_BOUND ( 'NONE', #40214, .T. ) ;
#42935=CARTESIAN_POINT ( 'NONE',  ( 4.889044754487288813, -9.933478907102429645, -6.734253674175185722 ) ) ;
#42936=ORIENTED_EDGE ( 'NONE', *, *, #11173, .T. ) ;
#42938=VERTEX_POINT ( 'NONE', #33168 ) ;
#42940=CARTESIAN_POINT ( 'NONE',  ( 35.00000000000000000, 3.511814412392283646, 11.66953048682395355 ) ) ;
#42941=EDGE_CURVE ( 'NONE', #44564, #44595, #45745, .T. ) ;
#42942=EDGE_CURVE ( 'NONE', #11977, #29813, #58540, .T. ) ;
#42943=ORIENTED_EDGE ( 'NONE', *, *, #21685, .T. ) ;
#42947=EDGE_CURVE ( 'NONE', #12619, #2058, #38036, .T. ) ;
#42949=EDGE_LOOP ( 'NONE', ( #49885, #58198, #16857, #45909 ) ) ;
#42951=ORIENTED_EDGE ( 'NONE', *, *, #50892, .T. ) ;
#42952=DIRECTION ( 'NONE',  ( 0.000000000000000000, -0.01356324068817998940, 0.9999080150203990547 ) ) ;
#42953=CARTESIAN_POINT ( 'NONE',  ( -37.00000000000000711, 0.000000000000000000, 0.000000000000000000 ) ) ;
#42955=CARTESIAN_POINT ( 'NONE',  ( -17.74495101254168716, -6.568451298135349781, 10.04738369426859279 ) ) ;
#42958=EDGE_CURVE ( 'NONE', #64815, #11282, #43137, .T. ) ;
#42959=CIRCLE ( 'NONE', #57848, 5.000000000000000000 ) ;
#42960=CIRCLE ( 'NONE', #40833, 5.000000000000000888 ) ;
#42963=CARTESIAN_POINT ( 'NONE',  ( -28.85619398320021745, 3.750539801530000439, 11.39883551934754280 ) ) ;
#42964=LINE ( 'NONE', #17037, #6246 ) ;
#42968=CIRCLE ( 'NONE', #62067, 12.18649999999999878 ) ;
#42969=ORIENTED_EDGE ( 'NONE', *, *, #26962, .T. ) ;
#42972=ORIENTED_EDGE ( 'NONE', *, *, #17599, .T. ) ;
#42976=ORIENTED_EDGE ( 'NONE', *, *, #28228, .T. ) ;
#42977=UNCERTAINTY_MEASURE_WITH_UNIT (LENGTH_MEASURE( 1.000000000000000082E-05 ), #58470, 'distance_accuracy_value', 'NONE');
#42978=DIRECTION ( 'NONE',  ( 0.000000000000000000, 0.9847383929261624980, -0.1740410799127578012 ) ) ;
#42981=CARTESIAN_POINT ( 'NONE',  ( 35.00000000000000000, 2.968224442958566911, 11.81949347079743440 ) ) ;
#42982=EDGE_LOOP ( 'NONE', ( #21078, #578, #3360, #24436 ) ) ;
#42983=VERTEX_POINT ( 'NONE', #59760 ) ;
#42984=DIRECTION ( 'NONE',  ( -1.000000000000000000, 0.000000000000000000, 0.000000000000000000 ) ) ;
#42988=LINE ( 'NONE', #7087, #29373 ) ;
#42989=DIRECTION ( 'NONE',  ( 0.000000000000000000, -1.000000000000000000, 0.000000000000000000 ) ) ;
#42990=CARTESIAN_POINT ( 'NONE',  ( 18.53913913034530125, 6.074311044188305253, 10.35926595326936628 ) ) ;
#42991=EDGE_CURVE ( 'NONE', #38246, #3342, #38343, .T. ) ;
#42992=ORIENTED_EDGE ( 'NONE', *, *, #22683, .T. ) ;
#42993=VECTOR ( 'NONE', #23414, 1000.000000000000000 ) ;
#42995=CARTESIAN_POINT ( 'NONE',  ( -36.00000000000000711, 7.882940143791919319, -10.02106554660700333 ) ) ;
#42997=CARTESIAN_POINT ( 'NONE',  ( -25.54417658651491863, 4.240019242199842608, 11.22596262356930197 ) ) ;
#43002=CARTESIAN_POINT ( 'NONE',  ( 37.00000000000000711, -5.556331110570486231, -11.47561260193575272 ) ) ;
#43006=CIRCLE ( 'NONE', #15388, 5.000000000000000888 ) ;
#43009=EDGE_CURVE ( 'NONE', #24268, #2113, #6012, .T. ) ;
#43012=CARTESIAN_POINT ( 'NONE',  ( 13.37150665029400542, 12.72374181243443303, -4.532386660038074666 ) ) ;
#43013=ORIENTED_EDGE ( 'NONE', *, *, #44428, .F. ) ;
#43014=VERTEX_POINT ( 'NONE', #14823 ) ;
#43016=ORIENTED_EDGE ( 'NONE', *, *, #55095, .F. ) ;
#43017=ORIENTED_EDGE ( 'NONE', *, *, #27568, .T. ) ;
#43018=CARTESIAN_POINT ( 'NONE',  ( 37.00000000000000711, 4.705694406421931860E-17, -3.469127814946512892E-15 ) ) ;
#43022=LINE ( 'NONE', #53679, #15716 ) ;
#43025=DIRECTION ( 'NONE',  ( 1.000000000000000000, 0.000000000000000000, -0.000000000000000000 ) ) ;
#43026=ORIENTED_EDGE ( 'NONE', *, *, #52372, .T. ) ;
#43034=DIRECTION ( 'NONE',  ( 0.000000000000000000, 0.4380125133593974485, -0.8989688749565157844 ) ) ;
#43037=CYLINDRICAL_SURFACE ( 'NONE', #46112, 5.000000000000000888 ) ;
#43038=CARTESIAN_POINT ( 'NONE',  ( -29.43980975494970309, -3.641506875706030488, 11.43413432115373318 ) ) ;
#43041=EDGE_CURVE ( 'NONE', #24391, #16668, #29476, .T. ) ;
#43042=FACE_OUTER_BOUND ( 'NONE', #22121, .T. ) ;
#43045=LINE ( 'NONE', #17790, #29103 ) ;
#43049=ORIENTED_EDGE ( 'NONE', *, *, #37172, .F. ) ;
#43052=ORIENTED_EDGE ( 'NONE', *, *, #43239, .T. ) ;
#43054=CYLINDRICAL_SURFACE ( 'NONE', #3396, 4.999999999999999112 ) ;
#43055=CIRCLE ( 'NONE', #22917, 5.000000000000001776 ) ;
#43057=ORIENTED_EDGE ( 'NONE', *, *, #26930, .T. ) ;
#43058=DIRECTION ( 'NONE',  ( 1.000000000000000000, 0.000000000000000000, 0.000000000000000000 ) ) ;
#43060=LINE ( 'NONE', #53389, #30100 ) ;
#43063=CARTESIAN_POINT ( 'NONE',  ( -27.47732806285103990, 11.55817606591125646, -3.277555523800877779 ) ) ;
#43066=CARTESIAN_POINT ( 'NONE',  ( 35.00000000000000000, 3.473736367725426266, 12.26766708251987481 ) ) ;
#43068=EDGE_CURVE ( 'NONE', #54831, #29266, #24858, .T. ) ;
#43070=ORIENTED_EDGE ( 'NONE', *, *, #48526, .T. ) ;
#43071=CARTESIAN_POINT ( 'NONE',  ( 24.85883792449336838, 0.06046942610558726783, -12.00622078180220953 ) ) ;
#43072=ORIENTED_EDGE ( 'NONE', *, *, #8067, .F. ) ;
#43073=VERTEX_POINT ( 'NONE', #24497 ) ;
#43074=CARTESIAN_POINT ( 'NONE',  ( -26.47549526795953767, 12.14959199744532192, 5.886054789876417281 ) ) ;
#43076=CARTESIAN_POINT ( 'NONE',  ( -24.53407633983860947, 11.34666137335572778, 7.317014004570370211 ) ) ;
#43077=EDGE_CURVE ( 'NONE', #9614, #61242, #34778, .T. ) ;
#43083=FACE_OUTER_BOUND ( 'NONE', #47870, .T. ) ;
#43084=CARTESIAN_POINT ( 'NONE',  ( 35.00000000000000000, 11.68758509253246558, -1.171570255487653700 ) ) ;
#43086=ORIENTED_EDGE ( 'NONE', *, *, #30526, .T. ) ;
#43088=ORIENTED_EDGE ( 'NONE', *, *, #10726, .F. ) ;
#43089=CARTESIAN_POINT ( 'NONE',  ( -37.00000000000000711, 7.379373053629018742, -10.39746860227882763 ) ) ;
#43091=CARTESIAN_POINT ( 'NONE',  ( 9.632875692954998570, 2.208857168211140642, 13.31978269373658641 ) ) ;
#43099=FACE_OUTER_BOUND ( 'NONE', #25698, .T. ) ;
#43101=CARTESIAN_POINT ( 'NONE',  ( -8.891032880924175430, -12.93614229090407974, -3.860857758255645589 ) ) ;
#43103=LINE ( 'NONE', #2902, #46811 ) ;
#43105=ORIENTED_EDGE ( 'NONE', *, *, #28790, .T. ) ;
#43109=CARTESIAN_POINT ( 'NONE',  ( 10.48620311856346454, 8.250315036047107142, 8.713914264323181058 ) ) ;
#43112=ORIENTED_EDGE ( 'NONE', *, *, #3153, .F. ) ;
#43113=FACE_OUTER_BOUND ( 'NONE', #31401, .T. ) ;
#43114=DIRECTION ( 'NONE',  ( 0.000000000000000000, -0.01356324068817992175, 0.9999080150203990547 ) ) ;
#43115=DIRECTION ( 'NONE',  ( -1.000000000000000000, 0.000000000000000000, -0.000000000000000000 ) ) ;
#43116=CARTESIAN_POINT ( 'NONE',  ( -35.00000000000000000, 0.000000000000000000, 0.000000000000000000 ) ) ;
#43117=EDGE_CURVE ( 'NONE', #53955, #40199, #40415, .T. ) ;
#43118=AXIS2_PLACEMENT_3D ( 'NONE', #10367, #54948, #29663 ) ;
#43120=DIRECTION ( 'NONE',  ( 1.000000000000000000, 0.000000000000000000, 0.000000000000000000 ) ) ;
#43121=AXIS2_PLACEMENT_3D ( 'NONE', #61946, #2426, #1769 ) ;
#43122=ORIENTED_EDGE ( 'NONE', *, *, #25027, .F. ) ;
#43126=ORIENTED_EDGE ( 'NONE', *, *, #61473, .F. ) ;
#43127=CARTESIAN_POINT ( 'NONE',  ( -10.95212338237647920, -9.902220863987562183, -6.778349501228825069 ) ) ;
#43129=DIRECTION ( 'NONE',  ( 0.000000000000000000, 0.01356324068817991828, -0.9999080150203990547 ) ) ;
#43131=DIRECTION ( 'NONE',  ( 1.000000000000000000, 0.000000000000000000, 0.000000000000000000 ) ) ;
#43132=EDGE_CURVE ( 'NONE', #29075, #16670, #46847, .T. ) ;
#43134=ORIENTED_EDGE ( 'NONE', *, *, #14048, .F. ) ;
#43137=LINE ( 'NONE', #58806, #17083 ) ;
#43139=CARTESIAN_POINT ( 'NONE',  ( 22.05617246934747300, -13.47655295422364041, -0.7978008018308943017 ) ) ;
#43140=CARTESIAN_POINT ( 'NONE',  ( 35.00000000000000000, 4.705694406421931860E-17, -3.469127814946512892E-15 ) ) ;
#43141=CARTESIAN_POINT ( 'NONE',  ( 35.00000000000000000, 2.936739658819871313, -11.37311665002364869 ) ) ;
#43142=EDGE_CURVE ( 'NONE', #16581, #25502, #18186, .T. ) ;
#43144=DIRECTION ( 'NONE',  ( 0.000000000000000000, -1.000000000000000000, 0.000000000000000000 ) ) ;
#43145=VERTEX_POINT ( 'NONE', #1860 ) ;
#43146=EDGE_CURVE ( 'NONE', #48363, #8671, #6463, .T. ) ;
#43147=ORIENTED_EDGE ( 'NONE', *, *, #4608, .F. ) ;
#43148=DIRECTION ( 'NONE',  ( 1.000000000000000000, 0.000000000000000000, 0.000000000000000000 ) ) ;
#43149=VERTEX_POINT ( 'NONE', #26151 ) ;
#43151=DIRECTION ( 'NONE',  ( 1.000000000000000000, 0.000000000000000000, 0.000000000000000000 ) ) ;
#43152=LINE ( 'NONE', #31542, #18379 ) ;
#43153=EDGE_CURVE ( 'NONE', #47268, #26437, #51078, .T. ) ;
#43154=B_SPLINE_CURVE_WITH_KNOTS ( 'NONE', 3,
 ( #40234, #34903, #60523, #35245, #3734, #23990, #41216, #5685, #50576, #30584, #60867, #8, #36577, #61501, #51567, #51234, #6016, #356 ),
 .UNSPECIFIED., .F., .F.,
 ( 4, 2, 2, 2, 2, 2, 2, 2, 4 ),
 ( 4.336808689942017736E-19, 0.001378279384175299478, 0.002756558768350598522, 0.004134838152525898217, 0.005513117536701197044, 0.006891396920876495871, 0.008269676305051794699, 0.009647955689227093526, 0.01102623507340239235 ),
 .UNSPECIFIED. ) ;
#43155=CARTESIAN_POINT ( 'NONE',  ( -9.351388602708162523, -12.99278190472486827, -3.665735721005250358 ) ) ;
#43156=ORIENTED_EDGE ( 'NONE', *, *, #9586, .T. ) ;
#43157=DIRECTION ( 'NONE',  ( 0.000000000000000000, -0.01356324068817998940, 0.9999080150203990547 ) ) ;
#43160=ADVANCED_FACE ( 'NONE', ( #51443 ), #26462, .T. ) ;
#43161=EDGE_LOOP ( 'NONE', ( #58226, #31538, #65171, #20620 ) ) ;
#43162=ORIENTED_EDGE ( 'NONE', *, *, #15248, .T. ) ;
#43164=ORIENTED_EDGE ( 'NONE', *, *, #40392, .T. ) ;
#43166=ORIENTED_EDGE ( 'NONE', *, *, #48042, .F. ) ;
#43167=CIRCLE ( 'NONE', #4981, 5.000000000000000888 ) ;
#43168=ORIENTED_EDGE ( 'NONE', *, *, #38918, .F. ) ;
#43175=CIRCLE ( 'NONE', #26197, 12.18649999999999878 ) ;
#43176=EDGE_CURVE ( 'NONE', #46663, #23557, #11753, .T. ) ;
#43177=DIRECTION ( 'NONE',  ( 0.000000000000000000, 0.8989688749565172277, 0.4380125133593943398 ) ) ;
#43181=EDGE_CURVE ( 'NONE', #60526, #63812, #62679, .T. ) ;
#43182=LINE ( 'NONE', #63147, #17272 ) ;
#43183=DIRECTION ( 'NONE',  ( -1.000000000000000000, 0.000000000000000000, -0.000000000000000000 ) ) ;
#43184=CARTESIAN_POINT ( 'NONE',  ( 29.72982303775677337, 7.929557435711985569, 9.020309769402173217 ) ) ;
#43188=DIRECTION ( 'NONE',  ( -1.000000000000000000, 0.000000000000000000, 0.000000000000000000 ) ) ;
#43190=DIRECTION ( 'NONE',  ( 0.000000000000000000, 0.01356324068818000328, -0.9999080150203990547 ) ) ;
#43193=CYLINDRICAL_SURFACE ( 'NONE', #44684, 5.000000000000000888 ) ;
#43194=LINE ( 'NONE', #22609, #64293 ) ;
#43198=ORIENTED_EDGE ( 'NONE', *, *, #28656, .T. ) ;
#43199=CARTESIAN_POINT ( 'NONE',  ( 35.00000000000000000, 10.62137734850267989, 5.015831474386340361 ) ) ;
#43200=CARTESIAN_POINT ( 'NONE',  ( 37.00000000000000711, 11.98254675519227952, -2.220215194441947482 ) ) ;
#43201=LINE ( 'NONE', #37895, #16297 ) ;
#43202=CARTESIAN_POINT ( 'NONE',  ( -3.764911300353465329, 12.33769845550319921, 5.494011308154752804 ) ) ;
#43203=EDGE_CURVE ( 'NONE', #37463, #18737, #56397, .T. ) ;
#43205=DIRECTION ( 'NONE',  ( -1.000000000000000000, 0.000000000000000000, 0.000000000000000000 ) ) ;
#43206=CIRCLE ( 'NONE', #50676, 12.18649999999999878 ) ;
#43208=FACE_OUTER_BOUND ( 'NONE', #51602, .T. ) ;
#43210=LINE ( 'NONE', #3677, #52197 ) ;
#43211=EDGE_CURVE ( 'NONE', #9488, #51996, #57065, .T. ) ;
#43212=EDGE_CURVE ( 'NONE', #59561, #57508, #57437, .T. ) ;
#43213=VECTOR ( 'NONE', #11664, 1000.000000000000000 ) ;
#43222=EDGE_LOOP ( 'NONE', ( #8996, #30084, #31360, #11992 ) ) ;
#43223=EDGE_CURVE ( 'NONE', #22151, #51572, #62729, .T. ) ;
#43224=VERTEX_POINT ( 'NONE', #5891 ) ;
#43225=EDGE_LOOP ( 'NONE', ( #11982, #5914, #6389, #58288 ) ) ;
#43227=CARTESIAN_POINT ( 'NONE',  ( -27.30975859563925212, 13.34112994997249757, -2.066478916269103294 ) ) ;
#43228=VERTEX_POINT ( 'NONE', #31456 ) ;
#43229=DIRECTION ( 'NONE',  ( 0.000000000000000000, -1.000000000000000000, 0.000000000000000000 ) ) ;
#43230=CARTESIAN_POINT ( 'NONE',  ( -35.00000000000000000, 11.23004253107764505, 4.732539170486304236 ) ) ;
#43233=CARTESIAN_POINT ( 'NONE',  ( -37.00000000000000711, -10.80478261802186246, 5.636262487437281976 ) ) ;
#43234=EDGE_CURVE ( 'NONE', #20539, #64321, #51757, .T. ) ;
#43236=ORIENTED_EDGE ( 'NONE', *, *, #44870, .T. ) ;
#43237=VERTEX_POINT ( 'NONE', #21139 ) ;
#43238=CARTESIAN_POINT ( 'NONE',  ( 0.2851083653049504285, -0.4107471485392698018, 11.99296822225285730 ) ) ;
#43239=EDGE_CURVE ( 'NONE', #7090, #57074, #56377, .T. ) ;
#43240=EDGE_LOOP ( 'NONE', ( #12015, #37987, #36543, #12631 ) ) ;
#43241=CARTESIAN_POINT ( 'NONE',  ( 8.626688775007931298, 3.155910342056009732, -13.12853318357805676 ) ) ;
#43242=ORIENTED_EDGE ( 'NONE', *, *, #42947, .T. ) ;
#43243=CARTESIAN_POINT ( 'NONE',  ( -35.00000000000000000, 11.42599468261435192, -4.237620530777677530 ) ) ;
#43244=EDGE_CURVE ( 'NONE', #14627, #217, #21827, .T. ) ;
#43246=CARTESIAN_POINT ( 'NONE',  ( -35.00000000000000000, 4.603882218679707705, -10.80631716521661900 ) ) ;
#43250=CARTESIAN_POINT ( 'NONE',  ( -27.01437459610461644, -11.79277645698183186, -2.220455681983952267 ) ) ;
#43251=EDGE_LOOP ( 'NONE', ( #4005, #64524, #4033, #19628 ) ) ;
#43252=ADVANCED_FACE ( 'NONE', ( #57388 ), #11814, .T. ) ;
#43253=CYLINDRICAL_SURFACE ( 'NONE', #27989, 12.75000000000000178 ) ;
#43255=DIRECTION ( 'NONE',  ( 0.000000000000000000, -0.01356324068817998940, 0.9999080150203990547 ) ) ;
#43256=CARTESIAN_POINT ( 'NONE',  ( -37.00000000000000711, 9.076753354954126607, -8.954052073409506818 ) ) ;
#43257=ADVANCED_FACE ( 'NONE', ( #59348 ), #53388, .T. ) ;
#43258=VERTEX_POINT ( 'NONE', #3846 ) ;
#43262=AXIS2_PLACEMENT_3D ( 'NONE', #61402, #51475, #20852 ) ;
#43264=VERTEX_POINT ( 'NONE', #23792 ) ;
#43266=DIRECTION ( 'NONE',  ( 0.000000000000000000, -0.6943713148249532896, 0.7196168960969895334 ) ) ;
#43267=VERTEX_POINT ( 'NONE', #48077 ) ;
#43268=LINE ( 'NONE', #24304, #52965 ) ;
#43269=DIRECTION ( 'NONE',  ( 1.000000000000000000, 0.000000000000000000, 0.000000000000000000 ) ) ;
#43271=CARTESIAN_POINT ( 'NONE',  ( 35.00000000000000000, 9.390600770288113353, 8.624332853795948495 ) ) ;
#43274=FACE_OUTER_BOUND ( 'NONE', #10403, .T. ) ;
#43281=DIRECTION ( 'NONE',  ( -1.000000000000000000, -1.836970198721029688E-16, 0.000000000000000000 ) ) ;
#43282=LINE ( 'NONE', #38967, #60129 ) ;
#43284=EDGE_CURVE ( 'NONE', #4396, #57223, #7482, .T. ) ;
#43285=CIRCLE ( 'NONE', #49673, 5.000000000000000000 ) ;
#43286=VERTEX_POINT ( 'NONE', #48408 ) ;
#43288=CIRCLE ( 'NONE', #57133, 5.000000000000001776 ) ;
#43291=( BOUNDED_CURVE ( )  B_SPLINE_CURVE ( 3, ( #23901, #13257, #18898, #39159 ),
 .UNSPECIFIED., .F., .F. ) 
 B_SPLINE_CURVE_WITH_KNOTS ( ( 4, 4 ),
 ( 1.570796326794895892, 1.607646890824687924 ),
 .UNSPECIFIED. ) 
 CURVE ( )  GEOMETRIC_REPRESENTATION_ITEM ( )  RATIONAL_B_SPLINE_CURVE ( ( 1.000000000000000000, 0.9998868395290251287, 0.9998868395290251287, 1.000000000000000000 ) ) 
 REPRESENTATION_ITEM ( '' )  );
#43292=CARTESIAN_POINT ( 'NONE',  ( -37.00000000000000711, 6.415447294506705589, 11.01837265713075631 ) ) ;
#43293=CARTESIAN_POINT ( 'NONE',  ( -37.00000000000000711, 5.636262487437317503, 10.80478261802183937 ) ) ;
#43295=DIRECTION ( 'NONE',  ( -1.000000000000000000, -0.000000000000000000, 0.000000000000000000 ) ) ;
#43296=ORIENTED_EDGE ( 'NONE', *, *, #49533, .F. ) ;
#43298=CARTESIAN_POINT ( 'NONE',  ( -17.19056858472901084, 2.658600115333382252, 11.70257571668042473 ) ) ;
#43302=CARTESIAN_POINT ( 'NONE',  ( -10.82054232775603708, -8.517672224558221927, -8.456986271403620137 ) ) ;
#43303=ADVANCED_FACE ( 'NONE', ( #8813 ), #28423, .T. ) ;
#43306=AXIS2_PLACEMENT_3D ( 'NONE', #41107, #9531, #61391 ) ;
#43307=VERTEX_POINT ( 'NONE', #28115 ) ;
#43314=CARTESIAN_POINT ( 'NONE',  ( -35.00000000000000000, 5.644643009979071202, 10.30098186818251982 ) ) ;
#43315=FACE_OUTER_BOUND ( 'NONE', #34259, .T. ) ;
#43317=ORIENTED_EDGE ( 'NONE', *, *, #25382, .F. ) ;
#43319=ORIENTED_EDGE ( 'NONE', *, *, #40282, .T. ) ;
#43320=CARTESIAN_POINT ( 'NONE',  ( -35.00000000000000000, 0.000000000000000000, 0.000000000000000000 ) ) ;
#43321=VERTEX_POINT ( 'NONE', #48725 ) ;
#43323=CARTESIAN_POINT ( 'NONE',  ( 47.00000000000000711, 4.705694406421931860E-17, -3.469127814946512892E-15 ) ) ;
#43324=ADVANCED_FACE ( 'NONE', ( #32736 ), #53046, .T. ) ;
#43325=DIRECTION ( 'NONE',  ( -1.000000000000000000, 0.000000000000000000, 0.000000000000000000 ) ) ;
#43326=DIRECTION ( 'NONE',  ( 0.000000000000000000, 0.01356324068817992175, -0.9999080150203990547 ) ) ;
#43328=CARTESIAN_POINT ( 'NONE',  ( 37.00000000000000711, -1.903127969211267700, -11.59095880812007628 ) ) ;
#43329=CARTESIAN_POINT ( 'NONE',  ( -37.00000000000000711, 6.564808257521928425, -10.93004082984011482 ) ) ;
#43330=EDGE_CURVE ( 'NONE', #48271, #39541, #49562, .T. ) ;
#43332=LINE ( 'NONE', #64282, #4061 ) ;
#43333=ORIENTED_EDGE ( 'NONE', *, *, #41675, .T. ) ;
#43335=ORIENTED_EDGE ( 'NONE', *, *, #615, .T. ) ;
#43343=EDGE_CURVE ( 'NONE', #14197, #27631, #52045, .T. ) ;
#43344=DIRECTION ( 'NONE',  ( 0.000000000000000000, 0.3218879778915905709, -0.9467777615094595811 ) ) ;
#43346=ORIENTED_EDGE ( 'NONE', *, *, #12221, .T. ) ;
#43348=CARTESIAN_POINT ( 'NONE',  ( -35.00000000000000000, -3.704519465651227694, -11.60979404548638705 ) ) ;
#43349=CIRCLE ( 'NONE', #40112, 12.18649999999999878 ) ;
#43350=CARTESIAN_POINT ( 'NONE',  ( 6.361445718264521432, -4.355102044641763648, -11.18181944858513077 ) ) ;
#43351=AXIS2_PLACEMENT_3D ( 'NONE', #27395, #16461, #47050 ) ;
#43353=DIRECTION ( 'NONE',  ( -1.000000000000000000, 0.000000000000000000, 0.000000000000000000 ) ) ;
#43356=CARTESIAN_POINT ( 'NONE',  ( -10.90165637462999904, -7.508992741355384304, 11.21895841913464587 ) ) ;
#43359=CARTESIAN_POINT ( 'NONE',  ( -37.00000000000000711, 0.000000000000000000, 0.000000000000000000 ) ) ;
#43362=CARTESIAN_POINT ( 'NONE',  ( -25.69594172210742045, 5.442502809504032868, 10.70006412471200719 ) ) ;
#43363=DIRECTION ( 'NONE',  ( 0.000000000000000000, -0.01356324068817998940, 0.9999080150203990547 ) ) ;
#43368=DIRECTION ( 'NONE',  ( -0.000000000000000000, -0.000000000000000000, -1.000000000000000000 ) ) ;
#43370=CARTESIAN_POINT ( 'NONE',  ( -35.00000000000000000, 0.4871980014163251327, -12.74068829017553384 ) ) ;
#43372=ORIENTED_EDGE ( 'NONE', *, *, #60658, .T. ) ;
#43373=ADVANCED_FACE ( 'NONE', ( #5136 ), #15092, .T. ) ;
#43374=ORIENTED_EDGE ( 'NONE', *, *, #54969, .F. ) ;
#43375=DIRECTION ( 'NONE',  ( -1.000000000000000000, 0.000000000000000000, -0.000000000000000000 ) ) ;
#43376=ADVANCED_FACE ( 'NONE', ( #50692 ), #4150, .F. ) ;
#43377=VECTOR ( 'NONE', #62590, 1000.000000000000000 ) ;
#43378=ORIENTED_EDGE ( 'NONE', *, *, #12198, .T. ) ;
#43379=CARTESIAN_POINT ( 'NONE',  ( -27.45775109278351067, 25.00000000000000000, -8.471355351200609007 ) ) ;
#43381=VECTOR ( 'NONE', #20312, 1000.000000000000000 ) ;
#43382=DIRECTION ( 'NONE',  ( -1.000000000000000000, 0.000000000000000000, 0.000000000000000000 ) ) ;
#43383=AXIS2_PLACEMENT_3D ( 'NONE', #61315, #19461, #31062 ) ;
#43385=CARTESIAN_POINT ( 'NONE',  ( -2.952869152607106251, -11.39722960915210592, 3.755417052241485365 ) ) ;
#43389=EDGE_LOOP ( 'NONE', ( #52079, #48511, #23718, #49030 ) ) ;
#43390=CARTESIAN_POINT ( 'NONE',  ( -35.00000000000000000, 0.000000000000000000, 0.000000000000000000 ) ) ;
#43391=ORIENTED_EDGE ( 'NONE', *, *, #26567, .T. ) ;
#43392=AXIS2_PLACEMENT_3D ( 'NONE', #63783, #18611, #13891 ) ;
#43395=CARTESIAN_POINT ( 'NONE',  ( -17.05443611520388103, 7.955356801464462890, 10.90867276502668659 ) ) ;
#43397=ADVANCED_FACE ( 'NONE', ( #10115 ), #60012, .T. ) ;
#43398=DIRECTION ( 'NONE',  ( -1.000000000000000000, -0.000000000000000000, 0.000000000000000000 ) ) ;
#43399=CARTESIAN_POINT ( 'NONE',  ( 23.56751799445461870, 2.000530838575146575, 11.83544039284797478 ) ) ;
#43400=CARTESIAN_POINT ( 'NONE',  ( 35.00000000000000000, 0.7536123767498499326, -11.72195762423410414 ) ) ;
#43405=CYLINDRICAL_SURFACE ( 'NONE', #37973, 12.18649999999999878 ) ;
#43406=EDGE_LOOP ( 'NONE', ( #61326, #57011, #21584, #56632 ) ) ;
#43407=DIRECTION ( 'NONE',  ( 0.000000000000000000, 0.01356324068817992001, -0.9999080150203990547 ) ) ;
#43408=ORIENTED_EDGE ( 'NONE', *, *, #39106, .T. ) ;
#43409=CARTESIAN_POINT ( 'NONE',  ( 35.00000000000000000, 9.430788938294046631, -7.718225330433843290 ) ) ;
#43411=DIRECTION ( 'NONE',  ( 1.000000000000000000, 0.000000000000000000, -0.000000000000000000 ) ) ;
#43416=AXIS2_PLACEMENT_3D ( 'NONE', #56551, #30289, #5026 ) ;
#43417=CARTESIAN_POINT ( 'NONE',  ( -7.287102677926684535, -8.374986170366028659, -10.59034548381062812 ) ) ;
#43418=ORIENTED_EDGE ( 'NONE', *, *, #57899, .T. ) ;
#43420=CIRCLE ( 'NONE', #54020, 5.000000000000000000 ) ;
#43421=ORIENTED_EDGE ( 'NONE', *, *, #35035, .F. ) ;
#43424=CYLINDRICAL_SURFACE ( 'NONE', #64834, 5.000000000000000888 ) ;
#43425=CIRCLE ( 'NONE', #17958, 12.74999999999999822 ) ;
#43426=AXIS2_PLACEMENT_3D ( 'NONE', #53471, #22543, #16887 ) ;
#43427=CARTESIAN_POINT ( 'NONE',  ( 37.00000000000000711, 12.57916205664484188, 2.080187960898425281 ) ) ;
#43429=AXIS2_PLACEMENT_3D ( 'NONE', #20230, #25894, #46489 ) ;
#43431=ORIENTED_EDGE ( 'NONE', *, *, #31371, .F. ) ;
#43434=EDGE_CURVE ( 'NONE', #48464, #43665, #44221, .T. ) ;
#43435=CARTESIAN_POINT ( 'NONE',  ( 35.00000000000000000, -9.321877890560486435, -7.146664589317880178 ) ) ;
#43436=ORIENTED_EDGE ( 'NONE', *, *, #42392, .T. ) ;
#43439=CARTESIAN_POINT ( 'NONE',  ( 37.00000000000000711, 0.1652884326465054732, -12.18537902504609427 ) ) ;
#43440=AXIS2_PLACEMENT_3D ( 'NONE', #27734, #23758, #48381 ) ;
#43441=LINE ( 'NONE', #33488, #48726 ) ;
#43442=EDGE_CURVE ( 'NONE', #12647, #61044, #43175, .T. ) ;
#43445=ORIENTED_EDGE ( 'NONE', *, *, #50092, .F. ) ;
#43446=DIRECTION ( 'NONE',  ( -1.000000000000000000, -1.836970198721029688E-16, 0.000000000000000000 ) ) ;
#43447=CARTESIAN_POINT ( 'NONE',  ( 29.73007324000527873, 9.884457442835744345, 9.197707082462885708 ) ) ;
#43449=ORIENTED_EDGE ( 'NONE', *, *, #61162, .F. ) ;
#43450=CARTESIAN_POINT ( 'NONE',  ( -17.59645119676047287, 3.550355928000697325, -13.02595742310721150 ) ) ;
#43451=CARTESIAN_POINT ( 'NONE',  ( 37.00000000000000711, 4.705694406421931860E-17, -3.469127814946512892E-15 ) ) ;
#43453=EDGE_CURVE ( 'NONE', #16210, #29920, #45683, .T. ) ;
#43454=DIRECTION ( 'NONE',  ( 0.000000000000000000, 0.01356324068817998940, -0.9999080150203990547 ) ) ;
#43455=DIRECTION ( 'NONE',  ( 1.000000000000000000, 0.000000000000000000, -0.000000000000000000 ) ) ;
#43456=VERTEX_POINT ( 'NONE', #64637 ) ;
#43457=DIRECTION ( 'NONE',  ( 0.000000000000000000, 0.01356324068817998940, -0.9999080150203990547 ) ) ;
#43459=ORIENTED_EDGE ( 'NONE', *, *, #16319, .T. ) ;
#43462=CARTESIAN_POINT ( 'NONE',  ( -35.00000000000000000, -3.307597835713157242, -12.31350058095526734 ) ) ;
#43464=CARTESIAN_POINT ( 'NONE',  ( 35.00000000000000000, 11.65150730582934635, 1.488153103997001514 ) ) ;
#43467=EDGE_LOOP ( 'NONE', ( #49941, #34981, #43335, #22046 ) ) ;
#43468=ORIENTED_EDGE ( 'NONE', *, *, #48689, .F. ) ;
#43470=ORIENTED_EDGE ( 'NONE', *, *, #17993, .T. ) ;
#43473=VECTOR ( 'NONE', #26626, 1000.000000000000000 ) ;
#43474=CARTESIAN_POINT ( 'NONE',  ( 37.00000000000000711, -2.021542716731485001, -12.01765980939841505 ) ) ;
#43475=CARTESIAN_POINT ( 'NONE',  ( -18.25006854224444908, -9.443202773001939221, -9.647586298549935435 ) ) ;
#43479=( BOUNDED_CURVE ( )  B_SPLINE_CURVE ( 3, ( #17847, #18535, #44099, #64367 ),
 .UNSPECIFIED., .F., .F. ) 
 B_SPLINE_CURVE_WITH_KNOTS ( ( 4, 4 ),
 ( 5.656652915288876926, 5.682918742766132958 ),
 .UNSPECIFIED. ) 
 CURVE ( )  GEOMETRIC_REPRESENTATION_ITEM ( )  RATIONAL_B_SPLINE_CURVE ( ( 1.000000000000000000, 0.9999425096852141426, 0.9999425096852141426, 1.000000000000000000 ) ) 
 REPRESENTATION_ITEM ( '' )  );
#43481=CARTESIAN_POINT ( 'NONE',  ( 35.00000000000000000, 5.814360711498443912, 10.70999494708485678 ) ) ;
#43482=VERTEX_POINT ( 'NONE', #34403 ) ;
#43483=ORIENTED_EDGE ( 'NONE', *, *, #5712, .T. ) ;
#43484=DIRECTION ( 'NONE',  ( 0.000000000000000000, 0.9346839223284554299, -0.3554799084908935036 ) ) ;
#43485=ORIENTED_EDGE ( 'NONE', *, *, #63129, .T. ) ;
#43488=AXIS2_PLACEMENT_3D ( 'NONE', #46637, #1431, #37305 ) ;
#43491=DIRECTION ( 'NONE',  ( 0.000000000000000000, 0.9718671068226467646, -0.2355298848897482977 ) ) ;
#43494=DIRECTION ( 'NONE',  ( 0.000000000000000000, -0.01356324068817998940, 0.9999080150203990547 ) ) ;
#43497=ORIENTED_EDGE ( 'NONE', *, *, #6621, .T. ) ;
#43501=CARTESIAN_POINT ( 'NONE',  ( 35.00000000000000000, 4.986700593229853595, 10.63508530065516311 ) ) ;
#43502=CARTESIAN_POINT ( 'NONE',  ( 29.68692493517211872, 6.340234850405881417, 10.20038037279705456 ) ) ;
#43506=CARTESIAN_POINT ( 'NONE',  ( 35.00000000000000000, -8.352657516904727686, -8.258652103341406203 ) ) ;
#43507=AXIS2_PLACEMENT_3D ( 'NONE', #59254, #54907, #34924 ) ;
#43510=ORIENTED_EDGE ( 'NONE', *, *, #14472, .F. ) ;
#43513=ORIENTED_EDGE ( 'NONE', *, *, #26424, .F. ) ;
#43516=FACE_OUTER_BOUND ( 'NONE', #55000, .T. ) ;
#43517=CARTESIAN_POINT ( 'NONE',  ( 11.77567996792922322, -13.29583568948794792, -2.343173910231071133 ) ) ;
#43518=CARTESIAN_POINT ( 'NONE',  ( -10.48620311856347875, -9.720786832536937538, 9.367833439828908482 ) ) ;
#43519=EDGE_CURVE ( 'NONE', #40103, #64752, #63334, .T. ) ;
#43521=EDGE_LOOP ( 'NONE', ( #30498, #15465, #41077, #47828 ) ) ;
#43522=FACE_OUTER_BOUND ( 'NONE', #30441, .T. ) ;
#43523=DIRECTION ( 'NONE',  ( 1.000000000000000000, 0.000000000000000000, 0.000000000000000000 ) ) ;
#43524=CARTESIAN_POINT ( 'NONE',  ( -37.00000000000000711, 12.74921544981111232, -0.1414404973752590444 ) ) ;
#43526=AXIS2_PLACEMENT_3D ( 'NONE', #23540, #12894, #22892 ) ;
#43528=AXIS2_PLACEMENT_3D ( 'NONE', #8548, #28835, #3910 ) ;
#43537=ORIENTED_EDGE ( 'NONE', *, *, #20528, .T. ) ;
#43538=ORIENTED_EDGE ( 'NONE', *, *, #14745, .T. ) ;
#43539=DIRECTION ( 'NONE',  ( -1.000000000000000000, -0.000000000000000000, 0.000000000000000000 ) ) ;
#43542=DIRECTION ( 'NONE',  ( 0.000000000000000000, 0.01356324068817998940, -0.9999080150203989437 ) ) ;
#43550=ORIENTED_EDGE ( 'NONE', *, *, #37164, .F. ) ;
#43551=EDGE_LOOP ( 'NONE', ( #24689, #56085, #13025, #31762 ) ) ;
#43553=AXIS2_PLACEMENT_3D ( 'NONE', #5194, #15481, #25142 ) ;
#43556=ORIENTED_EDGE ( 'NONE', *, *, #13510, .F. ) ;
#43557=CARTESIAN_POINT ( 'NONE',  ( -25.54417658651491863, 25.00000000000000000, 11.22596262356930197 ) ) ;
#43563=ORIENTED_EDGE ( 'NONE', *, *, #28154, .F. ) ;
#43564=ORIENTED_EDGE ( 'NONE', *, *, #17020, .T. ) ;
#43565=CARTESIAN_POINT ( 'NONE',  ( -18.25006854224444908, -9.443202773001939221, 7.404452808139724063 ) ) ;
#43567=CARTESIAN_POINT ( 'NONE',  ( 9.385593601210327819, 1.699086665242807825, -13.39428285523520401 ) ) ;
#43568=ORIENTED_EDGE ( 'NONE', *, *, #9994, .F. ) ;
#43570=AXIS2_PLACEMENT_3D ( 'NONE', #21757, #42007, #12394 ) ;
#43577=EDGE_LOOP ( 'NONE', ( #19831, #50627, #133, #3258 ) ) ;
#43578=FACE_OUTER_BOUND ( 'NONE', #34138, .T. ) ;
#43580=FACE_OUTER_BOUND ( 'NONE', #62, .T. ) ;
#43584=CARTESIAN_POINT ( 'NONE',  ( 35.00000000000000000, 8.029056188533806093, 8.573591947375229338 ) ) ;
#43589=EDGE_CURVE ( 'NONE', #13921, #56844, #24066, .T. ) ;
#43590=ORIENTED_EDGE ( 'NONE', *, *, #35820, .F. ) ;
#43591=CARTESIAN_POINT ( 'NONE',  ( 29.51976981715666781, 25.00000000000000000, 11.09513982864076276 ) ) ;
#43592=AXIS2_PLACEMENT_3D ( 'NONE', #12908, #58826, #29192 ) ;
#43593=ORIENTED_EDGE ( 'NONE', *, *, #33239, .T. ) ;
#43594=CARTESIAN_POINT ( 'NONE',  ( 6.812204945636112896, -4.138731716409435712, -12.84993773446340803 ) ) ;
#43595=CARTESIAN_POINT ( 'NONE',  ( -37.00000000000000711, 8.551552972817082932, 8.052525312709914118 ) ) ;
#43597=CARTESIAN_POINT ( 'NONE',  ( -2.961933481642279986, 6.427243547134065871, 10.16558664581745930 ) ) ;
#43601=EDGE_LOOP ( 'NONE', ( #4578, #29812, #7904, #46527 ) ) ;
#43603=AXIS2_PLACEMENT_3D ( 'NONE', #57149, #26226, #46502 ) ;
#43606=CARTESIAN_POINT ( 'NONE',  ( 22.57855258442564761, -4.427776684447072952, -12.75322679295976691 ) ) ;
#43607=DIRECTION ( 'NONE',  ( 1.000000000000000000, 0.000000000000000000, 0.000000000000000000 ) ) ;
#43608=EDGE_CURVE ( 'NONE', #9125, #46774, #3603, .T. ) ;
#43611=DIRECTION ( 'NONE',  ( 1.000000000000000000, 0.000000000000000000, 0.000000000000000000 ) ) ;
#43614=AXIS2_PLACEMENT_3D ( 'NONE', #18108, #28732, #3497 ) ;
#43616=ADVANCED_FACE ( 'NONE', ( #32658 ), #32999, .T. ) ;
#43618=AXIS2_PLACEMENT_3D ( 'NONE', #65350, #40074, #60360 ) ;
#43619=EDGE_CURVE ( 'NONE', #43307, #48169, #19796, .T. ) ;
#43620=CIRCLE ( 'NONE', #2208, 12.74999999999999822 ) ;
#43621=VERTEX_POINT ( 'NONE', #2790 ) ;
#43622=DIRECTION ( 'NONE',  ( 1.000000000000000000, 0.000000000000000000, -0.000000000000000000 ) ) ;
#43623=B_SPLINE_CURVE_WITH_KNOTS ( 'NONE', 3,
 ( #5769, #21358, #46317, #11065, #47307, #41636, #50978, #1427, #21019, #11378, #56625, #56273, #16029, #6089, #26035, #30665, #16695, #31342, #61925, #16383, #10720, #26676 ),
 .UNSPECIFIED., .F., .F.,
 ( 4, 2, 2, 2, 2, 2, 2, 2, 2, 2, 4 ),
 ( 0.000000000000000000, 0.002098281408793136078, 0.003147422113189705852, 0.004196562817586277361, 0.004721133169784564633, 0.005245703521982852773, 0.005770273874181140045, 0.006294844226379429052, 0.007343984930776007933, 0.007868555282974301276, 0.008393125635172596355 ),
 .UNSPECIFIED. ) ;
#43625=DIRECTION ( 'NONE',  ( -1.000000000000000000, 0.000000000000000000, 0.000000000000000000 ) ) ;
#43626=ORIENTED_EDGE ( 'NONE', *, *, #52709, .T. ) ;
#43627=AXIS2_PLACEMENT_3D ( 'NONE', #322, #20600, #49558 ) ;
#43630=CARTESIAN_POINT ( 'NONE',  ( 36.00000000000000711, -12.54989509947652415, -2.250029553613715372 ) ) ;
#43631=VERTEX_POINT ( 'NONE', #7400 ) ;
#43633=ORIENTED_EDGE ( 'NONE', *, *, #45260, .T. ) ;
#43634=DIRECTION ( 'NONE',  ( 1.000000000000000000, 0.000000000000000000, 0.000000000000000000 ) ) ;
#43638=CARTESIAN_POINT ( 'NONE',  ( 2.473808721753356643, 1.776017171852686927, 13.38732973840310692 ) ) ;
#43640=AXIS2_PLACEMENT_3D ( 'NONE', #26651, #5744, #35947 ) ;
#43641=CARTESIAN_POINT ( 'NONE',  ( 18.23172779988076542, 7.217079634543730471, 9.598093013830757414 ) ) ;
#43642=ORIENTED_EDGE ( 'NONE', *, *, #48382, .F. ) ;
#43643=DIRECTION ( 'NONE',  ( 1.000000000000000000, 0.000000000000000000, 0.000000000000000000 ) ) ;
#43644=DIRECTION ( 'NONE',  ( 0.000000000000000000, -0.01356324068817992175, 0.9999080150203990547 ) ) ;
#43645=CARTESIAN_POINT ( 'NONE',  ( -35.00000000000000000, 0.1414404973752139416, 12.74921544981111232 ) ) ;
#43646=CARTESIAN_POINT ( 'NONE',  ( -27.16190680910944621, -11.80725687591872664, -2.143550592226117768 ) ) ;
#43647=ORIENTED_EDGE ( 'NONE', *, *, #11976, .F. ) ;
#43651=CARTESIAN_POINT ( 'NONE',  ( -17.74124556848530077, 13.28873043644716034, 2.478524752089698246 ) ) ;
#43656=DIRECTION ( 'NONE',  ( 0.000000000000000000, 0.9467777615094583599, 0.3218879778915939016 ) ) ;
#43657=VECTOR ( 'NONE', #34690, 1000.000000000000000 ) ;
#43664=DIRECTION ( 'NONE',  ( 0.000000000000000000, 0.01356324068817991828, -0.9999080150203990547 ) ) ;
#43665=VERTEX_POINT ( 'NONE', #13700 ) ;
#43666=ORIENTED_EDGE ( 'NONE', *, *, #29784, .F. ) ;
#43667=EDGE_CURVE ( 'NONE', #35323, #45277, #42988, .T. ) ;
#43668=LINE ( 'NONE', #58999, #9418 ) ;
#43674=VECTOR ( 'NONE', #10653, 1000.000000000000000 ) ;
#43675=CARTESIAN_POINT ( 'NONE',  ( -34.00000000000000000, -15.00000000000000000, 0.000000000000000000 ) ) ;
#43677=CIRCLE ( 'NONE', #1208, 5.000000000000001776 ) ;
#43681=DIRECTION ( 'NONE',  ( -1.000000000000000000, 0.000000000000000000, 0.000000000000000000 ) ) ;
#43682=VECTOR ( 'NONE', #36703, 1000.000000000000000 ) ;
#43683=CARTESIAN_POINT ( 'NONE',  ( 35.00000000000000000, 4.705694406421931860E-17, -3.469127814946512892E-15 ) ) ;
#43684=LINE ( 'NONE', #34367, #12630 ) ;
#43685=ADVANCED_FACE ( 'NONE', ( #58297 ), #27361, .T. ) ;
#43686=ADVANCED_FACE ( 'NONE', ( #65238 ), #29644, .T. ) ;
#43687=CARTESIAN_POINT ( 'NONE',  ( -17.87894447371652262, -11.34875452035182164, 3.899500356681847801 ) ) ;
#43688=CARTESIAN_POINT ( 'NONE',  ( -37.00000000000000711, -6.917234959366895808, 9.493370459201672773 ) ) ;
#43689=AXIS2_PLACEMENT_3D ( 'NONE', #7266, #27552, #12572 ) ;
#43691=CARTESIAN_POINT ( 'NONE',  ( -11.33725458716604706, -6.569267747456280837, 11.79584098982448914 ) ) ;
#43692=CARTESIAN_POINT ( 'NONE',  ( -10.65488365322695508, -5.750401750040496474, 12.22026421357526260 ) ) ;
#43693=CIRCLE ( 'NONE', #32005, 11.99999999999998579 ) ;
#43694=AXIS2_PLACEMENT_3D ( 'NONE', #57478, #52162, #1299 ) ;
#43695=EDGE_LOOP ( 'NONE', ( #3868, #16182, #15146, #52822 ) ) ;
#43700=ADVANCED_FACE ( 'NONE', ( #65543 ), #30322, .T. ) ;
#43701=AXIS2_PLACEMENT_3D ( 'NONE', #51825, #26534, #46823 ) ;
#43702=VECTOR ( 'NONE', #57850, 1000.000000000000000 ) ;
#43704=EDGE_CURVE ( 'NONE', #10053, #50233, #9180, .T. ) ;
#43706=LINE ( 'NONE', #59666, #43657 ) ;
#43707=ORIENTED_EDGE ( 'NONE', *, *, #51994, .F. ) ;
#43708=CARTESIAN_POINT ( 'NONE',  ( -17.90133771828480391, 4.124690485994089606, 12.85602718881228945 ) ) ;
#43710=DIRECTION ( 'NONE',  ( 1.000000000000000000, 0.000000000000000000, 0.000000000000000000 ) ) ;
#43717=CARTESIAN_POINT ( 'NONE',  ( 35.00000000000000000, -3.614449339633571512, -11.17622378668005290 ) ) ;
#43718=AXIS2_PLACEMENT_3D ( 'NONE', #60936, #16013, #31327 ) ;
#43719=VECTOR ( 'NONE', #35530, 1000.000000000000000 ) ;
#43721=CIRCLE ( 'NONE', #21429, 5.000000000000000888 ) ;
#43723=CARTESIAN_POINT ( 'NONE',  ( -21.17861794710831091, -13.00977982294134883, -3.604945070120774808 ) ) ;
#43726=VECTOR ( 'NONE', #40287, 1000.000000000000000 ) ;
#43728=LINE ( 'NONE', #27133, #33982 ) ;
#43732=CARTESIAN_POINT ( 'NONE',  ( 35.00000000000000000, 4.237620530777968852, 11.42599468261424178 ) ) ;
#43733=AXIS2_PLACEMENT_3D ( 'NONE', #2487, #3143, #23402 ) ;
#43734=VERTEX_POINT ( 'NONE', #5061 ) ;
#43736=CARTESIAN_POINT ( 'NONE',  ( -15.21025129788659136, 8.472317264167026352, 10.51053406556264314 ) ) ;
#43739=CYLINDRICAL_SURFACE ( 'NONE', #24773, 12.74999999999999822 ) ;
#43740=DIRECTION ( 'NONE',  ( 0.000000000000000000, 0.01356324068817998940, -0.9999080150203990547 ) ) ;
#43741=CYLINDRICAL_SURFACE ( 'NONE', #16534, 12.18649999999999878 ) ;
#43742=DIRECTION ( 'NONE',  ( 0.000000000000000000, -0.01356324068817999114, 0.9999080150203989437 ) ) ;
#43743=ORIENTED_EDGE ( 'NONE', *, *, #11104, .T. ) ;
#43746=DIRECTION ( 'NONE',  ( 0.000000000000000000, 0.8827602140260332186, -0.4698238015817332580 ) ) ;
#43747=DIRECTION ( 'NONE',  ( 0.000000000000000000, 0.01356324068817998940, -0.9999080150203990547 ) ) ;
#43750=CARTESIAN_POINT ( 'NONE',  ( -35.00000000000000000, 0.7008968033238767159, 12.16632754454236931 ) ) ;
#43751=ORIENTED_EDGE ( 'NONE', *, *, #23293, .T. ) ;
#43752=ADVANCED_FACE ( 'NONE', ( #24680 ), #59602, .T. ) ;
#43756=CYLINDRICAL_SURFACE ( 'NONE', #31020, 4.999999999999999112 ) ;
#43758=CIRCLE ( 'NONE', #23603, 12.75000000000000178 ) ;
#43760=CARTESIAN_POINT ( 'NONE',  ( -35.00000000000000000, 7.561043153947966999, 9.557269938331581116 ) ) ;
#43762=CIRCLE ( 'NONE', #36344, 5.000000000000001776 ) ;
#43763=DIRECTION ( 'NONE',  ( 0.000000000000000000, -0.9796553971857762111, -0.2006870767258790988 ) ) ;
#43765=ORIENTED_EDGE ( 'NONE', *, *, #27584, .F. ) ;
#43766=ADVANCED_FACE ( 'NONE', ( #45285 ), #39640, .T. ) ;
#43767=DIRECTION ( 'NONE',  ( -1.000000000000000000, 0.000000000000000000, -0.000000000000000000 ) ) ;
#43768=EDGE_CURVE ( 'NONE', #61650, #53266, #35293, .T. ) ;
#43770=FACE_OUTER_BOUND ( 'NONE', #15733, .T. ) ;
#43771=VECTOR ( 'NONE', #59629, 1000.000000000000000 ) ;
#43772=ADVANCED_FACE ( 'NONE', ( #19037 ), #14032, .T. ) ;
#43773=AXIS2_PLACEMENT_3D ( 'NONE', #5881, #61693, #6191 ) ;
#43775=DIRECTION ( 'NONE',  ( 0.000000000000000000, 0.01356324068817998940, -0.9999080150203989437 ) ) ;
#43778=DIRECTION ( 'NONE',  ( 1.000000000000000000, 0.000000000000000000, 0.000000000000000000 ) ) ;
#43781=DIRECTION ( 'NONE',  ( 1.000000000000000000, 0.000000000000000000, 0.000000000000000000 ) ) ;
#43784=DIRECTION ( 'NONE',  ( 0.000000000000000000, 0.9718671068226466536, -0.2355298848897482422 ) ) ;
#43786=CARTESIAN_POINT ( 'NONE',  ( -37.00000000000000711, -12.14284015767849390, -1.030638227056693834 ) ) ;
#43787=EDGE_CURVE ( 'NONE', #58300, #57308, #40277, .T. ) ;
#43788=ADVANCED_FACE ( 'NONE', ( #14668 ), #44604, .T. ) ;
#43789=LINE ( 'NONE', #34460, #139 ) ;
#43790=CIRCLE ( 'NONE', #37419, 12.18649999999999700 ) ;
#43791=CARTESIAN_POINT ( 'NONE',  ( -17.54726996257253191, -12.93490414535027710, 3.865003848717349033 ) ) ;
#43794=CARTESIAN_POINT ( 'NONE',  ( -37.00000000000000711, -12.09831040184925222, 1.463443770872732141 ) ) ;
#43796=VERTEX_POINT ( 'NONE', #9359 ) ;
#43797=CARTESIAN_POINT ( 'NONE',  ( -10.21993208096348660, -3.717392186318608793, -12.98382749989833052 ) ) ;
#43798=FACE_OUTER_BOUND ( 'NONE', #20553, .T. ) ;
#43799=DIRECTION ( 'NONE',  ( 0.000000000000000000, -0.01356324068817998940, 0.9999080150203990547 ) ) ;
#43800=VECTOR ( 'NONE', #6364, 1000.000000000000000 ) ;
#43802=CARTESIAN_POINT ( 'NONE',  ( -9.658042753202595421, -11.20703797639928112, -7.536491558063052487 ) ) ;
#43803=AXIS2_PLACEMENT_3D ( 'NONE', #64459, #59177, #59487 ) ;
#43805=CARTESIAN_POINT ( 'NONE',  ( 35.00000000000000000, 4.705694406421931860E-17, -3.469127814946512892E-15 ) ) ;
#43806=ORIENTED_EDGE ( 'NONE', *, *, #62194, .T. ) ;
#43807=CARTESIAN_POINT ( 'NONE',  ( -35.00000000000000000, 0.000000000000000000, 0.000000000000000000 ) ) ;
#43811=DIRECTION ( 'NONE',  ( 1.000000000000000000, -0.000000000000000000, 0.000000000000000000 ) ) ;
#43812=CARTESIAN_POINT ( 'NONE',  ( 10.48620311856346454, 8.250315036047107142, 10.68561190601526611 ) ) ;
#43813=CARTESIAN_POINT ( 'NONE',  ( -35.00000000000000000, -10.84030624090601869, -6.711949091238257559 ) ) ;
#43814=CARTESIAN_POINT ( 'NONE',  ( -16.98800322446194855, 2.922502605998049674, -13.17987020110343543 ) ) ;
#43816=VERTEX_POINT ( 'NONE', #4410 ) ;
#43822=CARTESIAN_POINT ( 'NONE',  ( 37.00000000000000711, 7.745827850123149005, 10.12742074351888100 ) ) ;
#43823=CARTESIAN_POINT ( 'NONE',  ( 37.00000000000000711, -12.46157735505187247, 2.696588552979187536 ) ) ;
#43824=ORIENTED_EDGE ( 'NONE', *, *, #5858, .F. ) ;
#43826=EDGE_CURVE ( 'NONE', #63134, #14001, #34950, .T. ) ;
#43828=DIRECTION ( 'NONE',  ( -1.000000000000000000, 0.000000000000000000, 0.000000000000000000 ) ) ;
#43830=ORIENTED_EDGE ( 'NONE', *, *, #20735, .T. ) ;
#43831=AXIS2_PLACEMENT_3D ( 'NONE', #21920, #61816, #16270 ) ;
#43832=ORIENTED_EDGE ( 'NONE', *, *, #38334, .T. ) ;
#43833=DIRECTION ( 'NONE',  ( -1.000000000000000000, 0.000000000000000000, 0.000000000000000000 ) ) ;
#43834=DIRECTION ( 'NONE',  ( -1.000000000000000000, 0.000000000000000000, 0.000000000000000000 ) ) ;
#43835=ORIENTED_EDGE ( 'NONE', *, *, #45542, .F. ) ;
#43836=ORIENTED_EDGE ( 'NONE', *, *, #57622, .F. ) ;
#43837=CARTESIAN_POINT ( 'NONE',  ( 35.00000000000000000, 1.463443770872944194, 12.09831040184922024 ) ) ;
#43840=DIRECTION ( 'NONE',  ( -1.000000000000000000, -0.000000000000000000, 0.000000000000000000 ) ) ;
#43841=EDGE_CURVE ( 'NONE', #60276, #34377, #15591, .T. ) ;
#43842=CARTESIAN_POINT ( 'NONE',  ( -35.00000000000000000, 0.000000000000000000, 0.000000000000000000 ) ) ;
#43844=EDGE_LOOP ( 'NONE', ( #27260, #23741, #23052, #35300 ) ) ;
#43847=CYLINDRICAL_SURFACE ( 'NONE', #280, 12.18649999999999878 ) ;
#43848=CARTESIAN_POINT ( 'NONE',  ( -37.00000000000000711, -4.986700593229626222, -10.63508530065527147 ) ) ;
#43852=CARTESIAN_POINT ( 'NONE',  ( -37.00000000000000711, -9.040300684349640292, -7.499679039484155041 ) ) ;
#43853=LINE ( 'NONE', #23584, #2673 ) ;
#43854=AXIS2_PLACEMENT_3D ( 'NONE', #26239, #21236, #40881 ) ;
#43855=DIRECTION ( 'NONE',  ( 0.000000000000000000, -0.01356324068817998940, 0.9999080150203990547 ) ) ;
#43858=ORIENTED_EDGE ( 'NONE', *, *, #58339, .T. ) ;
#43860=ORIENTED_EDGE ( 'NONE', *, *, #36409, .T. ) ;
#43862=DIRECTION ( 'NONE',  ( 0.000000000000000000, -0.01356324068817992175, 0.9999080150203990547 ) ) ;
#43866=VERTEX_POINT ( 'NONE', #52 ) ;
#43868=CARTESIAN_POINT ( 'NONE',  ( -27.31188777422505964, 8.574970748528185638, -8.395320217058440448 ) ) ;
#43870=CARTESIAN_POINT ( 'NONE',  ( -35.00000000000000000, -10.42955799785324444, 6.303578524886909840 ) ) ;
#43873=CARTESIAN_POINT ( 'NONE',  ( -37.00000000000000711, -0.2661492558804205988, 12.18359334611896472 ) ) ;
#43874=ORIENTED_EDGE ( 'NONE', *, *, #22467, .F. ) ;
#43875=VECTOR ( 'NONE', #58237, 1000.000000000000000 ) ;
#43877=ORIENTED_EDGE ( 'NONE', *, *, #18344, .F. ) ;
#43880=EDGE_CURVE ( 'NONE', #34726, #2019, #61269, .T. ) ;
#43881=EDGE_CURVE ( 'NONE', #45989, #42736, #28328, .T. ) ;
#43882=AXIS2_PLACEMENT_3D ( 'NONE', #55923, #6057, #5065 ) ;
#43884=ORIENTED_EDGE ( 'NONE', *, *, #60167, .T. ) ;
#43886=CARTESIAN_POINT ( 'NONE',  ( -36.00000000000000711, 7.238157050195776598, -10.49626516989263614 ) ) ;
#43887=( BOUNDED_CURVE ( )  B_SPLINE_CURVE ( 3, ( #6319, #36222, #57520, #679 ),
 .UNSPECIFIED., .F., .F. ) 
 B_SPLINE_CURVE_WITH_KNOTS ( ( 4, 4 ),
 ( 4.985513291461030505, 4.993910677237380469 ),
 .UNSPECIFIED. ) 
 CURVE ( )  GEOMETRIC_REPRESENTATION_ITEM ( )  RATIONAL_B_SPLINE_CURVE ( ( 1.000000000000000000, 0.9999941236679763534, 0.9999941236679763534, 1.000000000000000000 ) ) 
 REPRESENTATION_ITEM ( '' )  );
#43892=ORIENTED_EDGE ( 'NONE', *, *, #57490, .T. ) ;
#43893=AXIS2_PLACEMENT_3D ( 'NONE', #22775, #38035, #48385 ) ;
#43894=CIRCLE ( 'NONE', #51376, 5.000000000000000888 ) ;
#43895=ORIENTED_EDGE ( 'NONE', *, *, #38046, .F. ) ;
#43898=AXIS2_PLACEMENT_3D ( 'NONE', #14090, #34380, #15070 ) ;
#43899=CARTESIAN_POINT ( 'NONE',  ( 32.00000000000000000, -14.99999999999997513, 0.000000000000000000 ) ) ;
#43900=AXIS2_PLACEMENT_3D ( 'NONE', #38226, #28272, #34231 ) ;
#43901=ADVANCED_FACE ( 'NONE', ( #6054 ), #41925, .T. ) ;
#43902=ORIENTED_EDGE ( 'NONE', *, *, #12422, .F. ) ;
#43903=DIRECTION ( 'NONE',  ( 0.000000000000000000, 0.6269146997507929475, 0.7790879021242551605 ) ) ;
#43904=LINE ( 'NONE', #43230, #16201 ) ;
#43907=EDGE_CURVE ( 'NONE', #37124, #13910, #16662, .T. ) ;
#43908=CARTESIAN_POINT ( 'NONE',  ( 37.00000000000000711, -5.927257550915237871, 10.64792938439761549 ) ) ;
#43911=CIRCLE ( 'NONE', #15228, 5.000000000000000888 ) ;
#43912=ORIENTED_EDGE ( 'NONE', *, *, #15732, .T. ) ;
#43913=CARTESIAN_POINT ( 'NONE',  ( -18.10791796330941494, -9.538085361946240681, 7.283445145555468514 ) ) ;
#43914=EDGE_CURVE ( 'NONE', #37661, #15944, #17285, .T. ) ;
#43918=VECTOR ( 'NONE', #39524, 1000.000000000000000 ) ;
#43919=VERTEX_POINT ( 'NONE', #46592 ) ;
#43921=DIRECTION ( 'NONE',  ( 1.000000000000000000, -0.000000000000000000, 0.000000000000000000 ) ) ;
#43922=CIRCLE ( 'NONE', #23762, 12.75000000000000178 ) ;
#43924=CARTESIAN_POINT ( 'NONE',  ( -35.00000000000000000, 3.511814412392118445, 11.66953048682401040 ) ) ;
#43926=ADVANCED_FACE ( 'NONE', ( #10350 ), #35934, .T. ) ;
#43928=ORIENTED_EDGE ( 'NONE', *, *, #15424, .F. ) ;
#43929=CARTESIAN_POINT ( 'NONE',  ( -47.00000000000000711, 0.000000000000000000, 0.000000000000000000 ) ) ;
#43930=CIRCLE ( 'NONE', #7805, 12.18649999999999878 ) ;
#43931=ORIENTED_EDGE ( 'NONE', *, *, #51147, .F. ) ;
#43933=ADVANCED_FACE ( 'NONE', ( #51279 ), #45952, .T. ) ;
#43934=VECTOR ( 'NONE', #22246, 1000.000000000000000 ) ;
#43936=ORIENTED_EDGE ( 'NONE', *, *, #11188, .T. ) ;
#43939=CARTESIAN_POINT ( 'NONE',  ( -27.19357181888462094, 25.00000000000000000, 5.138615876886901468 ) ) ;
#43941=ORIENTED_EDGE ( 'NONE', *, *, #5961, .F. ) ;
#43949=CARTESIAN_POINT ( 'NONE',  ( 13.04069548818232249, 11.52624043203086046, -3.362534750561068098 ) ) ;
#43950=ORIENTED_EDGE ( 'NONE', *, *, #14678, .T. ) ;
#43955=AXIS2_PLACEMENT_3D ( 'NONE', #59744, #34464, #54766 ) ;
#43957=AXIS2_PLACEMENT_3D ( 'NONE', #23164, #52126, #38791 ) ;
#43958=DIRECTION ( 'NONE',  ( -1.000000000000000000, 0.000000000000000000, 0.000000000000000000 ) ) ;
#43962=LINE ( 'NONE', #24660, #31125 ) ;
#43963=AXIS2_PLACEMENT_3D ( 'NONE', #57161, #43151, #8246 ) ;
#43966=CARTESIAN_POINT ( 'NONE',  ( -35.00000000000000000, 10.91536515067641844, 4.339012074900148619 ) ) ;
#43967=ORIENTED_EDGE ( 'NONE', *, *, #25720, .T. ) ;
#43969=FACE_OUTER_BOUND ( 'NONE', #34416, .T. ) ;
#43970=DIRECTION ( 'NONE',  ( -1.000000000000000000, 0.000000000000000000, -0.000000000000000000 ) ) ;
#43971=VECTOR ( 'NONE', #265, 1000.000000000000000 ) ;
#43974=VERTEX_POINT ( 'NONE', #405 ) ;
#43978=AXIS2_PLACEMENT_3D ( 'NONE', #51314, #52619, #16022 ) ;
#43979=EDGE_CURVE ( 'NONE', #44540, #62927, #1390, .T. ) ;
#43983=CARTESIAN_POINT ( 'NONE',  ( 35.00000000000000000, 4.705694406421931860E-17, -3.469127814946512892E-15 ) ) ;
#43986=DIRECTION ( 'NONE',  ( 0.000000000000000000, 0.5767582926624912343, 0.8169148498130317515 ) ) ;
#43987=EDGE_CURVE ( 'NONE', #16407, #34070, #32056, .T. ) ;
#43988=FACE_OUTER_BOUND ( 'NONE', #891, .T. ) ;
#43990=DIRECTION ( 'NONE',  ( 0.000000000000000000, 0.01356324068817998940, -0.9999080150203990547 ) ) ;
#43991=ORIENTED_EDGE ( 'NONE', *, *, #7260, .T. ) ;
#43996=DIRECTION ( 'NONE',  ( 0.000000000000000000, -0.7790879021242573810, 0.6269146997507903940 ) ) ;
#43997=CIRCLE ( 'NONE', #5804, 12.75000000000000178 ) ;
#43998=VERTEX_POINT ( 'NONE', #6367 ) ;
#43999=CARTESIAN_POINT ( 'NONE',  ( -35.00000000000000000, 2.216820770815248309, -11.53507381115581332 ) ) ;
#44000=CYLINDRICAL_SURFACE ( 'NONE', #47869, 12.75000000000000178 ) ;
#44003=DIRECTION ( 'NONE',  ( 0.8317381556525372810, -0.5551681190699946367, 0.000000000000000000 ) ) ;
#44004=EDGE_CURVE ( 'NONE', #49616, #17690, #26635, .T. ) ;
#44005=CARTESIAN_POINT ( 'NONE',  ( -8.724429002833421265, -2.835377106281230297, -13.19961944769576334 ) ) ;
#44006=DIRECTION ( 'NONE',  ( -1.000000000000000000, 0.000000000000000000, 0.000000000000000000 ) ) ;
#44007=CLOSED_SHELL ( 'NONE', ( #47697, #42285, #62309, #30725, #64308, #40075, #26296, #58424, #7490, #9019, #14648, #59228, #9561, #22092, #31397, #5441, #63395, #4200, #46036, #20189, #6908, #23113, #37801, #53552, #13557, #44337, #8203, #35335, #58687, #43616, #53620, #32912, #49026, #53778, #22322, #4737, #21298, #42538, #9826, #44408, #7140, #10634, #19009, #24789, #40914, #56130, #15622, #38121, #62446, #31182, #32725, #54590, #12318, #15231, #11830, #63835, #20176, #44818, #12148, #60503, #2943, #33970, #42410, #57756, #53094, #24476, #49433, #3780, #19125, #17078, #36433, #55250, #27790, #25516, #48113, #64310, #20117, #40936, #26290, #6649, #59014, #58917, #37297, #26298, #65071, #948, #15943, #1189, #35669, #6998, #51892, #39736, #57200, #50445, #547, #51908, #25151, #26971, #27028, #16159, #4734, #48900, #37524, #13490, #18131, #34955, #57351, #20241, #4768, #34602, #51831, #30059, #1293, #9582, #60197, #7737, #32569, #49443, #40783, #36732, #44214, #20208, #35768, #8882, #51755, #55568, #53885, #55122, #31231, #5016, #65003, #43324, #65663, #2572, #13720, #52639, #59841, #10206, #59587, #7962, #27517, #46958, #37518, #65509, #65132, #32090, #21868, #10923, #29331, #26120, #18466, #4106, #7724, #49839, #60079, #55451, #49851, #10661, #27335, #14159, #9494, #17221, #55588, #57446, #18961, #25688, #11321, #20016, #21149, #55800, #50327, #28166, #32254, #55014, #39943, #18798, #53692, #1584, #39275, #4353, #20924, #23101, #10969, #41043, #46183, #19841, #5359, #4225, #21008, #29406, #7142, #17666, #6250, #21310, #43160, #12713, #55704, #29809, #51826, #47005, #31132, #21546, #11045, #50790, #1031, #6563, #3829, #3670, #14180, #8366, #35514, #40348, #29354, #50818, #64954, #1908, #18562, #37055, #15060, #35436, #25083, #9891, #27976, #35215, #43752, #10193, #22910, #39338, #12759, #43700, #21395, #39788, #61376, #57822, #18040, #11693, #4566, #61079, #52303, #10024, #1834, #51555, #57925, #22138, #23626, #18711, #61266, #62277, #57457, #40273, #32675, #64474, #38575, #29539, #54613, #2951, #6870, #1765, #12633, #61903, #20876, #6853, #3818, #61010, #29141, #605, #52086, #65217, #3087, #50629, #40671, #47968, #53406, #259, #33463, #51213, #50139, #6818, #43257, #21119, #17024, #24554, #1376, #24313, #44350, #16967, #2291, #2576, #53210, #18605, #64897, #1889, #48880, #55371, #38836, #49374, #45199, #15334, #20364, #24196, #18445, #13131, #11551, #47576, #34381, #33476, #54687, #35272, #26480, #47490, #41056, #4436, #1677, #50482, #19741, #13622, #50805, #8412, #676, #36977, #837, #21575, #23669, #7807, #17214, #15063, #58065, #38887, #49791, #30369, #39041, #35551, #10629, #26669, #43252, #3345, #51531, #34840, #12216, #17183, #51634, #61321, #15900, #15255, #26550, #52694, #35579, #51748, #1660, #24142, #56546, #53019, #43686, #44682, #61479, #11338, #52035, #7810, #45634, #24472, #19680, #34515, #26739, #26621, #7918, #44026, #1321, #50084, #34003, #4996, #32157, #7554, #18631, #636, #5605, #47824, #16815, #517, #37738, #44051, #29122, #5038, #20067, #65754, #59641, #42767, #50401, #31871, #52592, #19952, #44888, #48055, #65562, #17213, #44126, #24658, #40987, #26410, #21987, #27546, #52728, #29139, #28923, #25784, #57547, #32630, #57853, #49124, #42099, #7335, #31889, #8709, #33323, #55062, #43397, #54015, #46107, #30987, #120, #17355, #48163, #44555, #37086, #38659, #62806, #53453, #1344, #36064, #41573, #3950, #11909, #52067, #44730, #24448, #12688, #47255, #13287, #47584, #41737, #39777, #44238, #5985, #34885, #39585, #31104, #45949, #40309, #14380, #36801, #711, #42160, #60187, #19061, #33555, #59180, #31426, #15889, #3704, #19625, #35861, #12847, #18408, #8128, #4488, #12594, #13596, #52401, #27010, #62570, #41321, #51391, #6173, #15472, #42363, #48336, #6352, #30680, #52560, #64785, #33012, #44090, #34922, #22881, #35771, #32841, #41103, #32295, #6410, #12107, #30391, #48081, #2749, #25460, #23902, #37321, #25638, #35845, #18771, #15541, #26141, #12983, #35120, #8846, #31304, #31046, #38185, #60704, #10547, #22460, #10124, #26134, #55091, #51838, #28715, #1693, #73, #32781, #12313, #6369, #18781, #982, #40050, #51911, #34646, #59198, #27245, #63923, #63162, #27046, #40352, #26191, #48310, #58098, #55214, #13295, #56458, #33405, #48644, #65499, #36492, #62361, #46874, #1391, #4862, #55064, #32700, #27752, #25609, #27717, #26650, #30616, #56230, #64489, #3098, #3212, #12229, #38556, #46629, #46219, #18727, #30619, #36425, #12766, #15754, #34376, #60680, #33807, #26677, #56971, #19435, #12921, #40923, #64730, #11941, #4189, #28580, #15409, #25859, #19932, #8207, #16858, #64528, #54348, #8627, #62759, #47767, #64924, #18257, #56729, #19520, #26499, #41088, #39383, #39020, #62347, #37565, #21939, #4966, #40059, #58955, #19963, #8306, #21068, #10287, #2313, #43933, #15953, #15521, #10581, #54599, #46567, #62938, #3008, #643, #23788, #55717, #64003, #56914, #46565, #48432, #44140, #58718, #45278, #63073, #63063, #20188, #24397, #63697, #27938, #29908, #43901, #18350, #49605, #41301, #65125, #9255, #11085, #13956, #65305, #50878, #20064, #32496, #14485, #62723, #40417, #10134, #56627, #14621, #27061, #61306, #22190, #41678, #42020, #43926, #28648, #57141, #55317, #59939, #567, #17836, #62969, #42360, #18860, #2744, #11486, #52323, #37477, #47091, #61459, #17969, #4819, #45793, #31448, #185, #56392, #38789, #38453, #7047, #5794, #50470, #30303, #50518, #30092, #4987, #65256, #16288, #458, #20433, #54940, #13969, #41853, #61038, #10638, #30921, #61115, #3407, #17206, #63972, #32341, #41108, #50592, #27482, #6931, #21697, #54394, #25854, #2971, #45612, #9344, #37724, #17731, #15294, #51319, #6683, #53684, #5719, #41700, #4508, #14309, #46266, #31315, #20724, #55418, #15047, #48591, #59365, #39304, #47073, #20719, #65444, #25739, #61944, #58815, #5134, #56636, #39201, #3172, #29316, #10718, #56835, #49044, #11218, #7710, #47369, #25782, #23009, #40414, #50928, #2107, #43788, #56190, #7428, #8107, #39174, #7914, #43303, #51353, #3380, #60010, #30023, #15858, #24121, #20065, #14665, #7843, #20134, #61862, #48940, #9961, #12396, #9612, #13499, #19033, #48362, #58249, #25541, #18946, #16936, #34703, #50169, #64198, #33117, #38032, #11117, #22370, #54511, #40069, #61387, #50976, #62414, #62071, #65533, #7435, #31521, #19821, #25863, #5333, #48999, #38723, #62497, #58951, #2877, #24243, #22985, #63297, #24123, #47686, #32420, #25918, #19332, #42600, #4531, #27748, #5801, #35797, #30088, #31283, #39228, #36637, #39110, #44585, #12132, #23495, #9337, #14726, #61904, #60797, #15453, #48137, #45404, #3415, #41644, #60830, #7406, #38290, #9419, #6496, #27803, #26843, #10556, #61405, #11836, #38951, #30478, #55903, #21135, #4291, #454, #1009, #63239, #39468, #21157, #33176, #25496, #47174, #53227, #9445, #63892, #54986, #19898, #45340, #21263, #18038, #55810, #24461, #2491, #16826, #42793, #16514, #25813, #9165, #41350, #43766, #59621, #23162, #60020, #57115, #16025, #17800, #8471, #2159, #44267, #21792, #14757, #15135, #60223, #4936, #28912, #55791, #19301, #22304, #19595, #28176, #63869, #10443, #62391, #31064, #60753, #1196, #55482, #30911, #41163, #3682, #42748, #29832, #25427, #22240, #21268, #13263, #37415, #29469, #49201, #13145, #12610, #12664, #22928, #27102, #22276, #47695, #6746, #25362, #6090, #57695, #14886, #27694, #49674, #6104, #52106, #49615, #43373, #63050, #26600, #22935, #14781, #19743, #34146, #20691, #4118, #33591, #40428, #18007, #3177, #14345, #5503, #3102, #56202, #3940, #60884, #38735, #13424, #25705, #63578, #8440, #14978, #40558, #8188, #46048, #23059, #4663, #13940, #38265, #54149, #23177, #11808, #49996, #63229, #34316, #51079, #39028, #8460, #41522, #37382, #11974, #23605, #30791, #21721, #52180, #48234, #43376, #23015, #46679, #42191, #31244, #52205, #54107, #61592, #43772, #32897, #60365, #56191, #9882, #15720, #44012, #26587, #45263, #32098, #41421, #55493, #51900, #24127, #32120, #4584, #19142, #14712, #57544, #45779, #40288, #21644, #23060, #5778, #43685, #843, #11608, #18179, #64320 ) ) ;
#44008=VERTEX_POINT ( 'NONE', #22291 ) ;
#44009=CARTESIAN_POINT ( 'NONE',  ( -35.00000000000000000, -11.86701198550358427, 2.772148766916072926 ) ) ;
#44010=ORIENTED_EDGE ( 'NONE', *, *, #21862, .T. ) ;
#44012=ADVANCED_FACE ( 'NONE', ( #33600 ), #27960, .T. ) ;
#44016=CYLINDRICAL_SURFACE ( 'NONE', #64157, 5.000000000000000000 ) ;
#44020=AXIS2_PLACEMENT_3D ( 'NONE', #52077, #38073, #11499 ) ;
#44021=DIRECTION ( 'NONE',  ( -1.000000000000000000, -0.000000000000000000, -0.000000000000000000 ) ) ;
#44022=DIRECTION ( 'NONE',  ( 0.000000000000000000, 0.01356324068817998940, -0.9999080150203990547 ) ) ;
#44023=EDGE_CURVE ( 'NONE', #50432, #9279, #33645, .T. ) ;
#44026=ADVANCED_FACE ( 'NONE', ( #3028 ), #22648, .T. ) ;
#44028=DIRECTION ( 'NONE',  ( 1.000000000000000000, -0.000000000000000000, 0.000000000000000000 ) ) ;
#44029=CARTESIAN_POINT ( 'NONE',  ( -37.00000000000000711, -5.710938531231627202, -11.39945968423477751 ) ) ;
#44034=DIRECTION ( 'NONE',  ( -1.000000000000000000, 0.000000000000000000, 0.000000000000000000 ) ) ;
#44037=CARTESIAN_POINT ( 'NONE',  ( 37.00000000000000711, 7.717887834988244045, -8.854740511458876639 ) ) ;
#44039=CARTESIAN_POINT ( 'NONE',  ( -25.16431053358520131, 6.644570256749198656, 9.998964924726404746 ) ) ;
#44040=DIRECTION ( 'NONE',  ( 0.000000000000000000, -0.01356324068817998940, 0.9999080150203990547 ) ) ;
#44041=AXIS2_PLACEMENT_3D ( 'NONE', #34445, #54748, #44738 ) ;
#44042=VERTEX_POINT ( 'NONE', #17978 ) ;
#44044=FACE_OUTER_BOUND ( 'NONE', #8703, .T. ) ;
#44045=CARTESIAN_POINT ( 'NONE',  ( -2.532614230583026593, 25.00000000000000000, 10.89930238848911337 ) ) ;
#44046=ORIENTED_EDGE ( 'NONE', *, *, #23404, .T. ) ;
#44047=CARTESIAN_POINT ( 'NONE',  ( 22.58560133430949080, 11.74609238061706940, -6.663691428441929077 ) ) ;
#44048=FACE_OUTER_BOUND ( 'NONE', #9285, .T. ) ;
#44049=ORIENTED_EDGE ( 'NONE', *, *, #24910, .F. ) ;
#44050=AXIS2_PLACEMENT_3D ( 'NONE', #62540, #7033, #21996 ) ;
#44051=ADVANCED_FACE ( 'NONE', ( #37605 ), #7016, .T. ) ;
#44052=VERTEX_POINT ( 'NONE', #27287 ) ;
#44054=AXIS2_PLACEMENT_3D ( 'NONE', #20986, #55263, #41267 ) ;
#44055=EDGE_CURVE ( 'NONE', #31243, #50772, #16646, .T. ) ;
#44056=ORIENTED_EDGE ( 'NONE', *, *, #2506, .F. ) ;
#44058=CARTESIAN_POINT ( 'NONE',  ( 35.00000000000000000, 1.903127969211351189, 11.59095880812005497 ) ) ;
#44062=DIRECTION ( 'NONE',  ( 1.000000000000000000, -0.000000000000000000, 0.000000000000000000 ) ) ;
#44063=ORIENTED_EDGE ( 'NONE', *, *, #884, .F. ) ;
#44065=EDGE_CURVE ( 'NONE', #41945, #5651, #37260, .T. ) ;
#44066=ORIENTED_EDGE ( 'NONE', *, *, #56223, .T. ) ;
#44067=DIRECTION ( 'NONE',  ( 0.000000000000000000, -0.8989688749565202253, -0.4380125133593881226 ) ) ;
#44068=VERTEX_POINT ( 'NONE', #2027 ) ;
#44069=ORIENTED_EDGE ( 'NONE', *, *, #26283, .T. ) ;
#44070=DIRECTION ( 'NONE',  ( -1.000000000000000000, 0.000000000000000000, 0.000000000000000000 ) ) ;
#44072=CARTESIAN_POINT ( 'NONE',  ( 36.00000000000000711, -11.10408318471055011, 6.265926637539606325 ) ) ;
#44075=DIRECTION ( 'NONE',  ( 0.000000000000000000, -0.01356324068817998940, 0.9999080150203990547 ) ) ;
#44077=VERTEX_POINT ( 'NONE', #23629 ) ;
#44080=ORIENTED_EDGE ( 'NONE', *, *, #12436, .F. ) ;
#44082=FACE_OUTER_BOUND ( 'NONE', #15208, .T. ) ;
#44085=LINE ( 'NONE', #33115, #39384 ) ;
#44090=ADVANCED_FACE ( 'NONE', ( #57572 ), #42559, .T. ) ;
#44092=EDGE_LOOP ( 'NONE', ( #62244, #19609, #18943, #21404 ) ) ;
#44093=AXIS2_PLACEMENT_3D ( 'NONE', #49037, #39932, #60215 ) ;
#44094=( BOUNDED_CURVE ( )  B_SPLINE_CURVE ( 3, ( #4495, #40703, #15429, #489 ),
 .UNSPECIFIED., .F., .F. ) 
 B_SPLINE_CURVE_WITH_KNOTS ( ( 4, 4 ),
 ( 1.199391138076630670, 1.218670143242656545 ),
 .UNSPECIFIED. ) 
 CURVE ( )  GEOMETRIC_REPRESENTATION_ITEM ( )  RATIONAL_B_SPLINE_CURVE ( ( 1.000000000000000000, 0.9999690269031535905, 0.9999690269031535905, 1.000000000000000000 ) ) 
 REPRESENTATION_ITEM ( '' )  );
#44099=CARTESIAN_POINT ( 'NONE',  ( -10.79971841461721382, -9.842872838453383011, 6.865048668419092337 ) ) ;
#44100=AXIS2_PLACEMENT_3D ( 'NONE', #39740, #53737, #44075 ) ;
#44103=CARTESIAN_POINT ( 'NONE',  ( -8.117819346152851168, -2.374925147350410715, -11.76537966265405188 ) ) ;
#44106=CARTESIAN_POINT ( 'NONE',  ( -37.00000000000000711, 3.827046518385245122, -11.56998259273173701 ) ) ;
#44107=ORIENTED_EDGE ( 'NONE', *, *, #29039, .F. ) ;
#44108=DIRECTION ( 'NONE',  ( -0.9746931518056332067, -0.2235469969004301727, 0.000000000000000000 ) ) ;
#44113=EDGE_CURVE ( 'NONE', #2142, #61832, #47912, .T. ) ;
#44115=EDGE_CURVE ( 'NONE', #18081, #16086, #3944, .T. ) ;
#44119=CARTESIAN_POINT ( 'NONE',  ( 29.14248432514131437, 11.83124089669624901, 6.514580338249294833 ) ) ;
#44121=ORIENTED_EDGE ( 'NONE', *, *, #31510, .T. ) ;
#44124=DIRECTION ( 'NONE',  ( 1.000000000000000000, 0.000000000000000000, 0.000000000000000000 ) ) ;
#44126=ADVANCED_FACE ( 'NONE', ( #28281 ), #48577, .T. ) ;
#44128=CARTESIAN_POINT ( 'NONE',  ( -37.00000000000000711, -11.73808581813438323, 0.4353888892047964587 ) ) ;
#44129=ORIENTED_EDGE ( 'NONE', *, *, #41064, .F. ) ;
#44131=CARTESIAN_POINT ( 'NONE',  ( 35.00000000000000000, 4.545979934229410269, -11.30684963584391234 ) ) ;
#44132=CARTESIAN_POINT ( 'NONE',  ( -37.00000000000000711, -11.07407352312210058, -3.916263239775468197 ) ) ;
#44133=CIRCLE ( 'NONE', #61131, 5.000000000000000888 ) ;
#44136=CYLINDRICAL_SURFACE ( 'NONE', #37544, 12.74999999999999822 ) ;
#44137=CARTESIAN_POINT ( 'NONE',  ( -35.00000000000000000, 0.000000000000000000, 0.000000000000000000 ) ) ;
#44138=CARTESIAN_POINT ( 'NONE',  ( -35.00000000000000000, 0.000000000000000000, 0.000000000000000000 ) ) ;
#44139=ORIENTED_EDGE ( 'NONE', *, *, #55631, .T. ) ;
#44140=ADVANCED_FACE ( 'NONE', ( #58903 ), #28936, .T. ) ;
#44143=ORIENTED_EDGE ( 'NONE', *, *, #28591, .T. ) ;
#44146=EDGE_CURVE ( 'NONE', #56061, #63467, #34241, .T. ) ;
#44147=CIRCLE ( 'NONE', #54791, 12.75000000000000178 ) ;
#44149=DIRECTION ( 'NONE',  ( 1.000000000000000000, 0.000000000000000000, 0.000000000000000000 ) ) ;
#44151=ORIENTED_EDGE ( 'NONE', *, *, #12603, .T. ) ;
#44153=CARTESIAN_POINT ( 'NONE',  ( 37.00000000000000711, 4.705694406421931860E-17, -3.469127814946512892E-15 ) ) ;
#44154=CARTESIAN_POINT ( 'NONE',  ( 24.89615308551568162, -1.134373919475322623, 13.45815213920829656 ) ) ;
#44155=ORIENTED_EDGE ( 'NONE', *, *, #4876, .F. ) ;
#44156=VERTEX_POINT ( 'NONE', #51112 ) ;
#44160=EDGE_LOOP ( 'NONE', ( #37252, #37364, #13191, #985 ) ) ;
#44163=FACE_OUTER_BOUND ( 'NONE', #1217, .T. ) ;
#44165=CYLINDRICAL_SURFACE ( 'NONE', #6534, 4.945031439545089391 ) ;
#44166=CARTESIAN_POINT ( 'NONE',  ( -35.00000000000000000, -9.512294188640947112, 6.891188680298791169 ) ) ;
#44167=EDGE_CURVE ( 'NONE', #32142, #27444, #19828, .T. ) ;
#44168=CARTESIAN_POINT ( 'NONE',  ( 36.00000000000000711, 5.556331110570566167, 11.47561260193570654 ) ) ;
#44171=CARTESIAN_POINT ( 'NONE',  ( -17.58491860973004961, 6.768086267375776899, 9.911307288218484501 ) ) ;
#44172=CARTESIAN_POINT ( 'NONE',  ( -21.17861794710831091, -13.00977982294134883, -3.604945070120774808 ) ) ;
#44175=CARTESIAN_POINT ( 'NONE',  ( -35.00000000000000000, -10.12742074351902133, 7.745827850122974034 ) ) ;
#44177=DIRECTION ( 'NONE',  ( 0.000000000000000000, -0.01356324068817991828, 0.9999080150203990547 ) ) ;
#44179=ORIENTED_EDGE ( 'NONE', *, *, #45424, .F. ) ;
#44180=CARTESIAN_POINT ( 'NONE',  ( -17.99470809830023654, 7.056672321075245335, -9.708842496525370791 ) ) ;
#44182=AXIS2_PLACEMENT_3D ( 'NONE', #64617, #49681, #4126 ) ;
#44183=ORIENTED_EDGE ( 'NONE', *, *, #43619, .T. ) ;
#44184=DIRECTION ( 'NONE',  ( 1.000000000000000000, 0.000000000000000000, -0.000000000000000000 ) ) ;
#44185=FACE_OUTER_BOUND ( 'NONE', #52463, .T. ) ;
#44188=DIRECTION ( 'NONE',  ( 0.000000000000000000, -0.9937233664769772323, 0.1118654143051511785 ) ) ;
#44190=ORIENTED_EDGE ( 'NONE', *, *, #20257, .T. ) ;
#44192=FACE_OUTER_BOUND ( 'NONE', #46476, .T. ) ;
#44194=CYLINDRICAL_SURFACE ( 'NONE', #52940, 12.74999999999999822 ) ;
#44199=ORIENTED_EDGE ( 'NONE', *, *, #27405, .T. ) ;
#44200=CARTESIAN_POINT ( 'NONE',  ( -37.00000000000000711, 7.561043153947966999, 9.557269938331581116 ) ) ;
#44203=CYLINDRICAL_SURFACE ( 'NONE', #6558, 12.74999999999999822 ) ;
#44205=VERTEX_POINT ( 'NONE', #8983 ) ;
#44207=CARTESIAN_POINT ( 'NONE',  ( -27.19357181888462094, 10.84410562793473431, 5.138615876886901468 ) ) ;
#44208=CARTESIAN_POINT ( 'NONE',  ( 37.00000000000000711, 4.705694406421931860E-17, -3.469127814946512892E-15 ) ) ;
#44213=ORIENTED_EDGE ( 'NONE', *, *, #35412, .F. ) ;
#44214=ADVANCED_FACE ( 'NONE', ( #44533 ), #56411, .T. ) ;
#44218=EDGE_CURVE ( 'NONE', #26747, #64221, #23098, .T. ) ;
#44221=CIRCLE ( 'NONE', #11329, 12.18649999999999878 ) ;
#44222=FACE_OUTER_BOUND ( 'NONE', #55162, .T. ) ;
#44223=FACE_BOUND ( 'NONE', #57245, .T. ) ;
#44224=EDGE_LOOP ( 'NONE', ( #26779, #43550, #62518, #39158 ) ) ;
#44225=AXIS2_PLACEMENT_3D ( 'NONE', #39282, #59578, #60226 ) ;
#44226=DIRECTION ( 'NONE',  ( -1.000000000000000000, 0.000000000000000000, -0.000000000000000000 ) ) ;
#44229=ORIENTED_EDGE ( 'NONE', *, *, #24056, .T. ) ;
#44230=EDGE_LOOP ( 'NONE', ( #49015, #35855, #59219, #28349 ) ) ;
#44232=ORIENTED_EDGE ( 'NONE', *, *, #50566, .F. ) ;
#44233=CARTESIAN_POINT ( 'NONE',  ( -36.00000000000000711, -2.696588552978969044, -12.46157735505192399 ) ) ;
#44234=VERTEX_POINT ( 'NONE', #10197 ) ;
#44235=EDGE_LOOP ( 'NONE', ( #24331, #22398, #61995, #17793 ) ) ;
#44236=ORIENTED_EDGE ( 'NONE', *, *, #25086, .F. ) ;
#44237=DIRECTION ( 'NONE',  ( 1.000000000000000000, 0.000000000000000000, 0.000000000000000000 ) ) ;
#44238=ADVANCED_FACE ( 'NONE', ( #23962 ), #61385, .T. ) ;
#44240=CARTESIAN_POINT ( 'NONE',  ( -47.00000000000000711, 0.000000000000000000, 0.000000000000000000 ) ) ;
#44243=ORIENTED_EDGE ( 'NONE', *, *, #485, .T. ) ;
#44245=ORIENTED_EDGE ( 'NONE', *, *, #7115, .F. ) ;
#44247=CARTESIAN_POINT ( 'NONE',  ( -17.77206147034625516, -6.466924801175856885, -11.85381836396156885 ) ) ;
#44249=CARTESIAN_POINT ( 'NONE',  ( -16.73444177318988579, 8.125847110238725080, 8.830413162243864633 ) ) ;
#44250=DIRECTION ( 'NONE',  ( -1.000000000000000000, 0.000000000000000000, -0.000000000000000000 ) ) ;
#44251=LINE ( 'NONE', #9314, #29134 ) ;
#44252=ORIENTED_EDGE ( 'NONE', *, *, #60552, .F. ) ;
#44258=DIRECTION ( 'NONE',  ( 0.000000000000000000, -0.8369827122275287357, -0.5472293298355359603 ) ) ;
#44259=CARTESIAN_POINT ( 'NONE',  ( -28.85619398320021745, 3.750539801530000439, 12.96855624952675612 ) ) ;
#44261=DIRECTION ( 'NONE',  ( -1.000000000000000000, 0.000000000000000000, 0.000000000000000000 ) ) ;
#44262=VERTEX_POINT ( 'NONE', #54553 ) ;
#44264=AXIS2_PLACEMENT_3D ( 'NONE', #37277, #27299, #27626 ) ;
#44267=ADVANCED_FACE ( 'NONE', ( #44222 ), #64492, .T. ) ;
#44269=( BOUNDED_CURVE ( )  B_SPLINE_CURVE ( 3, ( #6626, #51844, #47196, #1950 ),
 .UNSPECIFIED., .F., .F. ) 
 B_SPLINE_CURVE_WITH_KNOTS ( ( 4, 4 ),
 ( 4.384824308196885845, 4.401948620082515973 ),
 .UNSPECIFIED. ) 
 CURVE ( )  GEOMETRIC_REPRESENTATION_ITEM ( )  RATIONAL_B_SPLINE_CURVE ( ( 1.000000000000000000, 0.9999755633111596653, 0.9999755633111596653, 1.000000000000000000 ) ) 
 REPRESENTATION_ITEM ( '' )  );
#44270=CARTESIAN_POINT ( 'NONE',  ( -19.47984447937493613, -3.750539801530005768, 11.39883551934753925 ) ) ;
#44271=CARTESIAN_POINT ( 'NONE',  ( -35.00000000000000000, -2.527899948230555083, -12.49688848680886899 ) ) ;
#44274=DIRECTION ( 'NONE',  ( -1.000000000000000000, 0.000000000000000000, 0.000000000000000000 ) ) ;
#44277=ORIENTED_EDGE ( 'NONE', *, *, #50298, .F. ) ;
#44278=DIRECTION ( 'NONE',  ( 0.000000000000000000, 0.6269146997507930585, 0.7790879021242551605 ) ) ;
#44279=VERTEX_POINT ( 'NONE', #5566 ) ;
#44281=DIRECTION ( 'NONE',  ( 1.000000000000000000, 0.000000000000000000, 0.000000000000000000 ) ) ;
#44285=EDGE_CURVE ( 'NONE', #43866, #26911, #53870, .T. ) ;
#44287=ORIENTED_EDGE ( 'NONE', *, *, #32616, .T. ) ;
#44290=EDGE_CURVE ( 'NONE', #13265, #56863, #44311, .T. ) ;
#44295=ORIENTED_EDGE ( 'NONE', *, *, #35824, .F. ) ;
#44297=VECTOR ( 'NONE', #27720, 1000.000000000000000 ) ;
#44299=CARTESIAN_POINT ( 'NONE',  ( -35.00000000000000000, -1.591260454995328866, 12.08216339958900321 ) ) ;
#44300=CARTESIAN_POINT ( 'NONE',  ( -37.00000000000000711, 8.954052073409602741, 9.076753354954030684 ) ) ;
#44302=FACE_OUTER_BOUND ( 'NONE', #32883, .T. ) ;
#44303=EDGE_LOOP ( 'NONE', ( #36454, #48180, #40925, #61638 ) ) ;
#44304=LINE ( 'NONE', #38005, #22029 ) ;
#44305=VERTEX_POINT ( 'NONE', #58063 ) ;
#44306=AXIS2_PLACEMENT_3D ( 'NONE', #52908, #46944, #58230 ) ;
#44308=CYLINDRICAL_SURFACE ( 'NONE', #50015, 12.74999999999999822 ) ;
#44309=DIRECTION ( 'NONE',  ( 0.000000000000000000, 0.4380125133593913422, -0.8989688749565187820 ) ) ;
#44311=CIRCLE ( 'NONE', #30496, 5.000000000000000000 ) ;
#44312=CYLINDRICAL_SURFACE ( 'NONE', #36600, 5.000000000000000888 ) ;
#44315=ORIENTED_EDGE ( 'NONE', *, *, #7362, .T. ) ;
#44318=VERTEX_POINT ( 'NONE', #61718 ) ;
#44319=ORIENTED_EDGE ( 'NONE', *, *, #39999, .T. ) ;
#44324=LINE ( 'NONE', #27724, #62426 ) ;
#44327=CARTESIAN_POINT ( 'NONE',  ( 35.00000000000000000, -11.99999999999997335, 0.000000000000000000 ) ) ;
#44328=ORIENTED_EDGE ( 'NONE', *, *, #48042, .T. ) ;
#44331=CARTESIAN_POINT ( 'NONE',  ( -17.28242249393871077, -6.356211991155408469, 11.91462509628643396 ) ) ;
#44333=AXIS2_PLACEMENT_3D ( 'NONE', #7415, #2802, #53972 ) ;
#44334=EDGE_CURVE ( 'NONE', #40228, #50945, #14575, .T. ) ;
#44337=ADVANCED_FACE ( 'NONE', ( #57399 ), #41425, .T. ) ;
#44338=CARTESIAN_POINT ( 'NONE',  ( -7.720452942165356269, -2.151506517681229802, 13.32786889207912573 ) ) ;
#44339=EDGE_CURVE ( 'NONE', #20076, #153, #52084, .T. ) ;
#44340=ORIENTED_EDGE ( 'NONE', *, *, #21431, .F. ) ;
#44341=DIRECTION ( 'NONE',  ( 0.000000000000000000, -0.01356324068817992175, 0.9999080150203990547 ) ) ;
#44343=DIRECTION ( 'NONE',  ( 0.000000000000000000, 0.01356324068817998073, -0.9999080150203990547 ) ) ;
#44344=AXIS2_PLACEMENT_3D ( 'NONE', #46383, #57027, #47693 ) ;
#44347=FACE_OUTER_BOUND ( 'NONE', #16894, .T. ) ;
#44348=ORIENTED_EDGE ( 'NONE', *, *, #8180, .F. ) ;
#44350=ADVANCED_FACE ( 'NONE', ( #52747 ), #22143, .T. ) ;
#44352=DIRECTION ( 'NONE',  ( 0.000000000000000000, 0.8009703041134189627, 0.5987040770935648792 ) ) ;
#44353=ORIENTED_EDGE ( 'NONE', *, *, #4180, .T. ) ;
#44354=FACE_OUTER_BOUND ( 'NONE', #64973, .T. ) ;
#44358=DIRECTION ( 'NONE',  ( 0.000000000000000000, 0.01356324068818000848, -0.9999080150203990547 ) ) ;
#44359=EDGE_LOOP ( 'NONE', ( #8384, #59166, #48702, #19580 ) ) ;
#44361=DIRECTION ( 'NONE',  ( 0.000000000000000000, 0.01356324068817992175, -0.9999080150203990547 ) ) ;
#44362=CARTESIAN_POINT ( 'NONE',  ( -37.00000000000000711, -9.493370459201647904, -6.917234959366931335 ) ) ;
#44364=CARTESIAN_POINT ( 'NONE',  ( -35.00000000000000000, 10.99909370905157324, 5.246972444134057056 ) ) ;
#44366=DIRECTION ( 'NONE',  ( -0.000000000000000000, -1.000000000000000000, -0.000000000000000000 ) ) ;
#44367=CARTESIAN_POINT ( 'NONE',  ( -37.00000000000000711, 0.7008968033238769380, 12.16632754454237286 ) ) ;
#44368=ORIENTED_EDGE ( 'NONE', *, *, #52732, .T. ) ;
#44370=VERTEX_POINT ( 'NONE', #11508 ) ;
#44371=CARTESIAN_POINT ( 'NONE',  ( -35.00000000000000000, 11.99999999999999289, 1.469576158976823158E-15 ) ) ;
#44372=ORIENTED_EDGE ( 'NONE', *, *, #65136, .F. ) ;
#44373=ORIENTED_EDGE ( 'NONE', *, *, #17032, .T. ) ;
#44374=CARTESIAN_POINT ( 'NONE',  ( -25.79691289529483456, 11.91773619621119984, 6.342745573918120883 ) ) ;
#44376=AXIS2_PLACEMENT_3D ( 'NONE', #31245, #41865, #51550 ) ;
#44379=CARTESIAN_POINT ( 'NONE',  ( -35.00000000000000000, 9.060822531526156354, -7.474872387600913548 ) ) ;
#44381=ORIENTED_EDGE ( 'NONE', *, *, #25654, .F. ) ;
#44382=VECTOR ( 'NONE', #2227, 1000.000000000000000 ) ;
#44384=FACE_OUTER_BOUND ( 'NONE', #45472, .T. ) ;
#44387=DIRECTION ( 'NONE',  ( 1.000000000000000000, 0.000000000000000000, -0.000000000000000000 ) ) ;
#44388=AXIS2_PLACEMENT_3D ( 'NONE', #62008, #31087, #32383 ) ;
#44389=DIRECTION ( 'NONE',  ( 0.000000000000000000, 0.5472293298355273006, -0.8369827122275343978 ) ) ;
#44390=FACE_OUTER_BOUND ( 'NONE', #44891, .T. ) ;
#44391=DIRECTION ( 'NONE',  ( 1.000000000000000000, 0.000000000000000000, 0.000000000000000000 ) ) ;
#44394=CARTESIAN_POINT ( 'NONE',  ( -35.00000000000000000, 11.54110654723652196, -2.185196060783755279 ) ) ;
#44395=ORIENTED_EDGE ( 'NONE', *, *, #54726, .F. ) ;
#44396=ORIENTED_EDGE ( 'NONE', *, *, #25027, .T. ) ;
#44397=CARTESIAN_POINT ( 'NONE',  ( -35.00000000000000000, 10.07641281632186114, -6.036400161834460043 ) ) ;
#44398=CYLINDRICAL_SURFACE ( 'NONE', #3239, 12.18649999999999878 ) ;
#44401=CARTESIAN_POINT ( 'NONE',  ( 35.00000000000000000, -11.86701198550353986, 2.772148766916240348 ) ) ;
#44402=EDGE_CURVE ( 'NONE', #8191, #2866, #58458, .T. ) ;
#44403=DIRECTION ( 'NONE',  ( 0.000000000000000000, -0.3218879778916040602, 0.9467777615094549182 ) ) ;
#44404=DIRECTION ( 'NONE',  ( 0.000000000000000000, -0.01356324068817998940, 0.9999080150203990547 ) ) ;
#44405=CARTESIAN_POINT ( 'NONE',  ( 35.00000000000000000, -7.717887834988180984, 8.854740511458926377 ) ) ;
#44408=ADVANCED_FACE ( 'NONE', ( #53059 ), #12811, .T. ) ;
#44410=CARTESIAN_POINT ( 'NONE',  ( -20.92008205012190558, 11.37744109147144478, -3.816568647652260893 ) ) ;
#44411=CARTESIAN_POINT ( 'NONE',  ( 22.88594695219327235, -4.822122601967141264, -10.98850006195556261 ) ) ;
#44416=AXIS2_PLACEMENT_3D ( 'NONE', #38211, #63170, #42532 ) ;
#44417=CIRCLE ( 'NONE', #32738, 4.999999999999999112 ) ;
#44420=DIRECTION ( 'NONE',  ( 0.000000000000000000, 0.000000000000000000, -1.000000000000000000 ) ) ;
#44421=EDGE_CURVE ( 'NONE', #49715, #6120, #44768, .T. ) ;
#44424=VECTOR ( 'NONE', #34588, 1000.000000000000000 ) ;
#44425=DIRECTION ( 'NONE',  ( 1.000000000000000000, 0.000000000000000000, 0.000000000000000000 ) ) ;
#44426=FACE_OUTER_BOUND ( 'NONE', #30698, .T. ) ;
#44428=EDGE_CURVE ( 'NONE', #57229, #17445, #38424, .T. ) ;
#44429=AXIS2_PLACEMENT_3D ( 'NONE', #9235, #29517, #34517 ) ;
#44431=DIRECTION ( 'NONE',  ( 1.000000000000000000, 0.000000000000000000, 0.000000000000000000 ) ) ;
#44432=EDGE_CURVE ( 'NONE', #4911, #17999, #3858, .T. ) ;
#44434=EDGE_CURVE ( 'NONE', #9194, #33841, #22011, .T. ) ;
#44435=VERTEX_POINT ( 'NONE', #18808 ) ;
#44436=CARTESIAN_POINT ( 'NONE',  ( -35.00000000000000000, 10.91536515067641844, 4.339012074900148619 ) ) ;
#44437=CARTESIAN_POINT ( 'NONE',  ( -7.636175482883169607, 8.975028534027133631, -10.10016484640243206 ) ) ;
#44439=CARTESIAN_POINT ( 'NONE',  ( -16.32507661864641690, 8.302421046862596299, -10.64603329338183535 ) ) ;
#44440=DIRECTION ( 'NONE',  ( 0.000000000000000000, -0.01356324068817992175, 0.9999080150203990547 ) ) ;
#44443=EDGE_CURVE ( 'NONE', #7895, #8559, #39066, .T. ) ;
#44444=FACE_OUTER_BOUND ( 'NONE', #16680, .T. ) ;
#44445=FACE_OUTER_BOUND ( 'NONE', #61790, .T. ) ;
#44446=ORIENTED_EDGE ( 'NONE', *, *, #37572, .T. ) ;
#44447=ORIENTED_EDGE ( 'NONE', *, *, #29721, .F. ) ;
#44448=CARTESIAN_POINT ( 'NONE',  ( -19.16592786555497696, -4.507658645640362671, -11.12154949745637822 ) ) ;
#44452=AXIS2_PLACEMENT_3D ( 'NONE', #40918, #24641, #40582 ) ;
#44454=ORIENTED_EDGE ( 'NONE', *, *, #20799, .F. ) ;
#44457=AXIS2_PLACEMENT_3D ( 'NONE', #35324, #25691, #24713 ) ;
#44458=CARTESIAN_POINT ( 'NONE',  ( 23.47278007031500735, -4.309240334934965055, 12.79762753354781424 ) ) ;
#44460=ORIENTED_EDGE ( 'NONE', *, *, #42171, .F. ) ;
#44461=DIRECTION ( 'NONE',  ( -1.000000000000000000, 0.000000000000000000, 0.000000000000000000 ) ) ;
#44462=DIRECTION ( 'NONE',  ( -1.000000000000000000, -0.000000000000000000, 0.000000000000000000 ) ) ;
#44463=VERTEX_POINT ( 'NONE', #45698 ) ;
#44464=CARTESIAN_POINT ( 'NONE',  ( 6.145364549962366141, -8.619588047944827025, -8.357433972611021389 ) ) ;
#44465=ORIENTED_EDGE ( 'NONE', *, *, #45552, .T. ) ;
#44468=CIRCLE ( 'NONE', #23230, 12.18649999999999878 ) ;
#44470=DIRECTION ( 'NONE',  ( 0.000000000000000000, 0.01356324068817998940, -0.9999080150203990547 ) ) ;
#44473=AXIS2_PLACEMENT_3D ( 'NONE', #29619, #39613, #60224 ) ;
#44476=CARTESIAN_POINT ( 'NONE',  ( -15.23330792070994022, 7.971159899242214131, 8.970046877445025046 ) ) ;
#44480=CARTESIAN_POINT ( 'NONE',  ( -19.63490967323701142, 13.44825352614632052, -1.323441864413900770 ) ) ;
#44484=EDGE_CURVE ( 'NONE', #5002, #6117, #32618, .T. ) ;
#44485=AXIS2_PLACEMENT_3D ( 'NONE', #38031, #48696, #54345 ) ;
#44486=DIRECTION ( 'NONE',  ( -1.000000000000000000, 0.000000000000000000, 0.000000000000000000 ) ) ;
#44489=ORIENTED_EDGE ( 'NONE', *, *, #62906, .T. ) ;
#44492=CARTESIAN_POINT ( 'NONE',  ( -35.00000000000000000, 6.307491713049167004, -9.908974237959577991 ) ) ;
#44494=CARTESIAN_POINT ( 'NONE',  ( 37.00000000000000711, -11.73808581813437613, 0.4353888892049613824 ) ) ;
#44496=ORIENTED_EDGE ( 'NONE', *, *, #11953, .F. ) ;
#44498=CARTESIAN_POINT ( 'NONE',  ( -35.00000000000000000, 12.38385022362081855, 3.033604067594621867 ) ) ;
#44500=CYLINDRICAL_SURFACE ( 'NONE', #5160, 5.000000000000000888 ) ;
#44502=CIRCLE ( 'NONE', #8397, 12.75000000000000178 ) ;
#44503=CARTESIAN_POINT ( 'NONE',  ( 35.00000000000000000, 4.705694406421931860E-17, -3.469127814946512892E-15 ) ) ;
#44505=DIRECTION ( 'NONE',  ( 1.000000000000000000, -0.000000000000000000, -0.000000000000000000 ) ) ;
#44509=DIRECTION ( 'NONE',  ( 1.000000000000000000, 0.000000000000000000, 0.000000000000000000 ) ) ;
#44512=AXIS2_PLACEMENT_3D ( 'NONE', #4219, #24488, #44765 ) ;
#44513=VERTEX_POINT ( 'NONE', #65630 ) ;
#44514=VERTEX_POINT ( 'NONE', #55353 ) ;
#44516=EDGE_CURVE ( 'NONE', #33199, #64603, #41122, .T. ) ;
#44517=AXIS2_PLACEMENT_3D ( 'NONE', #5705, #36254, #25977 ) ;
#44520=DIRECTION ( 'NONE',  ( 0.000000000000000000, 0.9937233664769756780, -0.1118654143051654171 ) ) ;
#44522=EDGE_CURVE ( 'NONE', #7430, #15987, #12445, .T. ) ;
#44524=CARTESIAN_POINT ( 'NONE',  ( -18.89934820819560102, -11.99999999999998934, 0.3178145231930626369 ) ) ;
#44526=ORIENTED_EDGE ( 'NONE', *, *, #52931, .F. ) ;
#44527=AXIS2_PLACEMENT_3D ( 'NONE', #36197, #25582, #55184 ) ;
#44528=VERTEX_POINT ( 'NONE', #40368 ) ;
#44529=DIRECTION ( 'NONE',  ( -1.000000000000000000, 0.000000000000000000, 0.000000000000000000 ) ) ;
#44531=EDGE_LOOP ( 'NONE', ( #9688, #47847, #29263, #64209 ) ) ;
#44533=FACE_OUTER_BOUND ( 'NONE', #32048, .T. ) ;
#44534=FACE_BOUND ( 'NONE', #31820, .T. ) ;
#44537=DIRECTION ( 'NONE',  ( 1.000000000000000000, 0.000000000000000000, -0.000000000000000000 ) ) ;
#44539=EDGE_LOOP ( 'NONE', ( #77, #25006, #56652, #52683 ) ) ;
#44540=VERTEX_POINT ( 'NONE', #21419 ) ;
#44544=ORIENTED_EDGE ( 'NONE', *, *, #50647, .T. ) ;
#44545=ORIENTED_EDGE ( 'NONE', *, *, #41245, .F. ) ;
#44546=ORIENTED_EDGE ( 'NONE', *, *, #52565, .T. ) ;
#44549=CIRCLE ( 'NONE', #6327, 4.999999999999999112 ) ;
#44550=AXIS2_PLACEMENT_3D ( 'NONE', #63959, #59637, #13098 ) ;
#44551=FACE_OUTER_BOUND ( 'NONE', #13104, .T. ) ;
#44552=DIRECTION ( 'NONE',  ( -1.000000000000000000, 0.000000000000000000, 0.000000000000000000 ) ) ;
#44553=ORIENTED_EDGE ( 'NONE', *, *, #51882, .T. ) ;
#44554=CARTESIAN_POINT ( 'NONE',  ( 37.00000000000000711, -3.340853584269612764, -11.26103545359855040 ) ) ;
#44555=ADVANCED_FACE ( 'NONE', ( #31066 ), #31700, .T. ) ;
#44556=ORIENTED_EDGE ( 'NONE', *, *, #43787, .T. ) ;
#44557=CARTESIAN_POINT ( 'NONE',  ( 35.00000000000000000, -6.657191900728386180, -9.677500615117878624 ) ) ;
#44558=CARTESIAN_POINT ( 'NONE',  ( -35.00000000000000000, 10.43555801961483098, -5.391785509270847321 ) ) ;
#44560=DIRECTION ( 'NONE',  ( 0.000000000000000000, 0.01356324068817998940, -0.9999080150203990547 ) ) ;
#44562=DIRECTION ( 'NONE',  ( -1.000000000000000000, 0.000000000000000000, -0.000000000000000000 ) ) ;
#44563=VECTOR ( 'NONE', #42549, 1000.000000000000000 ) ;
#44564=VERTEX_POINT ( 'NONE', #5828 ) ;
#44567=VECTOR ( 'NONE', #13127, 1000.000000000000000 ) ;
#44568=ORIENTED_EDGE ( 'NONE', *, *, #46386, .F. ) ;
#44572=CARTESIAN_POINT ( 'NONE',  ( -3.318310207868118589, 7.727984809976963909, 9.215577152005407058 ) ) ;
#44573=CARTESIAN_POINT ( 'NONE',  ( 13.39520346909927184, 10.59327504029797851, -5.642169197513929646 ) ) ;
#44574=EDGE_CURVE ( 'NONE', #52575, #1524, #17785, .T. ) ;
#44575=EDGE_LOOP ( 'NONE', ( #65642, #6809, #38396, #22908 ) ) ;
#44578=LINE ( 'NONE', #3410, #1976 ) ;
#44579=EDGE_CURVE ( 'NONE', #46339, #5624, #791, .T. ) ;
#44583=FACE_OUTER_BOUND ( 'NONE', #17843, .T. ) ;
#44584=LINE ( 'NONE', #64235, #30127 ) ;
#44585=ADVANCED_FACE ( 'NONE', ( #36382 ), #46685, .T. ) ;
#44586=CIRCLE ( 'NONE', #65806, 12.74999999999999822 ) ;
#44587=AXIS2_PLACEMENT_3D ( 'NONE', #18533, #18831, #28799 ) ;
#44589=CARTESIAN_POINT ( 'NONE',  ( 9.976349855587246296, -11.94372303670957081, -1.164441368110342490 ) ) ;
#44595=VERTEX_POINT ( 'NONE', #47671 ) ;
#44596=ORIENTED_EDGE ( 'NONE', *, *, #20034, .T. ) ;
#44597=VERTEX_POINT ( 'NONE', #47359 ) ;
#44599=AXIS2_PLACEMENT_3D ( 'NONE', #63423, #45124, #3919 ) ;
#44600=EDGE_CURVE ( 'NONE', #48767, #23964, #6456, .T. ) ;
#44601=LINE ( 'NONE', #39637, #44841 ) ;
#44604=CYLINDRICAL_SURFACE ( 'NONE', #49606, 4.999999999999999112 ) ;
#44605=AXIS2_PLACEMENT_3D ( 'NONE', #42069, #48072, #32091 ) ;
#44608=VERTEX_POINT ( 'NONE', #37021 ) ;
#44609=DIRECTION ( 'NONE',  ( -1.000000000000000000, 0.000000000000000000, 0.000000000000000000 ) ) ;
#44614=CARTESIAN_POINT ( 'NONE',  ( -35.00000000000000000, 0.000000000000000000, 0.000000000000000000 ) ) ;
#44615=ORIENTED_EDGE ( 'NONE', *, *, #20257, .F. ) ;
#44617=AXIS2_PLACEMENT_3D ( 'NONE', #10698, #25678, #23470 ) ;
#44622=DIRECTION ( 'NONE',  ( 1.000000000000000000, -0.000000000000000000, 0.000000000000000000 ) ) ;
#44623=DIRECTION ( 'NONE',  ( 0.000000000000000000, -0.01356324068817998940, 0.9999080150203990547 ) ) ;
#44624=CARTESIAN_POINT ( 'NONE',  ( -9.574630011864375234, -3.691104384415131001, -12.98917911986310081 ) ) ;
#44626=CARTESIAN_POINT ( 'NONE',  ( 10.12151447205148536, 13.48202713789778429, -0.7009852765882638170 ) ) ;
#44627=ORIENTED_EDGE ( 'NONE', *, *, #9899, .T. ) ;
#44631=LINE ( 'NONE', #59633, #45437 ) ;
#44632=ORIENTED_EDGE ( 'NONE', *, *, #6773, .T. ) ;
#44634=ORIENTED_EDGE ( 'NONE', *, *, #37619, .F. ) ;
#44635=CARTESIAN_POINT ( 'NONE',  ( -37.00000000000000711, -1.908798535168293897, -12.60630747491665282 ) ) ;
#44637=CARTESIAN_POINT ( 'NONE',  ( -47.00000000000000711, 0.000000000000000000, 0.000000000000000000 ) ) ;
#44639=CARTESIAN_POINT ( 'NONE',  ( 37.00000000000000711, 2.905556151562782574, 11.38112321385047210 ) ) ;
#44642=VECTOR ( 'NONE', #11778, 1000.000000000000000 ) ;
#44644=AXIS2_PLACEMENT_3D ( 'NONE', #2849, #7152, #2169 ) ;
#44645=DIRECTION ( 'NONE',  ( -1.000000000000000000, 0.000000000000000000, 0.000000000000000000 ) ) ;
#44647=EDGE_LOOP ( 'NONE', ( #31112, #4264, #52350, #50679 ) ) ;
#44648=DIRECTION ( 'NONE',  ( 0.000000000000000000, 0.01356324068817998940, -0.9999080150203990547 ) ) ;
#44651=EDGE_CURVE ( 'NONE', #13952, #49136, #10368, .T. ) ;
#44652=EDGE_CURVE ( 'NONE', #32109, #8260, #39944, .T. ) ;
#44653=ORIENTED_EDGE ( 'NONE', *, *, #8556, .T. ) ;
#44655=AXIS2_PLACEMENT_3D ( 'NONE', #61573, #36309, #56616 ) ;
#44656=VECTOR ( 'NONE', #55725, 1000.000000000000000 ) ;
#44659=CIRCLE ( 'NONE', #27838, 12.18649999999999878 ) ;
#44660=CARTESIAN_POINT ( 'NONE',  ( -10.90165637463000259, -7.712772661594503809, -11.08256590525389385 ) ) ;
#44661=ORIENTED_EDGE ( 'NONE', *, *, #39239, .T. ) ;
#44662=DIRECTION ( 'NONE',  ( -1.000000000000000000, 0.000000000000000000, 0.000000000000000000 ) ) ;
#44664=DIRECTION ( 'NONE',  ( 1.000000000000000000, -0.000000000000000000, 0.000000000000000000 ) ) ;
#44665=AXIS2_PLACEMENT_3D ( 'NONE', #39246, #32936, #28301 ) ;
#44666=LINE ( 'NONE', #10410, #47992 ) ;
#44667=DIRECTION ( 'NONE',  ( 0.000000000000000000, 0.01356324068817991828, -0.9999080150203990547 ) ) ;
#44668=AXIS2_PLACEMENT_3D ( 'NONE', #33926, #39902, #28953 ) ;
#44669=ORIENTED_EDGE ( 'NONE', *, *, #64731, .F. ) ;
#44670=CARTESIAN_POINT ( 'NONE',  ( 35.00000000000000000, 4.705694406421931860E-17, -3.469127814946512892E-15 ) ) ;
#44671=CARTESIAN_POINT ( 'NONE',  ( -37.00000000000000711, 9.512294188641000403, -6.891188680298720115 ) ) ;
#44672=CARTESIAN_POINT ( 'NONE',  ( 22.88594695219327235, -4.822122601967141264, 25.00000000000000000 ) ) ;
#44674=CARTESIAN_POINT ( 'NONE',  ( 8.555237949900300620, 3.417757171820648310, 13.06309840801727162 ) ) ;
#44675=VECTOR ( 'NONE', #30387, 1000.000000000000000 ) ;
#44676=DIRECTION ( 'NONE',  ( 1.000000000000000000, 0.000000000000000000, 0.000000000000000000 ) ) ;
#44677=VERTEX_POINT ( 'NONE', #58987 ) ;
#44678=EDGE_CURVE ( 'NONE', #21209, #5898, #36912, .T. ) ;
#44679=VERTEX_POINT ( 'NONE', #33016 ) ;
#44681=CARTESIAN_POINT ( 'NONE',  ( -36.00000000000000711, 6.415447294506706477, 11.01837265713075631 ) ) ;
#44682=ADVANCED_FACE ( 'NONE', ( #57991 ), #52983, .T. ) ;
#44683=CIRCLE ( 'NONE', #35140, 5.000000000000001776 ) ;
#44684=AXIS2_PLACEMENT_3D ( 'NONE', #17940, #16952, #7290 ) ;
#44689=LINE ( 'NONE', #39722, #30105 ) ;
#44690=CIRCLE ( 'NONE', #21360, 5.000000000000000888 ) ;
#44693=LINE ( 'NONE', #54040, #28721 ) ;
#44694=ORIENTED_EDGE ( 'NONE', *, *, #2841, .T. ) ;
#44696=VERTEX_POINT ( 'NONE', #37697 ) ;
#44697=CARTESIAN_POINT ( 'NONE',  ( -35.00000000000000000, 12.18632975068353019, 0.06441628369840693424 ) ) ;
#44698=ORIENTED_EDGE ( 'NONE', *, *, #8039, .T. ) ;
#44699=ORIENTED_EDGE ( 'NONE', *, *, #5818, .F. ) ;
#44701=VECTOR ( 'NONE', #885, 1000.000000000000000 ) ;
#44704=CIRCLE ( 'NONE', #12815, 12.74999999999999822 ) ;
#44705=EDGE_CURVE ( 'NONE', #12978, #8671, #17749, .T. ) ;
#44706=CARTESIAN_POINT ( 'NONE',  ( 24.07863249974178999, 1.047192704403120844, 11.95862630624809420 ) ) ;
#44709=VECTOR ( 'NONE', #28983, 1000.000000000000000 ) ;
#44710=EDGE_LOOP ( 'NONE', ( #64324, #46212, #8048, #64822 ) ) ;
#44711=CIRCLE ( 'NONE', #29855, 5.000000000000000000 ) ;
#44712=EDGE_CURVE ( 'NONE', #43321, #44959, #64576, .T. ) ;
#44713=ORIENTED_EDGE ( 'NONE', *, *, #64861, .T. ) ;
#44716=VERTEX_POINT ( 'NONE', #2804 ) ;
#44717=AXIS2_PLACEMENT_3D ( 'NONE', #34069, #29731, #64333 ) ;
#44719=EDGE_LOOP ( 'NONE', ( #20327, #25085, #30626, #62936 ) ) ;
#44723=CARTESIAN_POINT ( 'NONE',  ( -4.806344283790351390, -7.508992741355383416, 25.00000000000000000 ) ) ;
#44726=EDGE_CURVE ( 'NONE', #43974, #49728, #18886, .T. ) ;
#44728=AXIS2_PLACEMENT_3D ( 'NONE', #40557, #35873, #45227 ) ;
#44730=ADVANCED_FACE ( 'NONE', ( #12402 ), #3461, .T. ) ;
#44731=ORIENTED_EDGE ( 'NONE', *, *, #59298, .F. ) ;
#44734=FACE_OUTER_BOUND ( 'NONE', #12918, .T. ) ;
#44736=AXIS2_PLACEMENT_3D ( 'NONE', #65450, #40178, #33892 ) ;
#44737=AXIS2_PLACEMENT_3D ( 'NONE', #16781, #22425, #42047 ) ;
#44738=DIRECTION ( 'NONE',  ( 0.000000000000000000, -0.01356324068817991828, 0.9999080150203990547 ) ) ;
#44739=CIRCLE ( 'NONE', #6502, 12.75000000000000178 ) ;
#44740=DIRECTION ( 'NONE',  ( 0.000000000000000000, -0.6943713148249690548, 0.7196168960969742123 ) ) ;
#44741=EDGE_CURVE ( 'NONE', #2944, #57171, #13547, .T. ) ;
#44742=CARTESIAN_POINT ( 'NONE',  ( 6.406045832739715173, -9.118602296057780165, -9.956832946668152218 ) ) ;
#44743=DIRECTION ( 'NONE',  ( -1.000000000000000000, 0.000000000000000000, -0.000000000000000000 ) ) ;
#44744=B_SPLINE_CURVE_WITH_KNOTS ( 'NONE', 3,
 ( #41151, #25543, #45491, #51505, #64231, #15875, #5953, #19905, #60802, #15239, #51165, #65441 ),
 .UNSPECIFIED., .F., .F.,
 ( 4, 2, 2, 2, 2, 4 ),
 ( 0.005924275648040054458, 0.006464403524968336673, 0.007004531401896618888, 0.008084787155753182450, 0.009165042909609746880, 0.01024529866346631131 ),
 .UNSPECIFIED. ) ;
#44745=DIRECTION ( 'NONE',  ( 0.000000000000000000, 0.7617968321374901652, 0.6478160128811921714 ) ) ;
#44746=CARTESIAN_POINT ( 'NONE',  ( -37.00000000000000711, 11.81949347079751256, -2.968224442958276921 ) ) ;
#44747=ORIENTED_EDGE ( 'NONE', *, *, #43239, .F. ) ;
#44749=DIRECTION ( 'NONE',  ( 0.000000000000000000, -0.01356324068817998593, 0.9999080150203990547 ) ) ;
#44750=DIRECTION ( 'NONE',  ( 1.000000000000000000, 0.000000000000000000, 0.000000000000000000 ) ) ;
#44751=VECTOR ( 'NONE', #8172, 1000.000000000000000 ) ;
#44752=AXIS2_PLACEMENT_3D ( 'NONE', #21035, #41314, #27338 ) ;
#44753=CIRCLE ( 'NONE', #46914, 12.18650000000000055 ) ;
#44758=CARTESIAN_POINT ( 'NONE',  ( -35.00000000000000000, -12.08216339958899788, -1.591260454995368390 ) ) ;
#44759=AXIS2_PLACEMENT_3D ( 'NONE', #52007, #26731, #57663 ) ;
#44763=CARTESIAN_POINT ( 'NONE',  ( -28.14392221313259057, -12.90664841586573530, -3.969767364051066227 ) ) ;
#44765=DIRECTION ( 'NONE',  ( 0.000000000000000000, 0.01356324068817992175, -0.9999080150203990547 ) ) ;
#44768=B_SPLINE_CURVE_WITH_KNOTS ( 'NONE', 3,
 ( #33440, #13784, #58736, #28127, #28768, #2874, #8166, #49418, #14122, #53405, #18147, #7853, #48741, #33100, #48422, #34417, #27789, #23458, #49084, #38421, #44374, #39394, #38083, #43074, #28437, #19122, #8485, #22818 ),
 .UNSPECIFIED., .F., .F.,
 ( 4, 2, 2, 2, 2, 2, 2, 2, 2, 2, 2, 2, 2, 4 ),
 ( 0.000000000000000000, 0.001016716753235190340, 0.002033433506470380681, 0.003050150259705570587, 0.003558508636323166625, 0.004066867012940762229, 0.004575225389558358266, 0.005083583766175953436, 0.005591942142793548606, 0.006100300519411143776, 0.006608658896028738947, 0.007117017272646334117, 0.007625375649263929287, 0.008133734025881524457 ),
 .UNSPECIFIED. ) ;
#44769=CARTESIAN_POINT ( 'NONE',  ( -37.00000000000000711, -11.59095880812009582, 1.903127969211145132 ) ) ;
#44770=ORIENTED_EDGE ( 'NONE', *, *, #33030, .F. ) ;
#44772=CARTESIAN_POINT ( 'NONE',  ( -8.901467632063809532, 10.71271741810010170, -8.221947568083972868 ) ) ;
#44773=CARTESIAN_POINT ( 'NONE',  ( -35.00000000000000000, 0.000000000000000000, 0.000000000000000000 ) ) ;
#44774=DIRECTION ( 'NONE',  ( -1.000000000000000000, -0.000000000000000000, 0.000000000000000000 ) ) ;
#44780=VERTEX_POINT ( 'NONE', #29034 ) ;
#44781=AXIS2_PLACEMENT_3D ( 'NONE', #12236, #27520, #47817 ) ;
#44782=ORIENTED_EDGE ( 'NONE', *, *, #50598, .T. ) ;
#44783=CARTESIAN_POINT ( 'NONE',  ( -17.97425243782675253, -5.939124358307740437, -10.42822101977554361 ) ) ;
#44785=CIRCLE ( 'NONE', #60749, 12.74999999999999822 ) ;
#44786=CARTESIAN_POINT ( 'NONE',  ( 37.00000000000000711, 9.063649021438955344, -8.146229107149434157 ) ) ;
#44788=VECTOR ( 'NONE', #13367, 1000.000000000000000 ) ;
#44789=EDGE_CURVE ( 'NONE', #20190, #61052, #19721, .T. ) ;
#44790=CARTESIAN_POINT ( 'NONE',  ( -21.24030193723618609, 25.00000000000000000, -5.230344621181295395 ) ) ;
#44792=DIRECTION ( 'NONE',  ( 0.000000000000000000, -0.01356324068817992175, 0.9999080150203990547 ) ) ;
#44793=CARTESIAN_POINT ( 'NONE',  ( 12.90485164427657239, 10.90052374342006303, -5.021923595418537722 ) ) ;
#44795=CARTESIAN_POINT ( 'NONE',  ( 22.88594695219327235, -4.822122601967141264, 12.60940655271284427 ) ) ;
#44798=DIRECTION ( 'NONE',  ( -0.000000000000000000, -1.000000000000000000, -0.000000000000000000 ) ) ;
#44799=EDGE_CURVE ( 'NONE', #30305, #53784, #12982, .T. ) ;
#44806=FACE_OUTER_BOUND ( 'NONE', #57501, .T. ) ;
#44807=VECTOR ( 'NONE', #60147, 1000.000000000000000 ) ;
#44809=DIRECTION ( 'NONE',  ( 1.000000000000000000, 0.000000000000000000, 0.000000000000000000 ) ) ;
#44810=VECTOR ( 'NONE', #56644, 1000.000000000000000 ) ;
#44811=CARTESIAN_POINT ( 'NONE',  ( -35.00000000000000000, 5.636262487437317503, 10.80478261802183937 ) ) ;
#44815=DIRECTION ( 'NONE',  ( 0.000000000000000000, 0.9551603052523468529, -0.2960891610144544828 ) ) ;
#44816=VECTOR ( 'NONE', #45294, 1000.000000000000000 ) ;
#44817=DIRECTION ( 'NONE',  ( 0.000000000000000000, -0.9999080150203990547, -0.01356324068816951688 ) ) ;
#44818=ADVANCED_FACE ( 'NONE', ( #60260 ), #4085, .T. ) ;
#44819=CARTESIAN_POINT ( 'NONE',  ( 35.00000000000000000, 4.705694406421931860E-17, -3.469127814946512892E-15 ) ) ;
#44820=CARTESIAN_POINT ( 'NONE',  ( 11.74548640120467979, 10.73597826697114677, -8.184666801472349817 ) ) ;
#44821=CARTESIAN_POINT ( 'NONE',  ( 24.35372750138188991, -1.446416020193747931, 13.42696394628527479 ) ) ;
#44822=DIRECTION ( 'NONE',  ( -1.000000000000000000, -0.000000000000000000, 0.000000000000000000 ) ) ;
#44826=EDGE_CURVE ( 'NONE', #1597, #62432, #22049, .T. ) ;
#44827=VERTEX_POINT ( 'NONE', #25025 ) ;
#44829=EDGE_CURVE ( 'NONE', #61242, #11917, #12498, .T. ) ;
#44830=AXIS2_PLACEMENT_3D ( 'NONE', #1588, #31803, #7528 ) ;
#44831=ORIENTED_EDGE ( 'NONE', *, *, #40900, .F. ) ;
#44832=CARTESIAN_POINT ( 'NONE',  ( -3.433867940172757649, -8.302961779614593141, 8.673267303339269318 ) ) ;
#44834=DIRECTION ( 'NONE',  ( 0.000000000000000000, 0.01356324068817998940, -0.9999080150203989437 ) ) ;
#44835=EDGE_CURVE ( 'NONE', #63621, #13407, #64526, .T. ) ;
#44839=CARTESIAN_POINT ( 'NONE',  ( 35.00000000000000000, 4.705694406421931860E-17, -3.469127814946512892E-15 ) ) ;
#44841=VECTOR ( 'NONE', #14358, 1000.000000000000000 ) ;
#44842=DIRECTION ( 'NONE',  ( 0.000000000000000000, 0.01356324068818000848, -0.9999080150203990547 ) ) ;
#44845=AXIS2_PLACEMENT_3D ( 'NONE', #25522, #10546, #50803 ) ;
#44846=CARTESIAN_POINT ( 'NONE',  ( -35.00000000000000000, 0.4353888892048373149, 11.73808581813438323 ) ) ;
#44847=( BOUNDED_CURVE ( )  B_SPLINE_CURVE ( 3, ( #8781, #8127, #28395, #43350 ),
 .UNSPECIFIED., .F., .F. ) 
 B_SPLINE_CURVE_WITH_KNOTS ( ( 4, 4 ),
 ( 5.064515163936929909, 5.083794169102955784 ),
 .UNSPECIFIED. ) 
 CURVE ( )  GEOMETRIC_REPRESENTATION_ITEM ( )  RATIONAL_B_SPLINE_CURVE ( ( 1.000000000000000000, 0.9999690269031535905, 0.9999690269031535905, 1.000000000000000000 ) ) 
 REPRESENTATION_ITEM ( '' )  );
#44848=VERTEX_POINT ( 'NONE', #45298 ) ;
#44850=B_SPLINE_CURVE_WITH_KNOTS ( 'NONE', 3,
 ( #59115, #59416, #49469, #24166, #34772, #30144, #28834, #19179, #50109, #55413, #43802, #3601, #29471, #39452, #59754, #13839 ),
 .UNSPECIFIED., .F., .F.,
 ( 4, 2, 2, 2, 2, 2, 2, 4 ),
 ( 0.000000000000000000, 0.001179563962946403180, 0.001769345944419603144, 0.002359127925892802891, 0.003538691888839202819, 0.004718255851785603180, 0.007077383777678405638, 0.009436511703571208096 ),
 .UNSPECIFIED. ) ;
#44851=ORIENTED_EDGE ( 'NONE', *, *, #20493, .F. ) ;
#44853=CARTESIAN_POINT ( 'NONE',  ( 35.00000000000000000, -1.113475361586580226, -12.70128625845192438 ) ) ;
#44855=AXIS2_PLACEMENT_3D ( 'NONE', #31142, #24850, #56407 ) ;
#44859=ORIENTED_EDGE ( 'NONE', *, *, #54760, .F. ) ;
#44860=DIRECTION ( 'NONE',  ( 1.000000000000000000, -0.000000000000000000, 0.000000000000000000 ) ) ;
#44861=VERTEX_POINT ( 'NONE', #40292 ) ;
#44862=CARTESIAN_POINT ( 'NONE',  ( 12.47628546223243617, 0.000000000000000000, -13.50000000000000178 ) ) ;
#44863=CARTESIAN_POINT ( 'NONE',  ( 35.00000000000000000, -11.13736569743270621, 4.946702696913284569 ) ) ;
#44865=CARTESIAN_POINT ( 'NONE',  ( -37.00000000000000711, 0.000000000000000000, 0.000000000000000000 ) ) ;
#44867=CARTESIAN_POINT ( 'NONE',  ( 36.00000000000000711, 12.38385022362086119, 3.033604067594442899 ) ) ;
#44869=VERTEX_POINT ( 'NONE', #10054 ) ;
#44870=EDGE_CURVE ( 'NONE', #57900, #6726, #30336, .T. ) ;
#44873=CARTESIAN_POINT ( 'NONE',  ( 0.09505445835107226293, -0.1369421331495649097, 13.50000000000000355 ) ) ;
#44874=DIRECTION ( 'NONE',  ( 0.000000000000000000, 0.7381862504171974315, -0.6745969609292639113 ) ) ;
#44878=CIRCLE ( 'NONE', #16214, 4.999999999999999112 ) ;
#44879=FACE_BOUND ( 'NONE', #49171, .T. ) ;
#44880=ORIENTED_EDGE ( 'NONE', *, *, #43009, .T. ) ;
#44881=LINE ( 'NONE', #49880, #44978 ) ;
#44885=ORIENTED_EDGE ( 'NONE', *, *, #60542, .F. ) ;
#44888=ADVANCED_FACE ( 'NONE', ( #3006 ), #49539, .T. ) ;
#44889=ORIENTED_EDGE ( 'NONE', *, *, #49272, .T. ) ;
#44890=CARTESIAN_POINT ( 'NONE',  ( -36.00000000000000711, -11.90598845858530730, -4.561791185930541559 ) ) ;
#44891=EDGE_LOOP ( 'NONE', ( #2814, #1432, #24111, #18096 ) ) ;
#44892=AXIS2_PLACEMENT_3D ( 'NONE', #6429, #36993, #57299 ) ;
#44895=ORIENTED_EDGE ( 'NONE', *, *, #19514, .F. ) ;
#44896=CYLINDRICAL_SURFACE ( 'NONE', #56364, 5.000000000000000000 ) ;
#44898=AXIS2_PLACEMENT_3D ( 'NONE', #49939, #43970, #19361 ) ;
#44899=CARTESIAN_POINT ( 'NONE',  ( -35.00000000000000000, 7.718225330433806874, 9.430788938294076829 ) ) ;
#44900=DIRECTION ( 'NONE',  ( 0.000000000000000000, -0.01356324068817991828, 0.9999080150203990547 ) ) ;
#44901=VERTEX_POINT ( 'NONE', #44200 ) ;
#44902=DIRECTION ( 'NONE',  ( -1.000000000000000000, -0.000000000000000000, 0.000000000000000000 ) ) ;
#44903=ORIENTED_EDGE ( 'NONE', *, *, #40785, .F. ) ;
#44904=DIRECTION ( 'NONE',  ( 0.000000000000000000, 0.6943713148249639477, -0.7196168960969794304 ) ) ;
#44905=CARTESIAN_POINT ( 'NONE',  ( -37.00000000000000711, -8.295159312811792418, -8.927548052240984688 ) ) ;
#44906=ORIENTED_EDGE ( 'NONE', *, *, #63377, .T. ) ;
#44908=FACE_OUTER_BOUND ( 'NONE', #49624, .T. ) ;
#44909=DIRECTION ( 'NONE',  ( -0.7648446667472313942, 0.000000000000000000, 0.6442147435043042991 ) ) ;
#44910=EDGE_CURVE ( 'NONE', #53880, #42172, #49685, .T. ) ;
#44911=EDGE_LOOP ( 'NONE', ( #15646, #32680, #31525, #7453 ) ) ;
#44912=CIRCLE ( 'NONE', #42760, 12.18649999999999878 ) ;
#44913=ORIENTED_EDGE ( 'NONE', *, *, #22422, .T. ) ;
#44916=ORIENTED_EDGE ( 'NONE', *, *, #64686, .T. ) ;
#44918=CARTESIAN_POINT ( 'NONE',  ( 37.00000000000000711, 4.705694406421931860E-17, -3.469127814946512892E-15 ) ) ;
#44922=LINE ( 'NONE', #61201, #11772 ) ;
#44923=CARTESIAN_POINT ( 'NONE',  ( 13.40637569210417368, 10.89743038486300719, -5.029693541956189229 ) ) ;
#44925=CARTESIAN_POINT ( 'NONE',  ( -37.00000000000000711, 0.000000000000000000, 0.000000000000000000 ) ) ;
#44930=CARTESIAN_POINT ( 'NONE',  ( 37.00000000000000711, 4.705694406421931860E-17, -3.469127814946512892E-15 ) ) ;
#44933=LINE ( 'NONE', #19351, #29000 ) ;
#44936=CIRCLE ( 'NONE', #16280, 5.000000000000001776 ) ;
#44937=AXIS2_PLACEMENT_3D ( 'NONE', #27207, #47500, #57817 ) ;
#44938=EDGE_CURVE ( 'NONE', #61338, #95, #33720, .T. ) ;
#44939=ORIENTED_EDGE ( 'NONE', *, *, #24942, .F. ) ;
#44940=DIRECTION ( 'NONE',  ( -1.000000000000000000, 0.000000000000000000, 0.000000000000000000 ) ) ;
#44942=VERTEX_POINT ( 'NONE', #38562 ) ;
#44943=CARTESIAN_POINT ( 'NONE',  ( 35.00000000000000000, 11.72195762423409704, 0.7536123767498881243 ) ) ;
#44946=VECTOR ( 'NONE', #13994, 1000.000000000000000 ) ;
#44947=CARTESIAN_POINT ( 'NONE',  ( -37.00000000000000711, 0.000000000000000000, 0.000000000000000000 ) ) ;
#44949=AXIS2_PLACEMENT_3D ( 'NONE', #5271, #10908, #60799 ) ;
#44952=ORIENTED_EDGE ( 'NONE', *, *, #61557, .F. ) ;
#44953=CARTESIAN_POINT ( 'NONE',  ( 29.39893672795668778, -9.588109978674381750, 7.219804916327976052 ) ) ;
#44956=CARTESIAN_POINT ( 'NONE',  ( 35.00000000000000000, -3.916263239775270577, 11.07407352312216453 ) ) ;
#44957=DIRECTION ( 'NONE',  ( 0.000000000000000000, -0.01356324068818000328, 0.9999080150203990547 ) ) ;
#44958=LINE ( 'NONE', #24341, #46073 ) ;
#44959=VERTEX_POINT ( 'NONE', #13923 ) ;
#44961=DIRECTION ( 'NONE',  ( 1.000000000000000000, -0.000000000000000000, 0.000000000000000000 ) ) ;
#44964=DIRECTION ( 'NONE',  ( 0.000000000000000000, 0.1118654143051546757, 0.9937233664769770103 ) ) ;
#44966=ORIENTED_EDGE ( 'NONE', *, *, #6269, .T. ) ;
#44970=ORIENTED_EDGE ( 'NONE', *, *, #36785, .F. ) ;
#44972=ORIENTED_EDGE ( 'NONE', *, *, #7345, .T. ) ;
#44973=DIRECTION ( 'NONE',  ( -0.6845106172691086677, 0.000000000000000000, -0.7290028908350527637 ) ) ;
#44974=DIRECTION ( 'NONE',  ( -1.000000000000000000, 0.000000000000000000, -0.000000000000000000 ) ) ;
#44975=EDGE_CURVE ( 'NONE', #58033, #49868, #2955, .T. ) ;
#44976=DIRECTION ( 'NONE',  ( 1.000000000000000000, 0.000000000000000000, 0.000000000000000000 ) ) ;
#44977=DIRECTION ( 'NONE',  ( 1.000000000000000000, 0.000000000000000000, 0.000000000000000000 ) ) ;
#44978=VECTOR ( 'NONE', #3365, 1000.000000000000000 ) ;
#44979=CYLINDRICAL_SURFACE ( 'NONE', #43118, 4.999999999999999112 ) ;
#44982=CARTESIAN_POINT ( 'NONE',  ( 35.00000000000000000, -4.545979934229326780, 11.30684963584393543 ) ) ;
#44983=CARTESIAN_POINT ( 'NONE',  ( 35.00000000000000000, 3.916263239775349625, -11.07407352312214144 ) ) ;
#44984=VERTEX_POINT ( 'NONE', #54473 ) ;
#44986=CARTESIAN_POINT ( 'NONE',  ( 13.41004496935349799, -12.48441396568899187, -5.141889352316721506 ) ) ;
#44987=VERTEX_POINT ( 'NONE', #2644 ) ;
#44988=B_SPLINE_CURVE_WITH_KNOTS ( 'NONE', 3,
 ( #6275, #946, #61139, #42140, #6603, #26219, #21214, #5629, #41834, #62122, #41162, #41488, #35833, #11567, #20583, #11254, #16240, #31841, #1621, #61783, #56134, #56475, #630, #56830 ),
 .UNSPECIFIED., .F., .F.,
 ( 4, 2, 2, 2, 2, 2, 2, 2, 2, 2, 2, 4 ),
 ( 2.637977740025101358E-18, 0.001239215294917696492, 0.001858822942376543328, 0.002478430589835390382, 0.003717645884753084055, 0.004337253532211930891, 0.004956861179670778161, 0.005576468827129624564, 0.006196076474588470100, 0.007435291769506157701, 0.008674507064423846170, 0.009913722359341532037 ),
 .UNSPECIFIED. ) ;
#44989=AXIS2_PLACEMENT_3D ( 'NONE', #39800, #59426, #49477 ) ;
#44990=ORIENTED_EDGE ( 'NONE', *, *, #25008, .F. ) ;
#44992=AXIS2_PLACEMENT_3D ( 'NONE', #35640, #44977, #19725 ) ;
#44994=DIRECTION ( 'NONE',  ( 0.000000000000000000, 0.6745969609292609137, 0.7381862504172000961 ) ) ;
#44995=CARTESIAN_POINT ( 'NONE',  ( 35.00000000000000000, -8.573591947375261313, 8.029056188533775895 ) ) ;
#44997=EDGE_CURVE ( 'NONE', #7860, #16892, #50735, .T. ) ;
#44998=CIRCLE ( 'NONE', #59858, 5.000000000000001776 ) ;
#44999=CARTESIAN_POINT ( 'NONE',  ( 36.00000000000000711, 0.9416912585476251429, 12.71517666308946382 ) ) ;
#45000=LINE ( 'NONE', #24067, #50386 ) ;
#45002=AXIS2_PLACEMENT_3D ( 'NONE', #53461, #1367, #51906 ) ;
#45005=AXIS2_PLACEMENT_3D ( 'NONE', #41137, #20213, #40489 ) ;
#45007=CARTESIAN_POINT ( 'NONE',  ( -18.51542011345573613, -4.386464785673767075, 12.76797095508238300 ) ) ;
#45009=AXIS2_PLACEMENT_3D ( 'NONE', #45633, #40650, #15381 ) ;
#45010=AXIS2_PLACEMENT_3D ( 'NONE', #50033, #60322, #24760 ) ;
#45014=FACE_OUTER_BOUND ( 'NONE', #32762, .T. ) ;
#45018=CARTESIAN_POINT ( 'NONE',  ( 37.00000000000000711, 4.705694406421931860E-17, -3.469127814946512892E-15 ) ) ;
#45023=ORIENTED_EDGE ( 'NONE', *, *, #21816, .T. ) ;
#45024=DIRECTION ( 'NONE',  ( 1.000000000000000000, -0.000000000000000000, 0.000000000000000000 ) ) ;
#45026=DIRECTION ( 'NONE',  ( 0.000000000000000000, -0.01356324068817998940, 0.9999080150203990547 ) ) ;
#45027=ORIENTED_EDGE ( 'NONE', *, *, #62909, .F. ) ;
#45029=CARTESIAN_POINT ( 'NONE',  ( -37.00000000000000711, 0.000000000000000000, 0.000000000000000000 ) ) ;
#45030=ORIENTED_EDGE ( 'NONE', *, *, #5870, .T. ) ;
#45032=CIRCLE ( 'NONE', #14215, 12.74999999999999822 ) ;
#45033=ORIENTED_EDGE ( 'NONE', *, *, #9137, .T. ) ;
#45035=EDGE_CURVE ( 'NONE', #47412, #20061, #35836, .T. ) ;
#45039=SHAPE_REPRESENTATION ( 'tweezer drum assembly', ( #24966 ), #7986 ) ;
#45040=DIRECTION ( 'NONE',  ( -1.000000000000000000, 0.000000000000000000, -0.000000000000000000 ) ) ;
#45041=DIRECTION ( 'NONE',  ( -1.000000000000000000, 0.000000000000000000, 0.000000000000000000 ) ) ;
#45042=AXIS2_PLACEMENT_3D ( 'NONE', #33475, #29147, #64369 ) ;
#45046=ORIENTED_EDGE ( 'NONE', *, *, #6986, .F. ) ;
#45047=DIRECTION ( 'NONE',  ( 1.000000000000000000, -0.000000000000000000, 0.000000000000000000 ) ) ;
#45050=CARTESIAN_POINT ( 'NONE',  ( 37.00000000000000711, 11.47758908105697806, 2.497432891016712286 ) ) ;
#45051=AXIS2_PLACEMENT_3D ( 'NONE', #65094, #54491, #23574 ) ;
#45052=ORIENTED_EDGE ( 'NONE', *, *, #13889, .T. ) ;
#45056=EDGE_CURVE ( 'NONE', #58885, #16670, #20998, .T. ) ;
#45057=AXIS2_PLACEMENT_3D ( 'NONE', #47710, #46721, #2154 ) ;
#45060=DIRECTION ( 'NONE',  ( 0.000000000000000000, -0.9467777615094538080, -0.3218879778916074463 ) ) ;
#45061=DIRECTION ( 'NONE',  ( 1.000000000000000000, 0.000000000000000000, 0.000000000000000000 ) ) ;
#45062=ORIENTED_EDGE ( 'NONE', *, *, #61498, .T. ) ;
#45064=ORIENTED_EDGE ( 'NONE', *, *, #21202, .F. ) ;
#45065=LINE ( 'NONE', #35054, #65590 ) ;
#45068=B_SPLINE_CURVE_WITH_KNOTS ( 'NONE', 3,
 ( #47896, #38221, #17644, #33249, #21389, #46657, #56979, #16061, #48252, #63489 ),
 .UNSPECIFIED., .F., .F.,
 ( 4, 2, 2, 2, 4 ),
 ( 0.000000000000000000, 0.001114213790187107336, 0.002228427580374214671, 0.003342641370561322007, 0.004456855160748429343 ),
 .UNSPECIFIED. ) ;
#45072=B_SPLINE_CURVE_WITH_KNOTS ( 'NONE', 3,
 ( #49153, #3918, #39136, #23878, #59429, #8894, #40110, #59766 ),
 .UNSPECIFIED., .F., .F.,
 ( 4, 2, 2, 4 ),
 ( 0.000000000000000000, 0.002717879308656051540, 0.004076818962984075576, 0.005435758617312099611 ),
 .UNSPECIFIED. ) ;
#45074=DIRECTION ( 'NONE',  ( 0.000000000000000000, 0.8369827122275362852, 0.5472293298355244140 ) ) ;
#45076=CARTESIAN_POINT ( 'NONE',  ( -11.37391343693395562, -6.796058610810909784, -9.899934513732258523 ) ) ;
#45078=CARTESIAN_POINT ( 'NONE',  ( -37.00000000000000711, -9.217970097227665249, -7.971186206369574201 ) ) ;
#45079=ORIENTED_EDGE ( 'NONE', *, *, #53569, .F. ) ;
#45080=VERTEX_POINT ( 'NONE', #30482 ) ;
#45082=AXIS2_PLACEMENT_3D ( 'NONE', #22804, #43058, #3179 ) ;
#45083=DIRECTION ( 'NONE',  ( 1.000000000000000000, 0.000000000000000000, 0.000000000000000000 ) ) ;
#45084=CIRCLE ( 'NONE', #14266, 5.000000000000000888 ) ;
#45085=CYLINDRICAL_SURFACE ( 'NONE', #43618, 12.75000000000000178 ) ;
#45086=EDGE_CURVE ( 'NONE', #41139, #27477, #32655, .T. ) ;
#45087=CARTESIAN_POINT ( 'NONE',  ( 6.800436580320503133, -6.134824022537911148, 10.31531696979683410 ) ) ;
#45090=CARTESIAN_POINT ( 'NONE',  ( -10.60692174091447981, -5.627218222672255798, -10.60063337488197632 ) ) ;
#45092=CYLINDRICAL_SURFACE ( 'NONE', #32192, 5.000000000000000888 ) ;
#45094=ORIENTED_EDGE ( 'NONE', *, *, #7883, .F. ) ;
#45101=CYLINDRICAL_SURFACE ( 'NONE', #41458, 12.18649999999999878 ) ;
#45102=EDGE_CURVE ( 'NONE', #44008, #33918, #19812, .T. ) ;
#45103=EDGE_LOOP ( 'NONE', ( #54240, #37720, #63595, #63889 ) ) ;
#45104=EDGE_CURVE ( 'NONE', #17490, #6738, #40124, .T. ) ;
#45105=CARTESIAN_POINT ( 'NONE',  ( -8.891032880924177206, 12.93614229090409395, -3.860857758255646921 ) ) ;
#45109=EDGE_CURVE ( 'NONE', #64126, #54960, #842, .T. ) ;
#45110=FACE_OUTER_BOUND ( 'NONE', #3590, .T. ) ;
#45111=CARTESIAN_POINT ( 'NONE',  ( 35.00000000000000000, -3.805206332242389244, 12.16893194857553340 ) ) ;
#45112=CARTESIAN_POINT ( 'NONE',  ( -35.00000000000000000, -4.545979934229492869, 11.30684963584387681 ) ) ;
#45114=DIRECTION ( 'NONE',  ( -1.000000000000000000, 0.000000000000000000, 0.000000000000000000 ) ) ;
#45116=LINE ( 'NONE', #9510, #4293 ) ;
#45120=CARTESIAN_POINT ( 'NONE',  ( -32.00000000000000000, 5.510910596163098430E-16, 0.000000000000000000 ) ) ;
#45121=CYLINDRICAL_SURFACE ( 'NONE', #36127, 12.75000000000000178 ) ;
#45124=DIRECTION ( 'NONE',  ( -1.000000000000000000, -1.836970198721029688E-16, -0.000000000000000000 ) ) ;
#45126=CIRCLE ( 'NONE', #47282, 5.000000000000000000 ) ;
#45127=ORIENTED_EDGE ( 'NONE', *, *, #13774, .T. ) ;
#45129=ORIENTED_EDGE ( 'NONE', *, *, #17329, .T. ) ;
#45132=EDGE_CURVE ( 'NONE', #40821, #35283, #17654, .T. ) ;
#45133=FACE_OUTER_BOUND ( 'NONE', #11278, .T. ) ;
#45136=VECTOR ( 'NONE', #18928, 1000.000000000000000 ) ;
#45138=FACE_OUTER_BOUND ( 'NONE', #48276, .T. ) ;
#45140=VERTEX_POINT ( 'NONE', #30797 ) ;
#45141=CARTESIAN_POINT ( 'NONE',  ( 37.00000000000000711, 1.456211999474505969, 11.65554240571055011 ) ) ;
#45143=CARTESIAN_POINT ( 'NONE',  ( 37.00000000000000711, -8.699265615723044576, -8.534258022646067587 ) ) ;
#45146=AXIS2_PLACEMENT_3D ( 'NONE', #61237, #49957, #44964 ) ;
#45148=CARTESIAN_POINT ( 'NONE',  ( -7.287102677926679206, 8.374986170366049976, -10.59034548381062102 ) ) ;
#45150=CARTESIAN_POINT ( 'NONE',  ( -35.00000000000000000, 11.67026961469348123, 4.564151185897115326 ) ) ;
#45151=ORIENTED_EDGE ( 'NONE', *, *, #40451, .F. ) ;
#45152=CARTESIAN_POINT ( 'NONE',  ( -37.00000000000000711, 0.000000000000000000, 0.000000000000000000 ) ) ;
#45156=CARTESIAN_POINT ( 'NONE',  ( -20.34436657951988181, 13.27874470876743729, -2.506383895450033261 ) ) ;
#45158=DIRECTION ( 'NONE',  ( 1.000000000000000000, 0.000000000000000000, 0.000000000000000000 ) ) ;
#45160=DIRECTION ( 'NONE',  ( 0.000000000000000000, 0.8009703041134145218, 0.5987040770935704304 ) ) ;
#45161=EDGE_CURVE ( 'NONE', #22647, #11898, #24859, .T. ) ;
#45162=AXIS2_PLACEMENT_3D ( 'NONE', #23678, #3405, #7718 ) ;
#45163=VERTEX_POINT ( 'NONE', #15515 ) ;
#45165=ORIENTED_EDGE ( 'NONE', *, *, #13311, .T. ) ;
#45168=DIRECTION ( 'NONE',  ( -1.000000000000000000, -0.000000000000000000, 0.000000000000000000 ) ) ;
#45175=CYLINDRICAL_SURFACE ( 'NONE', #16810, 12.74999999999999822 ) ;
#45179=ORIENTED_EDGE ( 'NONE', *, *, #26941, .F. ) ;
#45180=EDGE_CURVE ( 'NONE', #33526, #23975, #37903, .T. ) ;
#45181=DIRECTION ( 'NONE',  ( 0.000000000000000000, -0.2355298848897586228, -0.9718671068226442111 ) ) ;
#45182=VERTEX_POINT ( 'NONE', #34797 ) ;
#45186=CARTESIAN_POINT ( 'NONE',  ( -7.181456785175555524, -5.890186129966251904, -10.45493698471458188 ) ) ;
#45187=DIRECTION ( 'NONE',  ( 0.000000000000000000, -0.01356324068817991307, 0.9999080150203990547 ) ) ;
#45188=CIRCLE ( 'NONE', #44100, 12.75000000000000178 ) ;
#45190=EDGE_CURVE ( 'NONE', #19934, #45235, #22148, .T. ) ;
#45193=ORIENTED_EDGE ( 'NONE', *, *, #10570, .F. ) ;
#45194=CARTESIAN_POINT ( 'NONE',  ( -37.00000000000000711, -8.766823244862047559, 7.817610399097479679 ) ) ;
#45195=CARTESIAN_POINT ( 'NONE',  ( 36.00000000000000711, 7.094637218249506994, 10.59380114696461916 ) ) ;
#45197=DIRECTION ( 'NONE',  ( -1.000000000000000000, 0.000000000000000000, 0.000000000000000000 ) ) ;
#45198=DIRECTION ( 'NONE',  ( 0.000000000000000000, 0.01356324068817998940, -0.9999080150203989437 ) ) ;
#45199=ADVANCED_FACE ( 'NONE', ( #52437 ), #51774, .T. ) ;
#45200=LINE ( 'NONE', #23041, #22172 ) ;
#45201=FACE_OUTER_BOUND ( 'NONE', #17292, .T. ) ;
#45202=ORIENTED_EDGE ( 'NONE', *, *, #21248, .T. ) ;
#45203=CARTESIAN_POINT ( 'NONE',  ( -8.841892098821560353, -8.618917129353741657, -8.357420571532406584 ) ) ;
#45204=VERTEX_POINT ( 'NONE', #1229 ) ;
#45205=ORIENTED_EDGE ( 'NONE', *, *, #46205, .F. ) ;
#45208=AXIS2_PLACEMENT_3D ( 'NONE', #23333, #47954, #48617 ) ;
#45210=ORIENTED_EDGE ( 'NONE', *, *, #26458, .T. ) ;
#45213=ORIENTED_EDGE ( 'NONE', *, *, #33284, .F. ) ;
#45215=DIRECTION ( 'NONE',  ( -1.000000000000000000, 0.000000000000000000, 0.000000000000000000 ) ) ;
#45216=CARTESIAN_POINT ( 'NONE',  ( 17.11285760380292231, 10.50878607827772804, 5.793619504978376078 ) ) ;
#45218=ORIENTED_EDGE ( 'NONE', *, *, #9075, .F. ) ;
#45219=VERTEX_POINT ( 'NONE', #62371 ) ;
#45220=EDGE_CURVE ( 'NONE', #57171, #29799, #6544, .T. ) ;
#45222=EDGE_LOOP ( 'NONE', ( #41879, #52156, #19264, #3856 ) ) ;
#45226=VERTEX_POINT ( 'NONE', #6876 ) ;
#45227=DIRECTION ( 'NONE',  ( 0.000000000000000000, -0.01356324068817998940, 0.9999080150203990547 ) ) ;
#45229=DIRECTION ( 'NONE',  ( 1.000000000000000000, 0.000000000000000000, 0.000000000000000000 ) ) ;
#45231=ORIENTED_EDGE ( 'NONE', *, *, #38814, .F. ) ;
#45232=AXIS2_PLACEMENT_3D ( 'NONE', #16753, #62616, #12406 ) ;
#45233=DIRECTION ( 'NONE',  ( -1.000000000000000000, 0.000000000000000000, -0.000000000000000000 ) ) ;
#45234=CIRCLE ( 'NONE', #16521, 4.999999999999999112 ) ;
#45235=VERTEX_POINT ( 'NONE', #888 ) ;
#45236=CARTESIAN_POINT ( 'NONE',  ( 37.00000000000000711, -12.18359334611896472, -0.2661492558802951991 ) ) ;
#45242=VECTOR ( 'NONE', #5406, 1000.000000000000000 ) ;
#45243=EDGE_CURVE ( 'NONE', #21897, #54995, #10272, .T. ) ;
#45245=EDGE_LOOP ( 'NONE', ( #24423, #38589, #36736, #15393 ) ) ;
#45247=( BOUNDED_CURVE ( )  B_SPLINE_CURVE ( 3, ( #56662, #21392, #48255, #27595 ),
 .UNSPECIFIED., .F., .F. ) 
 B_SPLINE_CURVE_WITH_KNOTS ( ( 4, 4 ),
 ( 1.289813438233471610, 1.322487409060285168 ),
 .UNSPECIFIED. ) 
 CURVE ( )  GEOMETRIC_REPRESENTATION_ITEM ( )  RATIONAL_B_SPLINE_CURVE ( ( 1.000000000000000000, 0.9999110362812402286, 0.9999110362812402286, 1.000000000000000000 ) ) 
 REPRESENTATION_ITEM ( '' )  );
#45249=CARTESIAN_POINT ( 'NONE',  ( -24.35967074841363456, -9.892812110492778643, 9.188125470810931006 ) ) ;
#45253=DIRECTION ( 'NONE',  ( 0.000000000000000000, 0.01356324068817999114, -0.9999080150203989437 ) ) ;
#45254=ORIENTED_EDGE ( 'NONE', *, *, #38899, .T. ) ;
#45256=CARTESIAN_POINT ( 'NONE',  ( -17.54726996257253191, -11.36053454945672136, 3.865003848717349033 ) ) ;
#45258=DIRECTION ( 'NONE',  ( -1.000000000000000000, 0.000000000000000000, 0.000000000000000000 ) ) ;
#45259=DIRECTION ( 'NONE',  ( -0.000000000000000000, -0.000000000000000000, -1.000000000000000000 ) ) ;
#45260=EDGE_CURVE ( 'NONE', #41945, #24950, #45420, .T. ) ;
#45263=ADVANCED_FACE ( 'NONE', ( #53417 ), #64025, .T. ) ;
#45265=DIRECTION ( 'NONE',  ( 0.000000000000000000, -0.01356324068817991828, 0.9999080150203990547 ) ) ;
#45266=CARTESIAN_POINT ( 'NONE',  ( -35.00000000000000000, -11.42599468261432527, 4.237620530777758354 ) ) ;
#45277=VERTEX_POINT ( 'NONE', #2882 ) ;
#45278=ADVANCED_FACE ( 'NONE', ( #7505 ), #38767, .T. ) ;
#45280=VERTEX_POINT ( 'NONE', #2556 ) ;
#45283=ORIENTED_EDGE ( 'NONE', *, *, #28993, .T. ) ;
#45284=EDGE_CURVE ( 'NONE', #25983, #31872, #29402, .T. ) ;
#45285=FACE_OUTER_BOUND ( 'NONE', #56766, .T. ) ;
#45290=FACE_OUTER_BOUND ( 'NONE', #7395, .T. ) ;
#45292=ORIENTED_EDGE ( 'NONE', *, *, #61867, .F. ) ;
#45293=EDGE_CURVE ( 'NONE', #54568, #1623, #3936, .T. ) ;
#45294=DIRECTION ( 'NONE',  ( 1.000000000000000000, -0.000000000000000000, -0.000000000000000000 ) ) ;
#45296=CARTESIAN_POINT ( 'NONE',  ( 35.00000000000000000, -2.627174906296994905, -11.44858830469739530 ) ) ;
#45298=CARTESIAN_POINT ( 'NONE',  ( 35.00000000000000000, 12.71517666308947803, -0.9416912585474880304 ) ) ;
#45300=DIRECTION ( 'NONE',  ( -1.000000000000000000, 0.000000000000000000, -0.000000000000000000 ) ) ;
#45305=CARTESIAN_POINT ( 'NONE',  ( 35.00000000000000000, 8.052525312709883920, -8.551552972817113130 ) ) ;
#45306=DIRECTION ( 'NONE',  ( -0.000000000000000000, -0.000000000000000000, -1.000000000000000000 ) ) ;
#45307=CARTESIAN_POINT ( 'NONE',  ( 12.32157157451222496, 13.32610988528976570, -2.183319616765905025 ) ) ;
#45308=ORIENTED_EDGE ( 'NONE', *, *, #62250, .F. ) ;
#45309=FACE_OUTER_BOUND ( 'NONE', #17896, .T. ) ;
#45310=ORIENTED_EDGE ( 'NONE', *, *, #56243, .T. ) ;
#45311=CARTESIAN_POINT ( 'NONE',  ( 37.00000000000000711, 4.705694406421931860E-17, -3.469127814946512892E-15 ) ) ;
#45312=EDGE_LOOP ( 'NONE', ( #13149, #23360, #36001, #51534 ) ) ;
#45314=CARTESIAN_POINT ( 'NONE',  ( 24.90014556888634800, 8.538933172091805801, -8.433831666448901032 ) ) ;
#45318=CARTESIAN_POINT ( 'NONE',  ( -37.00000000000000711, 0.4353888892048373149, 11.73808581813438323 ) ) ;
#45321=AXIS2_PLACEMENT_3D ( 'NONE', #31613, #40951, #25657 ) ;
#45323=EDGE_CURVE ( 'NONE', #48416, #42832, #3545, .T. ) ;
#45324=ORIENTED_EDGE ( 'NONE', *, *, #29442, .T. ) ;
#45326=DIRECTION ( 'NONE',  ( 1.000000000000000000, -0.000000000000000000, 0.000000000000000000 ) ) ;
#45330=B_SPLINE_CURVE_WITH_KNOTS ( 'NONE', 3,
 ( #22396, #37705, #18426, #37362, #27383, #47678, #42660, #32678, #52991, #2473, #43012, #17756, #58318, #38013, #4776, #65568, #45307, #54659, #64278, #29666, #28698, #54323, #64584, #44626, #30008, #3470 ),
 .UNSPECIFIED., .F., .F.,
 ( 4, 2, 2, 2, 2, 2, 2, 2, 2, 2, 2, 2, 4 ),
 ( 0.000000000000000000, 0.001323017225618347038, 0.001984525838427520558, 0.002646034451236694077, 0.003969051676855037646, 0.005292068902473381214, 0.005953577515282554300, 0.006615086128091725651, 0.007938103353710070087, 0.008599611966519243172, 0.009261120579328416258, 0.009922629192137589343, 0.01058413780494676243 ),
 .UNSPECIFIED. ) ;
#45332=CARTESIAN_POINT ( 'NONE',  ( 22.57855258442565116, 3.026812727784649493, 25.00000000000000000 ) ) ;
#45339=CARTESIAN_POINT ( 'NONE',  ( 3.057491736622230061, 2.783847009521732030, 11.67432880372605020 ) ) ;
#45340=ADVANCED_FACE ( 'NONE', ( #16360 ), #21334, .T. ) ;
#45341=CARTESIAN_POINT ( 'NONE',  ( -35.00000000000000000, 0.000000000000000000, 0.000000000000000000 ) ) ;
#45342=VERTEX_POINT ( 'NONE', #35949 ) ;
#45345=DIRECTION ( 'NONE',  ( -1.000000000000000000, -0.000000000000000000, -0.000000000000000000 ) ) ;
#45346=ORIENTED_EDGE ( 'NONE', *, *, #17308, .T. ) ;
#45348=CARTESIAN_POINT ( 'NONE',  ( 35.00000000000000000, 4.705694406421931860E-17, -3.469127814946512892E-15 ) ) ;
#45349=VERTEX_POINT ( 'NONE', #56601 ) ;
#45350=VERTEX_POINT ( 'NONE', #11042 ) ;
#45351=ORIENTED_EDGE ( 'NONE', *, *, #31405, .F. ) ;
#45352=EDGE_CURVE ( 'NONE', #45530, #38028, #20354, .T. ) ;
#45354=ORIENTED_EDGE ( 'NONE', *, *, #14834, .T. ) ;
#45355=EDGE_CURVE ( 'NONE', #23572, #29673, #9221, .T. ) ;
#45356=CARTESIAN_POINT ( 'NONE',  ( -8.891032880924177206, -11.36194426013948444, -3.860857758255646921 ) ) ;
#45358=CYLINDRICAL_SURFACE ( 'NONE', #64083, 4.999999999999999112 ) ;
#45361=CARTESIAN_POINT ( 'NONE',  ( 23.97866493766117557, 2.287510638894525883, -13.30844455837636886 ) ) ;
#45365=DIRECTION ( 'NONE',  ( -0.7886918350401329603, -0.6147887355352468219, 0.000000000000000000 ) ) ;
#45367=DIRECTION ( 'NONE',  ( 0.000000000000000000, -0.01356324068817992175, 0.9999080150203990547 ) ) ;
#45368=VERTEX_POINT ( 'NONE', #60589 ) ;
#45369=ORIENTED_EDGE ( 'NONE', *, *, #63398, .F. ) ;
#45372=FACE_OUTER_BOUND ( 'NONE', #17789, .T. ) ;
#45374=EDGE_CURVE ( 'NONE', #46293, #25983, #12401, .T. ) ;
#45375=CARTESIAN_POINT ( 'NONE',  ( -19.80028988669405976, 11.89697986174693511, -1.598264803601076478 ) ) ;
#45376=CARTESIAN_POINT ( 'NONE',  ( 36.00000000000000711, 1.113475361586665491, 12.70128625845191195 ) ) ;
#45377=ORIENTED_EDGE ( 'NONE', *, *, #39564, .F. ) ;
#45378=ORIENTED_EDGE ( 'NONE', *, *, #39999, .F. ) ;
#45379=CARTESIAN_POINT ( 'NONE',  ( 47.00000000000000711, 4.705694406421931860E-17, -3.469127814946512892E-15 ) ) ;
#45382=CYLINDRICAL_SURFACE ( 'NONE', #8362, 13.50000000000000178 ) ;
#45387=AXIS2_PLACEMENT_3D ( 'NONE', #27702, #48352, #3459 ) ;
#45388=DIRECTION ( 'NONE',  ( 0.000000000000000000, -0.01356324068817998940, 0.9999080150203990547 ) ) ;
#45389=CARTESIAN_POINT ( 'NONE',  ( 35.00000000000000000, 11.29812557209481483, 3.213188559034117819 ) ) ;
#45391=ORIENTED_EDGE ( 'NONE', *, *, #14672, .F. ) ;
#45394=DIRECTION ( 'NONE',  ( -1.000000000000000000, -0.000000000000000000, 0.000000000000000000 ) ) ;
#45395=AXIS2_PLACEMENT_3D ( 'NONE', #47452, #62710, #7517 ) ;
#45396=CARTESIAN_POINT ( 'NONE',  ( -37.00000000000000711, -9.506317355798310942, -8.496612874013262484 ) ) ;
#45397=B_SPLINE_CURVE_WITH_KNOTS ( 'NONE', 3,
 ( #12588, #13893, #8931, #23241, #23580, #38190, #18270, #34186, #54494, #63149, #63784, #43184, #64133, #47862, #43502, #17615, #2321, #53177 ),
 .UNSPECIFIED., .F., .F.,
 ( 4, 2, 2, 2, 2, 2, 2, 2, 4 ),
 ( 0.000000000000000000, 0.001482986184832410168, 0.002965972369664820335, 0.004448958554497230503, 0.005931944739329640670, 0.007414930924162050838, 0.008897917108994461005, 0.01038090329382687117, 0.01186388947865928134 ),
 .UNSPECIFIED. ) ;
#45398=CARTESIAN_POINT ( 'NONE',  ( 35.00000000000000000, 6.711949091238142984, -10.84030624090608974 ) ) ;
#45399=CARTESIAN_POINT ( 'NONE',  ( 3.459614771489464946, -11.09853614738469396, 4.563167253695070258 ) ) ;
#45401=CARTESIAN_POINT ( 'NONE',  ( 37.00000000000000711, 11.91791701451269958, 2.544412758415708353 ) ) ;
#45402=DIRECTION ( 'NONE',  ( 0.000000000000000000, -0.4134677391718577510, -0.9105187689795923855 ) ) ;
#45404=ADVANCED_FACE ( 'NONE', ( #36634 ), #65561, .T. ) ;
#45405=ORIENTED_EDGE ( 'NONE', *, *, #36524, .F. ) ;
#45408=CYLINDRICAL_SURFACE ( 'NONE', #4689, 14.99999999999998757 ) ;
#45409=EDGE_CURVE ( 'NONE', #31390, #57924, #33642, .T. ) ;
#45410=DIRECTION ( 'NONE',  ( 0.000000000000000000, -0.01356324068818000328, 0.9999080150203990547 ) ) ;
#45412=VERTEX_POINT ( 'NONE', #55622 ) ;
#45414=LINE ( 'NONE', #46100, #39678 ) ;
#45416=ORIENTED_EDGE ( 'NONE', *, *, #54054, .T. ) ;
#45417=DIRECTION ( 'NONE',  ( 1.000000000000000000, 0.000000000000000000, 0.000000000000000000 ) ) ;
#45419=CARTESIAN_POINT ( 'NONE',  ( 35.00000000000000000, 11.17622378668006355, -3.614449339633533764 ) ) ;
#45420=B_SPLINE_CURVE_WITH_KNOTS ( 'NONE', 3,
 ( #42089, #47442, #42405, #17166, #52753, #21161, #7178, #31154, #27458, #47757, #15831, #36110, #5912, #26169, #41433, #36467, #38089, #55274, #58395, #17824, #7861, #12821, #18158, #9715, #4771, #33107 ),
 .UNSPECIFIED., .F., .F.,
 ( 4, 2, 2, 2, 2, 2, 2, 2, 2, 2, 2, 2, 4 ),
 ( 0.000000000000000000, 0.002656797653146665897, 0.003320997066433334973, 0.003985196479720003182, 0.005313595306293336130, 0.005977794719579998702, 0.006641994132866661273, 0.007306193546153324711, 0.007970392959439987282, 0.008634592372726649853, 0.009298791786013312424, 0.009962991199299976730, 0.01062719061258663930 ),
 .UNSPECIFIED. ) ;
#45421=DIRECTION ( 'NONE',  ( 1.000000000000000000, 0.000000000000000000, 0.000000000000000000 ) ) ;
#45424=EDGE_CURVE ( 'NONE', #54776, #55347, #38960, .T. ) ;
#45430=AXIS2_PLACEMENT_3D ( 'NONE', #22047, #17056, #6121 ) ;
#45432=DIRECTION ( 'NONE',  ( 1.000000000000000000, 0.000000000000000000, 0.000000000000000000 ) ) ;
#45435=CARTESIAN_POINT ( 'NONE',  ( -11.40165637462999904, -7.508992741355383416, 11.21895841913464409 ) ) ;
#45437=VECTOR ( 'NONE', #33027, 1000.000000000000000 ) ;
#45439=CARTESIAN_POINT ( 'NONE',  ( -35.00000000000000000, 0.000000000000000000, 0.000000000000000000 ) ) ;
#45441=CIRCLE ( 'NONE', #57142, 12.74999999999999822 ) ;
#45442=EDGE_CURVE ( 'NONE', #11288, #60004, #45967, .T. ) ;
#45444=CYLINDRICAL_SURFACE ( 'NONE', #51094, 12.74999999999999822 ) ;
#45445=VERTEX_POINT ( 'NONE', #61902 ) ;
#45446=CARTESIAN_POINT ( 'NONE',  ( -35.00000000000000000, 8.052525312710004712, -8.551552972816995890 ) ) ;
#45447=CARTESIAN_POINT ( 'NONE',  ( 9.975240977089113059, 11.94374578141113119, -1.164188000379794419 ) ) ;
#45448=CARTESIAN_POINT ( 'NONE',  ( 36.00000000000000711, 1.908798535168558352, 12.60630747491660486 ) ) ;
#45450=ORIENTED_EDGE ( 'NONE', *, *, #13034, .F. ) ;
#45451=DIRECTION ( 'NONE',  ( 0.000000000000000000, 0.7790879021242486102, -0.6269146997508011632 ) ) ;
#45453=CARTESIAN_POINT ( 'NONE',  ( 22.12621674078617318, -11.11704163603532081, -4.533068918720905671 ) ) ;
#45457=DIRECTION ( 'NONE',  ( 0.000000000000000000, 0.8515178078024887576, -0.5243256840888532722 ) ) ;
#45458=DIRECTION ( 'NONE',  ( 1.000000000000000000, 0.000000000000000000, -0.000000000000000000 ) ) ;
#45461=EDGE_CURVE ( 'NONE', #58933, #58366, #35743, .T. ) ;
#45464=EDGE_CURVE ( 'NONE', #47167, #57461, #61246, .T. ) ;
#45465=DIRECTION ( 'NONE',  ( -1.000000000000000000, -0.000000000000000000, 0.000000000000000000 ) ) ;
#45466=CARTESIAN_POINT ( 'NONE',  ( 11.35368172282957033, 13.35992779450903711, -1.943390003085933015 ) ) ;
#45467=CARTESIAN_POINT ( 'NONE',  ( -35.00000000000000000, -3.093009498344009955, 11.78745411414838884 ) ) ;
#45468=CARTESIAN_POINT ( 'NONE',  ( 8.437200413559441614, 4.476360154859203355, 25.00000000000000000 ) ) ;
#45469=FACE_OUTER_BOUND ( 'NONE', #6639, .T. ) ;
#45471=CIRCLE ( 'NONE', #10444, 5.000000000000000000 ) ;
#45472=EDGE_LOOP ( 'NONE', ( #39900, #46925, #58415, #7167 ) ) ;
#45473=EDGE_CURVE ( 'NONE', #50294, #3168, #15674, .T. ) ;
#45475=AXIS2_PLACEMENT_3D ( 'NONE', #58873, #19259, #33572 ) ;
#45478=DIRECTION ( 'NONE',  ( -1.000000000000000000, -0.000000000000000000, 0.000000000000000000 ) ) ;
#45479=CARTESIAN_POINT ( 'NONE',  ( 35.00000000000000000, 7.882940143791773657, -10.02106554660711524 ) ) ;
#45481=AXIS2_PLACEMENT_3D ( 'NONE', #35885, #56184, #4355 ) ;
#45483=LINE ( 'NONE', #286, #36052 ) ;
#45485=ORIENTED_EDGE ( 'NONE', *, *, #30998, .T. ) ;
#45486=CARTESIAN_POINT ( 'NONE',  ( 37.00000000000000711, 11.65150730582934635, 1.488153103997001514 ) ) ;
#45488=DIRECTION ( 'NONE',  ( 0.000000000000000000, 0.6269146997507929475, 0.7790879021242551605 ) ) ;
#45489=CIRCLE ( 'NONE', #44429, 12.18650000000000055 ) ;
#45491=CARTESIAN_POINT ( 'NONE',  ( 8.948006322247541888, 4.815211251969169659, -12.61333397820095570 ) ) ;
#45496=DIRECTION ( 'NONE',  ( 0.000000000000000000, 0.3807014730195220631, -0.9246979985058721985 ) ) ;
#45497=DIRECTION ( 'NONE',  ( 0.000000000000000000, 0.3807014730195152907, -0.9246979985058750851 ) ) ;
#45498=B_SPLINE_CURVE_WITH_KNOTS ( 'NONE', 3,
 ( #43356, #2836, #63631, #3156, #18106, #23418, #43692, #3495, #13748, #63980, #18461, #38716, #59018, #23768, #13431, #54010, #59988, #44338, #60297, #20393, #65592, #64946, #64614, #60968 ),
 .UNSPECIFIED., .F., .F.,
 ( 4, 2, 2, 2, 2, 2, 2, 2, 2, 2, 2, 4 ),
 ( 0.002913801881037346962, 0.003520887530297034471, 0.004127973179556721980, 0.005342144478076094397, 0.006556315776595466813, 0.007163401425855153888, 0.007770487075114840096, 0.008984658373634213380, 0.009591744022893901322, 0.01019882967215358580, 0.01141300097067296168, 0.01262717226919233410 ),
 .UNSPECIFIED. ) ;
#45499=CARTESIAN_POINT ( 'NONE',  ( 47.00000000000000711, 4.705694406421931860E-17, -3.469127814946512892E-15 ) ) ;
#45506=CARTESIAN_POINT ( 'NONE',  ( -35.00000000000000000, 0.000000000000000000, 0.000000000000000000 ) ) ;
#45507=DIRECTION ( 'NONE',  ( 1.000000000000000000, 0.000000000000000000, -0.000000000000000000 ) ) ;
#45510=CIRCLE ( 'NONE', #16848, 12.75000000000000178 ) ;
#45511=DIRECTION ( 'NONE',  ( 1.000000000000000000, 0.000000000000000000, -0.000000000000000000 ) ) ;
#45512=CARTESIAN_POINT ( 'NONE',  ( -27.78468958554971380, 25.00000000000000000, 8.565911087387465983 ) ) ;
#45515=CARTESIAN_POINT ( 'NONE',  ( -8.957233933390911673, -8.874460928901493517, -8.086001677246498431 ) ) ;
#45516=ORIENTED_EDGE ( 'NONE', *, *, #45086, .T. ) ;
#45518=CIRCLE ( 'NONE', #64634, 5.000000000000000888 ) ;
#45519=EDGE_CURVE ( 'NONE', #36643, #52670, #43167, .T. ) ;
#45521=ORIENTED_EDGE ( 'NONE', *, *, #775, .T. ) ;
#45522=PLANE ( 'NONE',  #11919 ) ;
#45523=VECTOR ( 'NONE', #48788, 1000.000000000000000 ) ;
#45524=EDGE_LOOP ( 'NONE', ( #64194, #6953, #18401, #25354 ) ) ;
#45525=VECTOR ( 'NONE', #23641, 1000.000000000000000 ) ;
#45526=CARTESIAN_POINT ( 'NONE',  ( 35.00000000000000000, -5.865551165830998670, 11.32068061209301035 ) ) ;
#45527=DIRECTION ( 'NONE',  ( 1.000000000000000000, 0.000000000000000000, -0.000000000000000000 ) ) ;
#45528=CARTESIAN_POINT ( 'NONE',  ( 16.94760237393649405, 10.49682181221983157, 5.815268149447246238 ) ) ;
#45530=VERTEX_POINT ( 'NONE', #2040 ) ;
#45531=VERTEX_POINT ( 'NONE', #32934 ) ;
#45534=ORIENTED_EDGE ( 'NONE', *, *, #23413, .T. ) ;
#45536=ORIENTED_EDGE ( 'NONE', *, *, #35759, .F. ) ;
#45537=ORIENTED_EDGE ( 'NONE', *, *, #1259, .T. ) ;
#45539=ORIENTED_EDGE ( 'NONE', *, *, #11173, .F. ) ;
#45542=EDGE_CURVE ( 'NONE', #52056, #64815, #20906, .T. ) ;
#45544=DIRECTION ( 'NONE',  ( 0.000000000000000000, -0.1387779952735677669, 0.9903235168508569553 ) ) ;
#45545=CARTESIAN_POINT ( 'NONE',  ( -35.00000000000000000, 0.2661492558805056974, -12.18359334611896116 ) ) ;
#45548=ORIENTED_EDGE ( 'NONE', *, *, #54696, .T. ) ;
#45549=DIRECTION ( 'NONE',  ( -0.000000000000000000, -0.000000000000000000, -1.000000000000000000 ) ) ;
#45550=EDGE_CURVE ( 'NONE', #31183, #21600, #7100, .T. ) ;
#45551=DIRECTION ( 'NONE',  ( -1.000000000000000000, 0.000000000000000000, 0.000000000000000000 ) ) ;
#45552=EDGE_CURVE ( 'NONE', #16066, #16210, #23019, .T. ) ;
#45556=CARTESIAN_POINT ( 'NONE',  ( -25.54417658651491863, 25.00000000000000000, 11.22596262356930197 ) ) ;
#45558=ORIENTED_EDGE ( 'NONE', *, *, #34472, .F. ) ;
#45559=EDGE_CURVE ( 'NONE', #8013, #40304, #42576, .T. ) ;
#45561=CIRCLE ( 'NONE', #32826, 12.75000000000000178 ) ;
#45563=EDGE_CURVE ( 'NONE', #33980, #5232, #50652, .T. ) ;
#45567=CARTESIAN_POINT ( 'NONE',  ( -35.00000000000000000, 0.000000000000000000, 0.000000000000000000 ) ) ;
#45569=ORIENTED_EDGE ( 'NONE', *, *, #22499, .F. ) ;
#45570=LINE ( 'NONE', #8130, #42993 ) ;
#45572=LINE ( 'NONE', #29613, #24741 ) ;
#45575=AXIS2_PLACEMENT_3D ( 'NONE', #41501, #35846, #644 ) ;
#45576=B_SPLINE_CURVE_WITH_KNOTS ( 'NONE', 3,
 ( #58292, #53305, #48335, #43302, #18052, #58636, #33344, #50291 ),
 .UNSPECIFIED., .F., .F.,
 ( 4, 2, 2, 4 ),
 ( 0.000000000000000000, 0.001617793918133567837, 0.002426690877200354032, 0.003235587836267140010 ),
 .UNSPECIFIED. ) ;
#45577=EDGE_CURVE ( 'NONE', #54027, #27642, #62226, .T. ) ;
#45578=AXIS2_PLACEMENT_3D ( 'NONE', #49846, #59183, #55152 ) ;
#45580=EDGE_CURVE ( 'NONE', #50423, #33155, #42246, .T. ) ;
#45581=CARTESIAN_POINT ( 'NONE',  ( -35.00000000000000000, -10.99909370905153594, -5.246972444134134328 ) ) ;
#45583=DIRECTION ( 'NONE',  ( 0.000000000000000000, -0.01356324068817999114, 0.9999080150203989437 ) ) ;
#45586=EDGE_LOOP ( 'NONE', ( #32038, #4066, #54552, #46164 ) ) ;
#45590=DIRECTION ( 'NONE',  ( -0.000000000000000000, -0.000000000000000000, -1.000000000000000000 ) ) ;
#45591=CARTESIAN_POINT ( 'NONE',  ( 35.00000000000000000, -5.130401251914806338, -11.05394794832827898 ) ) ;
#45592=ORIENTED_EDGE ( 'NONE', *, *, #57172, .F. ) ;
#45594=EDGE_LOOP ( 'NONE', ( #64948, #15652, #51846, #2325 ) ) ;
#45596=EDGE_CURVE ( 'NONE', #33067, #26019, #1801, .T. ) ;
#45599=ORIENTED_EDGE ( 'NONE', *, *, #30332, .F. ) ;
#45601=DIRECTION ( 'NONE',  ( 0.000000000000000000, -1.000000000000000000, 0.000000000000000000 ) ) ;
#45602=DIRECTION ( 'NONE',  ( 0.000000000000000000, 0.01356324068817998940, -0.9999080150203989437 ) ) ;
#45604=DIRECTION ( 'NONE',  ( 0.000000000000000000, -0.3554799084908832896, -0.9346839223284592046 ) ) ;
#45607=CARTESIAN_POINT ( 'NONE',  ( 37.00000000000000711, -10.25474254703957477, -6.584150480049516752 ) ) ;
#45608=ORIENTED_EDGE ( 'NONE', *, *, #62381, .T. ) ;
#45609=CYLINDRICAL_SURFACE ( 'NONE', #35269, 5.000000000000000888 ) ;
#45612=ADVANCED_FACE ( 'NONE', ( #7029 ), #52276, .T. ) ;
#45613=EDGE_LOOP ( 'NONE', ( #34728, #24670, #12944, #18642 ) ) ;
#45619=DIRECTION ( 'NONE',  ( 0.000000000000000000, 0.01356324068817298112, -0.9999080150203990547 ) ) ;
#45621=EDGE_CURVE ( 'NONE', #95, #6107, #17343, .T. ) ;
#45624=DIRECTION ( 'NONE',  ( 0.000000000000000000, -0.01356324068817998073, 0.9999080150203990547 ) ) ;
#45625=CARTESIAN_POINT ( 'NONE',  ( 7.278150647452634736, -5.674969998030102047, 12.25652322899233937 ) ) ;
#45626=VERTEX_POINT ( 'NONE', #12010 ) ;
#45627=VECTOR ( 'NONE', #43368, 1000.000000000000000 ) ;
#45628=LINE ( 'NONE', #60599, #17305 ) ;
#45629=( BOUNDED_CURVE ( )  B_SPLINE_CURVE ( 3, ( #35290, #48, #61229, #40949 ),
 .UNSPECIFIED., .F., .F. ) 
 B_SPLINE_CURVE_WITH_KNOTS ( ( 4, 4 ),
 ( 4.379469035996294224, 4.407264310173042432 ),
 .UNSPECIFIED. ) 
 CURVE ( )  GEOMETRIC_REPRESENTATION_ITEM ( )  RATIONAL_B_SPLINE_CURVE ( ( 1.000000000000000000, 0.9999356195973556627, 0.9999356195973556627, 1.000000000000000000 ) ) 
 REPRESENTATION_ITEM ( '' )  );
#45630=ORIENTED_EDGE ( 'NONE', *, *, #42941, .T. ) ;
#45631=CARTESIAN_POINT ( 'NONE',  ( -37.00000000000000711, 0.000000000000000000, 0.000000000000000000 ) ) ;
#45633=CARTESIAN_POINT ( 'NONE',  ( -37.00000000000000711, 7.817610399097512541, 8.766823244862019138 ) ) ;
#45634=ADVANCED_FACE ( 'NONE', ( #47929 ), #12335, .T. ) ;
#45636=CARTESIAN_POINT ( 'NONE',  ( -36.00000000000000711, 10.49626516989271252, 7.238157050195668241 ) ) ;
#45638=AXIS2_PLACEMENT_3D ( 'NONE', #49492, #3930, #8906 ) ;
#45641=CARTESIAN_POINT ( 'NONE',  ( 11.86932257037118177, 8.667155996924391204, -8.300945040779886597 ) ) ;
#45643=DIRECTION ( 'NONE',  ( 1.000000000000000000, 0.000000000000000000, 0.000000000000000000 ) ) ;
#45644=ORIENTED_EDGE ( 'NONE', *, *, #16344, .T. ) ;
#45645=EDGE_CURVE ( 'NONE', #54601, #31785, #25180, .T. ) ;
#45647=CARTESIAN_POINT ( 'NONE',  ( -36.00000000000000711, 5.300372733891805410, -11.59605747147781152 ) ) ;
#45648=CARTESIAN_POINT ( 'NONE',  ( -2.532614230583026593, 5.020478806276888584, 10.89930238848911337 ) ) ;
#45650=ORIENTED_EDGE ( 'NONE', *, *, #42275, .F. ) ;
#45653=AXIS2_PLACEMENT_3D ( 'NONE', #17951, #28573, #38214 ) ;
#45654=VECTOR ( 'NONE', #56800, 1000.000000000000000 ) ;
#45655=EDGE_CURVE ( 'NONE', #21860, #42381, #3979, .T. ) ;
#45656=EDGE_CURVE ( 'NONE', #28963, #27631, #39903, .T. ) ;
#45659=DIRECTION ( 'NONE',  ( -1.000000000000000000, 0.000000000000000000, 0.000000000000000000 ) ) ;
#45661=VERTEX_POINT ( 'NONE', #3379 ) ;
#45663=DIRECTION ( 'NONE',  ( -1.000000000000000000, 0.000000000000000000, 0.000000000000000000 ) ) ;
#45664=CARTESIAN_POINT ( 'NONE',  ( 3.968427614672949577, 6.597710521095812020, 10.03374174353559845 ) ) ;
#45665=AXIS2_PLACEMENT_3D ( 'NONE', #6863, #53394, #2541 ) ;
#45666=CARTESIAN_POINT ( 'NONE',  ( -35.00000000000000000, -10.68873102412847587, 6.950793414699756312 ) ) ;
#45667=CARTESIAN_POINT ( 'NONE',  ( 37.00000000000000711, 10.91072401419418192, 5.428340790341586342 ) ) ;
#45668=AXIS2_PLACEMENT_3D ( 'NONE', #13527, #33808, #39793 ) ;
#45669=ORIENTED_EDGE ( 'NONE', *, *, #64177, .T. ) ;
#45671=CARTESIAN_POINT ( 'NONE',  ( 3.291290029914074378, 8.250315036047103590, -8.713914264323182834 ) ) ;
#45673=ORIENTED_EDGE ( 'NONE', *, *, #27086, .T. ) ;
#45674=CARTESIAN_POINT ( 'NONE',  ( 37.00000000000000711, -8.624332853795991127, 9.390600770288079602 ) ) ;
#45676=ORIENTED_EDGE ( 'NONE', *, *, #52372, .F. ) ;
#45677=CIRCLE ( 'NONE', #42477, 5.000000000000000000 ) ;
#45680=EDGE_CURVE ( 'NONE', #19321, #31870, #52815, .T. ) ;
#45681=ORIENTED_EDGE ( 'NONE', *, *, #36263, .F. ) ;
#45682=DIRECTION ( 'NONE',  ( 0.000000000000000000, 0.01356324068817998940, -0.9999080150203990547 ) ) ;
#45683=LINE ( 'NONE', #65313, #31501 ) ;
#45685=CIRCLE ( 'NONE', #45051, 12.18650000000000411 ) ;
#45686=CARTESIAN_POINT ( 'NONE',  ( 35.00000000000000000, 2.627174906297071733, 11.44858830469737221 ) ) ;
#45689=CARTESIAN_POINT ( 'NONE',  ( 24.88574069546950085, -1.123412547988487775, -13.45466109831467705 ) ) ;
#45690=LINE ( 'NONE', #20430, #32974 ) ;
#45692=CARTESIAN_POINT ( 'NONE',  ( 3.780834652287974773, 8.352030633203074927, 8.616471685210687070 ) ) ;
#45694=DIRECTION ( 'NONE',  ( 0.000000000000000000, 0.7790879021242486102, -0.6269146997508011632 ) ) ;
#45695=ORIENTED_EDGE ( 'NONE', *, *, #20641, .F. ) ;
#45696=EDGE_CURVE ( 'NONE', #60506, #1959, #19869, .T. ) ;
#45697=VERTEX_POINT ( 'NONE', #64204 ) ;
#45698=CARTESIAN_POINT ( 'NONE',  ( 35.00000000000000000, 4.018060380616396365, -11.50504120060944757 ) ) ;
#45701=VECTOR ( 'NONE', #938, 1000.000000000000000 ) ;
#45703=CIRCLE ( 'NONE', #62673, 12.75000000000000178 ) ;
#45704=CARTESIAN_POINT ( 'NONE',  ( 47.00000000000000711, 4.705694406421931860E-17, -3.469127814946512892E-15 ) ) ;
#45705=CIRCLE ( 'NONE', #5367, 5.000000000000001776 ) ;
#45706=CARTESIAN_POINT ( 'NONE',  ( -35.00000000000000000, -5.246972444134095248, 10.99909370905155370 ) ) ;
#45708=ORIENTED_EDGE ( 'NONE', *, *, #23529, .F. ) ;
#45710=DIRECTION ( 'NONE',  ( 0.000000000000000000, 0.01356324068817999808, -0.9999080150203990547 ) ) ;
#45711=ORIENTED_EDGE ( 'NONE', *, *, #39361, .F. ) ;
#45712=EDGE_CURVE ( 'NONE', #11505, #48583, #23647, .T. ) ;
#45713=VERTEX_POINT ( 'NONE', #19310 ) ;
#45716=CARTESIAN_POINT ( 'NONE',  ( -37.00000000000000711, -11.74226168163341022, -0.3025107581132430723 ) ) ;
#45717=CARTESIAN_POINT ( 'NONE',  ( 37.00000000000000711, -4.983891302653661093, -11.73555825188274682 ) ) ;
#45718=LINE ( 'NONE', #24794, #8245 ) ;
#45721=CIRCLE ( 'NONE', #59545, 12.18650000000000055 ) ;
#45722=VERTEX_POINT ( 'NONE', #54879 ) ;
#45723=ORIENTED_EDGE ( 'NONE', *, *, #775, .F. ) ;
#45724=AXIS2_PLACEMENT_3D ( 'NONE', #49666, #4107, #24375 ) ;
#45725=CARTESIAN_POINT ( 'NONE',  ( 37.00000000000000711, 4.705694406421931860E-17, -3.469127814946512892E-15 ) ) ;
#45726=DIRECTION ( 'NONE',  ( 0.8386510381079236298, 0.5446691071471760903, -0.000000000000000000 ) ) ;
#45730=EDGE_CURVE ( 'NONE', #38995, #10202, #19646, .T. ) ;
#45733=CIRCLE ( 'NONE', #49975, 12.18650000000000055 ) ;
#45734=CARTESIAN_POINT ( 'NONE',  ( 22.57855258442565116, 3.026812727784649493, -13.15630665159948975 ) ) ;
#45735=CARTESIAN_POINT ( 'NONE',  ( -37.00000000000000711, -10.07641281632181673, 6.036400161834530209 ) ) ;
#45736=EDGE_CURVE ( 'NONE', #12199, #20112, #51221, .T. ) ;
#45742=CYLINDRICAL_SURFACE ( 'NONE', #14181, 12.74999999999999822 ) ;
#45743=AXIS2_PLACEMENT_3D ( 'NONE', #31439, #14805, #35090 ) ;
#45744=CIRCLE ( 'NONE', #20256, 12.18650000000000233 ) ;
#45745=CIRCLE ( 'NONE', #41510, 12.18649999999999878 ) ;
#45747=DIRECTION ( 'NONE',  ( 0.000000000000000000, 0.01356324068817992175, -0.9999080150203990547 ) ) ;
#45750=CARTESIAN_POINT ( 'NONE',  ( -36.00000000000000711, -4.983891302653499444, -11.73555825188281787 ) ) ;
#45752=ORIENTED_EDGE ( 'NONE', *, *, #46751, .F. ) ;
#45753=DIRECTION ( 'NONE',  ( 0.000000000000000000, -0.01356324068817999114, 0.9999080150203989437 ) ) ;
#45758=DIRECTION ( 'NONE',  ( 0.000000000000000000, -0.01356324068817999114, 0.9999080150203989437 ) ) ;
#45759=CIRCLE ( 'NONE', #13898, 5.000000000000000888 ) ;
#45760=AXIS2_PLACEMENT_3D ( 'NONE', #63866, #22677, #58240 ) ;
#45762=EDGE_CURVE ( 'NONE', #26019, #36323, #53868, .T. ) ;
#45764=ORIENTED_EDGE ( 'NONE', *, *, #36157, .T. ) ;
#45765=VECTOR ( 'NONE', #28004, 1000.000000000000000 ) ;
#45768=CARTESIAN_POINT ( 'NONE',  ( -9.181000754636428951, 11.30974670563849571, -7.379660233987727302 ) ) ;
#45770=CARTESIAN_POINT ( 'NONE',  ( 37.00000000000000711, 4.705694406421931860E-17, -3.469127814946512892E-15 ) ) ;
#45771=CARTESIAN_POINT ( 'NONE',  ( -37.00000000000000711, 0.000000000000000000, 0.000000000000000000 ) ) ;
#45772=AXIS2_PLACEMENT_3D ( 'NONE', #9605, #29903, #25244 ) ;
#45773=CYLINDRICAL_SURFACE ( 'NONE', #5831, 4.999999999999999112 ) ;
#45774=CARTESIAN_POINT ( 'NONE',  ( 35.00000000000000000, 2.346765782874432382, -11.95840593935202278 ) ) ;
#45775=ORIENTED_EDGE ( 'NONE', *, *, #23960, .F. ) ;
#45777=AXIS2_PLACEMENT_3D ( 'NONE', #53830, #63773, #8265 ) ;
#45778=ORIENTED_EDGE ( 'NONE', *, *, #12295, .F. ) ;
#45779=ADVANCED_FACE ( 'NONE', ( #11607 ), #52196, .T. ) ;
#45783=CARTESIAN_POINT ( 'NONE',  ( -17.97077823246242190, -9.629623312810583258, 9.462431742398617729 ) ) ;
#45784=EDGE_LOOP ( 'NONE', ( #43590, #21653, #1468, #18305 ) ) ;
#45785=AXIS2_PLACEMENT_3D ( 'NONE', #24284, #48924, #29587 ) ;
#45786=DIRECTION ( 'NONE',  ( 0.000000000000000000, -0.01356324068817999114, 0.9999080150203989437 ) ) ;
#45787=CARTESIAN_POINT ( 'NONE',  ( 12.28749691143031697, 11.61437747111016172, -3.022945891257621032 ) ) ;
#45788=FACE_BOUND ( 'NONE', #6949, .T. ) ;
#45790=VERTEX_POINT ( 'NONE', #31876 ) ;
#45792=CIRCLE ( 'NONE', #50022, 12.75000000000000178 ) ;
#45793=ADVANCED_FACE ( 'NONE', ( #16930 ), #6644, .T. ) ;
#45796=DIRECTION ( 'NONE',  ( 0.000000000000000000, 0.01356324068817998940, -0.9999080150203989437 ) ) ;
#45801=AXIS2_PLACEMENT_3D ( 'NONE', #31362, #123, #55662 ) ;
#45802=VECTOR ( 'NONE', #58694, 1000.000000000000000 ) ;
#45803=CARTESIAN_POINT ( 'NONE',  ( 25.05309951391468459, -8.823569016628452388, -8.132934882857099979 ) ) ;
#45804=DIRECTION ( 'NONE',  ( -1.000000000000000000, 0.000000000000000000, 0.000000000000000000 ) ) ;
#45805=AXIS2_PLACEMENT_3D ( 'NONE', #32968, #53937, #22343 ) ;
#45808=DIRECTION ( 'NONE',  ( 0.000000000000000000, 0.2355298848897447450, 0.9718671068226475418 ) ) ;
#45809=DIRECTION ( 'NONE',  ( -1.000000000000000000, 0.000000000000000000, 0.000000000000000000 ) ) ;
#45810=CARTESIAN_POINT ( 'NONE',  ( 12.44012537477689229, 11.41883593682970321, -7.203604244167406634 ) ) ;
#45811=CARTESIAN_POINT ( 'NONE',  ( -19.47984447937493613, -3.750539801530005768, 12.96855624952674724 ) ) ;
#45812=CARTESIAN_POINT ( 'NONE',  ( 10.48620311856346454, 8.250315036047107142, 25.00000000000000000 ) ) ;
#45813=DIRECTION ( 'NONE',  ( 1.000000000000000000, 0.000000000000000000, 0.000000000000000000 ) ) ;
#45814=CARTESIAN_POINT ( 'NONE',  ( -35.00000000000000000, -2.497432891016921008, 11.47758908105693720 ) ) ;
#45815=CIRCLE ( 'NONE', #39436, 5.000000000000000000 ) ;
#45817=AXIS2_PLACEMENT_3D ( 'NONE', #12691, #43281, #32970 ) ;
#45819=DIRECTION ( 'NONE',  ( 1.000000000000000000, 0.000000000000000000, -0.000000000000000000 ) ) ;
#45823=LINE ( 'NONE', #35163, #65707 ) ;
#45824=DIRECTION ( 'NONE',  ( 0.000000000000000000, -0.01356324068817991828, 0.9999080150203990547 ) ) ;
#45826=CIRCLE ( 'NONE', #51155, 12.74999999999999822 ) ;
#45828=DIRECTION ( 'NONE',  ( 0.000000000000000000, -0.8827602140260366603, 0.4698238015817268187 ) ) ;
#45832=AXIS2_PLACEMENT_3D ( 'NONE', #39753, #49435, #23828 ) ;
#45833=CARTESIAN_POINT ( 'NONE',  ( -37.00000000000000711, 0.000000000000000000, 0.000000000000000000 ) ) ;
#45835=CARTESIAN_POINT ( 'NONE',  ( -18.35038919876964059, -4.541481526684528092, 11.10824452668961193 ) ) ;
#45837=CYLINDRICAL_SURFACE ( 'NONE', #31877, 12.18649999999999878 ) ;
#45839=ORIENTED_EDGE ( 'NONE', *, *, #12428, .F. ) ;
#45841=AXIS2_PLACEMENT_3D ( 'NONE', #42642, #27056, #62947 ) ;
#45842=ORIENTED_EDGE ( 'NONE', *, *, #2328, .T. ) ;
#45843=AXIS2_PLACEMENT_3D ( 'NONE', #12546, #62768, #11263 ) ;
#45845=LINE ( 'NONE', #14264, #43719 ) ;
#45847=CARTESIAN_POINT ( 'NONE',  ( 35.00000000000000000, -12.54989509947652415, -2.250029553613715372 ) ) ;
#45848=AXIS2_PLACEMENT_3D ( 'NONE', #39128, #45114, #65375 ) ;
#45849=CIRCLE ( 'NONE', #46903, 5.000000000000000000 ) ;
#45850=AXIS2_PLACEMENT_3D ( 'NONE', #42287, #36347, #36674 ) ;
#45852=ORIENTED_EDGE ( 'NONE', *, *, #17584, .F. ) ;
#45853=CARTESIAN_POINT ( 'NONE',  ( -28.85619398320021745, 3.750539801530000439, 11.39883551934754280 ) ) ;
#45855=EDGE_CURVE ( 'NONE', #30464, #29745, #59187, .T. ) ;
#45857=CARTESIAN_POINT ( 'NONE',  ( -37.00000000000000711, 11.07407352312212723, 3.916263239775389149 ) ) ;
#45858=DIRECTION ( 'NONE',  ( 1.000000000000000000, -0.000000000000000000, 0.000000000000000000 ) ) ;
#45862=CARTESIAN_POINT ( 'NONE',  ( -9.994394625950207001, -3.431105229675856627, 11.50047856588473216 ) ) ;
#45866=DIRECTION ( 'NONE',  ( 0.000000000000000000, 0.01356324068817998940, -0.9999080150203990547 ) ) ;
#45867=AXIS2_PLACEMENT_3D ( 'NONE', #31226, #65780, #61153 ) ;
#45872=AXIS2_PLACEMENT_3D ( 'NONE', #1442, #31353, #21722 ) ;
#45874=ORIENTED_EDGE ( 'NONE', *, *, #42434, .T. ) ;
#45875=DIRECTION ( 'NONE',  ( -1.000000000000000000, 0.000000000000000000, 0.000000000000000000 ) ) ;
#45876=LINE ( 'NONE', #39892, #27550 ) ;
#45879=ORIENTED_EDGE ( 'NONE', *, *, #16648, .T. ) ;
#45881=ORIENTED_EDGE ( 'NONE', *, *, #56435, .T. ) ;
#45883=VERTEX_POINT ( 'NONE', #17601 ) ;
#45884=EDGE_CURVE ( 'NONE', #33198, #36759, #10324, .T. ) ;
#45886=ORIENTED_EDGE ( 'NONE', *, *, #59555, .T. ) ;
#45888=ORIENTED_EDGE ( 'NONE', *, *, #47128, .F. ) ;
#45895=ORIENTED_EDGE ( 'NONE', *, *, #64825, .F. ) ;
#45897=VECTOR ( 'NONE', #19138, 1000.000000000000000 ) ;
#45898=EDGE_LOOP ( 'NONE', ( #65749, #53869, #5041, #23127 ) ) ;
#45908=VECTOR ( 'NONE', #65104, 1000.000000000000000 ) ;
#45909=ORIENTED_EDGE ( 'NONE', *, *, #41490, .T. ) ;
#45910=DIRECTION ( 'NONE',  ( 0.000000000000000000, 0.9903235168508555120, 0.1387779952735781197 ) ) ;
#45912=CARTESIAN_POINT ( 'NONE',  ( -24.51086266037313521, -9.341341120805065401, 9.748122042855369429 ) ) ;
#45914=DIRECTION ( 'NONE',  ( -1.000000000000000000, 0.000000000000000000, 0.000000000000000000 ) ) ;
#45916=VERTEX_POINT ( 'NONE', #62798 ) ;
#45917=CYLINDRICAL_SURFACE ( 'NONE', #39859, 5.000000000000000888 ) ;
#45918=LINE ( 'NONE', #372, #37536 ) ;
#45919=DIRECTION ( 'NONE',  ( 0.000000000000000000, 0.01356324068817991828, -0.9999080150203990547 ) ) ;
#45920=CARTESIAN_POINT ( 'NONE',  ( 22.98496193214445782, -11.91169011612080197, -6.361484732325027203 ) ) ;
#45922=EDGE_CURVE ( 'NONE', #24889, #42846, #62335, .T. ) ;
#45924=CIRCLE ( 'NONE', #9824, 4.999999999999999112 ) ;
#45925=AXIS2_PLACEMENT_3D ( 'NONE', #23559, #43833, #18593 ) ;
#45926=CARTESIAN_POINT ( 'NONE',  ( 35.00000000000000000, 0.2661492558803343345, -12.18359334611896649 ) ) ;
#45928=CYLINDRICAL_SURFACE ( 'NONE', #10232, 5.000000000000000888 ) ;
#45929=DIRECTION ( 'NONE',  ( -1.000000000000000000, -0.000000000000000000, 0.000000000000000000 ) ) ;
#45931=ORIENTED_EDGE ( 'NONE', *, *, #5994, .T. ) ;
#45932=AXIS2_PLACEMENT_3D ( 'NONE', #41128, #56098, #25864 ) ;
#45934=ORIENTED_EDGE ( 'NONE', *, *, #31100, .F. ) ;
#45935=PLANE ( 'NONE',  #9775 ) ;
#45937=CYLINDRICAL_SURFACE ( 'NONE', #9855, 12.18650000000000055 ) ;
#45939=EDGE_CURVE ( 'NONE', #5675, #27379, #51736, .T. ) ;
#45942=AXIS2_PLACEMENT_3D ( 'NONE', #28934, #49243, #39223 ) ;
#45944=ORIENTED_EDGE ( 'NONE', *, *, #31470, .T. ) ;
#45946=AXIS2_PLACEMENT_3D ( 'NONE', #36422, #31434, #51734 ) ;
#45949=ADVANCED_FACE ( 'NONE', ( #44806 ), #24203, .T. ) ;
#45950=ORIENTED_EDGE ( 'NONE', *, *, #26557, .T. ) ;
#45951=CARTESIAN_POINT ( 'NONE',  ( -35.00000000000000000, 5.428340790341860789, -10.91072401419405402 ) ) ;
#45952=CYLINDRICAL_SURFACE ( 'NONE', #25140, 12.74999999999999822 ) ;
#45953=DIRECTION ( 'NONE',  ( 0.000000000000000000, 0.9847383929261610547, -0.1740410799127650732 ) ) ;
#45959=VERTEX_POINT ( 'NONE', #23565 ) ;
#45960=LINE ( 'NONE', #50306, #44816 ) ;
#45961=ORIENTED_EDGE ( 'NONE', *, *, #894, .T. ) ;
#45963=CIRCLE ( 'NONE', #58751, 4.999999999999999112 ) ;
#45964=ORIENTED_EDGE ( 'NONE', *, *, #694, .F. ) ;
#45966=DIRECTION ( 'NONE',  ( 0.000000000000000000, 0.01356324068817998940, -0.9999080150203989437 ) ) ;
#45967=LINE ( 'NONE', #422, #2853 ) ;
#45970=DIRECTION ( 'NONE',  ( 1.000000000000000000, 0.000000000000000000, 0.000000000000000000 ) ) ;
#45972=CARTESIAN_POINT ( 'NONE',  ( 4.724233633166516455, -10.62268705308553329, 8.332287045309458406 ) ) ;
#45974=EDGE_CURVE ( 'NONE', #10832, #13628, #2901, .T. ) ;
#45975=B_SPLINE_CURVE_WITH_KNOTS ( 'NONE', 3,
 ( #20907, #6865, #37427, #52742, #2868, #2543, #62687, #58056, #51194, #22812 ),
 .UNSPECIFIED., .F., .F.,
 ( 4, 2, 2, 2, 4 ),
 ( 0.000000000000000000, 0.001081654908065314818, 0.002163309816130629636, 0.003244964724195944453, 0.004326619632261259271 ),
 .UNSPECIFIED. ) ;
#45976=FACE_OUTER_BOUND ( 'NONE', #60347, .T. ) ;
#45977=ORIENTED_EDGE ( 'NONE', *, *, #3584, .T. ) ;
#45978=CARTESIAN_POINT ( 'NONE',  ( 10.53916981844864509, -13.47532649378942260, -0.8438262861795845504 ) ) ;
#45979=ORIENTED_EDGE ( 'NONE', *, *, #45161, .F. ) ;
#45980=DIRECTION ( 'NONE',  ( 0.000000000000000000, 0.8696919319575201479, 0.4935949184179230786 ) ) ;
#45981=ORIENTED_EDGE ( 'NONE', *, *, #26062, .F. ) ;
#45983=LINE ( 'NONE', #26029, #36138 ) ;
#45985=DIRECTION ( 'NONE',  ( 1.000000000000000000, 0.000000000000000000, -0.000000000000000000 ) ) ;
#45988=CYLINDRICAL_SURFACE ( 'NONE', #38594, 4.999999999999998224 ) ;
#45989=VERTEX_POINT ( 'NONE', #28536 ) ;
#45990=CARTESIAN_POINT ( 'NONE',  ( 35.00000000000000000, 4.705694406421931860E-17, -3.469127814946512892E-15 ) ) ;
#45991=CYLINDRICAL_SURFACE ( 'NONE', #7974, 5.000000000000000000 ) ;
#45994=VECTOR ( 'NONE', #21968, 1000.000000000000000 ) ;
#45996=DIRECTION ( 'NONE',  ( 0.000000000000000000, -0.01356324068817998940, 0.9999080150203990547 ) ) ;
#45998=EDGE_CURVE ( 'NONE', #64338, #33727, #11372, .T. ) ;
#46001=CARTESIAN_POINT ( 'NONE',  ( 35.00000000000000000, 1.171570255487609291, 11.68758509253246380 ) ) ;
#46004=DIRECTION ( 'NONE',  ( 0.000000000000000000, 0.6269146997507987207, 0.7790879021242507196 ) ) ;
#46005=EDGE_LOOP ( 'NONE', ( #27400, #3995, #61254, #27712 ) ) ;
#46006=CARTESIAN_POINT ( 'NONE',  ( -37.00000000000000711, 11.37311665002359540, 2.936739658820077370 ) ) ;
#46007=CARTESIAN_POINT ( 'NONE',  ( -35.00000000000000000, 0.000000000000000000, 0.000000000000000000 ) ) ;
#46010=AXIS2_PLACEMENT_3D ( 'NONE', #45120, #39798, #9198 ) ;
#46011=EDGE_CURVE ( 'NONE', #40836, #7740, #38996, .T. ) ;
#46014=AXIS2_PLACEMENT_3D ( 'NONE', #58299, #63585, #47998 ) ;
#46015=ORIENTED_EDGE ( 'NONE', *, *, #19786, .T. ) ;
#46017=CARTESIAN_POINT ( 'NONE',  ( 37.00000000000000711, -10.70999494708488520, 5.814360711498399503 ) ) ;
#46018=CARTESIAN_POINT ( 'NONE',  ( -37.00000000000000711, 11.32068061209295529, 5.865551165831118574 ) ) ;
#46019=VECTOR ( 'NONE', #675, 1000.000000000000000 ) ;
#46020=DIRECTION ( 'NONE',  ( 0.000000000000000000, 0.000000000000000000, -1.000000000000000000 ) ) ;
#46021=ORIENTED_EDGE ( 'NONE', *, *, #30308, .T. ) ;
#46023=CARTESIAN_POINT ( 'NONE',  ( 37.00000000000000711, 7.718225330433935660, 9.430788938293964918 ) ) ;
#46024=EDGE_CURVE ( 'NONE', #59239, #21159, #64472, .T. ) ;
#46025=ORIENTED_EDGE ( 'NONE', *, *, #24222, .T. ) ;
#46027=ORIENTED_EDGE ( 'NONE', *, *, #61526, .T. ) ;
#46028=EDGE_CURVE ( 'NONE', #57486, #58933, #32614, .T. ) ;
#46030=DIRECTION ( 'NONE',  ( 0.000000000000000000, 0.01356324068817998940, -0.9999080150203989437 ) ) ;
#46032=CYLINDRICAL_SURFACE ( 'NONE', #14184, 12.75000000000000178 ) ;
#46033=DIRECTION ( 'NONE',  ( -0.000000000000000000, -1.000000000000000000, -0.000000000000000000 ) ) ;
#46036=ADVANCED_FACE ( 'NONE', ( #44163 ), #13877, .T. ) ;
#46038=DIRECTION ( 'NONE',  ( 0.000000000000000000, 0.000000000000000000, -1.000000000000000000 ) ) ;
#46040=PLANE ( 'NONE',  #16109 ) ;
#46043=CYLINDRICAL_SURFACE ( 'NONE', #43383, 12.75000000000000178 ) ;
#46044=VERTEX_POINT ( 'NONE', #19218 ) ;
#46045=AXIS2_PLACEMENT_3D ( 'NONE', #9073, #34651, #34968 ) ;
#46048=ADVANCED_FACE ( 'NONE', ( #39492 ), #59789, .F. ) ;
#46050=AXIS2_PLACEMENT_3D ( 'NONE', #52058, #15799, #36077 ) ;
#46051=CARTESIAN_POINT ( 'NONE',  ( -10.48620311856347875, -9.720786832536937538, -7.036071585506805448 ) ) ;
#46053=DIRECTION ( 'NONE',  ( 1.000000000000000000, 0.000000000000000000, -0.000000000000000000 ) ) ;
#46054=CARTESIAN_POINT ( 'NONE',  ( -35.00000000000000000, 2.497432891017006718, -11.47758908105691766 ) ) ;
#46056=EDGE_CURVE ( 'NONE', #60869, #57837, #19912, .T. ) ;
#46057=EDGE_LOOP ( 'NONE', ( #46530, #2607, #64214, #29552 ) ) ;
#46058=EDGE_LOOP ( 'NONE', ( #28645, #5824, #65403, #65014 ) ) ;
#46064=VERTEX_POINT ( 'NONE', #56428 ) ;
#46065=CIRCLE ( 'NONE', #25883, 12.74999999999999822 ) ;
#46066=DIRECTION ( 'NONE',  ( 1.000000000000000000, 0.000000000000000000, 0.000000000000000000 ) ) ;
#46069=CARTESIAN_POINT ( 'NONE',  ( 17.20489889795780769, -8.941181588450204387, 8.020780947141853190 ) ) ;
#46071=VECTOR ( 'NONE', #795, 1000.000000000000000 ) ;
#46072=DIRECTION ( 'NONE',  ( 1.000000000000000000, 0.000000000000000000, 0.000000000000000000 ) ) ;
#46073=VECTOR ( 'NONE', #10042, 1000.000000000000000 ) ;
#46074=ORIENTED_EDGE ( 'NONE', *, *, #58476, .F. ) ;
#46075=VECTOR ( 'NONE', #16198, 1000.000000000000000 ) ;
#46076=CYLINDRICAL_SURFACE ( 'NONE', #11556, 5.000000000000000888 ) ;
#46080=CARTESIAN_POINT ( 'NONE',  ( 6.769303024027612636, -6.819793210492989033, 9.875810308326745002 ) ) ;
#46081=CIRCLE ( 'NONE', #27996, 12.74999999999999822 ) ;
#46082=CARTESIAN_POINT ( 'NONE',  ( -17.83419946441818027, -9.720786832536937538, 25.00000000000000000 ) ) ;
#46085=FACE_OUTER_BOUND ( 'NONE', #25084, .T. ) ;
#46086=ORIENTED_EDGE ( 'NONE', *, *, #13218, .T. ) ;
#46090=EDGE_CURVE ( 'NONE', #14897, #52497, #60768, .T. ) ;
#46091=AXIS2_PLACEMENT_3D ( 'NONE', #39486, #13556, #54802 ) ;
#46094=EDGE_CURVE ( 'NONE', #7532, #53819, #12787, .T. ) ;
#46096=FACE_OUTER_BOUND ( 'NONE', #19241, .T. ) ;
#46097=CIRCLE ( 'NONE', #63074, 12.18649999999999878 ) ;
#46100=CARTESIAN_POINT ( 'NONE',  ( -27.01437459610461644, 25.00000000000000000, -8.240233560378637634 ) ) ;
#46105=CARTESIAN_POINT ( 'NONE',  ( -14.74450257587757029, 7.920733541773330444, -9.014605533771735679 ) ) ;
#46106=CARTESIAN_POINT ( 'NONE',  ( 37.00000000000000711, 4.705694406421931860E-17, -3.469127814946512892E-15 ) ) ;
#46107=ADVANCED_FACE ( 'NONE', ( #30493 ), #36120, .T. ) ;
#46108=VECTOR ( 'NONE', #56352, 1000.000000000000000 ) ;
#46111=DIRECTION ( 'NONE',  ( 0.000000000000000000, 0.01356324068817992001, -0.9999080150203990547 ) ) ;
#46112=AXIS2_PLACEMENT_3D ( 'NONE', #31432, #6832, #62997 ) ;
#46113=CARTESIAN_POINT ( 'NONE',  ( 35.00000000000000000, -5.143145423404194894, 11.66664283989685025 ) ) ;
#46118=CARTESIAN_POINT ( 'NONE',  ( -37.00000000000000711, 0.000000000000000000, -1.750000000000000000 ) ) ;
#46119=VECTOR ( 'NONE', #400, 1000.000000000000000 ) ;
#46120=CARTESIAN_POINT ( 'NONE',  ( 35.00000000000000000, -2.185196060783960892, -11.54110654723648466 ) ) ;
#46122=VERTEX_POINT ( 'NONE', #61094 ) ;
#46123=DIRECTION ( 'NONE',  ( -1.000000000000000000, -0.000000000000000000, 0.000000000000000000 ) ) ;
#46124=ORIENTED_EDGE ( 'NONE', *, *, #38002, .T. ) ;
#46125=CARTESIAN_POINT ( 'NONE',  ( 35.00000000000000000, -1.488153103996881610, 11.65150730582935701 ) ) ;
#46129=EDGE_CURVE ( 'NONE', #51211, #24505, #4030, .T. ) ;
#46131=ORIENTED_EDGE ( 'NONE', *, *, #63153, .T. ) ;
#46135=ORIENTED_EDGE ( 'NONE', *, *, #48168, .F. ) ;
#46136=ORIENTED_EDGE ( 'NONE', *, *, #23419, .F. ) ;
#46138=CARTESIAN_POINT ( 'NONE',  ( 29.21347414222148942, -9.161122334729320471, 9.924607052662393514 ) ) ;
#46139=CIRCLE ( 'NONE', #17458, 12.75000000000000178 ) ;
#46140=AXIS2_PLACEMENT_3D ( 'NONE', #21563, #36838, #6599 ) ;
#46142=CARTESIAN_POINT ( 'NONE',  ( 22.11355691832442005, -11.89259483616537594, -1.644240265049296879 ) ) ;
#46145=CARTESIAN_POINT ( 'NONE',  ( -28.62125010117446777, 3.140874940710094876, 11.58806648538879358 ) ) ;
#46146=CARTESIAN_POINT ( 'NONE',  ( -35.00000000000000000, 3.340853584269533716, 11.26103545359857350 ) ) ;
#46148=CARTESIAN_POINT ( 'NONE',  ( -37.00000000000000711, 11.13736569743281457, -4.946702696913053643 ) ) ;
#46150=CARTESIAN_POINT ( 'NONE',  ( 36.00000000000000711, 10.49626516989280844, 7.238157050195514586 ) ) ;
#46152=CARTESIAN_POINT ( 'NONE',  ( 21.97631981833123049, 11.77024062219680012, -2.366125064793188848 ) ) ;
#46153=DIRECTION ( 'NONE',  ( 0.000000000000000000, 0.01356324068818000328, -0.9999080150203990547 ) ) ;
#46155=DIRECTION ( 'NONE',  ( 0.000000000000000000, -0.04924826701373154203, -0.9987865678893285137 ) ) ;
#46159=AXIS2_PLACEMENT_3D ( 'NONE', #29482, #49784, #4235 ) ;
#46161=ORIENTED_EDGE ( 'NONE', *, *, #42492, .T. ) ;
#46164=ORIENTED_EDGE ( 'NONE', *, *, #23972, .T. ) ;
#46165=CARTESIAN_POINT ( 'NONE',  ( 35.00000000000000000, 3.033604067594578790, -12.38385022362083276 ) ) ;
#46166=LINE ( 'NONE', #36824, #19740 ) ;
#46168=DIRECTION ( 'NONE',  ( -1.000000000000000000, 0.000000000000000000, 0.000000000000000000 ) ) ;
#46170=DIRECTION ( 'NONE',  ( 1.000000000000000000, -0.000000000000000000, 0.000000000000000000 ) ) ;
#46172=EDGE_CURVE ( 'NONE', #48483, #35632, #34791, .T. ) ;
#46175=AXIS2_PLACEMENT_3D ( 'NONE', #20547, #10544, #30822 ) ;
#46176=DIRECTION ( 'NONE',  ( 0.000000000000000000, -0.01356324068817992175, 0.9999080150203990547 ) ) ;
#46178=ORIENTED_EDGE ( 'NONE', *, *, #44799, .T. ) ;
#46181=FACE_OUTER_BOUND ( 'NONE', #30181, .T. ) ;
#46182=DIRECTION ( 'NONE',  ( -1.000000000000000000, 0.000000000000000000, 0.000000000000000000 ) ) ;
#46183=ADVANCED_FACE ( 'NONE', ( #42415 ), #22495, .T. ) ;
#46185=CARTESIAN_POINT ( 'NONE',  ( -30.15636683828732245, -0.5078987883301536721, -13.49786359043454986 ) ) ;
#46186=B_SPLINE_CURVE_WITH_KNOTS ( 'NONE', 3,
 ( #49380, #54349, #18768, #63630, #43691, #49676, #19425, #9102, #33396, #64303, #8132, #23765, #28728, #18459, #33713, #64612, #59016, #59323, #3494, #59654, #63978, #9406, #50003, #24076, #18105, #4120, #48700, #4462 ),
 .UNSPECIFIED., .F., .F.,
 ( 4, 2, 2, 2, 2, 2, 2, 2, 2, 2, 2, 2, 2, 4 ),
 ( 0.003178514824100456618, 0.003833261448045587744, 0.004488008071990718870, 0.005142754695935849996, 0.005797501319880981122, 0.007106994567771237302, 0.007761741191716364958, 0.008416487815661493482, 0.009725981063551748795, 0.01038072768749687645, 0.01103547431144200411, 0.01169022093538713003, 0.01234496755933225769, 0.01365446080722251126 ),
 .UNSPECIFIED. ) ;
#46189=VERTEX_POINT ( 'NONE', #11847 ) ;
#46191=DIRECTION ( 'NONE',  ( -1.000000000000000000, -0.000000000000000000, 0.000000000000000000 ) ) ;
#46195=VECTOR ( 'NONE', #65352, 1000.000000000000000 ) ;
#46197=CARTESIAN_POINT ( 'NONE',  ( -35.00000000000000000, 0.000000000000000000, 0.000000000000000000 ) ) ;
#46201=EDGE_LOOP ( 'NONE', ( #60860, #9259, #5320, #15103 ) ) ;
#46202=CARTESIAN_POINT ( 'NONE',  ( -8.434691090653316792, -7.831301396948528115, -9.099002668205912414 ) ) ;
#46205=EDGE_CURVE ( 'NONE', #36007, #52324, #25224, .T. ) ;
#46208=CARTESIAN_POINT ( 'NONE',  ( 18.84867683979355846, 5.944105725974518251, 12.12095735156415088 ) ) ;
#46209=ORIENTED_EDGE ( 'NONE', *, *, #30224, .T. ) ;
#46212=ORIENTED_EDGE ( 'NONE', *, *, #45762, .T. ) ;
#46214=CYLINDRICAL_SURFACE ( 'NONE', #56216, 12.18650000000000055 ) ;
#46217=VERTEX_POINT ( 'NONE', #32769 ) ;
#46219=ADVANCED_FACE ( 'NONE', ( #46779 ), #46450, .T. ) ;
#46220=CARTESIAN_POINT ( 'NONE',  ( 1.275613388608518362, 1.084079264376230256, 13.45952210748621170 ) ) ;
#46224=EDGE_LOOP ( 'NONE', ( #26568, #32201, #32594, #55017 ) ) ;
#46226=DIRECTION ( 'NONE',  ( 1.000000000000000000, 0.000000000000000000, 0.000000000000000000 ) ) ;
#46229=FACE_OUTER_BOUND ( 'NONE', #51149, .T. ) ;
#46230=CARTESIAN_POINT ( 'NONE',  ( -7.181456785175555524, 8.540743096806467705, -10.45493698471458188 ) ) ;
#46235=DIRECTION ( 'NONE',  ( 1.000000000000000000, 0.000000000000000000, 0.000000000000000000 ) ) ;
#46236=DIRECTION ( 'NONE',  ( 0.000000000000000000, -0.01356324068817991828, 0.9999080150203990547 ) ) ;
#46237=DIRECTION ( 'NONE',  ( -1.000000000000000000, 0.000000000000000000, 0.000000000000000000 ) ) ;
#46238=CIRCLE ( 'NONE', #4223, 12.18650000000000055 ) ;
#46240=CARTESIAN_POINT ( 'NONE',  ( -29.68541646480307250, -1.416020129149132334, 25.00000000000000000 ) ) ;
#46241=DIRECTION ( 'NONE',  ( -1.000000000000000000, 0.000000000000000000, 0.000000000000000000 ) ) ;
#46242=VERTEX_POINT ( 'NONE', #27157 ) ;
#46243=DIRECTION ( 'NONE',  ( 1.000000000000000000, -0.000000000000000000, 0.000000000000000000 ) ) ;
#46244=EDGE_CURVE ( 'NONE', #62469, #34225, #54985, .T. ) ;
#46245=AXIS2_PLACEMENT_3D ( 'NONE', #47552, #33569, #1997 ) ;
#46246=VERTEX_POINT ( 'NONE', #899 ) ;
#46250=FACE_OUTER_BOUND ( 'NONE', #28952, .T. ) ;
#46252=ORIENTED_EDGE ( 'NONE', *, *, #51640, .T. ) ;
#46253=CARTESIAN_POINT ( 'NONE',  ( 22.57855258442565116, 3.026812727784649493, 25.00000000000000000 ) ) ;
#46254=DIRECTION ( 'NONE',  ( 1.000000000000000000, 0.000000000000000000, 0.000000000000000000 ) ) ;
#46255=CARTESIAN_POINT ( 'NONE',  ( 22.21785366982988918, 10.35091871611333936, -6.082120259086551073 ) ) ;
#46256=CARTESIAN_POINT ( 'NONE',  ( 23.18962579211675390, -11.76234302143509680, -6.631918700726934901 ) ) ;
#46257=B_SPLINE_CURVE_WITH_KNOTS ( 'NONE', 3,
 ( #34902, #60865, #14623, #354, #7, #35890, #20293, #39915, #20635, #55210, #55552, #51233, #5683, #9312 ),
 .UNSPECIFIED., .F., .F.,
 ( 4, 2, 2, 2, 2, 2, 4 ),
 ( 0.000000000000000000, 0.001702703996761801208, 0.002554055995142702137, 0.003405407993523602416, 0.004256759991904502695, 0.005108111990285404275, 0.006810815987047202230 ),
 .UNSPECIFIED. ) ;
#46258=CIRCLE ( 'NONE', #51583, 5.000000000000000000 ) ;
#46260=DIRECTION ( 'NONE',  ( 1.000000000000000000, -0.000000000000000000, 0.000000000000000000 ) ) ;
#46261=LINE ( 'NONE', #15962, #51912 ) ;
#46263=EDGE_CURVE ( 'NONE', #63438, #18084, #21173, .T. ) ;
#46266=ADVANCED_FACE ( 'NONE', ( #33461 ), #53751, .T. ) ;
#46267=VECTOR ( 'NONE', #46321, 1000.000000000000000 ) ;
#46268=ORIENTED_EDGE ( 'NONE', *, *, #20837, .F. ) ;
#46269=ORIENTED_EDGE ( 'NONE', *, *, #43826, .F. ) ;
#46270=FACE_OUTER_BOUND ( 'NONE', #16628, .T. ) ;
#46276=VERTEX_POINT ( 'NONE', #28789 ) ;
#46279=LINE ( 'NONE', #20977, #41710 ) ;
#46281=CARTESIAN_POINT ( 'NONE',  ( 6.661533233520610331, -4.211056110068226666, 12.82664335996205196 ) ) ;
#46282=DIRECTION ( 'NONE',  ( -1.000000000000000000, 0.000000000000000000, 0.000000000000000000 ) ) ;
#46283=ORIENTED_EDGE ( 'NONE', *, *, #1748, .F. ) ;
#46284=VECTOR ( 'NONE', #18544, 1000.000000000000000 ) ;
#46287=CYLINDRICAL_SURFACE ( 'NONE', #44054, 10.70557198542813815 ) ;
#46289=CARTESIAN_POINT ( 'NONE',  ( -25.75517367794919465, 7.863739964200370025, 10.97545609339454664 ) ) ;
#46290=ORIENTED_EDGE ( 'NONE', *, *, #18450, .T. ) ;
#46292=EDGE_LOOP ( 'NONE', ( #4486, #35837, #61655, #8832 ) ) ;
#46293=VERTEX_POINT ( 'NONE', #34432 ) ;
#46294=DIRECTION ( 'NONE',  ( -1.000000000000000000, 0.000000000000000000, 0.000000000000000000 ) ) ;
#46297=EDGE_CURVE ( 'NONE', #27860, #34161, #17832, .T. ) ;
#46298=CARTESIAN_POINT ( 'NONE',  ( 36.00000000000000711, -3.473736367725341001, -12.26766708251990501 ) ) ;
#46299=CYLINDRICAL_SURFACE ( 'NONE', #38875, 13.50000000000000178 ) ;
#46300=CARTESIAN_POINT ( 'NONE',  ( 25.05309951391468459, -10.77522019223763827, -8.132934882857099979 ) ) ;
#46302=CARTESIAN_POINT ( 'NONE',  ( -37.00000000000000711, 0.06441628369853459601, -12.18632975068353197 ) ) ;
#46303=CARTESIAN_POINT ( 'NONE',  ( 3.459614771489464946, -11.09853614738469396, 7.685863346768216253 ) ) ;
#46305=DIRECTION ( 'NONE',  ( 0.000000000000000000, -0.01356324068817991828, 0.9999080150203990547 ) ) ;
#46306=ORIENTED_EDGE ( 'NONE', *, *, #22629, .F. ) ;
#46307=CARTESIAN_POINT ( 'NONE',  ( 12.14944607613469429, -13.35043466913572452, -2.010111617055820421 ) ) ;
#46308=CARTESIAN_POINT ( 'NONE',  ( -35.00000000000000000, 0.000000000000000000, 0.000000000000000000 ) ) ;
#46310=ORIENTED_EDGE ( 'NONE', *, *, #16371, .F. ) ;
#46311=CARTESIAN_POINT ( 'NONE',  ( 36.00000000000000711, -9.196955404009232282, 8.830544224263041642 ) ) ;
#46312=DIRECTION ( 'NONE',  ( 0.000000000000000000, 0.5767582926624912343, 0.8169148498130317515 ) ) ;
#46313=CARTESIAN_POINT ( 'NONE',  ( 36.00000000000000711, -6.950793414699864670, -10.68873102412840304 ) ) ;
#46314=FACE_OUTER_BOUND ( 'NONE', #41463, .T. ) ;
#46316=ORIENTED_EDGE ( 'NONE', *, *, #5099, .T. ) ;
#46317=CARTESIAN_POINT ( 'NONE',  ( -17.37691089814359913, -8.897415436183450765, -8.081796101290189327 ) ) ;
#46318=EDGE_CURVE ( 'NONE', #45959, #19382, #65556, .T. ) ;
#46319=VERTEX_POINT ( 'NONE', #19139 ) ;
#46321=DIRECTION ( 'NONE',  ( 1.000000000000000000, 0.000000000000000000, 0.000000000000000000 ) ) ;
#46322=EDGE_CURVE ( 'NONE', #15001, #48921, #33772, .T. ) ;
#46323=DIRECTION ( 'NONE',  ( -1.000000000000000000, 0.000000000000000000, 0.000000000000000000 ) ) ;
#46324=ORIENTED_EDGE ( 'NONE', *, *, #44285, .F. ) ;
#46326=EDGE_CURVE ( 'NONE', #57839, #9138, #13482, .T. ) ;
#46327=AXIS2_PLACEMENT_3D ( 'NONE', #47365, #7106, #27380 ) ;
#46328=CARTESIAN_POINT ( 'NONE',  ( 24.90014556888634800, -8.538933172091784485, -8.433831666448899256 ) ) ;
#46330=CARTESIAN_POINT ( 'NONE',  ( 35.00000000000000000, 4.705694406421931860E-17, -3.469127814946512892E-15 ) ) ;
#46334=FACE_OUTER_BOUND ( 'NONE', #1885, .T. ) ;
#46335=CARTESIAN_POINT ( 'NONE',  ( -35.00000000000000000, 0.000000000000000000, 0.000000000000000000 ) ) ;
#46337=CARTESIAN_POINT ( 'NONE',  ( -15.80994330493005329, 7.912403392364937282, 10.93820572742344233 ) ) ;
#46338=CARTESIAN_POINT ( 'NONE',  ( 18.50840396092215201, -8.755750366309635879, 10.29967764056247503 ) ) ;
#46339=VERTEX_POINT ( 'NONE', #24133 ) ;
#46341=CARTESIAN_POINT ( 'NONE',  ( 2.712198850443733100, 3.199880535692022576, -11.57168736659367703 ) ) ;
#46347=VERTEX_POINT ( 'NONE', #48111 ) ;
#46348=ORIENTED_EDGE ( 'NONE', *, *, #38027, .F. ) ;
#46350=EDGE_LOOP ( 'NONE', ( #31555, #39756, #33921, #26620 ) ) ;
#46351=DIRECTION ( 'NONE',  ( 0.000000000000000000, 0.01356324068817998940, -0.9999080150203990547 ) ) ;
#46355=ORIENTED_EDGE ( 'NONE', *, *, #48663, .F. ) ;
#46356=DIRECTION ( 'NONE',  ( -0.000000000000000000, -1.000000000000000000, -0.000000000000000000 ) ) ;
#46358=CARTESIAN_POINT ( 'NONE',  ( 37.00000000000000711, 3.916263239775349625, -11.07407352312214144 ) ) ;
#46359=CARTESIAN_POINT ( 'NONE',  ( 35.00000000000000000, 10.25474254703961918, 6.584150480049438592 ) ) ;
#46364=VERTEX_POINT ( 'NONE', #13178 ) ;
#46366=CARTESIAN_POINT ( 'NONE',  ( 35.00000000000000000, -8.029056188533749250, -8.573591947375291511 ) ) ;
#46370=ORIENTED_EDGE ( 'NONE', *, *, #55751, .F. ) ;
#46371=DIRECTION ( 'NONE',  ( 1.000000000000000000, 0.000000000000000000, 0.000000000000000000 ) ) ;
#46372=AXIS2_PLACEMENT_3D ( 'NONE', #3180, #27773, #28757 ) ;
#46374=ORIENTED_EDGE ( 'NONE', *, *, #10647, .F. ) ;
#46375=ORIENTED_EDGE ( 'NONE', *, *, #13754, .T. ) ;
#46377=VERTEX_POINT ( 'NONE', #58407 ) ;
#46379=DIRECTION ( 'NONE',  ( 0.000000000000000000, -0.01356324068817998940, 0.9999080150203990547 ) ) ;
#46380=DIRECTION ( 'NONE',  ( 1.000000000000000000, 0.000000000000000000, -0.000000000000000000 ) ) ;
#46381=DIRECTION ( 'NONE',  ( 1.000000000000000000, 0.000000000000000000, 0.000000000000000000 ) ) ;
#46383=CARTESIAN_POINT ( 'NONE',  ( 35.00000000000000000, 7.717887834988244045, -8.854740511458876639 ) ) ;
#46384=CARTESIAN_POINT ( 'NONE',  ( -36.00000000000000711, 11.32068061209295529, 5.865551165831118574 ) ) ;
#46386=EDGE_CURVE ( 'NONE', #36091, #31267, #17835, .T. ) ;
#46387=FACE_OUTER_BOUND ( 'NONE', #62460, .T. ) ;
#46388=EDGE_CURVE ( 'NONE', #20539, #54418, #40073, .T. ) ;
#46389=ORIENTED_EDGE ( 'NONE', *, *, #51478, .F. ) ;
#46392=CARTESIAN_POINT ( 'NONE',  ( 4.897912363208013709, -9.936743041242092289, 6.735674725481181291 ) ) ;
#46393=DIRECTION ( 'NONE',  ( -1.000000000000000000, -0.000000000000000000, 0.000000000000000000 ) ) ;
#46395=CARTESIAN_POINT ( 'NONE',  ( 24.07798446190206221, 1.048718167601086826, -13.46309495289836100 ) ) ;
#46397=CARTESIAN_POINT ( 'NONE',  ( 3.925267077142222671, 5.821403683822743425, -10.49580640056087155 ) ) ;
#46398=CARTESIAN_POINT ( 'NONE',  ( 9.743605816575051648, 1.293910771361904910, -11.93188251073744865 ) ) ;
#46399=ORIENTED_EDGE ( 'NONE', *, *, #11770, .T. ) ;
#46400=CYLINDRICAL_SURFACE ( 'NONE', #17623, 12.75000000000000178 ) ;
#46401=DIRECTION ( 'NONE',  ( 0.000000000000000000, 0.3554799084908900619, 0.9346839223284567622 ) ) ;
#46402=LINE ( 'NONE', #65672, #13154 ) ;
#46405=EDGE_CURVE ( 'NONE', #42318, #17913, #45718, .T. ) ;
#46406=CARTESIAN_POINT ( 'NONE',  ( -25.25756445130008387, 9.783230075093738876, 6.955975781903453559 ) ) ;
#46408=( BOUNDED_CURVE ( )  B_SPLINE_CURVE ( 3, ( #14021, #28665, #63913, #23702 ),
 .UNSPECIFIED., .F., .F. ) 
 B_SPLINE_CURVE_WITH_KNOTS ( ( 4, 4 ),
 ( 4.526278477422524205, 4.545842283345725932 ),
 .UNSPECIFIED. ) 
 CURVE ( )  GEOMETRIC_REPRESENTATION_ITEM ( )  RATIONAL_B_SPLINE_CURVE ( ( 1.000000000000000000, 0.9999681050458084641, 0.9999681050458084641, 1.000000000000000000 ) ) 
 REPRESENTATION_ITEM ( '' )  );
#46411=DIRECTION ( 'NONE',  ( -0.000000000000000000, -1.000000000000000000, -0.000000000000000000 ) ) ;
#46413=EDGE_CURVE ( 'NONE', #57223, #61765, #5074, .T. ) ;
#46415=CARTESIAN_POINT ( 'NONE',  ( -9.351388602708162523, -12.99278190472486827, -3.665735721005250358 ) ) ;
#46417=DIRECTION ( 'NONE',  ( 0.000000000000000000, 0.01356324068817998940, -0.9999080150203990547 ) ) ;
#46418=FACE_OUTER_BOUND ( 'NONE', #47194, .T. ) ;
#46420=CARTESIAN_POINT ( 'NONE',  ( 35.00000000000000000, 4.705694406421931860E-17, -3.469127814946512892E-15 ) ) ;
#46422=ORIENTED_EDGE ( 'NONE', *, *, #20872, .T. ) ;
#46424=DIRECTION ( 'NONE',  ( 1.000000000000000000, 0.000000000000000000, 0.000000000000000000 ) ) ;
#46425=CARTESIAN_POINT ( 'NONE',  ( 35.00000000000000000, 9.677500615117898164, -6.657191900728355094 ) ) ;
#46426=CARTESIAN_POINT ( 'NONE',  ( -35.00000000000000000, -12.14284015767849390, -1.030638227056693834 ) ) ;
#46431=ORIENTED_EDGE ( 'NONE', *, *, #46090, .T. ) ;
#46433=ORIENTED_EDGE ( 'NONE', *, *, #64611, .T. ) ;
#46434=CARTESIAN_POINT ( 'NONE',  ( 37.00000000000000711, 3.645068577060024850, -11.16627499335656815 ) ) ;
#46438=ORIENTED_EDGE ( 'NONE', *, *, #34931, .F. ) ;
#46440=DIRECTION ( 'NONE',  ( 0.000000000000000000, -0.01356324068817991828, 0.9999080150203990547 ) ) ;
#46441=FACE_BOUND ( 'NONE', #3269, .T. ) ;
#46442=ORIENTED_EDGE ( 'NONE', *, *, #46604, .F. ) ;
#46444=CARTESIAN_POINT ( 'NONE',  ( 3.291290029914074378, 8.250315036047103590, 25.00000000000000000 ) ) ;
#46446=ORIENTED_EDGE ( 'NONE', *, *, #29158, .F. ) ;
#46449=CARTESIAN_POINT ( 'NONE',  ( -35.00000000000000000, 11.91791701451266405, 2.544412758415886877 ) ) ;
#46450=CYLINDRICAL_SURFACE ( 'NONE', #31588, 12.74999999999999822 ) ;
#46451=FACE_OUTER_BOUND ( 'NONE', #13318, .T. ) ;
#46454=VECTOR ( 'NONE', #57007, 1000.000000000000000 ) ;
#46455=LINE ( 'NONE', #6564, #64146 ) ;
#46456=EDGE_LOOP ( 'NONE', ( #33025, #20611, #52026, #40610 ) ) ;
#46461=DIRECTION ( 'NONE',  ( 1.000000000000000000, 0.000000000000000000, 0.000000000000000000 ) ) ;
#46462=DIRECTION ( 'NONE',  ( 0.000000000000000000, -0.01356324068817998940, 0.9999080150203990547 ) ) ;
#46467=ORIENTED_EDGE ( 'NONE', *, *, #23504, .T. ) ;
#46468=DIRECTION ( 'NONE',  ( 0.000000000000000000, -0.01356324068817998940, 0.9999080150203990547 ) ) ;
#46469=ORIENTED_EDGE ( 'NONE', *, *, #9217, .T. ) ;
#46470=CARTESIAN_POINT ( 'NONE',  ( 37.00000000000000711, 4.705694406421931860E-17, -3.469127814946512892E-15 ) ) ;
#46475=EDGE_CURVE ( 'NONE', #23572, #62927, #47555, .T. ) ;
#46476=EDGE_LOOP ( 'NONE', ( #47609, #7994, #31158, #9973, #62149, #33830 ) ) ;
#46483=AXIS2_PLACEMENT_3D ( 'NONE', #36205, #5997, #62153 ) ;
#46484=EDGE_CURVE ( 'NONE', #19993, #59672, #18883, .T. ) ;
#46486=LINE ( 'NONE', #15876, #45701 ) ;
#46487=VECTOR ( 'NONE', #27475, 1000.000000000000000 ) ;
#46488=ORIENTED_EDGE ( 'NONE', *, *, #36342, .T. ) ;
#46489=DIRECTION ( 'NONE',  ( 0.000000000000000000, -0.01356324068817998940, 0.9999080150203990547 ) ) ;
#46490=EDGE_CURVE ( 'NONE', #9134, #48396, #56029, .T. ) ;
#46491=ORIENTED_EDGE ( 'NONE', *, *, #20555, .T. ) ;
#46492=CARTESIAN_POINT ( 'NONE',  ( 35.00000000000000000, -12.05416472667166516, -1.791059740004382617 ) ) ;
#46495=AXIS2_PLACEMENT_3D ( 'NONE', #37375, #56350, #41714 ) ;
#46498=ORIENTED_EDGE ( 'NONE', *, *, #57607, .T. ) ;
#46499=ORIENTED_EDGE ( 'NONE', *, *, #61348, .T. ) ;
#46501=ORIENTED_EDGE ( 'NONE', *, *, #6592, .F. ) ;
#46502=DIRECTION ( 'NONE',  ( 0.000000000000000000, 0.3807014730195220631, -0.9246979985058721985 ) ) ;
#46504=DIRECTION ( 'NONE',  ( 1.000000000000000000, 0.000000000000000000, -0.000000000000000000 ) ) ;
#46507=CARTESIAN_POINT ( 'NONE',  ( 10.75853767213705225, 7.830989516993144051, -9.092612561015865680 ) ) ;
#46508=CARTESIAN_POINT ( 'NONE',  ( -11.40165637463000081, -7.157122913318663571, 9.642566250083232759 ) ) ;
#46510=CARTESIAN_POINT ( 'NONE',  ( 37.00000000000000711, 4.705694406421931860E-17, -3.469127814946512892E-15 ) ) ;
#46511=EDGE_LOOP ( 'NONE', ( #44526, #34542, #50099, #45644 ) ) ;
#46514=EDGE_CURVE ( 'NONE', #48534, #54954, #829, .T. ) ;
#46519=CYLINDRICAL_SURFACE ( 'NONE', #29080, 5.000000000000000888 ) ;
#46522=VERTEX_POINT ( 'NONE', #11143 ) ;
#46523=ORIENTED_EDGE ( 'NONE', *, *, #29208, .F. ) ;
#46524=DIRECTION ( 'NONE',  ( -1.000000000000000000, 0.000000000000000000, 0.000000000000000000 ) ) ;
#46526=CYLINDRICAL_SURFACE ( 'NONE', #53942, 5.000000000000000888 ) ;
#46527=ORIENTED_EDGE ( 'NONE', *, *, #65726, .T. ) ;
#46528=EDGE_CURVE ( 'NONE', #3374, #62061, #52867, .T. ) ;
#46530=ORIENTED_EDGE ( 'NONE', *, *, #39954, .T. ) ;
#46531=DIRECTION ( 'NONE',  ( -1.000000000000000000, 0.000000000000000000, 0.000000000000000000 ) ) ;
#46533=AXIS2_PLACEMENT_3D ( 'NONE', #6966, #36885, #27236 ) ;
#46536=CARTESIAN_POINT ( 'NONE',  ( -35.00000000000000000, -10.43555801961479190, 5.391785509270926369 ) ) ;
#46538=CARTESIAN_POINT ( 'NONE',  ( -37.00000000000000711, -12.74613886779085270, 0.3137578094508789439 ) ) ;
#46539=CIRCLE ( 'NONE', #7274, 12.18650000000000055 ) ;
#46540=VERTEX_POINT ( 'NONE', #52031 ) ;
#46544=DIRECTION ( 'NONE',  ( 0.000000000000000000, 0.000000000000000000, -1.000000000000000000 ) ) ;
#46548=DIRECTION ( 'NONE',  ( 0.000000000000000000, 0.01356324068818000328, -0.9999080150203990547 ) ) ;
#46550=CIRCLE ( 'NONE', #2999, 5.000000000000000000 ) ;
#46551=EDGE_CURVE ( 'NONE', #11376, #37516, #32652, .T. ) ;
#46552=ORIENTED_EDGE ( 'NONE', *, *, #11490, .F. ) ;
#46553=CARTESIAN_POINT ( 'NONE',  ( -35.00000000000000000, -4.725891942574680371, -10.75351884295732496 ) ) ;
#46554=ORIENTED_EDGE ( 'NONE', *, *, #52857, .T. ) ;
#46558=DIRECTION ( 'NONE',  ( -1.000000000000000000, 0.000000000000000000, 0.000000000000000000 ) ) ;
#46560=VERTEX_POINT ( 'NONE', #21443 ) ;
#46561=DIRECTION ( 'NONE',  ( 0.000000000000000000, -0.5767582926625031137, -0.8169148498130233138 ) ) ;
#46562=CARTESIAN_POINT ( 'NONE',  ( -37.00000000000000711, 4.041347439435861943, 11.02904044024210428 ) ) ;
#46563=CARTESIAN_POINT ( 'NONE',  ( -37.00000000000000711, 11.74614673114903951, 0.01609748574465447862 ) ) ;
#46564=CARTESIAN_POINT ( 'NONE',  ( 21.94480751494469573, -13.23013732071854065, -2.711352612237130977 ) ) ;
#46565=ADVANCED_FACE ( 'NONE', ( #62629 ), #52371, .T. ) ;
#46566=CIRCLE ( 'NONE', #48707, 12.18650000000000233 ) ;
#46567=ADVANCED_FACE ( 'NONE', ( #26755 ), #52692, .T. ) ;
#46571=EDGE_CURVE ( 'NONE', #56112, #3010, #1508, .T. ) ;
#46572=LINE ( 'NONE', #12962, #56448 ) ;
#46574=CARTESIAN_POINT ( 'NONE',  ( 35.00000000000000000, 2.346765782874432382, -11.95840593935202278 ) ) ;
#46575=AXIS2_PLACEMENT_3D ( 'NONE', #38780, #63057, #59078 ) ;
#46578=AXIS2_PLACEMENT_3D ( 'NONE', #32325, #47967, #48626 ) ;
#46579=EDGE_LOOP ( 'NONE', ( #56012, #12060, #7220, #50244 ) ) ;
#46582=LINE ( 'NONE', #9684, #19423 ) ;
#46583=AXIS2_PLACEMENT_3D ( 'NONE', #7351, #2051, #17351 ) ;
#46585=ORIENTED_EDGE ( 'NONE', *, *, #24430, .F. ) ;
#46586=ORIENTED_EDGE ( 'NONE', *, *, #51761, .T. ) ;
#46589=CARTESIAN_POINT ( 'NONE',  ( 28.16540852905778181, -10.96212297253492807, 4.899974118361737574 ) ) ;
#46590=CARTESIAN_POINT ( 'NONE',  ( 35.00000000000000000, 8.534258022646096009, -8.699265615723016154 ) ) ;
#46592=CARTESIAN_POINT ( 'NONE',  ( -37.00000000000000711, -5.428340790341781741, 10.91072401419408777 ) ) ;
#46593=DIRECTION ( 'NONE',  ( 1.000000000000000000, 0.000000000000000000, 0.000000000000000000 ) ) ;
#46599=DIRECTION ( 'NONE',  ( 0.000000000000000000, 0.01356324068817992175, -0.9999080150203990547 ) ) ;
#46601=DIRECTION ( 'NONE',  ( -1.000000000000000000, 0.000000000000000000, 0.000000000000000000 ) ) ;
#46602=ORIENTED_EDGE ( 'NONE', *, *, #14071, .F. ) ;
#46603=CYLINDRICAL_SURFACE ( 'NONE', #11395, 4.999999999999999112 ) ;
#46604=EDGE_CURVE ( 'NONE', #45916, #36640, #34018, .T. ) ;
#46605=CARTESIAN_POINT ( 'NONE',  ( 9.687175622948609899, -11.98570860552670325, -0.5854820436212360146 ) ) ;
#46606=DIRECTION ( 'NONE',  ( -1.000000000000000000, 0.000000000000000000, 0.000000000000000000 ) ) ;
#46608=DIRECTION ( 'NONE',  ( -1.000000000000000000, 0.000000000000000000, 0.000000000000000000 ) ) ;
#46609=AXIS2_PLACEMENT_3D ( 'NONE', #60213, #44261, #14635 ) ;
#46610=CARTESIAN_POINT ( 'NONE',  ( 35.00000000000000000, 4.705694406421931860E-17, -3.469127814946512892E-15 ) ) ;
#46614=CARTESIAN_POINT ( 'NONE',  ( 7.043522766805570434, -7.889587943819550198, 10.96282566889193966 ) ) ;
#46616=DIRECTION ( 'NONE',  ( -1.000000000000000000, 0.000000000000000000, 0.000000000000000000 ) ) ;
#46617=ORIENTED_EDGE ( 'NONE', *, *, #62763, .F. ) ;
#46621=EDGE_CURVE ( 'NONE', #19062, #65236, #44324, .T. ) ;
#46623=ORIENTED_EDGE ( 'NONE', *, *, #58258, .F. ) ;
#46626=DIRECTION ( 'NONE',  ( -1.000000000000000000, 0.000000000000000000, -0.000000000000000000 ) ) ;
#46627=LINE ( 'NONE', #56953, #1929 ) ;
#46628=AXIS2_PLACEMENT_3D ( 'NONE', #26105, #6812, #1818 ) ;
#46629=ADVANCED_FACE ( 'NONE', ( #64291 ), #13735, .T. ) ;
#46630=AXIS2_PLACEMENT_3D ( 'NONE', #1930, #22199, #37830 ) ;
#46632=ORIENTED_EDGE ( 'NONE', *, *, #30455, .T. ) ;
#46633=CARTESIAN_POINT ( 'NONE',  ( 36.00000000000000711, -11.32068061209299259, -5.865551165831042191 ) ) ;
#46634=VERTEX_POINT ( 'NONE', #54335 ) ;
#46636=CARTESIAN_POINT ( 'NONE',  ( -35.00000000000000000, 5.644643009979071202, 10.30098186818251982 ) ) ;
#46637=CARTESIAN_POINT ( 'NONE',  ( 37.00000000000000711, -10.49591321039684289, -5.273331777780305707 ) ) ;
#46638=VERTEX_POINT ( 'NONE', #58010 ) ;
#46639=CIRCLE ( 'NONE', #56174, 5.000000000000001776 ) ;
#46641=EDGE_CURVE ( 'NONE', #50238, #1113, #33037, .T. ) ;
#46644=LINE ( 'NONE', #57286, #44810 ) ;
#46646=CARTESIAN_POINT ( 'NONE',  ( 37.00000000000000711, 3.511814412392283646, 11.66953048682395355 ) ) ;
#46650=CIRCLE ( 'NONE', #53015, 12.18649999999999878 ) ;
#46651=EDGE_LOOP ( 'NONE', ( #30225, #626, #42892, #58794 ) ) ;
#46652=CARTESIAN_POINT ( 'NONE',  ( -16.26295706671148977, 7.784749528947430441, 11.02953652074824653 ) ) ;
#46653=CARTESIAN_POINT ( 'NONE',  ( -35.00000000000000000, -8.954052073409537016, -9.076753354954094632 ) ) ;
#46656=DIRECTION ( 'NONE',  ( -1.000000000000000000, 0.000000000000000000, -0.000000000000000000 ) ) ;
#46657=CARTESIAN_POINT ( 'NONE',  ( 9.272947129449288894, 6.113238480130934960, -10.33161780435538724 ) ) ;
#46660=DIRECTION ( 'NONE',  ( 0.000000000000000000, 0.01356324068817998940, -0.9999080150203990547 ) ) ;
#46663=VERTEX_POINT ( 'NONE', #32691 ) ;
#46664=ORIENTED_EDGE ( 'NONE', *, *, #57349, .T. ) ;
#46665=CYLINDRICAL_SURFACE ( 'NONE', #26313, 13.50000000000000178 ) ;
#46666=ORIENTED_EDGE ( 'NONE', *, *, #57973, .T. ) ;
#46667=CARTESIAN_POINT ( 'NONE',  ( -35.00000000000000000, 0.000000000000000000, 0.000000000000000000 ) ) ;
#46669=CIRCLE ( 'NONE', #25451, 12.75000000000000178 ) ;
#46670=DIRECTION ( 'NONE',  ( -1.000000000000000000, -0.000000000000000000, 0.000000000000000000 ) ) ;
#46672=EDGE_CURVE ( 'NONE', #61242, #20003, #55036, .T. ) ;
#46674=DIRECTION ( 'NONE',  ( 1.000000000000000000, 0.000000000000000000, 0.000000000000000000 ) ) ;
#46677=DIRECTION ( 'NONE',  ( -0.000000000000000000, -0.000000000000000000, -1.000000000000000000 ) ) ;
#46678=ORIENTED_EDGE ( 'NONE', *, *, #32633, .F. ) ;
#46679=ADVANCED_FACE ( 'NONE', ( #3481 ), #53005, .T. ) ;
#46681=ORIENTED_EDGE ( 'NONE', *, *, #50156, .T. ) ;
#46682=DIRECTION ( 'NONE',  ( -1.000000000000000000, 0.000000000000000000, 0.000000000000000000 ) ) ;
#46683=VECTOR ( 'NONE', #42165, 1000.000000000000000 ) ;
#46684=ORIENTED_EDGE ( 'NONE', *, *, #25201, .T. ) ;
#46685=CYLINDRICAL_SURFACE ( 'NONE', #54949, 4.999999999999999112 ) ;
#46687=DIRECTION ( 'NONE',  ( 0.000000000000000000, -0.1118654143051685257, -0.9937233664769753450 ) ) ;
#46688=ORIENTED_EDGE ( 'NONE', *, *, #13218, .F. ) ;
#46689=EDGE_CURVE ( 'NONE', #16670, #40781, #13100, .T. ) ;
#46690=DIRECTION ( 'NONE',  ( 1.000000000000000000, 0.000000000000000000, 0.000000000000000000 ) ) ;
#46691=CARTESIAN_POINT ( 'NONE',  ( -20.33921151711751207, 11.75255037028624017, -2.499576093431243873 ) ) ;
#46693=EDGE_LOOP ( 'NONE', ( #9305, #35808, #3245, #40126 ) ) ;
#46696=CYLINDRICAL_SURFACE ( 'NONE', #12531, 10.20557198542813815 ) ;
#46697=ORIENTED_EDGE ( 'NONE', *, *, #17039, .F. ) ;
#46698=VERTEX_POINT ( 'NONE', #33380 ) ;
#46700=DIRECTION ( 'NONE',  ( -1.000000000000000000, 0.000000000000000000, 0.000000000000000000 ) ) ;
#46702=FACE_OUTER_BOUND ( 'NONE', #30800, .T. ) ;
#46705=CIRCLE ( 'NONE', #20125, 12.18649999999999878 ) ;
#46706=AXIS2_PLACEMENT_3D ( 'NONE', #15213, #50490, #30820 ) ;
#46707=DIRECTION ( 'NONE',  ( 0.000000000000000000, 0.01356324068817991481, -0.9999080150203990547 ) ) ;
#46709=ORIENTED_EDGE ( 'NONE', *, *, #18619, .T. ) ;
#46714=DIRECTION ( 'NONE',  ( 1.000000000000000000, -0.000000000000000000, 0.000000000000000000 ) ) ;
#46715=LINE ( 'NONE', #26118, #14091 ) ;
#46716=AXIS2_PLACEMENT_3D ( 'NONE', #29551, #44860, #19275 ) ;
#46718=CARTESIAN_POINT ( 'NONE',  ( -35.00000000000000000, 12.74068829017553917, 0.4871980014161916284 ) ) ;
#46719=DIRECTION ( 'NONE',  ( 0.000000000000000000, 0.01356324068817998940, -0.9999080150203990547 ) ) ;
#46721=DIRECTION ( 'NONE',  ( -1.000000000000000000, 0.000000000000000000, 0.000000000000000000 ) ) ;
#46725=CYLINDRICAL_SURFACE ( 'NONE', #26967, 13.50000000000000178 ) ;
#46726=AXIS2_PLACEMENT_3D ( 'NONE', #39563, #14928, #59866 ) ;
#46727=EDGE_CURVE ( 'NONE', #48921, #52081, #43022, .T. ) ;
#46730=EDGE_LOOP ( 'NONE', ( #58466, #25614, #56921, #47250 ) ) ;
#46731=DIRECTION ( 'NONE',  ( -1.000000000000000000, 0.000000000000000000, 0.000000000000000000 ) ) ;
#46732=DIRECTION ( 'NONE',  ( 0.000000000000000000, 0.6269146997507929475, 0.7790879021242551605 ) ) ;
#46734=EDGE_LOOP ( 'NONE', ( #10578, #50515, #31195, #28050 ) ) ;
#46736=FACE_OUTER_BOUND ( 'NONE', #65537, .T. ) ;
#46737=DIRECTION ( 'NONE',  ( 0.000000000000000000, -0.01356324068817991828, 0.9999080150203990547 ) ) ;
#46738=CARTESIAN_POINT ( 'NONE',  ( -35.00000000000000000, -11.17622378668009020, 3.614449339633449387 ) ) ;
#46746=VERTEX_POINT ( 'NONE', #23749 ) ;
#46747=CARTESIAN_POINT ( 'NONE',  ( -35.00000000000000000, 0.000000000000000000, 0.000000000000000000 ) ) ;
#46748=DIRECTION ( 'NONE',  ( 0.000000000000000000, -0.8696919319575238116, -0.4935949184179166949 ) ) ;
#46750=CARTESIAN_POINT ( 'NONE',  ( -3.986346267772003404, -10.46471259782063967, 8.566942944689746042 ) ) ;
#46751=EDGE_CURVE ( 'NONE', #32447, #63134, #65599, .T. ) ;
#46752=CARTESIAN_POINT ( 'NONE',  ( -8.294914047376659383, 6.473484522924868756, -10.13498875827578516 ) ) ;
#46753=DIRECTION ( 'NONE',  ( -0.000000000000000000, -0.000000000000000000, -1.000000000000000000 ) ) ;
#46754=CARTESIAN_POINT ( 'NONE',  ( 36.00000000000000711, -11.73555825188272905, 4.983891302653701061 ) ) ;
#46755=ORIENTED_EDGE ( 'NONE', *, *, #27251, .F. ) ;
#46756=EDGE_CURVE ( 'NONE', #32028, #10291, #30661, .T. ) ;
#46757=ORIENTED_EDGE ( 'NONE', *, *, #32975, .F. ) ;
#46758=CARTESIAN_POINT ( 'NONE',  ( -35.00000000000000000, -10.39746860227885428, -7.379373053628982326 ) ) ;
#46759=ORIENTED_EDGE ( 'NONE', *, *, #36622, .F. ) ;
#46761=AXIS2_PLACEMENT_3D ( 'NONE', #10590, #20902, #31223 ) ;
#46763=EDGE_CURVE ( 'NONE', #3878, #61089, #45441, .T. ) ;
#46764=FACE_OUTER_BOUND ( 'NONE', #50071, .T. ) ;
#46767=DIRECTION ( 'NONE',  ( -1.000000000000000000, 0.000000000000000000, 0.000000000000000000 ) ) ;
#46769=DIRECTION ( 'NONE',  ( 1.000000000000000000, 0.000000000000000000, 0.000000000000000000 ) ) ;
#46771=ORIENTED_EDGE ( 'NONE', *, *, #22245, .T. ) ;
#46773=DIRECTION ( 'NONE',  ( 0.9207114435679737419, 0.000000000000000000, -0.3902440745007897949 ) ) ;
#46774=VERTEX_POINT ( 'NONE', #25359 ) ;
#46776=CARTESIAN_POINT ( 'NONE',  ( 35.00000000000000000, 4.705694406421931860E-17, -3.469127814946512892E-15 ) ) ;
#46778=CARTESIAN_POINT ( 'NONE',  ( 10.28770264580773741, 1.469485120472078465, 13.42064909261541317 ) ) ;
#46779=FACE_OUTER_BOUND ( 'NONE', #60553, .T. ) ;
#46780=CARTESIAN_POINT ( 'NONE',  ( 37.00000000000000711, -9.700295462048712736, -7.376655759824850556 ) ) ;
#46781=DIRECTION ( 'NONE',  ( -1.000000000000000000, -0.000000000000000000, -0.000000000000000000 ) ) ;
#46782=EDGE_CURVE ( 'NONE', #60035, #40488, #52905, .T. ) ;
#46783=DIRECTION ( 'NONE',  ( 0.000000000000000000, -0.2006870767258747690, 0.9796553971857770993 ) ) ;
#46787=CARTESIAN_POINT ( 'NONE',  ( 22.36482863261543486, 11.96441317219527889, -0.9234811557364158707 ) ) ;
#46791=DIRECTION ( 'NONE',  ( -1.000000000000000000, 0.000000000000000000, 0.000000000000000000 ) ) ;
#46795=VECTOR ( 'NONE', #63740, 1000.000000000000000 ) ;
#46798=VERTEX_POINT ( 'NONE', #19409 ) ;
#46805=DIRECTION ( 'NONE',  ( 0.000000000000000000, 0.01356324068817998940, -0.9999080150203989437 ) ) ;
#46807=FACE_OUTER_BOUND ( 'NONE', #63064, .T. ) ;
#46809=EDGE_CURVE ( 'NONE', #25218, #47218, #6167, .T. ) ;
#46810=CIRCLE ( 'NONE', #47909, 5.000000000000000888 ) ;
#46811=VECTOR ( 'NONE', #3567, 1000.000000000000000 ) ;
#46812=CARTESIAN_POINT ( 'NONE',  ( 37.00000000000000711, 12.26766708251991567, -3.473736367725300145 ) ) ;
#46815=ORIENTED_EDGE ( 'NONE', *, *, #36881, .T. ) ;
#46817=ORIENTED_EDGE ( 'NONE', *, *, #59126, .F. ) ;
#46818=CARTESIAN_POINT ( 'NONE',  ( -37.00000000000000711, -2.080187960898652655, 12.57916205664480636 ) ) ;
#46819=CARTESIAN_POINT ( 'NONE',  ( -37.00000000000000711, -8.258652103341496797, 8.352657516904644197 ) ) ;
#46820=DIRECTION ( 'NONE',  ( 1.000000000000000000, 0.000000000000000000, 0.000000000000000000 ) ) ;
#46821=AXIS2_PLACEMENT_3D ( 'NONE', #14944, #24619, #35235 ) ;
#46823=DIRECTION ( 'NONE',  ( 0.000000000000000000, 0.01356324068817998940, -0.9999080150203989437 ) ) ;
#46825=ORIENTED_EDGE ( 'NONE', *, *, #53688, .F. ) ;
#46826=ORIENTED_EDGE ( 'NONE', *, *, #50266, .F. ) ;
#46827=FACE_OUTER_BOUND ( 'NONE', #6629, .T. ) ;
#46829=CIRCLE ( 'NONE', #18174, 12.18650000000000055 ) ;
#46830=LINE ( 'NONE', #5970, #36192 ) ;
#46833=CARTESIAN_POINT ( 'NONE',  ( 37.00000000000000711, -12.17626345777663310, 0.4993900848168664752 ) ) ;
#46834=CYLINDRICAL_SURFACE ( 'NONE', #10966, 12.75000000000000178 ) ;
#46835=EDGE_CURVE ( 'NONE', #51873, #18418, #9352, .T. ) ;
#46838=ORIENTED_EDGE ( 'NONE', *, *, #36964, .T. ) ;
#46839=AXIS2_PLACEMENT_3D ( 'NONE', #27119, #6847, #22449 ) ;
#46840=EDGE_CURVE ( 'NONE', #55692, #48877, #50335, .T. ) ;
#46842=ORIENTED_EDGE ( 'NONE', *, *, #50230, .T. ) ;
#46843=LINE ( 'NONE', #1308, #64140 ) ;
#46844=CIRCLE ( 'NONE', #28752, 12.18650000000000055 ) ;
#46846=VECTOR ( 'NONE', #1521, 1000.000000000000000 ) ;
#46847=CIRCLE ( 'NONE', #13882, 4.999999999999999112 ) ;
#46848=CYLINDRICAL_SURFACE ( 'NONE', #39395, 4.999999999999999112 ) ;
#46849=ORIENTED_EDGE ( 'NONE', *, *, #7887, .T. ) ;
#46852=CIRCLE ( 'NONE', #26678, 4.999999999999999112 ) ;
#46853=LINE ( 'NONE', #21594, #19105 ) ;
#46854=EDGE_CURVE ( 'NONE', #38347, #64141, #46550, .T. ) ;
#46855=ORIENTED_EDGE ( 'NONE', *, *, #6676, .T. ) ;
#46856=ORIENTED_EDGE ( 'NONE', *, *, #30741, .F. ) ;
#46857=CARTESIAN_POINT ( 'NONE',  ( 2.846142546918067229, 3.504604795492467062, 13.04310330258398487 ) ) ;
#46860=DIRECTION ( 'NONE',  ( 0.000000000000000000, -0.6943713148249690548, 0.7196168960969744344 ) ) ;
#46863=ORIENTED_EDGE ( 'NONE', *, *, #7054, .F. ) ;
#46864=EDGE_CURVE ( 'NONE', #43014, #31870, #20374, .T. ) ;
#46865=AXIS2_PLACEMENT_3D ( 'NONE', #42484, #51847, #62142 ) ;
#46868=CIRCLE ( 'NONE', #161, 5.000000000000000000 ) ;
#46871=CARTESIAN_POINT ( 'NONE',  ( -35.00000000000000000, 4.545979934229578134, -11.30684963584384128 ) ) ;
#46873=AXIS2_PLACEMENT_3D ( 'NONE', #25788, #32960, #22329 ) ;
#46874=ADVANCED_FACE ( 'NONE', ( #15387 ), #35658, .T. ) ;
#46877=CARTESIAN_POINT ( 'NONE',  ( -10.48620311856347875, -9.720786832536937538, -9.367833439828894271 ) ) ;
#46878=DIRECTION ( 'NONE',  ( 1.000000000000000000, 0.000000000000000000, -0.000000000000000000 ) ) ;
#46879=VECTOR ( 'NONE', #54305, 1000.000000000000000 ) ;
#46880=EDGE_CURVE ( 'NONE', #34055, #53931, #46627, .T. ) ;
#46881=DIRECTION ( 'NONE',  ( 0.000000000000000000, 0.01356324068817992175, -0.9999080150203990547 ) ) ;
#46885=ORIENTED_EDGE ( 'NONE', *, *, #45284, .F. ) ;
#46887=AXIS2_PLACEMENT_3D ( 'NONE', #14939, #10612, #30898 ) ;
#46892=AXIS2_PLACEMENT_3D ( 'NONE', #13389, #54933, #29648 ) ;
#46894=AXIS2_PLACEMENT_3D ( 'NONE', #50201, #46504, #36179 ) ;
#46895=DIRECTION ( 'NONE',  ( -0.000000000000000000, -0.000000000000000000, -1.000000000000000000 ) ) ;
#46899=CARTESIAN_POINT ( 'NONE',  ( 24.17631672541061150, 8.757354005739776071, -8.209550701608334222 ) ) ;
#46901=CIRCLE ( 'NONE', #36248, 4.999999999999999112 ) ;
#46902=EDGE_CURVE ( 'NONE', #13538, #23831, #39082, .T. ) ;
#46903=AXIS2_PLACEMENT_3D ( 'NONE', #62801, #42178, #52838 ) ;
#46905=FACE_OUTER_BOUND ( 'NONE', #53908, .T. ) ;
#46908=CARTESIAN_POINT ( 'NONE',  ( -19.89498410467781753, -11.69391641137695181, -2.712006120889818739 ) ) ;
#46911=AXIS2_PLACEMENT_3D ( 'NONE', #47114, #32116, #52434 ) ;
#46912=EDGE_CURVE ( 'NONE', #26984, #42603, #40117, .T. ) ;
#46913=ORIENTED_EDGE ( 'NONE', *, *, #29698, .T. ) ;
#46914=AXIS2_PLACEMENT_3D ( 'NONE', #35167, #39848, #5265 ) ;
#46919=DIRECTION ( 'NONE',  ( 1.000000000000000000, -0.000000000000000000, 0.000000000000000000 ) ) ;
#46920=CARTESIAN_POINT ( 'NONE',  ( -35.00000000000000000, 7.376655759825023750, -9.700295462048581285 ) ) ;
#46921=ORIENTED_EDGE ( 'NONE', *, *, #52569, .T. ) ;
#46924=ORIENTED_EDGE ( 'NONE', *, *, #59174, .F. ) ;
#46925=ORIENTED_EDGE ( 'NONE', *, *, #27999, .F. ) ;
#46928=EDGE_LOOP ( 'NONE', ( #3135, #54311, #1966, #25014 ) ) ;
#46929=CARTESIAN_POINT ( 'NONE',  ( 36.00000000000000711, -11.39945968423467448, 5.710938531231827042 ) ) ;
#46930=AXIS2_PLACEMENT_3D ( 'NONE', #5682, #40909, #24717 ) ;
#46931=CARTESIAN_POINT ( 'NONE',  ( 37.00000000000000711, 10.75351884295727345, -4.725891942574794058 ) ) ;
#46932=ORIENTED_EDGE ( 'NONE', *, *, #54912, .F. ) ;
#46933=DIRECTION ( 'NONE',  ( -0.000000000000000000, -0.000000000000000000, -1.000000000000000000 ) ) ;
#46935=CARTESIAN_POINT ( 'NONE',  ( 23.19453373513495720, -4.581577854755520818, 11.09405916972947814 ) ) ;
#46936=ORIENTED_EDGE ( 'NONE', *, *, #52715, .T. ) ;
#46937=CARTESIAN_POINT ( 'NONE',  ( -37.00000000000000711, 9.896810808925497582, -7.110831038798171910 ) ) ;
#46938=ORIENTED_EDGE ( 'NONE', *, *, #17641, .T. ) ;
#46939=DIRECTION ( 'NONE',  ( 0.000000000000000000, 0.01356324068817998940, -0.9999080150203989437 ) ) ;
#46944=DIRECTION ( 'NONE',  ( -1.000000000000000000, -0.000000000000000000, 0.000000000000000000 ) ) ;
#46945=AXIS2_PLACEMENT_3D ( 'NONE', #51438, #35758, #46111 ) ;
#46946=AXIS2_PLACEMENT_3D ( 'NONE', #51472, #35136, #41117 ) ;
#46948=CIRCLE ( 'NONE', #54359, 5.000000000000000000 ) ;
#46949=LINE ( 'NONE', #57592, #15956 ) ;
#46952=ORIENTED_EDGE ( 'NONE', *, *, #53392, .T. ) ;
#46954=CARTESIAN_POINT ( 'NONE',  ( -7.489022030332961322, 25.00000000000000000, -10.84914964302385521 ) ) ;
#46955=VERTEX_POINT ( 'NONE', #16380 ) ;
#46956=DIRECTION ( 'NONE',  ( 0.000000000000000000, -0.01356324068817999114, 0.9999080150203989437 ) ) ;
#46958=ADVANCED_FACE ( 'NONE', ( #46314 ), #31003, .T. ) ;
#46960=CARTESIAN_POINT ( 'NONE',  ( 37.00000000000000711, 7.094637218249506994, 10.59380114696461916 ) ) ;
#46962=CARTESIAN_POINT ( 'NONE',  ( -35.00000000000000000, 0.000000000000000000, 0.000000000000000000 ) ) ;
#46963=DIRECTION ( 'NONE',  ( 1.000000000000000000, 0.000000000000000000, 0.000000000000000000 ) ) ;
#46964=VECTOR ( 'NONE', #35646, 1000.000000000000000 ) ;
#46966=AXIS2_PLACEMENT_3D ( 'NONE', #65372, #15160, #59413 ) ;
#46969=CARTESIAN_POINT ( 'NONE',  ( -35.00000000000000000, 0.000000000000000000, 0.000000000000000000 ) ) ;
#46971=DIRECTION ( 'NONE',  ( -1.000000000000000000, 0.000000000000000000, 0.000000000000000000 ) ) ;
#46976=ORIENTED_EDGE ( 'NONE', *, *, #41849, .T. ) ;
#46980=AXIS2_PLACEMENT_3D ( 'NONE', #37208, #47536, #1982 ) ;
#46981=EDGE_CURVE ( 'NONE', #25112, #9350, #27404, .T. ) ;
#46983=DIRECTION ( 'NONE',  ( 1.000000000000000000, 0.000000000000000000, 0.000000000000000000 ) ) ;
#46986=CARTESIAN_POINT ( 'NONE',  ( -9.351388602708162523, 25.00000000000000000, -3.665735721005252135 ) ) ;
#46987=LINE ( 'NONE', #26696, #9908 ) ;
#46988=EDGE_CURVE ( 'NONE', #3801, #40116, #12536, .T. ) ;
#46990=AXIS2_PLACEMENT_3D ( 'NONE', #13768, #64633, #49063 ) ;
#46991=CIRCLE ( 'NONE', #44845, 5.000000000000000888 ) ;
#46992=B_SPLINE_CURVE_WITH_KNOTS ( 'NONE', 3,
 ( #57263, #11688, #62890, #11369, #31641, #52922, #57603, #27005, #51953, #27638, #38945, #53259, #44249, #4027, #7705, #38616, #29293, #59233, #12666, #54585, #54247, #13655, #37949, #13341 ),
 .UNSPECIFIED., .F., .F.,
 ( 4, 2, 2, 2, 2, 2, 2, 2, 2, 2, 2, 4 ),
 ( 0.003159056194143415250, 0.004024695253672650602, 0.004890334313201885087, 0.005755973372731119572, 0.006621612432260354925, 0.007054431962024973468, 0.007487251491789592879, 0.007920071021554212290, 0.008352890551318830833, 0.008785710081083440703, 0.009218529610848048839, 0.01008416867037726684 ),
 .UNSPECIFIED. ) ;
#46994=CARTESIAN_POINT ( 'NONE',  ( -16.58214495380866893, 7.650095523388448449, 11.12376028359556557 ) ) ;
#46995=CARTESIAN_POINT ( 'NONE',  ( -37.00000000000000711, 0.000000000000000000, 0.000000000000000000 ) ) ;
#46996=( BOUNDED_CURVE ( )  B_SPLINE_CURVE ( 3, ( #39493, #45148, #64431, #59457 ),
 .UNSPECIFIED., .F., .F. ) 
 B_SPLINE_CURVE_WITH_KNOTS ( ( 4, 4 ),
 ( 5.598218072871999240, 5.645776840021275333 ),
 .UNSPECIFIED. ) 
 CURVE ( )  GEOMETRIC_REPRESENTATION_ITEM ( )  RATIONAL_B_SPLINE_CURVE ( ( 1.000000000000000000, 0.9998115225205463918, 0.9998115225205463918, 1.000000000000000000 ) ) 
 REPRESENTATION_ITEM ( '' )  );
#46998=CARTESIAN_POINT ( 'NONE',  ( -35.00000000000000000, 11.78745411414839594, 3.093009498343968211 ) ) ;
#47001=ORIENTED_EDGE ( 'NONE', *, *, #54726, .T. ) ;
#47002=CYLINDRICAL_SURFACE ( 'NONE', #32006, 4.999999999999999112 ) ;
#47003=ORIENTED_EDGE ( 'NONE', *, *, #55933, .F. ) ;
#47005=ADVANCED_FACE ( 'NONE', ( #51315 ), #754, .T. ) ;
#47009=EDGE_CURVE ( 'NONE', #65324, #40853, #45489, .T. ) ;
#47010=AXIS2_PLACEMENT_3D ( 'NONE', #30542, #29554, #19613 ) ;
#47013=CARTESIAN_POINT ( 'NONE',  ( -25.11474465335534489, -9.573234766864146650, 7.237578467736122789 ) ) ;
#47015=FACE_OUTER_BOUND ( 'NONE', #8752, .T. ) ;
#47016=DIRECTION ( 'NONE',  ( 0.000000000000000000, -0.8827602140260264463, 0.4698238015817460256 ) ) ;
#47018=AXIS2_PLACEMENT_3D ( 'NONE', #9613, #29265, #40541 ) ;
#47019=CYLINDRICAL_SURFACE ( 'NONE', #9837, 17.75474371510546234 ) ;
#47020=AXIS2_PLACEMENT_3D ( 'NONE', #51466, #21514, #46773 ) ;
#47023=CARTESIAN_POINT ( 'NONE',  ( -27.19357181888462094, 10.84410562793473431, 5.138615876886901468 ) ) ;
#47024=ORIENTED_EDGE ( 'NONE', *, *, #55196, .F. ) ;
#47025=DIRECTION ( 'NONE',  ( -0.000000000000000000, -1.000000000000000000, -0.000000000000000000 ) ) ;
#47026=ORIENTED_EDGE ( 'NONE', *, *, #7061, .F. ) ;
#47027=DIRECTION ( 'NONE',  ( -1.000000000000000000, 0.000000000000000000, 0.000000000000000000 ) ) ;
#47028=EDGE_LOOP ( 'NONE', ( #2228, #65107, #33663, #22641 ) ) ;
#47029=CARTESIAN_POINT ( 'NONE',  ( -35.00000000000000000, 0.000000000000000000, 0.000000000000000000 ) ) ;
#47031=EDGE_CURVE ( 'NONE', #17645, #42662, #21096, .T. ) ;
#47033=ORIENTED_EDGE ( 'NONE', *, *, #20214, .F. ) ;
#47034=CARTESIAN_POINT ( 'NONE',  ( -37.00000000000000711, -6.265926637539413591, -11.10408318471066380 ) ) ;
#47035=CARTESIAN_POINT ( 'NONE',  ( -35.00000000000000000, 5.710938531231712467, 11.39945968423473310 ) ) ;
#47039=CIRCLE ( 'NONE', #1370, 12.75000000000000178 ) ;
#47040=EDGE_LOOP ( 'NONE', ( #29329, #60841, #26222, #1378 ) ) ;
#47042=ORIENTED_EDGE ( 'NONE', *, *, #38198, .T. ) ;
#47043=AXIS2_PLACEMENT_3D ( 'NONE', #26883, #57816, #37511 ) ;
#47045=DIRECTION ( 'NONE',  ( -1.000000000000000000, 0.000000000000000000, 0.000000000000000000 ) ) ;
#47046=AXIS2_PLACEMENT_3D ( 'NONE', #17248, #37522, #27878 ) ;
#47050=DIRECTION ( 'NONE',  ( 0.000000000000000000, 0.01356324068817998940, -0.9999080150203990547 ) ) ;
#47051=AXIS2_PLACEMENT_3D ( 'NONE', #31741, #32071, #46401 ) ;
#47052=DIRECTION ( 'NONE',  ( 1.000000000000000000, 0.000000000000000000, 0.000000000000000000 ) ) ;
#47055=CARTESIAN_POINT ( 'NONE',  ( -37.00000000000000711, -10.70999494708496869, 5.814360711498252954 ) ) ;
#47057=AXIS2_PLACEMENT_3D ( 'NONE', #41551, #46243, #55882 ) ;
#47058=FACE_OUTER_BOUND ( 'NONE', #8782, .T. ) ;
#47059=CARTESIAN_POINT ( 'NONE',  ( -3.818603701402922823, -10.58165328604947319, 5.676754050214040781 ) ) ;
#47060=CIRCLE ( 'NONE', #38551, 12.74999999999999822 ) ;
#47063=CYLINDRICAL_SURFACE ( 'NONE', #22614, 12.18650000000000055 ) ;
#47064=EDGE_CURVE ( 'NONE', #62523, #28210, #54816, .T. ) ;
#47066=VECTOR ( 'NONE', #56945, 1000.000000000000000 ) ;
#47067=LINE ( 'NONE', #42049, #48017 ) ;
#47073=ADVANCED_FACE ( 'NONE', ( #33550 ), #24541, .T. ) ;
#47075=DIRECTION ( 'NONE',  ( -1.000000000000000000, -0.000000000000000000, 0.000000000000000000 ) ) ;
#47076=CARTESIAN_POINT ( 'NONE',  ( -27.10970334550012595, -12.25602637579915033, 5.660463253225340274 ) ) ;
#47077=ORIENTED_EDGE ( 'NONE', *, *, #54950, .T. ) ;
#47078=CARTESIAN_POINT ( 'NONE',  ( -37.00000000000000711, -4.725891942574680371, -10.75351884295732496 ) ) ;
#47079=DIRECTION ( 'NONE',  ( 0.000000000000000000, 0.01356324068817998940, -0.9999080150203989437 ) ) ;
#47082=DIRECTION ( 'NONE',  ( -1.000000000000000000, 0.000000000000000000, 0.000000000000000000 ) ) ;
#47084=CARTESIAN_POINT ( 'NONE',  ( -35.00000000000000000, 11.16627499335650242, 3.645068577060221582 ) ) ;
#47085=EDGE_CURVE ( 'NONE', #54640, #35397, #34890, .T. ) ;
#47086=AXIS2_PLACEMENT_3D ( 'NONE', #46197, #5294, #41843 ) ;
#47087=CIRCLE ( 'NONE', #30074, 5.000000000000000000 ) ;
#47090=DIRECTION ( 'NONE',  ( -1.000000000000000000, 0.000000000000000000, 0.000000000000000000 ) ) ;
#47091=ADVANCED_FACE ( 'NONE', ( #33859 ), #23240, .T. ) ;
#47093=CIRCLE ( 'NONE', #43900, 4.999999999999999112 ) ;
#47094=FACE_OUTER_BOUND ( 'NONE', #52951, .T. ) ;
#47095=VERTEX_POINT ( 'NONE', #18268 ) ;
#47096=CARTESIAN_POINT ( 'NONE',  ( -35.00000000000000000, -8.029056188533626681, -8.573591947375405198 ) ) ;
#47099=FACE_OUTER_BOUND ( 'NONE', #61716, .T. ) ;
#47100=DIRECTION ( 'NONE',  ( -0.5446691071471760903, 0.8386510381079236298, 0.000000000000000000 ) ) ;
#47101=VECTOR ( 'NONE', #2060, 1000.000000000000000 ) ;
#47104=ORIENTED_EDGE ( 'NONE', *, *, #23767, .T. ) ;
#47106=CARTESIAN_POINT ( 'NONE',  ( -29.43980975494970309, -3.641506875706030488, 12.99959336572439561 ) ) ;
#47107=AXIS2_PLACEMENT_3D ( 'NONE', #4289, #24562, #44842 ) ;
#47111=EDGE_CURVE ( 'NONE', #59819, #29583, #56121, .T. ) ;
#47112=CIRCLE ( 'NONE', #54570, 12.18649999999999878 ) ;
#47114=CARTESIAN_POINT ( 'NONE',  ( 37.00000000000000711, 4.705694406421931860E-17, -3.469127814946512892E-15 ) ) ;
#47115=ORIENTED_EDGE ( 'NONE', *, *, #31424, .F. ) ;
#47118=DIRECTION ( 'NONE',  ( -1.000000000000000000, -1.836970198721029688E-16, -0.000000000000000000 ) ) ;
#47125=CARTESIAN_POINT ( 'NONE',  ( 37.00000000000000711, 5.921969905510355403, -10.14408668126215929 ) ) ;
#47126=CARTESIAN_POINT ( 'NONE',  ( -36.00000000000000711, -1.113475361586399925, -12.70128625845194215 ) ) ;
#47128=EDGE_CURVE ( 'NONE', #10479, #37783, #6260, .T. ) ;
#47129=DIRECTION ( 'NONE',  ( 1.000000000000000000, 0.000000000000000000, 0.000000000000000000 ) ) ;
#47131=CIRCLE ( 'NONE', #23773, 12.74999999999999822 ) ;
#47132=LINE ( 'NONE', #56434, #46075 ) ;
#47133=ORIENTED_EDGE ( 'NONE', *, *, #38267, .F. ) ;
#47134=CARTESIAN_POINT ( 'NONE',  ( -35.00000000000000000, -11.44858830469742017, 2.627174906296871448 ) ) ;
#47136=LINE ( 'NONE', #57773, #26846 ) ;
#47137=DIRECTION ( 'NONE',  ( 0.000000000000000000, 0.01356324068817998940, -0.9999080150203990547 ) ) ;
#47138=AXIS2_PLACEMENT_3D ( 'NONE', #17775, #7129, #37387 ) ;
#47139=CARTESIAN_POINT ( 'NONE',  ( -7.594175326315255603, 6.461734609435446863, -10.13293342493276761 ) ) ;
#47142=VECTOR ( 'NONE', #5078, 1000.000000000000000 ) ;
#47143=DIRECTION ( 'NONE',  ( 0.000000000000000000, -0.01356324068818000328, 0.9999080150203990547 ) ) ;
#47144=VERTEX_POINT ( 'NONE', #49511 ) ;
#47145=VECTOR ( 'NONE', #45929, 1000.000000000000000 ) ;
#47146=ORIENTED_EDGE ( 'NONE', *, *, #62381, .F. ) ;
#47147=DIRECTION ( 'NONE',  ( 1.000000000000000000, 0.000000000000000000, 0.000000000000000000 ) ) ;
#47148=EDGE_CURVE ( 'NONE', #31240, #46242, #14717, .T. ) ;
#47149=ORIENTED_EDGE ( 'NONE', *, *, #51730, .F. ) ;
#47150=DIRECTION ( 'NONE',  ( 0.000000000000000000, -0.9246979985058764173, -0.3807014730195119045 ) ) ;
#47151=DIRECTION ( 'NONE',  ( -1.000000000000000000, 0.000000000000000000, 0.000000000000000000 ) ) ;
#47152=CIRCLE ( 'NONE', #20560, 5.000000000000000000 ) ;
#47155=DIRECTION ( 'NONE',  ( 0.000000000000000000, 0.01356324068817998940, -0.9999080150203989437 ) ) ;
#47156=ORIENTED_EDGE ( 'NONE', *, *, #3009, .F. ) ;
#47159=FACE_OUTER_BOUND ( 'NONE', #48867, .T. ) ;
#47162=VECTOR ( 'NONE', #19375, 1000.000000000000000 ) ;
#47165=CARTESIAN_POINT ( 'NONE',  ( 35.00000000000000000, 4.705694406421931860E-17, -3.469127814946512892E-15 ) ) ;
#47167=VERTEX_POINT ( 'NONE', #39504 ) ;
#47169=DIRECTION ( 'NONE',  ( 0.000000000000000000, 0.6269146997507986097, 0.7790879021242506086 ) ) ;
#47171=CARTESIAN_POINT ( 'NONE',  ( 10.48620311856346454, 8.250315036047107142, -10.68561190601526789 ) ) ;
#47174=ADVANCED_FACE ( 'NONE', ( #59797 ), #14230, .T. ) ;
#47176=DIRECTION ( 'NONE',  ( 0.000000000000000000, 0.01356324068817998940, -0.9999080150203990547 ) ) ;
#47177=EDGE_LOOP ( 'NONE', ( #31076, #14386, #10591, #15518 ) ) ;
#47180=EDGE_CURVE ( 'NONE', #38246, #433, #25320, .T. ) ;
#47181=ORIENTED_EDGE ( 'NONE', *, *, #44443, .F. ) ;
#47182=DIRECTION ( 'NONE',  ( -1.000000000000000000, -0.000000000000000000, 0.000000000000000000 ) ) ;
#47184=CYLINDRICAL_SURFACE ( 'NONE', #2282, 4.999999999999999112 ) ;
#47189=ORIENTED_EDGE ( 'NONE', *, *, #48260, .F. ) ;
#47190=AXIS2_PLACEMENT_3D ( 'NONE', #47096, #52072, #57064 ) ;
#47192=VECTOR ( 'NONE', #6922, 1000.000000000000000 ) ;
#47194=EDGE_LOOP ( 'NONE', ( #35839, #33851, #29343, #30324 ) ) ;
#47195=DIRECTION ( 'NONE',  ( 0.000000000000000000, -0.01356324068817991481, 0.9999080150203990547 ) ) ;
#47196=CARTESIAN_POINT ( 'NONE',  ( -9.197504613504071003, 11.40546504581822695, -3.730959538268481257 ) ) ;
#47199=ORIENTED_EDGE ( 'NONE', *, *, #26044, .T. ) ;
#47200=DIRECTION ( 'NONE',  ( -1.000000000000000000, -0.000000000000000000, 0.000000000000000000 ) ) ;
#47202=DIRECTION ( 'NONE',  ( 0.000000000000000000, 0.9999080150203989437, 0.01356324068817649567 ) ) ;
#47205=CARTESIAN_POINT ( 'NONE',  ( -37.00000000000000711, 5.814360711498292034, 10.70999494708494737 ) ) ;
#47206=VERTEX_POINT ( 'NONE', #40479 ) ;
#47207=ORIENTED_EDGE ( 'NONE', *, *, #60729, .T. ) ;
#47210=ORIENTED_EDGE ( 'NONE', *, *, #65425, .T. ) ;
#47212=CIRCLE ( 'NONE', #63136, 12.75000000000000178 ) ;
#47215=DIRECTION ( 'NONE',  ( -0.000000000000000000, -0.000000000000000000, -1.000000000000000000 ) ) ;
#47218=VERTEX_POINT ( 'NONE', #30818 ) ;
#47220=EDGE_LOOP ( 'NONE', ( #63803, #9857, #13155, #38952 ) ) ;
#47221=( BOUNDED_CURVE ( )  B_SPLINE_CURVE ( 3, ( #52666, #37011, #11737, #32024 ),
 .UNSPECIFIED., .F., .F. ) 
 B_SPLINE_CURVE_WITH_KNOTS ( ( 4, 4 ),
 ( 4.594111722311771118, 4.635963600959730258 ),
 .UNSPECIFIED. ) 
 CURVE ( )  GEOMETRIC_REPRESENTATION_ITEM ( )  RATIONAL_B_SPLINE_CURVE ( ( 1.000000000000000000, 0.9998540403475023597, 0.9998540403475023597, 1.000000000000000000 ) ) 
 REPRESENTATION_ITEM ( '' )  );
#47223=AXIS2_PLACEMENT_3D ( 'NONE', #21667, #61539, #15982 ) ;
#47224=CARTESIAN_POINT ( 'NONE',  ( 47.00000000000000711, 4.705694406421931860E-17, -3.469127814946512892E-15 ) ) ;
#47226=LINE ( 'NONE', #11304, #3154 ) ;
#47229=CIRCLE ( 'NONE', #55716, 5.000000000000000888 ) ;
#47232=CARTESIAN_POINT ( 'NONE',  ( -37.00000000000000711, 0.000000000000000000, 0.000000000000000000 ) ) ;
#47233=ORIENTED_EDGE ( 'NONE', *, *, #14028, .T. ) ;
#47234=EDGE_CURVE ( 'NONE', #64575, #6120, #24075, .T. ) ;
#47235=FACE_OUTER_BOUND ( 'NONE', #18592, .T. ) ;
#47239=EDGE_CURVE ( 'NONE', #17397, #28779, #50824, .T. ) ;
#47242=CIRCLE ( 'NONE', #33402, 5.000000000000000000 ) ;
#47244=DIRECTION ( 'NONE',  ( -0.000000000000000000, -1.000000000000000000, -0.000000000000000000 ) ) ;
#47245=CARTESIAN_POINT ( 'NONE',  ( 23.59428955459845412, 9.152238998900841693, -7.766884395375215355 ) ) ;
#47246=DIRECTION ( 'NONE',  ( 0.000000000000000000, 0.2355298848897517117, 0.9718671068226459875 ) ) ;
#47247=EDGE_CURVE ( 'NONE', #16971, #13636, #54005, .T. ) ;
#47250=ORIENTED_EDGE ( 'NONE', *, *, #63538, .T. ) ;
#47251=EDGE_CURVE ( 'NONE', #51616, #55813, #9900, .T. ) ;
#47255=ADVANCED_FACE ( 'NONE', ( #30186 ), #5930, .T. ) ;
#47256=AXIS2_PLACEMENT_3D ( 'NONE', #7240, #27869, #48178 ) ;
#47258=EDGE_CURVE ( 'NONE', #13243, #36795, #65733, .T. ) ;
#47260=DIRECTION ( 'NONE',  ( -1.000000000000000000, -0.000000000000000000, 0.000000000000000000 ) ) ;
#47262=DIRECTION ( 'NONE',  ( -0.000000000000000000, -0.000000000000000000, -1.000000000000000000 ) ) ;
#47265=VERTEX_POINT ( 'NONE', #600 ) ;
#47267=ORIENTED_EDGE ( 'NONE', *, *, #57411, .F. ) ;
#47268=VERTEX_POINT ( 'NONE', #20861 ) ;
#47269=DIRECTION ( 'NONE',  ( 1.000000000000000000, 0.000000000000000000, 0.000000000000000000 ) ) ;
#47270=CIRCLE ( 'NONE', #51557, 5.000000000000001776 ) ;
#47271=CARTESIAN_POINT ( 'NONE',  ( 10.48620311856346454, 8.250315036047107142, 8.713914264323181058 ) ) ;
#47272=ORIENTED_EDGE ( 'NONE', *, *, #5950, .T. ) ;
#47274=DIRECTION ( 'NONE',  ( 0.000000000000000000, -0.01356324068817991828, 0.9999080150203990547 ) ) ;
#47275=VERTEX_POINT ( 'NONE', #41129 ) ;
#47278=CARTESIAN_POINT ( 'NONE',  ( -35.00000000000000000, 12.60630747491665815, -1.908798535168240607 ) ) ;
#47279=VERTEX_POINT ( 'NONE', #61411 ) ;
#47281=ORIENTED_EDGE ( 'NONE', *, *, #20910, .T. ) ;
#47282=AXIS2_PLACEMENT_3D ( 'NONE', #22371, #12387, #42637 ) ;
#47283=CARTESIAN_POINT ( 'NONE',  ( 12.47628546223243617, 0.000000000000000000, -13.50000000000000178 ) ) ;
#47284=CARTESIAN_POINT ( 'NONE',  ( -17.85006501957281699, -6.222042789639135485, 11.98374378373027582 ) ) ;
#47286=DIRECTION ( 'NONE',  ( 0.000000000000000000, -0.2618041379715496664, 0.9651210252299831094 ) ) ;
#47287=EDGE_CURVE ( 'NONE', #8090, #49536, #15850, .T. ) ;
#47289=DIRECTION ( 'NONE',  ( 0.000000000000000000, 0.5243256840888563808, 0.8515178078024867592 ) ) ;
#47293=ORIENTED_EDGE ( 'NONE', *, *, #25341, .F. ) ;
#47294=CARTESIAN_POINT ( 'NONE',  ( 35.00000000000000000, -12.18632975068352664, -0.06441628369832411161 ) ) ;
#47295=AXIS2_PLACEMENT_3D ( 'NONE', #44925, #34917, #55226 ) ;
#47296=EDGE_LOOP ( 'NONE', ( #39130, #27674, #16486, #19557 ) ) ;
#47298=DIRECTION ( 'NONE',  ( 0.000000000000000000, 0.01356324068817998940, -0.9999080150203990547 ) ) ;
#47299=VERTEX_POINT ( 'NONE', #42107 ) ;
#47300=EDGE_CURVE ( 'NONE', #42662, #56972, #28496, .T. ) ;
#47304=ORIENTED_EDGE ( 'NONE', *, *, #48984, .F. ) ;
#47306=ORIENTED_EDGE ( 'NONE', *, *, #46172, .F. ) ;
#47307=CARTESIAN_POINT ( 'NONE',  ( -17.16021277067101281, -7.891355405082562058, -9.047158298165973278 ) ) ;
#47311=CARTESIAN_POINT ( 'NONE',  ( -2.532614230583023041, -12.88560382747352584, 4.026315189028235153 ) ) ;
#47313=EDGE_CURVE ( 'NONE', #30591, #34726, #62481, .T. ) ;
#47314=CARTESIAN_POINT ( 'NONE',  ( -17.65431273644522392, -7.797115439854604979, 9.126847883897077907 ) ) ;
#47315=VERTEX_POINT ( 'NONE', #11220 ) ;
#47316=CYLINDRICAL_SURFACE ( 'NONE', #41209, 12.18650000000000055 ) ;
#47318=CYLINDRICAL_SURFACE ( 'NONE', #34101, 3.309571291727934295 ) ;
#47322=EDGE_CURVE ( 'NONE', #32142, #48941, #1251, .T. ) ;
#47323=LINE ( 'NONE', #52947, #11809 ) ;
#47327=ORIENTED_EDGE ( 'NONE', *, *, #60423, .F. ) ;
#47328=EDGE_CURVE ( 'NONE', #13395, #34161, #57197, .T. ) ;
#47329=CARTESIAN_POINT ( 'NONE',  ( 35.00000000000000000, 11.95840593935204765, 2.346765782874299155 ) ) ;
#47331=AXIS2_PLACEMENT_3D ( 'NONE', #50821, #46170, #26205 ) ;
#47332=ORIENTED_EDGE ( 'NONE', *, *, #7064, .F. ) ;
#47336=EDGE_CURVE ( 'NONE', #53158, #42300, #32463, .T. ) ;
#47337=DIRECTION ( 'NONE',  ( 1.000000000000000000, -0.000000000000000000, 0.000000000000000000 ) ) ;
#47338=ORIENTED_EDGE ( 'NONE', *, *, #63275, .F. ) ;
#47340=ORIENTED_EDGE ( 'NONE', *, *, #5519, .T. ) ;
#47341=ORIENTED_EDGE ( 'NONE', *, *, #30587, .F. ) ;
#47342=VECTOR ( 'NONE', #64498, 1000.000000000000000 ) ;
#47345=CARTESIAN_POINT ( 'NONE',  ( 37.00000000000000711, -11.73463472867578261, -3.287724142101374536 ) ) ;
#47347=DIRECTION ( 'NONE',  ( 1.000000000000000000, 0.000000000000000000, 0.000000000000000000 ) ) ;
#47348=CARTESIAN_POINT ( 'NONE',  ( 35.00000000000000000, -2.497432891016756251, 11.47758908105696740 ) ) ;
#47352=CARTESIAN_POINT ( 'NONE',  ( 37.00000000000000711, 10.14433819232443490, 6.753013023069604159 ) ) ;
#47353=LINE ( 'NONE', #18066, #55254 ) ;
#47354=ORIENTED_EDGE ( 'NONE', *, *, #7007, .T. ) ;
#47355=CARTESIAN_POINT ( 'NONE',  ( -28.21004269438542522, 10.37327567629658631, -6.041082299521756127 ) ) ;
#47356=ORIENTED_EDGE ( 'NONE', *, *, #54678, .T. ) ;
#47358=ORIENTED_EDGE ( 'NONE', *, *, #8392, .T. ) ;
#47359=CARTESIAN_POINT ( 'NONE',  ( 37.00000000000000711, -12.60630747491661374, 1.908798535168511057 ) ) ;
#47360=CYLINDRICAL_SURFACE ( 'NONE', #62899, 4.999999999999999112 ) ;
#47362=CIRCLE ( 'NONE', #36578, 4.999999999999999112 ) ;
#47364=EDGE_CURVE ( 'NONE', #20627, #50714, #1170, .T. ) ;
#47365=CARTESIAN_POINT ( 'NONE',  ( -37.00000000000000711, 6.280308599560139093, 9.926225166347048656 ) ) ;
#47368=ORIENTED_EDGE ( 'NONE', *, *, #26702, .T. ) ;
#47369=ADVANCED_FACE ( 'NONE', ( #53090 ), #7529, .T. ) ;
#47374=EDGE_CURVE ( 'NONE', #19607, #14001, #27451, .T. ) ;
#47375=DIRECTION ( 'NONE',  ( 0.000000000000000000, 0.01356324068817998940, -0.9999080150203990547 ) ) ;
#47376=DIRECTION ( 'NONE',  ( 1.000000000000000000, -0.000000000000000000, 0.000000000000000000 ) ) ;
#47378=DIRECTION ( 'NONE',  ( -1.000000000000000000, 0.000000000000000000, 0.000000000000000000 ) ) ;
#47381=AXIS2_PLACEMENT_3D ( 'NONE', #53668, #28375, #39321 ) ;
#47382=CARTESIAN_POINT ( 'NONE',  ( 36.00000000000000711, -8.954052073409666690, -9.076753354953966735 ) ) ;
#47383=VECTOR ( 'NONE', #14089, 1000.000000000000000 ) ;
#47385=CARTESIAN_POINT ( 'NONE',  ( 22.57855258442565116, 3.026812727784649493, -13.15630665159948975 ) ) ;
#47387=DIRECTION ( 'NONE',  ( -0.000000000000000000, -1.000000000000000000, -0.000000000000000000 ) ) ;
#47388=EDGE_CURVE ( 'NONE', #30904, #25281, #64610, .T. ) ;
#47390=EDGE_CURVE ( 'NONE', #57717, #61894, #28465, .T. ) ;
#47393=DIRECTION ( 'NONE',  ( 0.000000000000000000, -0.8515178078024923103, 0.5243256840888473880 ) ) ;
#47397=DIRECTION ( 'NONE',  ( 1.000000000000000000, 0.000000000000000000, 0.000000000000000000 ) ) ;
#47399=CARTESIAN_POINT ( 'NONE',  ( -28.41827485489077532, 3.509237424706437292, 25.00000000000000000 ) ) ;
#47401=DIRECTION ( 'NONE',  ( 1.000000000000000000, -0.000000000000000000, 0.000000000000000000 ) ) ;
#47403=EDGE_CURVE ( 'NONE', #29168, #27894, #7285, .T. ) ;
#47405=CARTESIAN_POINT ( 'NONE',  ( -24.79507913871908542, 8.359778566926882704, 8.617069398609862318 ) ) ;
#47406=CARTESIAN_POINT ( 'NONE',  ( -24.92180037670109627, -9.674391025304601044, 9.421401640134503097 ) ) ;
#47408=DIRECTION ( 'NONE',  ( 0.000000000000000000, 0.01356324068817991828, -0.9999080150203990547 ) ) ;
#47412=VERTEX_POINT ( 'NONE', #3220 ) ;
#47415=CARTESIAN_POINT ( 'NONE',  ( 37.00000000000000711, 4.705694406421931860E-17, -3.469127814946512892E-15 ) ) ;
#47416=DIRECTION ( 'NONE',  ( 0.000000000000000000, 0.6478160128811947249, -0.7617968321374878338 ) ) ;
#47418=CARTESIAN_POINT ( 'NONE',  ( -37.00000000000000711, 0.4871980014163251882, -12.74068829017553561 ) ) ;
#47420=AXIS2_PLACEMENT_3D ( 'NONE', #41021, #11107, #487 ) ;
#47423=DIRECTION ( 'NONE',  ( 1.000000000000000000, 0.000000000000000000, 0.000000000000000000 ) ) ;
#47424=DIRECTION ( 'NONE',  ( 1.000000000000000000, 0.000000000000000000, 0.000000000000000000 ) ) ;
#47425=CARTESIAN_POINT ( 'NONE',  ( 24.39609475304860453, -1.096898803462643457, -11.95519569193159803 ) ) ;
#47427=CARTESIAN_POINT ( 'NONE',  ( -3.090922707259200930, -7.896884802510032664, 10.95603262241157161 ) ) ;
#47432=CARTESIAN_POINT ( 'NONE',  ( -18.08686583997241115, 5.151216734910855521, 10.83812558286605920 ) ) ;
#47434=DIRECTION ( 'NONE',  ( 0.000000000000000000, -0.8369827122275287357, -0.5472293298355359603 ) ) ;
#47439=CARTESIAN_POINT ( 'NONE',  ( 36.00000000000000711, 12.63095688309029008, -1.738225594540043772 ) ) ;
#47441=EDGE_CURVE ( 'NONE', #44318, #57839, #935, .T. ) ;
#47442=CARTESIAN_POINT ( 'NONE',  ( -25.19729880547092549, -5.013571510455943958, 10.93379378137424496 ) ) ;
#47444=ORIENTED_EDGE ( 'NONE', *, *, #54179, .T. ) ;
#47445=ORIENTED_EDGE ( 'NONE', *, *, #48623, .T. ) ;
#47447=EDGE_LOOP ( 'NONE', ( #4683, #46885, #17336, #41223 ) ) ;
#47448=DIRECTION ( 'NONE',  ( 1.000000000000000000, 0.000000000000000000, 0.000000000000000000 ) ) ;
#47450=CARTESIAN_POINT ( 'NONE',  ( 37.00000000000000711, 8.295159312811978936, 8.927548052240801724 ) ) ;
#47451=CARTESIAN_POINT ( 'NONE',  ( -35.00000000000000000, -5.391785509270885512, -10.43555801961481677 ) ) ;
#47452=CARTESIAN_POINT ( 'NONE',  ( -37.00000000000000711, 0.000000000000000000, 0.000000000000000000 ) ) ;
#47455=CARTESIAN_POINT ( 'NONE',  ( -35.00000000000000000, -10.49591321039677005, -5.273331777780449592 ) ) ;
#47456=ORIENTED_EDGE ( 'NONE', *, *, #62470, .T. ) ;
#47459=DIRECTION ( 'NONE',  ( -1.000000000000000000, 0.000000000000000000, 0.000000000000000000 ) ) ;
#47460=EDGE_CURVE ( 'NONE', #9681, #19811, #49110, .T. ) ;
#47464=CARTESIAN_POINT ( 'NONE',  ( -35.00000000000000000, -6.475373545682229448, -10.32377448871674908 ) ) ;
#47465=EDGE_CURVE ( 'NONE', #24124, #37122, #49772, .T. ) ;
#47466=ORIENTED_EDGE ( 'NONE', *, *, #37901, .T. ) ;
#47467=ORIENTED_EDGE ( 'NONE', *, *, #22429, .F. ) ;
#47468=CARTESIAN_POINT ( 'NONE',  ( -35.00000000000000000, 0.000000000000000000, 0.000000000000000000 ) ) ;
#47469=EDGE_LOOP ( 'NONE', ( #29018, #9801, #15224, #49565 ) ) ;
#47470=CARTESIAN_POINT ( 'NONE',  ( 35.00000000000000000, -11.74614673114903596, -0.01609748574441245694 ) ) ;
#47471=CARTESIAN_POINT ( 'NONE',  ( -28.71071236259718162, 3.670376459565066085, -11.42521152978763155 ) ) ;
#47472=CARTESIAN_POINT ( 'NONE',  ( 37.00000000000000711, -5.300372733891562049, 11.59605747147791810 ) ) ;
#47476=LINE ( 'NONE', #51811, #4565 ) ;
#47477=CARTESIAN_POINT ( 'NONE',  ( -29.68541646480311869, -1.416020129149132334, -13.42553116244736877 ) ) ;
#47478=CARTESIAN_POINT ( 'NONE',  ( 8.937200413558842982, 4.476360154859214902, 12.73625532737129795 ) ) ;
#47480=CARTESIAN_POINT ( 'NONE',  ( -35.00000000000000000, -9.217970097227665249, -7.971186206369574201 ) ) ;
#47481=CARTESIAN_POINT ( 'NONE',  ( 37.00000000000000711, 4.705694406421931860E-17, -3.469127814946512892E-15 ) ) ;
#47486=DIRECTION ( 'NONE',  ( 0.000000000000000000, -0.01356324068817991828, 0.9999080150203990547 ) ) ;
#47487=DIRECTION ( 'NONE',  ( 0.000000000000000000, -0.01356324068817998940, 0.9999080150203990547 ) ) ;
#47488=DIRECTION ( 'NONE',  ( 0.000000000000000000, -0.2006870767258747690, 0.9796553971857770993 ) ) ;
#47489=CARTESIAN_POINT ( 'NONE',  ( 3.459614771489464946, -11.09853614738469396, 7.685863346768216253 ) ) ;
#47490=ADVANCED_FACE ( 'NONE', ( #39419 ), #33130, .T. ) ;
#47491=ORIENTED_EDGE ( 'NONE', *, *, #36810, .F. ) ;
#47496=LINE ( 'NONE', #31530, #55557 ) ;
#47498=VECTOR ( 'NONE', #4783, 1000.000000000000000 ) ;
#47499=CYLINDRICAL_SURFACE ( 'NONE', #48197, 10.20557198542813815 ) ;
#47500=DIRECTION ( 'NONE',  ( 1.000000000000000000, 0.000000000000000000, 0.000000000000000000 ) ) ;
#47505=CARTESIAN_POINT ( 'NONE',  ( -20.79170840334646542, -11.34110549087206898, -3.921648409140116698 ) ) ;
#47507=AXIS2_PLACEMENT_3D ( 'NONE', #18253, #33538, #53828 ) ;
#47509=CARTESIAN_POINT ( 'NONE',  ( 22.19144544426022492, -12.08131399901154701, -6.034850276811086545 ) ) ;
#47510=DIRECTION ( 'NONE',  ( 0.000000000000000000, 0.01356324068817998940, -0.9999080150203990547 ) ) ;
#47511=AXIS2_PLACEMENT_3D ( 'NONE', #54051, #44070, #64339 ) ;
#47512=DIRECTION ( 'NONE',  ( 1.000000000000000000, 0.000000000000000000, -0.000000000000000000 ) ) ;
#47513=ORIENTED_EDGE ( 'NONE', *, *, #34677, .F. ) ;
#47514=CARTESIAN_POINT ( 'NONE',  ( -36.00000000000000711, 3.640372113593720371, -12.21925492305358496 ) ) ;
#47518=ORIENTED_EDGE ( 'NONE', *, *, #26117, .T. ) ;
#47520=DIRECTION ( 'NONE',  ( -1.000000000000000000, -0.000000000000000000, -0.000000000000000000 ) ) ;
#47522=ORIENTED_EDGE ( 'NONE', *, *, #21882, .F. ) ;
#47524=VERTEX_POINT ( 'NONE', #41060 ) ;
#47531=DIRECTION ( 'NONE',  ( -1.000000000000000000, -0.000000000000000000, -0.000000000000000000 ) ) ;
#47533=ORIENTED_EDGE ( 'NONE', *, *, #54448, .F. ) ;
#47534=CARTESIAN_POINT ( 'NONE',  ( -4.975205859172452172, -1.416020129149132778, 11.91616074890920451 ) ) ;
#47536=DIRECTION ( 'NONE',  ( 1.000000000000000000, 0.000000000000000000, 0.000000000000000000 ) ) ;
#47539=DIRECTION ( 'NONE',  ( 1.000000000000000000, 0.000000000000000000, -0.000000000000000000 ) ) ;
#47542=ORIENTED_EDGE ( 'NONE', *, *, #48536, .T. ) ;
#47543=DIRECTION ( 'NONE',  ( -1.000000000000000000, 0.000000000000000000, 0.000000000000000000 ) ) ;
#47546=CARTESIAN_POINT ( 'NONE',  ( -35.00000000000000000, -6.547236723514086698, 9.752226076388870624 ) ) ;
#47549=FACE_OUTER_BOUND ( 'NONE', #30992, .T. ) ;
#47552=CARTESIAN_POINT ( 'NONE',  ( 37.00000000000000711, -3.213188559034160452, 11.29812557209479706 ) ) ;
#47553=DIRECTION ( 'NONE',  ( 1.000000000000000000, 0.000000000000000000, 0.000000000000000000 ) ) ;
#47554=CARTESIAN_POINT ( 'NONE',  ( 35.00000000000000000, -6.946017217730008575, -10.01317267707884184 ) ) ;
#47555=CIRCLE ( 'NONE', #46495, 12.18649999999999878 ) ;
#47562=EDGE_CURVE ( 'NONE', #52191, #35667, #8382, .T. ) ;
#47563=ORIENTED_EDGE ( 'NONE', *, *, #48375, .T. ) ;
#47566=LINE ( 'NONE', #11978, #8795 ) ;
#47571=EDGE_LOOP ( 'NONE', ( #46678, #34027, #34439, #47042 ) ) ;
#47572=VERTEX_POINT ( 'NONE', #5854 ) ;
#47575=DIRECTION ( 'NONE',  ( 1.000000000000000000, 0.000000000000000000, 0.000000000000000000 ) ) ;
#47576=ADVANCED_FACE ( 'NONE', ( #836 ), #30432, .T. ) ;
#47577=ORIENTED_EDGE ( 'NONE', *, *, #51967, .T. ) ;
#47578=CARTESIAN_POINT ( 'NONE',  ( -35.00000000000000000, -5.273331777780412288, 10.49591321039678959 ) ) ;
#47580=CIRCLE ( 'NONE', #23138, 5.000000000000001776 ) ;
#47581=ORIENTED_EDGE ( 'NONE', *, *, #44829, .T. ) ;
#47582=CYLINDRICAL_SURFACE ( 'NONE', #29040, 5.000000000000001776 ) ;
#47584=ADVANCED_FACE ( 'NONE', ( #60050 ), #46076, .T. ) ;
#47586=CARTESIAN_POINT ( 'NONE',  ( 23.47346277817274185, -4.308697950774896590, 11.20435082111871417 ) ) ;
#47587=EDGE_LOOP ( 'NONE', ( #33044, #45, #733, #21696 ) ) ;
#47588=ORIENTED_EDGE ( 'NONE', *, *, #21566, .T. ) ;
#47589=AXIS2_PLACEMENT_3D ( 'NONE', #52363, #6149, #42025 ) ;
#47592=ORIENTED_EDGE ( 'NONE', *, *, #45680, .T. ) ;
#47595=CARTESIAN_POINT ( 'NONE',  ( -19.69476066079020171, -4.201994156881551312, 12.82938989607585789 ) ) ;
#47596=CARTESIAN_POINT ( 'NONE',  ( -19.55198024779261701, -3.902068674853255814, 11.34897822738861528 ) ) ;
#47599=DIRECTION ( 'NONE',  ( 0.000000000000000000, 0.01356324068817998940, -0.9999080150203990547 ) ) ;
#47600=EDGE_CURVE ( 'NONE', #16758, #47785, #40218, .T. ) ;
#47602=CYLINDRICAL_SURFACE ( 'NONE', #49102, 12.18650000000000055 ) ;
#47605=ORIENTED_EDGE ( 'NONE', *, *, #38376, .F. ) ;
#47606=DIRECTION ( 'NONE',  ( 0.000000000000000000, -0.01356324068817999114, 0.9999080150203989437 ) ) ;
#47608=DIRECTION ( 'NONE',  ( -1.000000000000000000, 0.000000000000000000, 0.000000000000000000 ) ) ;
#47609=ORIENTED_EDGE ( 'NONE', *, *, #13570, .T. ) ;
#47611=CARTESIAN_POINT ( 'NONE',  ( -27.27855387000350262, 12.26939275170278343, 5.631341004100471892 ) ) ;
#47612=CYLINDRICAL_SURFACE ( 'NONE', #43978, 4.999999999999999112 ) ;
#47613=ORIENTED_EDGE ( 'NONE', *, *, #43442, .T. ) ;
#47616=EDGE_CURVE ( 'NONE', #40241, #8833, #2021, .T. ) ;
#47618=ORIENTED_EDGE ( 'NONE', *, *, #2018, .T. ) ;
#47619=DIRECTION ( 'NONE',  ( 0.000000000000000000, -0.01356324068817998940, 0.9999080150203990547 ) ) ;
#47620=DIRECTION ( 'NONE',  ( -1.000000000000000000, 0.000000000000000000, 0.000000000000000000 ) ) ;
#47623=ORIENTED_EDGE ( 'NONE', *, *, #53102, .F. ) ;
#47624=CYLINDRICAL_SURFACE ( 'NONE', #63466, 12.75000000000000178 ) ;
#47626=CIRCLE ( 'NONE', #18966, 12.18650000000000055 ) ;
#47627=CARTESIAN_POINT ( 'NONE',  ( 37.00000000000000711, 4.705694406421931860E-17, -3.469127814946512892E-15 ) ) ;
#47632=CARTESIAN_POINT ( 'NONE',  ( -37.00000000000000711, 0.000000000000000000, 0.000000000000000000 ) ) ;
#47633=CYLINDRICAL_SURFACE ( 'NONE', #26153, 12.18650000000000055 ) ;
#47636=ORIENTED_EDGE ( 'NONE', *, *, #11944, .T. ) ;
#47637=CARTESIAN_POINT ( 'NONE',  ( 35.00000000000000000, 10.14433819232443490, 6.753013023069603271 ) ) ;
#47638=CARTESIAN_POINT ( 'NONE',  ( 35.00000000000000000, 4.237174932027400587, 12.02534193257715600 ) ) ;
#47639=VERTEX_POINT ( 'NONE', #60701 ) ;
#47644=DIRECTION ( 'NONE',  ( -1.000000000000000000, 0.000000000000000000, 0.000000000000000000 ) ) ;
#47645=ORIENTED_EDGE ( 'NONE', *, *, #15248, .F. ) ;
#47646=EDGE_CURVE ( 'NONE', #50397, #56080, #13685, .T. ) ;
#47648=VERTEX_POINT ( 'NONE', #188 ) ;
#47649=ORIENTED_EDGE ( 'NONE', *, *, #25734, .F. ) ;
#47650=DIRECTION ( 'NONE',  ( 0.000000000000000000, -0.01356324068818000328, 0.9999080150203990547 ) ) ;
#47651=AXIS2_PLACEMENT_3D ( 'NONE', #7716, #1749, #6405 ) ;
#47652=EDGE_CURVE ( 'NONE', #55512, #9384, #41308, .T. ) ;
#47653=ORIENTED_EDGE ( 'NONE', *, *, #47148, .T. ) ;
#47655=CARTESIAN_POINT ( 'NONE',  ( 0.9963060071168140519, 0.1253731440146732823, 13.50289960222859875 ) ) ;
#47656=CARTESIAN_POINT ( 'NONE',  ( 145.1370849898475797, 3.309064568108273190E-14, 0.000000000000000000 ) ) ;
#47658=ORIENTED_EDGE ( 'NONE', *, *, #10166, .F. ) ;
#47664=CARTESIAN_POINT ( 'NONE',  ( -24.33622492195127407, 7.892808082209504583, 9.041745503709938347 ) ) ;
#47665=ORIENTED_EDGE ( 'NONE', *, *, #28396, .T. ) ;
#47667=EDGE_CURVE ( 'NONE', #33621, #59239, #50075, .T. ) ;
#47670=ORIENTED_EDGE ( 'NONE', *, *, #19231, .F. ) ;
#47671=CARTESIAN_POINT ( 'NONE',  ( 35.00000000000000000, -0.4993900848168272288, -12.17626345777663488 ) ) ;
#47673=AXIS2_PLACEMENT_3D ( 'NONE', #40190, #34557, #55169 ) ;
#47675=EDGE_LOOP ( 'NONE', ( #13055, #16222, #53384, #43824 ) ) ;
#47676=CYLINDRICAL_SURFACE ( 'NONE', #2825, 12.74999999999999822 ) ;
#47678=CARTESIAN_POINT ( 'NONE',  ( 13.11132293240999758, 11.59456066430334609, -6.918089050757264324 ) ) ;
#47679=ORIENTED_EDGE ( 'NONE', *, *, #42349, .F. ) ;
#47680=VECTOR ( 'NONE', #37316, 1000.000000000000000 ) ;
#47681=EDGE_LOOP ( 'NONE', ( #37469, #50498, #3683, #8363 ) ) ;
#47683=ORIENTED_EDGE ( 'NONE', *, *, #57411, .T. ) ;
#47684=EDGE_CURVE ( 'NONE', #9977, #41254, #25373, .T. ) ;
#47685=AXIS2_PLACEMENT_3D ( 'NONE', #45152, #30499, #25514 ) ;
#47686=ADVANCED_FACE ( 'NONE', ( #47058 ), #21448, .T. ) ;
#47687=ORIENTED_EDGE ( 'NONE', *, *, #1987, .T. ) ;
#47688=LINE ( 'NONE', #33032, #37012 ) ;
#47689=CARTESIAN_POINT ( 'NONE',  ( -18.49080574448680991, -12.00000000000057909, -4.407108900774715188E-13 ) ) ;
#47691=CARTESIAN_POINT ( 'NONE',  ( -47.00000000000000711, 0.000000000000000000, 0.000000000000000000 ) ) ;
#47693=DIRECTION ( 'NONE',  ( 0.000000000000000000, 0.4134677391718512562, 0.9105187689795954942 ) ) ;
#47695=ADVANCED_FACE ( 'NONE', ( #36738 ), #57031, .F. ) ;
#47697=ADVANCED_FACE ( 'NONE', ( #37381 ), #21103, .F. ) ;
#47698=ORIENTED_EDGE ( 'NONE', *, *, #24835, .T. ) ;
#47701=CARTESIAN_POINT ( 'NONE',  ( -37.00000000000000711, -7.817610399097453922, -8.766823244862070652 ) ) ;
#47703=DIRECTION ( 'NONE',  ( 0.000000000000000000, 0.01356324068817991828, -0.9999080150203990547 ) ) ;
#47704=AXIS2_PLACEMENT_3D ( 'NONE', #20557, #45478, #14245 ) ;
#47705=FACE_OUTER_BOUND ( 'NONE', #3784, .T. ) ;
#47706=AXIS2_PLACEMENT_3D ( 'NONE', #56619, #61917, #1740 ) ;
#47708=CARTESIAN_POINT ( 'NONE',  ( 10.27842187895016224, 1.477547723869735874, -11.90968538141293998 ) ) ;
#47710=CARTESIAN_POINT ( 'NONE',  ( -35.00000000000000000, 0.000000000000000000, 0.000000000000000000 ) ) ;
#47712=CARTESIAN_POINT ( 'NONE',  ( 47.00000000000000711, 4.705694406421931860E-17, -3.469127814946512892E-15 ) ) ;
#47717=CYLINDRICAL_SURFACE ( 'NONE', #58537, 12.75000000000000178 ) ;
#47718=VECTOR ( 'NONE', #31205, 1000.000000000000000 ) ;
#47719=ORIENTED_EDGE ( 'NONE', *, *, #65343, .T. ) ;
#47720=DIRECTION ( 'NONE',  ( 1.000000000000000000, 0.000000000000000000, 0.000000000000000000 ) ) ;
#47721=FACE_OUTER_BOUND ( 'NONE', #62619, .T. ) ;
#47727=VERTEX_POINT ( 'NONE', #1826 ) ;
#47729=AXIS2_PLACEMENT_3D ( 'NONE', #51324, #46323, #56960 ) ;
#47730=ORIENTED_EDGE ( 'NONE', *, *, #2808, .T. ) ;
#47731=CARTESIAN_POINT ( 'NONE',  ( -4.989057617119011745, -0.9162120371760335003, -11.96497202265568660 ) ) ;
#47732=DIRECTION ( 'NONE',  ( 1.000000000000000000, 0.000000000000000000, -0.000000000000000000 ) ) ;
#47733=ORIENTED_EDGE ( 'NONE', *, *, #21091, .T. ) ;
#47737=DIRECTION ( 'NONE',  ( 0.000000000000000000, -0.01356324068817998940, 0.9999080150203990547 ) ) ;
#47739=CARTESIAN_POINT ( 'NONE',  ( -2.952869152607111136, -7.581333670610126418, 11.17020052527586138 ) ) ;
#47740=CARTESIAN_POINT ( 'NONE',  ( 26.34661844826604593, 13.08594712317291986, 3.317828791472332117 ) ) ;
#47741=LINE ( 'NONE', #53051, #25490 ) ;
#47744=EDGE_CURVE ( 'NONE', #39914, #14488, #46639, .T. ) ;
#47745=ORIENTED_EDGE ( 'NONE', *, *, #30914, .F. ) ;
#47746=CARTESIAN_POINT ( 'NONE',  ( -37.00000000000000711, 9.390600770287994337, 8.624332853796092380 ) ) ;
#47747=EDGE_LOOP ( 'NONE', ( #33611, #46252, #14426, #58804 ) ) ;
#47748=ORIENTED_EDGE ( 'NONE', *, *, #44600, .T. ) ;
#47753=CIRCLE ( 'NONE', #32872, 5.000000000000000000 ) ;
#47755=CARTESIAN_POINT ( 'NONE',  ( 22.78386511336923093, 3.290201280387628824, 13.09362067330721757 ) ) ;
#47757=CARTESIAN_POINT ( 'NONE',  ( -24.31546255402668422, -8.695390788176707630, 8.272891244190285320 ) ) ;
#47758=CIRCLE ( 'NONE', #59427, 12.75000000000000178 ) ;
#47761=VERTEX_POINT ( 'NONE', #22417 ) ;
#47762=CARTESIAN_POINT ( 'NONE',  ( -37.00000000000000711, -9.430788938294107027, 7.718225330433774900 ) ) ;
#47764=CARTESIAN_POINT ( 'NONE',  ( -37.00000000000000711, 0.000000000000000000, 0.000000000000000000 ) ) ;
#47766=CARTESIAN_POINT ( 'NONE',  ( 8.937200413558842982, 4.476360154859214902, 12.73625532737129795 ) ) ;
#47767=ADVANCED_FACE ( 'NONE', ( #62985 ), #12427, .T. ) ;
#47769=VECTOR ( 'NONE', #8011, 1000.000000000000000 ) ;
#47770=DIRECTION ( 'NONE',  ( 0.000000000000000000, 0.5243256840888563808, 0.8515178078024867592 ) ) ;
#47772=EDGE_CURVE ( 'NONE', #29225, #51071, #7318, .T. ) ;
#47775=ORIENTED_EDGE ( 'NONE', *, *, #34808, .T. ) ;
#47776=( BOUNDED_CURVE ( )  B_SPLINE_CURVE ( 3, ( #49016, #18750, #39007, #13726 ),
 .UNSPECIFIED., .F., .F. ) 
 B_SPLINE_CURVE_WITH_KNOTS ( ( 4, 4 ),
 ( 4.607305308089706841, 4.644469214066985430 ),
 .UNSPECIFIED. ) 
 CURVE ( )  GEOMETRIC_REPRESENTATION_ITEM ( )  RATIONAL_B_SPLINE_CURVE ( ( 1.000000000000000000, 0.9998849069861288630, 0.9998849069861288630, 1.000000000000000000 ) ) 
 REPRESENTATION_ITEM ( '' )  );
#47777=ORIENTED_EDGE ( 'NONE', *, *, #9405, .F. ) ;
#47778=EDGE_CURVE ( 'NONE', #13458, #20614, #44847, .T. ) ;
#47780=CARTESIAN_POINT ( 'NONE',  ( -9.183025528901289647, -11.31491075083350495, -7.371853674845621818 ) ) ;
#47782=AXIS2_PLACEMENT_3D ( 'NONE', #978, #11281, #36199 ) ;
#47783=CARTESIAN_POINT ( 'NONE',  ( -37.00000000000000711, -4.946702696913093611, -11.13736569743279681 ) ) ;
#47785=VERTEX_POINT ( 'NONE', #7799 ) ;
#47787=ORIENTED_EDGE ( 'NONE', *, *, #26628, .T. ) ;
#47789=LINE ( 'NONE', #63077, #42017 ) ;
#47790=DIRECTION ( 'NONE',  ( 0.000000000000000000, 0.01356324068817991828, -0.9999080150203990547 ) ) ;
#47792=ORIENTED_EDGE ( 'NONE', *, *, #47460, .T. ) ;
#47794=DIRECTION ( 'NONE',  ( 0.000000000000000000, -0.1118654143051685396, -0.9937233664769753450 ) ) ;
#47795=CARTESIAN_POINT ( 'NONE',  ( -35.00000000000000000, -12.74068829017553384, -0.4871980014162800021 ) ) ;
#47797=AXIS2_PLACEMENT_3D ( 'NONE', #6677, #56559, #26948 ) ;
#47798=EDGE_CURVE ( 'NONE', #3402, #53501, #29624, .T. ) ;
#47799=AXIS2_PLACEMENT_3D ( 'NONE', #11861, #48124, #37128 ) ;
#47800=DIRECTION ( 'NONE',  ( 0.000000000000000000, -0.4935949184179134752, 0.8696919319575254770 ) ) ;
#47801=EDGE_CURVE ( 'NONE', #54960, #50930, #15807, .T. ) ;
#47803=VERTEX_POINT ( 'NONE', #39025 ) ;
#47804=EDGE_LOOP ( 'NONE', ( #42651, #26113, #2281, #60487 ) ) ;
#47805=DIRECTION ( 'NONE',  ( 1.000000000000000000, -0.000000000000000000, 0.000000000000000000 ) ) ;
#47806=CARTESIAN_POINT ( 'NONE',  ( 18.84867683979356201, -5.944105725974474730, 12.12095735156416509 ) ) ;
#47807=CARTESIAN_POINT ( 'NONE',  ( 35.00000000000000000, 4.705694406421931860E-17, -3.469127814946512892E-15 ) ) ;
#47809=CARTESIAN_POINT ( 'NONE',  ( 37.00000000000000711, -8.146229107149464355, -9.063649021438928699 ) ) ;
#47814=EDGE_LOOP ( 'NONE', ( #62788, #53184, #64098, #26221 ) ) ;
#47815=CARTESIAN_POINT ( 'NONE',  ( -1.734723475976807094E-15, -3.469446951953614189E-15, 12.00000000000000178 ) ) ;
#47816=FACE_OUTER_BOUND ( 'NONE', #16390, .T. ) ;
#47817=DIRECTION ( 'NONE',  ( 0.000000000000000000, 0.01356324068817992175, -0.9999080150203990547 ) ) ;
#47819=DIRECTION ( 'NONE',  ( 0.000000000000000000, -0.01356324068817992522, 0.9999080150203990547 ) ) ;
#47822=ORIENTED_EDGE ( 'NONE', *, *, #17408, .F. ) ;
#47823=EDGE_CURVE ( 'NONE', #31374, #57610, #43684, .T. ) ;
#47824=ADVANCED_FACE ( 'NONE', ( #2831 ), #49034, .T. ) ;
#47825=ORIENTED_EDGE ( 'NONE', *, *, #60566, .F. ) ;
#47827=AXIS2_PLACEMENT_3D ( 'NONE', #26481, #46769, #36793 ) ;
#47828=ORIENTED_EDGE ( 'NONE', *, *, #11464, .T. ) ;
#47829=FILL_AREA_STYLE ('',( #32189 ) ) ;
#47831=CARTESIAN_POINT ( 'NONE',  ( 21.44386431903875234, -13.23489694407720663, -2.693023235911562452 ) ) ;
#47832=CARTESIAN_POINT ( 'NONE',  ( 17.22995070708839904, 10.79921756342612404, 8.109772993617433201 ) ) ;
#47835=AXIS2_PLACEMENT_3D ( 'NONE', #28058, #2806, #23068 ) ;
#47836=DIRECTION ( 'NONE',  ( 0.8914382917301157949, 0.000000000000000000, -0.4531421102008653112 ) ) ;
#47837=CYLINDRICAL_SURFACE ( 'NONE', #29676, 12.74999999999999822 ) ;
#47839=ORIENTED_EDGE ( 'NONE', *, *, #56783, .T. ) ;
#47840=ORIENTED_EDGE ( 'NONE', *, *, #53422, .F. ) ;
#47844=ORIENTED_EDGE ( 'NONE', *, *, #41479, .F. ) ;
#47845=CARTESIAN_POINT ( 'NONE',  ( 35.00000000000000000, -11.29812557209478996, -3.213188559034203529 ) ) ;
#47846=ORIENTED_EDGE ( 'NONE', *, *, #15300, .F. ) ;
#47847=ORIENTED_EDGE ( 'NONE', *, *, #57282, .T. ) ;
#47848=DIRECTION ( 'NONE',  ( 1.000000000000000000, 0.000000000000000000, 0.000000000000000000 ) ) ;
#47851=CIRCLE ( 'NONE', #7477, 12.18649999999999878 ) ;
#47854=DIRECTION ( 'NONE',  ( 0.000000000000000000, -0.01356324068817991828, 0.9999080150203990547 ) ) ;
#47855=FACE_OUTER_BOUND ( 'NONE', #8250, .T. ) ;
#47856=VECTOR ( 'NONE', #59844, 1000.000000000000000 ) ;
#47857=EDGE_CURVE ( 'NONE', #60345, #44318, #987, .T. ) ;
#47858=CARTESIAN_POINT ( 'NONE',  ( -35.00000000000000000, 9.240395740215735287, -7.251710744571480127 ) ) ;
#47859=ORIENTED_EDGE ( 'NONE', *, *, #64538, .T. ) ;
#47862=CARTESIAN_POINT ( 'NONE',  ( 29.71521259808911353, 6.759044707574296318, 9.927718093057791293 ) ) ;
#47863=DIRECTION ( 'NONE',  ( -1.000000000000000000, 0.000000000000000000, 0.000000000000000000 ) ) ;
#47864=DIRECTION ( 'NONE',  ( 0.000000000000000000, -0.6478160128811839558, 0.7617968321374970486 ) ) ;
#47866=ORIENTED_EDGE ( 'NONE', *, *, #59913, .F. ) ;
#47869=AXIS2_PLACEMENT_3D ( 'NONE', #49346, #39317, #53663 ) ;
#47870=EDGE_LOOP ( 'NONE', ( #11336, #13248, #54921, #58427 ) ) ;
#47871=CARTESIAN_POINT ( 'NONE',  ( 37.00000000000000711, 0.01609748574445066943, -11.74614673114903773 ) ) ;
#47874=VECTOR ( 'NONE', #26343, 1000.000000000000000 ) ;
#47877=VERTEX_POINT ( 'NONE', #3149 ) ;
#47878=DIRECTION ( 'NONE',  ( 0.000000000000000000, -0.9651210252299822212, -0.2618041379715529970 ) ) ;
#47879=CARTESIAN_POINT ( 'NONE',  ( -37.00000000000000711, 9.217970097227725645, 7.971186206369506699 ) ) ;
#47880=VECTOR ( 'NONE', #39582, 1000.000000000000000 ) ;
#47881=CARTESIAN_POINT ( 'NONE',  ( -18.04458733766117362, -12.91933584589293282, 3.916728392552376370 ) ) ;
#47882=DIRECTION ( 'NONE',  ( -0.000000000000000000, -1.000000000000000000, -0.000000000000000000 ) ) ;
#47883=AXIS2_PLACEMENT_3D ( 'NONE', #54878, #44237, #13329 ) ;
#47884=EDGE_CURVE ( 'NONE', #8663, #5051, #63614, .T. ) ;
#47886=ORIENTED_EDGE ( 'NONE', *, *, #18619, .F. ) ;
#47889=CIRCLE ( 'NONE', #38331, 5.000000000000000000 ) ;
#47892=AXIS2_PLACEMENT_3D ( 'NONE', #1910, #62402, #47150 ) ;
#47893=EDGE_CURVE ( 'NONE', #42133, #40353, #33708, .T. ) ;
#47894=VECTOR ( 'NONE', #37837, 1000.000000000000000 ) ;
#47895=ORIENTED_EDGE ( 'NONE', *, *, #4518, .T. ) ;
#47896=CARTESIAN_POINT ( 'NONE',  ( 10.75853767213705225, 7.830989516993144051, -9.092612561015865680 ) ) ;
#47900=AXIS2_PLACEMENT_3D ( 'NONE', #20456, #51049, #25119 ) ;
#47904=ORIENTED_EDGE ( 'NONE', *, *, #12556, .F. ) ;
#47906=ORIENTED_EDGE ( 'NONE', *, *, #49450, .F. ) ;
#47907=DIRECTION ( 'NONE',  ( 0.000000000000000000, -0.6269146997508042718, -0.7790879021242460567 ) ) ;
#47908=AXIS2_PLACEMENT_3D ( 'NONE', #7940, #37852, #57830 ) ;
#47909=AXIS2_PLACEMENT_3D ( 'NONE', #58697, #44034, #64306 ) ;
#47911=ORIENTED_EDGE ( 'NONE', *, *, #55567, .T. ) ;
#47912=LINE ( 'NONE', #2372, #1808 ) ;
#47914=LINE ( 'NONE', #2374, #52341 ) ;
#47916=CARTESIAN_POINT ( 'NONE',  ( -37.00000000000000711, -8.839356091079983102, -8.389074212634382022 ) ) ;
#47917=DIRECTION ( 'NONE',  ( 1.000000000000000000, 0.000000000000000000, 0.000000000000000000 ) ) ;
#47918=CARTESIAN_POINT ( 'NONE',  ( 24.19646710323674554, 1.946597173898756861, 11.84653191271039852 ) ) ;
#47921=DIRECTION ( 'NONE',  ( 0.000000000000000000, 0.9346839223284553189, -0.3554799084908935036 ) ) ;
#47923=CARTESIAN_POINT ( 'NONE',  ( -35.00000000000000000, 0.000000000000000000, 0.000000000000000000 ) ) ;
#47924=ORIENTED_EDGE ( 'NONE', *, *, #13804, .T. ) ;
#47928=EDGE_CURVE ( 'NONE', #54691, #56717, #15402, .T. ) ;
#47929=FACE_OUTER_BOUND ( 'NONE', #56117, .T. ) ;
#47931=DIRECTION ( 'NONE',  ( -0.000000000000000000, -1.000000000000000000, -0.000000000000000000 ) ) ;
#47933=DIRECTION ( 'NONE',  ( -1.000000000000000000, 0.000000000000000000, 0.000000000000000000 ) ) ;
#47934=ORIENTED_EDGE ( 'NONE', *, *, #59126, .T. ) ;
#47936=AXIS2_PLACEMENT_3D ( 'NONE', #47451, #11208, #31485 ) ;
#47939=LINE ( 'NONE', #42940, #21315 ) ;
#47940=AXIS2_PLACEMENT_3D ( 'NONE', #478, #51988, #1115 ) ;
#47941=ORIENTED_EDGE ( 'NONE', *, *, #53963, .F. ) ;
#47948=CIRCLE ( 'NONE', #56430, 4.999999999999999112 ) ;
#47951=FACE_OUTER_BOUND ( 'NONE', #13782, .T. ) ;
#47954=DIRECTION ( 'NONE',  ( 1.000000000000000000, 0.000000000000000000, 0.000000000000000000 ) ) ;
#47955=FACE_OUTER_BOUND ( 'NONE', #39209, .T. ) ;
#47956=CARTESIAN_POINT ( 'NONE',  ( -7.291047549687194262, 5.640864668324928388, -10.59540170654024749 ) ) ;
#47958=ORIENTED_EDGE ( 'NONE', *, *, #46129, .F. ) ;
#47959=DIRECTION ( 'NONE',  ( -1.000000000000000000, 0.000000000000000000, -0.000000000000000000 ) ) ;
#47960=VECTOR ( 'NONE', #33024, 1000.000000000000000 ) ;
#47964=CARTESIAN_POINT ( 'NONE',  ( -37.00000000000000711, 0.000000000000000000, 0.000000000000000000 ) ) ;
#47966=CARTESIAN_POINT ( 'NONE',  ( 22.46858150504636242, 12.34520901837059448, -5.474447245564200593 ) ) ;
#47967=DIRECTION ( 'NONE',  ( 1.000000000000000000, 0.000000000000000000, 0.000000000000000000 ) ) ;
#47968=ADVANCED_FACE ( 'NONE', ( #20059 ), #35980, .T. ) ;
#47969=FACE_OUTER_BOUND ( 'NONE', #18596, .T. ) ;
#47972=AXIS2_PLACEMENT_3D ( 'NONE', #57028, #46072, #36051 ) ;
#47974=VERTEX_POINT ( 'NONE', #450 ) ;
#47976=CARTESIAN_POINT ( 'NONE',  ( 6.023978964358256860, -8.806351789236446237, 10.23755192329234553 ) ) ;
#47977=CIRCLE ( 'NONE', #24623, 4.999999999999999112 ) ;
#47981=ORIENTED_EDGE ( 'NONE', *, *, #13925, .T. ) ;
#47982=CIRCLE ( 'NONE', #28700, 1.750000000000000000 ) ;
#47983=AXIS2_PLACEMENT_3D ( 'NONE', #53134, #7577, #27866 ) ;
#47984=CYLINDRICAL_SURFACE ( 'NONE', #30974, 5.000000000000000888 ) ;
#47985=ORIENTED_EDGE ( 'NONE', *, *, #15250, .F. ) ;
#47986=EDGE_CURVE ( 'NONE', #31670, #22816, #60978, .T. ) ;
#47988=VERTEX_POINT ( 'NONE', #55649 ) ;
#47989=VERTEX_POINT ( 'NONE', #60961 ) ;
#47991=CIRCLE ( 'NONE', #63876, 12.18650000000000055 ) ;
#47992=VECTOR ( 'NONE', #30687, 1000.000000000000000 ) ;
#47993=ORIENTED_EDGE ( 'NONE', *, *, #24056, .F. ) ;
#47995=CARTESIAN_POINT ( 'NONE',  ( -24.94425671793833388, -9.239554407049443085, 7.659171101073906307 ) ) ;
#47996=CARTESIAN_POINT ( 'NONE',  ( 0.6525221082932635142, -0.1557174252009511373, 13.50151297108246595 ) ) ;
#47997=DIRECTION ( 'NONE',  ( -1.000000000000000000, -0.000000000000000000, 0.000000000000000000 ) ) ;
#47998=DIRECTION ( 'NONE',  ( 0.000000000000000000, -0.01356324068817998940, 0.9999080150203990547 ) ) ;
#47999=VERTEX_POINT ( 'NONE', #5434 ) ;
#48002=DIRECTION ( 'NONE',  ( -1.000000000000000000, 0.000000000000000000, 0.000000000000000000 ) ) ;
#48003=DIRECTION ( 'NONE',  ( -1.000000000000000000, 0.000000000000000000, 0.000000000000000000 ) ) ;
#48004=ORIENTED_EDGE ( 'NONE', *, *, #3153, .T. ) ;
#48008=EDGE_LOOP ( 'NONE', ( #13968, #14056, #60725, #24384 ) ) ;
#48010=AXIS2_PLACEMENT_3D ( 'NONE', #76, #56607, #21002 ) ;
#48013=AXIS2_PLACEMENT_3D ( 'NONE', #12533, #27851, #32812 ) ;
#48014=PLANE ( 'NONE',  #40839 ) ;
#48016=DIRECTION ( 'NONE',  ( -1.000000000000000000, 0.000000000000000000, 0.000000000000000000 ) ) ;
#48017=VECTOR ( 'NONE', #47397, 1000.000000000000000 ) ;
#48021=ORIENTED_EDGE ( 'NONE', *, *, #51569, .F. ) ;
#48022=VECTOR ( 'NONE', #7024, 1000.000000000000000 ) ;
#48024=DIRECTION ( 'NONE',  ( 0.000000000000000000, -0.5987040770935561085, 0.8009703041134255130 ) ) ;
#48026=DIRECTION ( 'NONE',  ( 1.000000000000000000, 0.000000000000000000, 0.000000000000000000 ) ) ;
#48028=CARTESIAN_POINT ( 'NONE',  ( 145.1370849898475797, 3.309064568108273190E-14, 0.000000000000000000 ) ) ;
#48030=CARTESIAN_POINT ( 'NONE',  ( 36.00000000000000711, 12.26766708251991567, -3.473736367725301033 ) ) ;
#48032=AXIS2_PLACEMENT_3D ( 'NONE', #59378, #18169, #38777 ) ;
#48033=VERTEX_POINT ( 'NONE', #11072 ) ;
#48034=LINE ( 'NONE', #25521, #34473 ) ;
#48039=LINE ( 'NONE', #1829, #63012 ) ;
#48042=EDGE_CURVE ( 'NONE', #58393, #13080, #18024, .T. ) ;
#48044=CARTESIAN_POINT ( 'NONE',  ( -37.00000000000000711, 0.000000000000000000, 0.000000000000000000 ) ) ;
#48045=EDGE_CURVE ( 'NONE', #33727, #42381, #21712, .T. ) ;
#48046=CARTESIAN_POINT ( 'NONE',  ( 10.67051787153030595, 1.171189490780102593, -11.94370412967601780 ) ) ;
#48049=CARTESIAN_POINT ( 'NONE',  ( 37.00000000000000711, 4.705694406421931860E-17, -3.469127814946512892E-15 ) ) ;
#48050=CARTESIAN_POINT ( 'NONE',  ( -19.47984447937493613, -3.750539801530005768, 25.00000000000000000 ) ) ;
#48051=CYLINDRICAL_SURFACE ( 'NONE', #14125, 12.74999999999999822 ) ;
#48052=CARTESIAN_POINT ( 'NONE',  ( 35.00000000000000000, -0.7536123767497623360, 11.72195762423410237 ) ) ;
#48053=AXIS2_PLACEMENT_3D ( 'NONE', #48088, #57396, #52427 ) ;
#48054=AXIS2_PLACEMENT_3D ( 'NONE', #11480, #52062, #6511 ) ;
#48055=ADVANCED_FACE ( 'NONE', ( #11382 ), #57278, .T. ) ;
#48056=DIRECTION ( 'NONE',  ( -1.000000000000000000, 0.000000000000000000, -0.000000000000000000 ) ) ;
#48058=AXIS2_PLACEMENT_3D ( 'NONE', #3701, #23963, #13951 ) ;
#48059=ORIENTED_EDGE ( 'NONE', *, *, #33853, .T. ) ;
#48060=CARTESIAN_POINT ( 'NONE',  ( 17.82596851127161841, -8.594641745053730020, 8.387315214446159573 ) ) ;
#48063=CARTESIAN_POINT ( 'NONE',  ( 10.75853767213705048, 7.830989516993144051, 10.99661780661416088 ) ) ;
#48065=ORIENTED_EDGE ( 'NONE', *, *, #54223, .T. ) ;
#48066=DIRECTION ( 'NONE',  ( -1.000000000000000000, -1.836970198721029688E-16, 0.000000000000000000 ) ) ;
#48067=DIRECTION ( 'NONE',  ( 0.000000000000000000, 0.01356324068817998940, -0.9999080150203989437 ) ) ;
#48068=EDGE_LOOP ( 'NONE', ( #30950, #731, #33305, #38201 ) ) ;
#48069=ORIENTED_EDGE ( 'NONE', *, *, #58682, .T. ) ;
#48070=LINE ( 'NONE', #27431, #7645 ) ;
#48071=EDGE_CURVE ( 'NONE', #63981, #4532, #21187, .T. ) ;
#48072=DIRECTION ( 'NONE',  ( -1.000000000000000000, 0.000000000000000000, 0.000000000000000000 ) ) ;
#48074=EDGE_CURVE ( 'NONE', #26195, #50843, #62564, .T. ) ;
#48075=DIRECTION ( 'NONE',  ( -1.000000000000000000, 0.000000000000000000, 0.000000000000000000 ) ) ;
#48076=CIRCLE ( 'NONE', #10897, 4.999999999999999112 ) ;
#48077=CARTESIAN_POINT ( 'NONE',  ( 37.00000000000000711, 6.946017217730083182, 10.01317267707878678 ) ) ;
#48078=CARTESIAN_POINT ( 'NONE',  ( -37.00000000000000711, -4.237620530777717498, -11.42599468261433771 ) ) ;
#48079=CARTESIAN_POINT ( 'NONE',  ( -35.00000000000000000, 3.916263239775508165, -11.07407352312208459 ) ) ;
#48080=CARTESIAN_POINT ( 'NONE',  ( -27.39656561727367290, 9.459410533876226879, -7.405734381554731627 ) ) ;
#48081=ADVANCED_FACE ( 'NONE', ( #31652 ), #1753, .T. ) ;
#48083=CYLINDRICAL_SURFACE ( 'NONE', #45665, 4.999999999999998224 ) ;
#48088=CARTESIAN_POINT ( 'NONE',  ( 37.00000000000000711, 4.705694406421931860E-17, -3.469127814946512892E-15 ) ) ;
#48093=CARTESIAN_POINT ( 'NONE',  ( -14.64443717355071151, 8.412151427010677196, 10.55874966731845710 ) ) ;
#48096=AXIS2_PLACEMENT_3D ( 'NONE', #34938, #18719, #34624 ) ;
#48099=ORIENTED_EDGE ( 'NONE', *, *, #46689, .T. ) ;
#48100=DIRECTION ( 'NONE',  ( 1.000000000000000000, 0.000000000000000000, 0.000000000000000000 ) ) ;
#48101=DIRECTION ( 'NONE',  ( 0.000000000000000000, -0.01356324068817998940, 0.9999080150203990547 ) ) ;
#48102=CARTESIAN_POINT ( 'NONE',  ( 37.00000000000000711, 2.527899948230813987, 12.49688848680881037 ) ) ;
#48103=VERTEX_POINT ( 'NONE', #6407 ) ;
#48104=ORIENTED_EDGE ( 'NONE', *, *, #1493, .T. ) ;
#48106=ORIENTED_EDGE ( 'NONE', *, *, #27487, .T. ) ;
#48107=CIRCLE ( 'NONE', #50246, 12.18649999999999878 ) ;
#48108=CARTESIAN_POINT ( 'NONE',  ( -35.00000000000000000, 11.67026961469348123, 4.564151185897117102 ) ) ;
#48110=CARTESIAN_POINT ( 'NONE',  ( 36.00000000000000711, 11.10408318471059452, -6.265926637539535271 ) ) ;
#48111=CARTESIAN_POINT ( 'NONE',  ( -37.00000000000000711, -3.033604067594665388, 12.38385022362080967 ) ) ;
#48113=ADVANCED_FACE ( 'NONE', ( #42270 ), #21364, .T. ) ;
#48114=EDGE_CURVE ( 'NONE', #5549, #44780, #41965, .T. ) ;
#48117=CARTESIAN_POINT ( 'NONE',  ( -35.00000000000000000, 9.821084925794572484, 7.215058775251292467 ) ) ;
#48118=ORIENTED_EDGE ( 'NONE', *, *, #22198, .F. ) ;
#48119=LINE ( 'NONE', #2896, #44382 ) ;
#48120=ORIENTED_EDGE ( 'NONE', *, *, #24861, .T. ) ;
#48122=DIRECTION ( 'NONE',  ( 1.000000000000000000, 0.000000000000000000, 0.000000000000000000 ) ) ;
#48123=DIRECTION ( 'NONE',  ( 1.000000000000000000, 0.000000000000000000, -0.000000000000000000 ) ) ;
#48124=DIRECTION ( 'NONE',  ( 1.000000000000000000, 0.000000000000000000, 0.000000000000000000 ) ) ;
#48125=EDGE_CURVE ( 'NONE', #32242, #6535, #15855, .T. ) ;
#48126=CARTESIAN_POINT ( 'NONE',  ( 29.51976981715666781, 4.571419055710094881, 11.09513982864076276 ) ) ;
#48127=ORIENTED_EDGE ( 'NONE', *, *, #10807, .F. ) ;
#48128=ORIENTED_EDGE ( 'NONE', *, *, #52269, .F. ) ;
#48129=AXIS2_PLACEMENT_3D ( 'NONE', #50085, #34752, #9827 ) ;
#48132=ORIENTED_EDGE ( 'NONE', *, *, #31753, .F. ) ;
#48133=CARTESIAN_POINT ( 'NONE',  ( -35.00000000000000000, 0.000000000000000000, 0.000000000000000000 ) ) ;
#48134=CARTESIAN_POINT ( 'NONE',  ( 37.00000000000000711, 4.705694406421931860E-17, -3.469127814946512892E-15 ) ) ;
#48137=ADVANCED_FACE ( 'NONE', ( #19634 ), #15914, .T. ) ;
#48138=EDGE_LOOP ( 'NONE', ( #12349, #24096, #25618, #19917 ) ) ;
#48142=CIRCLE ( 'NONE', #31121, 5.000000000000000000 ) ;
#48145=CIRCLE ( 'NONE', #1437, 12.74999999999999822 ) ;
#48146=CIRCLE ( 'NONE', #37488, 4.999999999999998224 ) ;
#48149=ORIENTED_EDGE ( 'NONE', *, *, #19207, .F. ) ;
#48150=CARTESIAN_POINT ( 'NONE',  ( -35.00000000000000000, -12.01765980939843281, 2.021542716731355771 ) ) ;
#48151=CARTESIAN_POINT ( 'NONE',  ( 29.68049421394466236, 10.47771764608172695, 8.515736641621126424 ) ) ;
#48152=EDGE_CURVE ( 'NONE', #15867, #4408, #23338, .T. ) ;
#48156=CARTESIAN_POINT ( 'NONE',  ( -11.37097780465418140, -6.763195055119394006, -11.69186615500488280 ) ) ;
#48161=CARTESIAN_POINT ( 'NONE',  ( -29.06964327085373156, 3.363168872084723038, -13.08058491801428680 ) ) ;
#48163=ADVANCED_FACE ( 'NONE', ( #24605 ), #46214, .T. ) ;
#48164=CIRCLE ( 'NONE', #56651, 12.18650000000000055 ) ;
#48165=ORIENTED_EDGE ( 'NONE', *, *, #58276, .T. ) ;
#48166=VERTEX_POINT ( 'NONE', #329 ) ;
#48168=EDGE_CURVE ( 'NONE', #42404, #35654, #45876, .T. ) ;
#48169=VERTEX_POINT ( 'NONE', #60174 ) ;
#48171=DIRECTION ( 'NONE',  ( 0.000000000000000000, -0.01356324068817991828, 0.9999080150203990547 ) ) ;
#48173=DIRECTION ( 'NONE',  ( 0.000000000000000000, 0.4935949184179261318, -0.8696919319575183716 ) ) ;
#48175=B_SPLINE_CURVE_WITH_KNOTS ( 'NONE', 3,
 ( #58118, #38137, #12532, #43450, #58795, #28828, #53466, #13835, #32811, #58446 ),
 .UNSPECIFIED., .F., .F.,
 ( 4, 2, 2, 2, 4 ),
 ( 1.734723475976807094E-18, 0.0006656689435785632762, 0.001331337887157124818, 0.001997006830735686359, 0.002662675774314247901 ),
 .UNSPECIFIED. ) ;
#48176=CIRCLE ( 'NONE', #22676, 5.000000000000000888 ) ;
#48177=EDGE_CURVE ( 'NONE', #24790, #43796, #59816, .T. ) ;
#48178=DIRECTION ( 'NONE',  ( -1.000000000000000000, 0.000000000000000000, 0.000000000000000000 ) ) ;
#48179=CARTESIAN_POINT ( 'NONE',  ( -37.00000000000000711, -1.791059740004510070, 12.05416472667165273 ) ) ;
#48180=ORIENTED_EDGE ( 'NONE', *, *, #6269, .F. ) ;
#48181=ORIENTED_EDGE ( 'NONE', *, *, #59830, .T. ) ;
#48182=CYLINDRICAL_SURFACE ( 'NONE', #10874, 12.18650000000000055 ) ;
#48183=ORIENTED_EDGE ( 'NONE', *, *, #33124, .T. ) ;
#48185=FACE_OUTER_BOUND ( 'NONE', #15321, .T. ) ;
#48186=AXIS2_PLACEMENT_3D ( 'NONE', #23633, #64496, #4331 ) ;
#48189=DIRECTION ( 'NONE',  ( -1.000000000000000000, 0.000000000000000000, -0.000000000000000000 ) ) ;
#48192=DIRECTION ( 'NONE',  ( -1.000000000000000000, -0.000000000000000000, -0.000000000000000000 ) ) ;
#48193=ORIENTED_EDGE ( 'NONE', *, *, #56293, .T. ) ;
#48194=EDGE_LOOP ( 'NONE', ( #38274, #40055, #64254, #47687 ) ) ;
#48195=DIRECTION ( 'NONE',  ( -1.000000000000000000, 0.000000000000000000, 0.000000000000000000 ) ) ;
#48197=AXIS2_PLACEMENT_3D ( 'NONE', #2626, #22889, #53482 ) ;
#48198=CARTESIAN_POINT ( 'NONE',  ( 35.00000000000000000, -4.732539170486179003, 11.23004253107769124 ) ) ;
#48199=ORIENTED_EDGE ( 'NONE', *, *, #36887, .T. ) ;
#48202=DIRECTION ( 'NONE',  ( 1.000000000000000000, 0.000000000000000000, 0.000000000000000000 ) ) ;
#48205=DIRECTION ( 'NONE',  ( -0.000000000000000000, -0.000000000000000000, -1.000000000000000000 ) ) ;
#48209=EDGE_CURVE ( 'NONE', #3036, #6695, #64695, .T. ) ;
#48210=ORIENTED_EDGE ( 'NONE', *, *, #46902, .T. ) ;
#48211=AXIS2_PLACEMENT_3D ( 'NONE', #4555, #13831, #8535 ) ;
#48212=CARTESIAN_POINT ( 'NONE',  ( 37.00000000000000711, -9.063649021438894948, 8.146229107149494553 ) ) ;
#48216=DIRECTION ( 'NONE',  ( 1.000000000000000000, 0.000000000000000000, 0.000000000000000000 ) ) ;
#48218=AXIS2_PLACEMENT_3D ( 'NONE', #36646, #35964, #20704 ) ;
#48219=DIRECTION ( 'NONE',  ( 1.000000000000000000, 0.000000000000000000, 0.000000000000000000 ) ) ;
#48220=DIRECTION ( 'NONE',  ( 0.000000000000000000, 0.01356324068817992522, -0.9999080150203990547 ) ) ;
#48222=EDGE_CURVE ( 'NONE', #37848, #27274, #42376, .T. ) ;
#48223=CARTESIAN_POINT ( 'NONE',  ( -27.45775109278351067, -10.51123867646838050, -8.471355351200609007 ) ) ;
#48224=VECTOR ( 'NONE', #15428, 1000.000000000000000 ) ;
#48225=ORIENTED_EDGE ( 'NONE', *, *, #57490, .F. ) ;
#48226=DIRECTION ( 'NONE',  ( 0.000000000000000000, 0.01356324068817992175, -0.9999080150203990547 ) ) ;
#48230=AXIS2_PLACEMENT_3D ( 'NONE', #39755, #60355, #24135 ) ;
#48231=CARTESIAN_POINT ( 'NONE',  ( 35.00000000000000000, 4.705694406421931860E-17, -3.469127814946512892E-15 ) ) ;
#48234=ADVANCED_FACE ( 'NONE', ( #24940 ), #656, .F. ) ;
#48237=CARTESIAN_POINT ( 'NONE',  ( 22.57855258442564761, -4.427776684447072952, 12.75322679295976691 ) ) ;
#48247=AXIS2_PLACEMENT_3D ( 'NONE', #698, #55892, #8447 ) ;
#48250=CIRCLE ( 'NONE', #28059, 12.18650000000000055 ) ;
#48251=ORIENTED_EDGE ( 'NONE', *, *, #23159, .F. ) ;
#48252=CARTESIAN_POINT ( 'NONE',  ( 8.937200413559445167, 4.820175079577382782, -10.99560042399104098 ) ) ;
#48253=EDGE_CURVE ( 'NONE', #39576, #52203, #52825, .T. ) ;
#48254=EDGE_LOOP ( 'NONE', ( #4238, #61381 ) ) ;
#48255=CARTESIAN_POINT ( 'NONE',  ( 26.25882823526612597, -13.04980996862088638, 3.460358416528618530 ) ) ;
#48256=CARTESIAN_POINT ( 'NONE',  ( 35.00000000000000000, 4.705694406421931860E-17, -3.469127814946512892E-15 ) ) ;
#48257=VECTOR ( 'NONE', #25805, 1000.000000000000000 ) ;
#48260=EDGE_CURVE ( 'NONE', #55068, #11977, #977, .T. ) ;
#48262=VERTEX_POINT ( 'NONE', #16599 ) ;
#48263=AXIS2_PLACEMENT_3D ( 'NONE', #17770, #38361, #44022 ) ;
#48264=ORIENTED_EDGE ( 'NONE', *, *, #21455, .F. ) ;
#48265=ORIENTED_EDGE ( 'NONE', *, *, #14745, .F. ) ;
#48267=VECTOR ( 'NONE', #16784, 1000.000000000000000 ) ;
#48269=DIRECTION ( 'NONE',  ( 1.000000000000000000, 0.000000000000000000, 0.000000000000000000 ) ) ;
#48271=VERTEX_POINT ( 'NONE', #52520 ) ;
#48273=AXIS2_PLACEMENT_3D ( 'NONE', #36613, #47269, #11341 ) ;
#48274=CARTESIAN_POINT ( 'NONE',  ( -37.00000000000000711, 4.732539170486427693, -11.23004253107759176 ) ) ;
#48275=CARTESIAN_POINT ( 'NONE',  ( 35.00000000000000000, 6.102719229070673990, -10.54834585426222304 ) ) ;
#48276=EDGE_LOOP ( 'NONE', ( #7424, #29667, #10670, #11287 ) ) ;
#48277=ORIENTED_EDGE ( 'NONE', *, *, #26494, .F. ) ;
#48278=DIRECTION ( 'NONE',  ( 0.000000000000000000, -0.01356324068817999114, 0.9999080150203989437 ) ) ;
#48286=CARTESIAN_POINT ( 'NONE',  ( 35.00000000000000000, -1.791059740004336875, 12.05416472667166694 ) ) ;
#48289=CARTESIAN_POINT ( 'NONE',  ( -27.47719885066990742, -11.55823979936119450, -3.277255182065942574 ) ) ;
#48290=ORIENTED_EDGE ( 'NONE', *, *, #4045, .F. ) ;
#48293=VERTEX_POINT ( 'NONE', #56856 ) ;
#48294=PLANE ( 'NONE',  #4114 ) ;
#48295=CARTESIAN_POINT ( 'NONE',  ( -35.00000000000000000, 11.65554240571059275, -1.456211999474221086 ) ) ;
#48296=EDGE_LOOP ( 'NONE', ( #2125, #3511, #51229, #24143 ) ) ;
#48302=VERTEX_POINT ( 'NONE', #1647 ) ;
#48305=FACE_OUTER_BOUND ( 'NONE', #39638, .T. ) ;
#48306=CARTESIAN_POINT ( 'NONE',  ( 35.00000000000000000, -11.68758509253247091, 1.171570255487570655 ) ) ;
#48309=CARTESIAN_POINT ( 'NONE',  ( -17.83799997667700055, -8.694692931027089955, 8.293044525567449199 ) ) ;
#48310=ADVANCED_FACE ( 'NONE', ( #21916 ), #47837, .T. ) ;
#48311=ORIENTED_EDGE ( 'NONE', *, *, #50128, .T. ) ;
#48312=DIRECTION ( 'NONE',  ( 1.000000000000000000, 0.000000000000000000, -0.000000000000000000 ) ) ;
#48313=EDGE_CURVE ( 'NONE', #34842, #15906, #37855, .T. ) ;
#48314=CIRCLE ( 'NONE', #19626, 12.18649999999999878 ) ;
#48316=CARTESIAN_POINT ( 'NONE',  ( 22.22325956648730383, 13.44453809516076248, -1.271158126962866897 ) ) ;
#48318=DIRECTION ( 'NONE',  ( 1.000000000000000000, 0.000000000000000000, 0.000000000000000000 ) ) ;
#48324=ORIENTED_EDGE ( 'NONE', *, *, #14834, .F. ) ;
#48328=ORIENTED_EDGE ( 'NONE', *, *, #15262, .T. ) ;
#48330=ORIENTED_EDGE ( 'NONE', *, *, #65790, .F. ) ;
#48333=EDGE_LOOP ( 'NONE', ( #45895, #15738, #51427, #49258 ) ) ;
#48335=CARTESIAN_POINT ( 'NONE',  ( -10.71044032080790309, -9.069509059426344777, -7.875876655957959827 ) ) ;
#48336=ADVANCED_FACE ( 'NONE', ( #57241 ), #11668, .T. ) ;
#48338=ORIENTED_EDGE ( 'NONE', *, *, #31160, .T. ) ;
#48340=CARTESIAN_POINT ( 'NONE',  ( 3.128546914509915844, 2.910026699185261467, 13.18839757576990479 ) ) ;
#48341=DIRECTION ( 'NONE',  ( 1.000000000000000000, 0.000000000000000000, -0.000000000000000000 ) ) ;
#48342=CARTESIAN_POINT ( 'NONE',  ( -35.00000000000000000, 0.000000000000000000, 0.000000000000000000 ) ) ;
#48344=CIRCLE ( 'NONE', #19665, 12.18649999999999878 ) ;
#48348=CYLINDRICAL_SURFACE ( 'NONE', #60564, 12.74999999999999822 ) ;
#48349=ORIENTED_EDGE ( 'NONE', *, *, #65732, .T. ) ;
#48352=DIRECTION ( 'NONE',  ( -1.000000000000000000, 0.000000000000000000, 0.000000000000000000 ) ) ;
#48353=ORIENTED_EDGE ( 'NONE', *, *, #26868, .T. ) ;
#48357=CYLINDRICAL_SURFACE ( 'NONE', #4309, 12.75000000000000178 ) ;
#48358=CARTESIAN_POINT ( 'NONE',  ( -2.532614230583022152, 11.30437021680556242, 4.026315189028233377 ) ) ;
#48362=ADVANCED_FACE ( 'NONE', ( #16989 ), #37267, .T. ) ;
#48363=VERTEX_POINT ( 'NONE', #52895 ) ;
#48365=VERTEX_POINT ( 'NONE', #58907 ) ;
#48367=ORIENTED_EDGE ( 'NONE', *, *, #23363, .T. ) ;
#48369=DIRECTION ( 'NONE',  ( 0.000000000000000000, -1.000000000000000000, 0.000000000000000000 ) ) ;
#48370=CARTESIAN_POINT ( 'NONE',  ( -37.00000000000000711, -12.02534193257724304, 4.237174932027182095 ) ) ;
#48373=LINE ( 'NONE', #13101, #15058 ) ;
#48374=CIRCLE ( 'NONE', #19687, 12.18650000000000411 ) ;
#48375=EDGE_CURVE ( 'NONE', #13554, #32930, #54217, .T. ) ;
#48376=CARTESIAN_POINT ( 'NONE',  ( -37.00000000000000711, -9.752226076388847531, -6.547236723514122225 ) ) ;
#48380=DIRECTION ( 'NONE',  ( 1.000000000000000000, 0.000000000000000000, 0.000000000000000000 ) ) ;
#48381=DIRECTION ( 'NONE',  ( 0.000000000000000000, -0.01356324068818000848, 0.9999080150203990547 ) ) ;
#48382=EDGE_CURVE ( 'NONE', #8260, #10101, #35524, .T. ) ;
#48385=DIRECTION ( 'NONE',  ( 0.000000000000000000, -0.4935949184179136418, 0.8696919319575254770 ) ) ;
#48386=AXIS2_PLACEMENT_3D ( 'NONE', #5354, #35904, #41899 ) ;
#48388=DIRECTION ( 'NONE',  ( 0.000000000000000000, -0.01356324068817991307, 0.9999080150203990547 ) ) ;
#48390=ORIENTED_EDGE ( 'NONE', *, *, #14629, .F. ) ;
#48392=FACE_OUTER_BOUND ( 'NONE', #11225, .T. ) ;
#48394=CARTESIAN_POINT ( 'NONE',  ( 35.00000000000000000, 4.705694406421931860E-17, -3.469127814946512892E-15 ) ) ;
#48396=VERTEX_POINT ( 'NONE', #64191 ) ;
#48397=CARTESIAN_POINT ( 'NONE',  ( 19.28625800530496903, -1.699513388191772778, 11.87904264843580471 ) ) ;
#48399=ORIENTED_EDGE ( 'NONE', *, *, #7271, .T. ) ;
#48403=ORIENTED_EDGE ( 'NONE', *, *, #61102, .T. ) ;
#48407=CYLINDRICAL_SURFACE ( 'NONE', #60987, 4.999999999999999112 ) ;
#48408=CARTESIAN_POINT ( 'NONE',  ( 35.00000000000000000, -10.84030624090611106, -6.711949091238110121 ) ) ;
#48411=CARTESIAN_POINT ( 'NONE',  ( 35.00000000000000000, 4.705694406421931860E-17, -3.469127814946512892E-15 ) ) ;
#48412=DIRECTION ( 'NONE',  ( 0.000000000000000000, 0.7617968321374855023, 0.6478160128811972784 ) ) ;
#48415=CARTESIAN_POINT ( 'NONE',  ( 37.00000000000000711, 8.927548052240892318, -8.295159312811890118 ) ) ;
#48416=VERTEX_POINT ( 'NONE', #42564 ) ;
#48418=VERTEX_POINT ( 'NONE', #48274 ) ;
#48420=ORIENTED_EDGE ( 'NONE', *, *, #49712, .F. ) ;
#48422=CARTESIAN_POINT ( 'NONE',  ( -25.01550185040246532, 11.25207016924878367, 7.460967861423081438 ) ) ;
#48424=DIRECTION ( 'NONE',  ( 0.4622435816439406930, 0.000000000000000000, -0.8867529933577791290 ) ) ;
#48426=DIRECTION ( 'NONE',  ( -1.000000000000000000, 0.000000000000000000, 0.000000000000000000 ) ) ;
#48427=CIRCLE ( 'NONE', #24014, 5.000000000000000888 ) ;
#48428=DIRECTION ( 'NONE',  ( 0.000000000000000000, 0.9105187689795940509, -0.4134677391718546424 ) ) ;
#48429=ORIENTED_EDGE ( 'NONE', *, *, #20601, .T. ) ;
#48432=ADVANCED_FACE ( 'NONE', ( #22981 ), #62867, .T. ) ;
#48435=VERTEX_POINT ( 'NONE', #43233 ) ;
#48436=DIRECTION ( 'NONE',  ( 0.000000000000000000, -0.01356324068817998940, 0.9999080150203990547 ) ) ;
#48438=EDGE_LOOP ( 'NONE', ( #31843, #17400, #38976, #22883 ) ) ;
#48439=CARTESIAN_POINT ( 'NONE',  ( 29.19808783025697707, -7.805332973316843059, 11.01506521398892069 ) ) ;
#48441=DIRECTION ( 'NONE',  ( 1.000000000000000000, 0.000000000000000000, 0.000000000000000000 ) ) ;
#48442=AXIS2_PLACEMENT_3D ( 'NONE', #42327, #42021, #1809 ) ;
#48443=CARTESIAN_POINT ( 'NONE',  ( 37.00000000000000711, -7.817610399097575602, -8.766823244861962294 ) ) ;
#48445=CARTESIAN_POINT ( 'NONE',  ( -29.68541646480307250, -1.416020129149132334, 13.42553116244733680 ) ) ;
#48446=EDGE_CURVE ( 'NONE', #13869, #21040, #5256, .T. ) ;
#48447=CARTESIAN_POINT ( 'NONE',  ( 36.00000000000000711, 9.196955404009292678, -8.830544224262981245 ) ) ;
#48448=ORIENTED_EDGE ( 'NONE', *, *, #34116, .T. ) ;
#48450=EDGE_CURVE ( 'NONE', #53140, #37516, #3033, .T. ) ;
#48451=ORIENTED_EDGE ( 'NONE', *, *, #46756, .T. ) ;
#48454=CARTESIAN_POINT ( 'NONE',  ( -37.00000000000000711, -1.738225594539907659, -12.63095688309031139 ) ) ;
#48455=ORIENTED_EDGE ( 'NONE', *, *, #37814, .T. ) ;
#48456=FACE_OUTER_BOUND ( 'NONE', #10509, .T. ) ;
#48458=ORIENTED_EDGE ( 'NONE', *, *, #24661, .T. ) ;
#48464=VERTEX_POINT ( 'NONE', #43908 ) ;
#48467=CARTESIAN_POINT ( 'NONE',  ( 35.00000000000000000, 4.705694406421931860E-17, -3.469127814946512892E-15 ) ) ;
#48471=ORIENTED_EDGE ( 'NONE', *, *, #10221, .T. ) ;
#48472=CYLINDRICAL_SURFACE ( 'NONE', #2588, 4.999999999999999112 ) ;
#48473=LINE ( 'NONE', #17873, #1025 ) ;
#48475=CARTESIAN_POINT ( 'NONE',  ( -9.522095209522213111, -2.893068788992850138, -13.18738133420595027 ) ) ;
#48477=CARTESIAN_POINT ( 'NONE',  ( -35.00000000000000000, -5.927257550915394191, 10.64792938439753378 ) ) ;
#48480=EDGE_CURVE ( 'NONE', #3315, #52686, #60539, .T. ) ;
#48482=CARTESIAN_POINT ( 'NONE',  ( 35.00000000000000000, -3.307597835713330880, -12.31350058095522115 ) ) ;
#48483=VERTEX_POINT ( 'NONE', #24272 ) ;
#48488=DIRECTION ( 'NONE',  ( 0.000000000000000000, 0.9970832820307036215, 0.07632122047556837152 ) ) ;
#48491=ORIENTED_EDGE ( 'NONE', *, *, #19638, .F. ) ;
#48492=VERTEX_POINT ( 'NONE', #3706 ) ;
#48493=EDGE_CURVE ( 'NONE', #53238, #22366, #5301, .T. ) ;
#48495=ORIENTED_EDGE ( 'NONE', *, *, #10821, .T. ) ;
#48496=PRESENTATION_STYLE_ASSIGNMENT (( #18231 ) ) ;
#48501=ORIENTED_EDGE ( 'NONE', *, *, #19984, .F. ) ;
#48502=DIRECTION ( 'NONE',  ( 1.000000000000000000, 0.000000000000000000, 0.000000000000000000 ) ) ;
#48503=CARTESIAN_POINT ( 'NONE',  ( 37.00000000000000711, 9.493370459201798894, 6.917234959366719060 ) ) ;
#48505=VERTEX_POINT ( 'NONE', #18968 ) ;
#48506=ORIENTED_EDGE ( 'NONE', *, *, #3698, .F. ) ;
#48507=CARTESIAN_POINT ( 'NONE',  ( 35.00000000000000000, 4.705694406421931860E-17, -3.469127814946512892E-15 ) ) ;
#48508=EDGE_CURVE ( 'NONE', #31872, #23983, #39272, .T. ) ;
#48509=EDGE_LOOP ( 'NONE', ( #33745, #32487, #56933, #28000 ) ) ;
#48510=FACE_OUTER_BOUND ( 'NONE', #58603, .T. ) ;
#48511=ORIENTED_EDGE ( 'NONE', *, *, #22499, .T. ) ;
#48515=CARTESIAN_POINT ( 'NONE',  ( 35.00000000000000000, 6.036400161834703404, 10.07641281632170838 ) ) ;
#48517=CARTESIAN_POINT ( 'NONE',  ( -47.00000000000000711, 0.000000000000000000, 0.000000000000000000 ) ) ;
#48519=AXIS2_PLACEMENT_3D ( 'NONE', #44362, #60321, #51014 ) ;
#48521=ORIENTED_EDGE ( 'NONE', *, *, #3057, .F. ) ;
#48524=DIRECTION ( 'NONE',  ( 0.000000000000000000, -0.01356324068817999114, 0.9999080150203989437 ) ) ;
#48526=EDGE_CURVE ( 'NONE', #1474, #26254, #27590, .T. ) ;
#48529=DIRECTION ( 'NONE',  ( -1.000000000000000000, 0.000000000000000000, 0.000000000000000000 ) ) ;
#48534=VERTEX_POINT ( 'NONE', #23966 ) ;
#48536=EDGE_CURVE ( 'NONE', #2417, #57976, #64817, .T. ) ;
#48537=EDGE_CURVE ( 'NONE', #45277, #57124, #26552, .T. ) ;
#48538=ORIENTED_EDGE ( 'NONE', *, *, #13804, .F. ) ;
#48539=DIRECTION ( 'NONE',  ( 0.000000000000000000, 0.9551603052523490733, -0.2960891610144476549 ) ) ;
#48545=ORIENTED_EDGE ( 'NONE', *, *, #59614, .T. ) ;
#48547=CARTESIAN_POINT ( 'NONE',  ( -35.00000000000000000, 0.000000000000000000, 0.000000000000000000 ) ) ;
#48548=CARTESIAN_POINT ( 'NONE',  ( -18.55833381744858457, -13.45545930202708007, 1.279848689959048658 ) ) ;
#48553=EDGE_LOOP ( 'NONE', ( #53756, #48738, #3841, #6942 ) ) ;
#48559=ORIENTED_EDGE ( 'NONE', *, *, #42991, .F. ) ;
#48560=VECTOR ( 'NONE', #38238, 1000.000000000000000 ) ;
#48562=CARTESIAN_POINT ( 'NONE',  ( -37.00000000000000711, -10.02106554660702820, -7.882940143791884680 ) ) ;
#48566=DIRECTION ( 'NONE',  ( 1.000000000000000000, 0.000000000000000000, 0.000000000000000000 ) ) ;
#48569=DIRECTION ( 'NONE',  ( 1.000000000000000000, 0.000000000000000000, 0.000000000000000000 ) ) ;
#48570=ORIENTED_EDGE ( 'NONE', *, *, #38187, .F. ) ;
#48571=EDGE_CURVE ( 'NONE', #36007, #29813, #55228, .T. ) ;
#48572=EDGE_LOOP ( 'NONE', ( #46759, #47199, #1870, #4758 ) ) ;
#48573=ORIENTED_EDGE ( 'NONE', *, *, #8955, .F. ) ;
#48575=CARTESIAN_POINT ( 'NONE',  ( 37.00000000000000711, -11.65554240571056077, 1.456211999474460672 ) ) ;
#48577=CYLINDRICAL_SURFACE ( 'NONE', #12407, 5.000000000000002665 ) ;
#48579=ORIENTED_EDGE ( 'NONE', *, *, #10380, .T. ) ;
#48581=DIRECTION ( 'NONE',  ( 1.000000000000000000, -0.000000000000000000, 0.000000000000000000 ) ) ;
#48582=DIRECTION ( 'NONE',  ( 1.000000000000000000, -0.000000000000000000, 0.000000000000000000 ) ) ;
#48583=VERTEX_POINT ( 'NONE', #4679 ) ;
#48584=ORIENTED_EDGE ( 'NONE', *, *, #54316, .F. ) ;
#48586=EDGE_CURVE ( 'NONE', #26931, #10291, #51667, .T. ) ;
#48588=CARTESIAN_POINT ( 'NONE',  ( -18.78798712546867122, 11.98387424500765697, -0.7129084681429045389 ) ) ;
#48589=ORIENTED_EDGE ( 'NONE', *, *, #50382, .F. ) ;
#48591=ADVANCED_FACE ( 'NONE', ( #50221 ), #19939, .T. ) ;
#48592=CARTESIAN_POINT ( 'NONE',  ( -37.00000000000000711, -8.017674001891851532, 9.913596905230088296 ) ) ;
#48594=MECHANICAL_DESIGN_GEOMETRIC_PRESENTATION_REPRESENTATION('',(#22176),#31574);
#48595=CYLINDRICAL_SURFACE ( 'NONE', #1712, 12.75000000000000178 ) ;
#48597=DIRECTION ( 'NONE',  ( -1.000000000000000000, -0.000000000000000000, 0.000000000000000000 ) ) ;
#48598=ORIENTED_EDGE ( 'NONE', *, *, #55672, .F. ) ;
#48599=DIRECTION ( 'NONE',  ( 1.000000000000000000, -0.000000000000000000, -0.000000000000000000 ) ) ;
#48600=EDGE_LOOP ( 'NONE', ( #49806, #64363, #10196, #44851 ) ) ;
#48607=AXIS2_PLACEMENT_3D ( 'NONE', #260, #40133, #45457 ) ;
#48609=ORIENTED_EDGE ( 'NONE', *, *, #64741, .F. ) ;
#48613=EDGE_CURVE ( 'NONE', #14694, #39894, #15915, .T. ) ;
#48614=EDGE_LOOP ( 'NONE', ( #5246, #60356, #26808, #45254 ) ) ;
#48615=CARTESIAN_POINT ( 'NONE',  ( -28.56462394502009516, 3.589878760083821341, 13.01421318288084450 ) ) ;
#48616=CARTESIAN_POINT ( 'NONE',  ( 37.00000000000000711, 6.475373545682446164, 10.32377448871660519 ) ) ;
#48617=DIRECTION ( 'NONE',  ( 0.000000000000000000, 0.2355298848897516562, 0.9718671068226458765 ) ) ;
#48619=CARTESIAN_POINT ( 'NONE',  ( -2.532614230583022152, 11.30437021680556242, 4.026315189028233377 ) ) ;
#48620=FACE_OUTER_BOUND ( 'NONE', #5346, .T. ) ;
#48621=ORIENTED_EDGE ( 'NONE', *, *, #55390, .T. ) ;
#48623=EDGE_CURVE ( 'NONE', #6133, #11272, #15596, .T. ) ;
#48625=CARTESIAN_POINT ( 'NONE',  ( -35.00000000000000000, -11.26103545359858060, 3.340853584269496412 ) ) ;
#48626=DIRECTION ( 'NONE',  ( 0.000000000000000000, 0.01356324068817998940, -0.9999080150203989437 ) ) ;
#48628=CARTESIAN_POINT ( 'NONE',  ( 7.006432388548472723, -4.543361190407962269, -11.11502132045045066 ) ) ;
#48630=VECTOR ( 'NONE', #9623, 1000.000000000000000 ) ;
#48632=CARTESIAN_POINT ( 'NONE',  ( 11.74548640120467979, -8.775604215601116920, -8.184666801472349817 ) ) ;
#48633=EDGE_CURVE ( 'NONE', #7338, #15890, #31855, .T. ) ;
#48634=CIRCLE ( 'NONE', #29477, 12.75000000000000178 ) ;
#48635=ORIENTED_EDGE ( 'NONE', *, *, #61486, .F. ) ;
#48638=DIRECTION ( 'NONE',  ( 1.000000000000000000, 0.000000000000000000, 0.000000000000000000 ) ) ;
#48639=ORIENTED_EDGE ( 'NONE', *, *, #59193, .F. ) ;
#48640=VECTOR ( 'NONE', #33693, 1000.000000000000000 ) ;
#48642=DIRECTION ( 'NONE',  ( -1.000000000000000000, 0.000000000000000000, 0.000000000000000000 ) ) ;
#48644=ADVANCED_FACE ( 'NONE', ( #25926 ), #20609, .T. ) ;
#48646=AXIS2_PLACEMENT_3D ( 'NONE', #55952, #20050, #34357 ) ;
#48648=CARTESIAN_POINT ( 'NONE',  ( 29.04793922789648875, -11.92654474506188222, 6.328478715807100308 ) ) ;
#48650=VERTEX_POINT ( 'NONE', #21917 ) ;
#48651=CARTESIAN_POINT ( 'NONE',  ( 37.00000000000000711, -6.415447294506781084, -11.01837265713071368 ) ) ;
#48653=FACE_OUTER_BOUND ( 'NONE', #36783, .T. ) ;
#48654=CARTESIAN_POINT ( 'NONE',  ( 17.27839441901508621, 10.52068335315811076, 5.771933972472480967 ) ) ;
#48656=DIRECTION ( 'NONE',  ( 0.000000000000000000, -0.01356324068817998940, 0.9999080150203990547 ) ) ;
#48657=CARTESIAN_POINT ( 'NONE',  ( -37.00000000000000711, -2.185196060783795691, -11.54110654723651486 ) ) ;
#48658=CARTESIAN_POINT ( 'NONE',  ( -29.43980975494970309, -3.641506875706030488, 11.43413432115373318 ) ) ;
#48660=ORIENTED_EDGE ( 'NONE', *, *, #23182, .T. ) ;
#48663=EDGE_CURVE ( 'NONE', #21056, #266, #56267, .T. ) ;
#48664=VERTEX_POINT ( 'NONE', #35860 ) ;
#48666=ORIENTED_EDGE ( 'NONE', *, *, #38757, .F. ) ;
#48667=CARTESIAN_POINT ( 'NONE',  ( -37.00000000000000711, 0.000000000000000000, 0.000000000000000000 ) ) ;
#48668=CYLINDRICAL_SURFACE ( 'NONE', #50055, 12.18650000000000055 ) ;
#48670=DIRECTION ( 'NONE',  ( 0.000000000000000000, 0.01356324068817998940, -0.9999080150203990547 ) ) ;
#48671=CARTESIAN_POINT ( 'NONE',  ( 35.00000000000000000, 0.1652884326465054732, -12.18537902504609427 ) ) ;
#48673=CARTESIAN_POINT ( 'NONE',  ( 37.00000000000000711, -9.506317355798431734, -8.496612874013129257 ) ) ;
#48675=ORIENTED_EDGE ( 'NONE', *, *, #19577, .T. ) ;
#48678=ORIENTED_EDGE ( 'NONE', *, *, #55402, .T. ) ;
#48679=VERTEX_POINT ( 'NONE', #36551 ) ;
#48682=CYLINDRICAL_SURFACE ( 'NONE', #41518, 4.999999999999999112 ) ;
#48685=EDGE_CURVE ( 'NONE', #10035, #1393, #25584, .T. ) ;
#48689=EDGE_CURVE ( 'NONE', #12619, #46217, #46853, .T. ) ;
#48690=CIRCLE ( 'NONE', #9340, 5.000000000000000888 ) ;
#48691=AXIS2_PLACEMENT_3D ( 'NONE', #43390, #33744, #13153 ) ;
#48693=DIRECTION ( 'NONE',  ( 1.000000000000000000, 0.000000000000000000, 0.000000000000000000 ) ) ;
#48694=CARTESIAN_POINT ( 'NONE',  ( -35.00000000000000000, 4.561791185930587744, -11.90598845858528776 ) ) ;
#48695=VECTOR ( 'NONE', #14310, 1000.000000000000000 ) ;
#48696=DIRECTION ( 'NONE',  ( 1.000000000000000000, 0.000000000000000000, -0.000000000000000000 ) ) ;
#48697=VECTOR ( 'NONE', #31493, 1000.000000000000000 ) ;
#48698=DIRECTION ( 'NONE',  ( 1.000000000000000000, 0.000000000000000000, 0.000000000000000000 ) ) ;
#48700=CARTESIAN_POINT ( 'NONE',  ( -5.434547206004880060, -0.9285584038156732278, 13.46803372541172195 ) ) ;
#48701=CARTESIAN_POINT ( 'NONE',  ( 8.937200413559443390, 4.476360154859203355, -11.13383131558893346 ) ) ;
#48702=ORIENTED_EDGE ( 'NONE', *, *, #21794, .F. ) ;
#48704=CARTESIAN_POINT ( 'NONE',  ( -35.00000000000000000, 0.7214809346828596759, 11.72397916322012712 ) ) ;
#48707=AXIS2_PLACEMENT_3D ( 'NONE', #2989, #38879, #48539 ) ;
#48708=CYLINDRICAL_SURFACE ( 'NONE', #41617, 12.18649999999999878 ) ;
#48709=DIRECTION ( 'NONE',  ( 0.000000000000000000, 0.9987865678893277366, -0.04924826701374931254 ) ) ;
#48711=EDGE_LOOP ( 'NONE', ( #6163, #49808, #56834, #43950 ) ) ;
#48714=DIRECTION ( 'NONE',  ( -1.000000000000000000, 0.000000000000000000, -0.000000000000000000 ) ) ;
#48715=ORIENTED_EDGE ( 'NONE', *, *, #27876, .T. ) ;
#48716=CARTESIAN_POINT ( 'NONE',  ( 35.00000000000000000, -3.645068577059948911, 11.16627499335658413 ) ) ;
#48719=EDGE_LOOP ( 'NONE', ( #48675, #59304, #49876, #50685 ) ) ;
#48721=CIRCLE ( 'NONE', #21076, 12.18649999999999878 ) ;
#48722=EDGE_CURVE ( 'NONE', #56593, #58586, #24409, .T. ) ;
#48723=ORIENTED_EDGE ( 'NONE', *, *, #25753, .F. ) ;
#48724=CYLINDRICAL_SURFACE ( 'NONE', #38719, 12.18649999999999878 ) ;
#48725=CARTESIAN_POINT ( 'NONE',  ( -37.00000000000000711, -7.094637218249278732, -10.59380114696477904 ) ) ;
#48726=VECTOR ( 'NONE', #18198, 1000.000000000000000 ) ;
#48727=CARTESIAN_POINT ( 'NONE',  ( -35.00000000000000000, 8.029056188533687077, 8.573591947375351907 ) ) ;
#48728=CIRCLE ( 'NONE', #13526, 5.000000000000000000 ) ;
#48732=ORIENTED_EDGE ( 'NONE', *, *, #30358, .F. ) ;
#48734=DIRECTION ( 'NONE',  ( 0.000000000000000000, -0.01356324068817998073, 0.9999080150203990547 ) ) ;
#48735=EDGE_CURVE ( 'NONE', #41230, #33435, #15905, .T. ) ;
#48736=ORIENTED_EDGE ( 'NONE', *, *, #17613, .T. ) ;
#48737=DIRECTION ( 'NONE',  ( 0.000000000000000000, -0.01356324068817991828, 0.9999080150203990547 ) ) ;
#48738=ORIENTED_EDGE ( 'NONE', *, *, #18415, .F. ) ;
#48739=AXIS2_PLACEMENT_3D ( 'NONE', #51059, #5517, #31093 ) ;
#48740=ORIENTED_EDGE ( 'NONE', *, *, #2815, .F. ) ;
#48741=CARTESIAN_POINT ( 'NONE',  ( -24.88582978492754805, 10.97013053255485104, 7.869802505931382086 ) ) ;
#48743=CARTESIAN_POINT ( 'NONE',  ( -4.020556197261224263, 8.897818130997190877, 8.054759335216724381 ) ) ;
#48748=ORIENTED_EDGE ( 'NONE', *, *, #36354, .F. ) ;
#48750=CARTESIAN_POINT ( 'NONE',  ( -35.00000000000000000, 9.321877890560440250, 7.146664589317944127 ) ) ;
#48752=FACE_OUTER_BOUND ( 'NONE', #47571, .T. ) ;
#48754=CARTESIAN_POINT ( 'NONE',  ( 37.00000000000000711, 0.4993900848169179896, 12.17626345777662777 ) ) ;
#48755=ORIENTED_EDGE ( 'NONE', *, *, #64683, .F. ) ;
#48759=DIRECTION ( 'NONE',  ( -1.000000000000000000, 0.000000000000000000, 0.000000000000000000 ) ) ;
#48760=CYLINDRICAL_SURFACE ( 'NONE', #41591, 12.75000000000000178 ) ;
#48762=CIRCLE ( 'NONE', #64669, 12.18650000000000055 ) ;
#48763=CARTESIAN_POINT ( 'NONE',  ( 36.00000000000000711, -1.738225594540087293, -12.63095688309028652 ) ) ;
#48764=VERTEX_POINT ( 'NONE', #1648 ) ;
#48766=CIRCLE ( 'NONE', #57259, 12.18650000000000055 ) ;
#48767=VERTEX_POINT ( 'NONE', #17255 ) ;
#48769=EDGE_CURVE ( 'NONE', #57005, #61089, #22573, .T. ) ;
#48770=FACE_OUTER_BOUND ( 'NONE', #4098, .T. ) ;
#48771=CARTESIAN_POINT ( 'NONE',  ( 35.00000000000000000, -12.14284015767850455, -1.030638227056526413 ) ) ;
#48772=CIRCLE ( 'NONE', #20087, 12.75000000000000178 ) ;
#48775=LINE ( 'NONE', #28803, #21708 ) ;
#48776=DIRECTION ( 'NONE',  ( -1.000000000000000000, 0.000000000000000000, 0.000000000000000000 ) ) ;
#48777=CIRCLE ( 'NONE', #6296, 5.000000000000000000 ) ;
#48780=DIRECTION ( 'NONE',  ( 0.000000000000000000, 0.5987040770935622147, -0.8009703041134208501 ) ) ;
#48781=CARTESIAN_POINT ( 'NONE',  ( -35.00000000000000000, 5.921969905510501064, -10.14408668126206869 ) ) ;
#48782=CARTESIAN_POINT ( 'NONE',  ( 0.2851083653049504285, -0.4107471485392698018, 25.00000000000000000 ) ) ;
#48783=ORIENTED_EDGE ( 'NONE', *, *, #20797, .T. ) ;
#48787=AXIS2_PLACEMENT_3D ( 'NONE', #56630, #51966, #22019 ) ;
#48788=DIRECTION ( 'NONE',  ( -1.000000000000000000, 0.000000000000000000, 0.000000000000000000 ) ) ;
#48789=EDGE_CURVE ( 'NONE', #38911, #5091, #38507, .T. ) ;
#48794=EDGE_CURVE ( 'NONE', #35378, #853, #32896, .T. ) ;
#48795=CARTESIAN_POINT ( 'NONE',  ( -20.55448987689497997, -11.44131724608703493, -3.631843722756310733 ) ) ;
#48796=CARTESIAN_POINT ( 'NONE',  ( 35.00000000000000000, 4.705694406421931860E-17, -3.469127814946512892E-15 ) ) ;
#48798=ORIENTED_EDGE ( 'NONE', *, *, #54223, .F. ) ;
#48801=DIRECTION ( 'NONE',  ( 0.000000000000000000, 0.6745969609292664648, 0.7381862504171951000 ) ) ;
#48802=CARTESIAN_POINT ( 'NONE',  ( 37.00000000000000711, 4.705694406421931860E-17, -3.469127814946512892E-15 ) ) ;
#48803=CARTESIAN_POINT ( 'NONE',  ( 47.00000000000000711, 4.705694406421931860E-17, -3.469127814946512892E-15 ) ) ;
#48805=AXIS2_PLACEMENT_3D ( 'NONE', #26202, #6254, #19897 ) ;
#48807=DIRECTION ( 'NONE',  ( 1.000000000000000000, 0.000000000000000000, 0.000000000000000000 ) ) ;
#48808=VERTEX_POINT ( 'NONE', #27885 ) ;
#48812=CARTESIAN_POINT ( 'NONE',  ( 37.00000000000000711, 4.705694406421931860E-17, -3.469127814946512892E-15 ) ) ;
#48815=LINE ( 'NONE', #2938, #4521 ) ;
#48817=DIRECTION ( 'NONE',  ( 1.000000000000000000, 0.000000000000000000, 0.000000000000000000 ) ) ;
#48818=DIRECTION ( 'NONE',  ( -1.000000000000000000, -0.000000000000000000, 0.000000000000000000 ) ) ;
#48819=EDGE_LOOP ( 'NONE', ( #55617, #34462, #15380, #23210 ) ) ;
#48820=ORIENTED_EDGE ( 'NONE', *, *, #29146, .T. ) ;
#48821=CARTESIAN_POINT ( 'NONE',  ( -37.00000000000000711, 10.99909370905157502, 5.246972444134057945 ) ) ;
#48822=ORIENTED_EDGE ( 'NONE', *, *, #41127, .F. ) ;
#48824=AXIS2_PLACEMENT_3D ( 'NONE', #42377, #33976, #47416 ) ;
#48826=EDGE_CURVE ( 'NONE', #31052, #15913, #11647, .T. ) ;
#48827=DIRECTION ( 'NONE',  ( 0.000000000000000000, -0.01356324068817998940, 0.9999080150203990547 ) ) ;
#48828=CIRCLE ( 'NONE', #18016, 12.18649999999999700 ) ;
#48833=ORIENTED_EDGE ( 'NONE', *, *, #55495, .F. ) ;
#48837=CARTESIAN_POINT ( 'NONE',  ( 35.00000000000000000, 0.06441628369836321921, -12.18632975068353019 ) ) ;
#48838=VERTEX_POINT ( 'NONE', #43481 ) ;
#48839=AXIS2_PLACEMENT_3D ( 'NONE', #10281, #44537, #30560 ) ;
#48841=DIRECTION ( 'NONE',  ( 0.000000000000000000, -0.01356324068817999114, 0.9999080150203989437 ) ) ;
#48844=DIRECTION ( 'NONE',  ( 0.000000000000000000, -0.07632122047555069122, 0.9970832820307048427 ) ) ;
#48846=FACE_OUTER_BOUND ( 'NONE', #24609, .T. ) ;
#48847=ORIENTED_EDGE ( 'NONE', *, *, #19074, .F. ) ;
#48849=CARTESIAN_POINT ( 'NONE',  ( -16.18260486426706279, 7.813572176425474858, 9.107691046539137858 ) ) ;
#48850=CARTESIAN_POINT ( 'NONE',  ( -19.02967556479643463, -13.50000000000023803, -2.066764320408402454E-13 ) ) ;
#48851=DIRECTION ( 'NONE',  ( -0.000000000000000000, -0.000000000000000000, -1.000000000000000000 ) ) ;
#48853=CARTESIAN_POINT ( 'NONE',  ( 23.76514404369831013, 1.691375342996074504, 13.39763565441737114 ) ) ;
#48855=CARTESIAN_POINT ( 'NONE',  ( -35.00000000000000000, 0.9416912585474430664, 12.71517666308948513 ) ) ;
#48856=PLANE ( 'NONE',  #1345 ) ;
#48857=EDGE_CURVE ( 'NONE', #42299, #46364, #58422, .T. ) ;
#48861=ORIENTED_EDGE ( 'NONE', *, *, #60782, .T. ) ;
#48862=CARTESIAN_POINT ( 'NONE',  ( 35.00000000000000000, -8.052525312709825300, 8.551552972817161091 ) ) ;
#48864=CARTESIAN_POINT ( 'NONE',  ( 11.90722734030137531, -13.26884457954574081, -2.492663574694747641 ) ) ;
#48866=CARTESIAN_POINT ( 'NONE',  ( -37.00000000000000711, 0.000000000000000000, 0.000000000000000000 ) ) ;
#48867=EDGE_LOOP ( 'NONE', ( #29907, #17592, #13900, #48120 ) ) ;
#48869=CARTESIAN_POINT ( 'NONE',  ( 37.00000000000000711, 8.954052073409734192, 9.076753354953895681 ) ) ;
#48870=DIRECTION ( 'NONE',  ( -1.000000000000000000, 0.000000000000000000, -0.000000000000000000 ) ) ;
#48872=AXIS2_PLACEMENT_3D ( 'NONE', #49480, #14829, #9865 ) ;
#48875=AXIS2_PLACEMENT_3D ( 'NONE', #41168, #15891, #62126 ) ;
#48876=CARTESIAN_POINT ( 'NONE',  ( -35.00000000000000000, 8.573591947375437172, -8.029056188533592930 ) ) ;
#48877=VERTEX_POINT ( 'NONE', #12910 ) ;
#48879=DIRECTION ( 'NONE',  ( 1.000000000000000000, 0.000000000000000000, 0.000000000000000000 ) ) ;
#48880=ADVANCED_FACE ( 'NONE', ( #13552 ), #25173, .T. ) ;
#48881=CARTESIAN_POINT ( 'NONE',  ( -35.00000000000000000, 0.000000000000000000, 0.000000000000000000 ) ) ;
#48882=DIRECTION ( 'NONE',  ( 0.000000000000000000, -0.01356324068817998940, 0.9999080150203990547 ) ) ;
#48884=ORIENTED_EDGE ( 'NONE', *, *, #14472, .T. ) ;
#48885=EDGE_CURVE ( 'NONE', #53880, #48166, #24193, .T. ) ;
#48895=VERTEX_POINT ( 'NONE', #4248 ) ;
#48896=EDGE_CURVE ( 'NONE', #30828, #64603, #4914, .T. ) ;
#48897=ORIENTED_EDGE ( 'NONE', *, *, #46094, .F. ) ;
#48898=EDGE_LOOP ( 'NONE', ( #8697, #7640, #39923, #23624 ) ) ;
#48899=CARTESIAN_POINT ( 'NONE',  ( 35.00000000000000000, 9.493370459201798894, 6.917234959366719060 ) ) ;
#48900=ADVANCED_FACE ( 'NONE', ( #64419 ), #20184, .T. ) ;
#48902=CYLINDRICAL_SURFACE ( 'NONE', #59752, 12.18650000000000055 ) ;
#48904=VECTOR ( 'NONE', #65772, 1000.000000000000000 ) ;
#48905=ORIENTED_EDGE ( 'NONE', *, *, #48508, .F. ) ;
#48907=DIRECTION ( 'NONE',  ( -1.000000000000000000, 0.000000000000000000, 0.000000000000000000 ) ) ;
#48908=EDGE_CURVE ( 'NONE', #19106, #1795, #13614, .T. ) ;
#48910=ORIENTED_EDGE ( 'NONE', *, *, #40179, .F. ) ;
#48911=CARTESIAN_POINT ( 'NONE',  ( -35.00000000000000000, -12.08151691381193160, 4.074242145635959211 ) ) ;
#48913=CARTESIAN_POINT ( 'NONE',  ( -4.590058209962335489, 6.612760447609789871, 25.00000000000000000 ) ) ;
#48914=ORIENTED_EDGE ( 'NONE', *, *, #62247, .T. ) ;
#48915=EDGE_LOOP ( 'NONE', ( #9357, #10284, #4213, #2837 ) ) ;
#48916=EDGE_CURVE ( 'NONE', #65629, #57005, #41439, .T. ) ;
#48917=CARTESIAN_POINT ( 'NONE',  ( -17.83419946441818027, -9.720786832536937538, 7.036071585506806336 ) ) ;
#48919=ORIENTED_EDGE ( 'NONE', *, *, #63618, .F. ) ;
#48920=FACE_OUTER_BOUND ( 'NONE', #53311, .T. ) ;
#48921=VERTEX_POINT ( 'NONE', #4590 ) ;
#48924=DIRECTION ( 'NONE',  ( 1.000000000000000000, 0.000000000000000000, 0.000000000000000000 ) ) ;
#48927=DIRECTION ( 'NONE',  ( -1.000000000000000000, 0.000000000000000000, -0.000000000000000000 ) ) ;
#48929=ORIENTED_EDGE ( 'NONE', *, *, #8229, .F. ) ;
#48932=ORIENTED_EDGE ( 'NONE', *, *, #54618, .T. ) ;
#48934=DIRECTION ( 'NONE',  ( 0.000000000000000000, -0.01356324068817998940, 0.9999080150203990547 ) ) ;
#48935=VERTEX_POINT ( 'NONE', #24860 ) ;
#48939=ORIENTED_EDGE ( 'NONE', *, *, #16819, .F. ) ;
#48940=ADVANCED_FACE ( 'NONE', ( #45138 ), #14842, .T. ) ;
#48941=VERTEX_POINT ( 'NONE', #9877 ) ;
#48943=CIRCLE ( 'NONE', #51016, 5.000000000000000888 ) ;
#48945=CARTESIAN_POINT ( 'NONE',  ( -28.41827485489077532, 3.509237424706436403, 13.03592162821792222 ) ) ;
#48946=CARTESIAN_POINT ( 'NONE',  ( -3.965961450091997964, -8.436165341159954423, 8.545892785218537568 ) ) ;
#48947=CARTESIAN_POINT ( 'NONE',  ( 37.00000000000000711, 4.705694406421931860E-17, -3.469127814946512892E-15 ) ) ;
#48948=DIRECTION ( 'NONE',  ( 0.000000000000000000, -0.9651210252299766701, -0.2618041379715732586 ) ) ;
#48951=EDGE_LOOP ( 'NONE', ( #34629, #62238, #60491, #55875 ) ) ;
#48954=CIRCLE ( 'NONE', #23441, 5.000000000000000000 ) ;
#48956=EDGE_CURVE ( 'NONE', #1650, #25546, #17012, .T. ) ;
#48957=DIRECTION ( 'NONE',  ( 1.000000000000000000, -0.000000000000000000, 0.000000000000000000 ) ) ;
#48959=VECTOR ( 'NONE', #51396, 1000.000000000000000 ) ;
#48960=DIRECTION ( 'NONE',  ( 0.000000000000000000, -0.1387779952735885280, 0.9903235168508540687 ) ) ;
#48961=CARTESIAN_POINT ( 'NONE',  ( 37.00000000000000711, 4.705694406421931860E-17, -3.469127814946512892E-15 ) ) ;
#48963=DIRECTION ( 'NONE',  ( -1.000000000000000000, -0.000000000000000000, 0.000000000000000000 ) ) ;
#48964=CARTESIAN_POINT ( 'NONE',  ( -35.00000000000000000, 11.65554240571059275, -1.456211999474221086 ) ) ;
#48965=DIRECTION ( 'NONE',  ( 0.000000000000000000, -0.2960891610144378849, -0.9551603052523519599 ) ) ;
#48966=B_SPLINE_CURVE_WITH_KNOTS ( 'NONE', 3,
 ( #35221, #9290, #20266, #5312, #35559, #35862, #51208, #65163, #64818, #29915, #54868, #15597, #50222, #19296, #34879, #30561, #29576, #4993, #19940, #60497, #30252, #40208, #39565, #9618 ),
 .UNSPECIFIED., .F., .F.,
 ( 4, 2, 2, 2, 2, 2, 2, 2, 2, 2, 2, 4 ),
 ( 1.939479807224432123E-18, 0.001396101111889962859, 0.002094151667834941687, 0.002792202223779921381, 0.004188303335669874700, 0.005584404447559828018, 0.006980505559449781336, 0.008376606671339735521, 0.009074657227284713482, 0.009772707783229691442, 0.01047075833917466940, 0.01116880889511964736 ),
 .UNSPECIFIED. ) ;
#48967=VECTOR ( 'NONE', #15013, 1000.000000000000000 ) ;
#48969=ORIENTED_EDGE ( 'NONE', *, *, #34232, .F. ) ;
#48970=CARTESIAN_POINT ( 'NONE',  ( 12.75582872833425796, -11.27687878257490794, -4.107405482825274845 ) ) ;
#48971=CIRCLE ( 'NONE', #28775, 4.999999999999999112 ) ;
#48972=VECTOR ( 'NONE', #63523, 1000.000000000000000 ) ;
#48973=ORIENTED_EDGE ( 'NONE', *, *, #12221, .F. ) ;
#48974=CARTESIAN_POINT ( 'NONE',  ( -37.00000000000000711, -11.50504120060940316, -4.018060380616521599 ) ) ;
#48983=CARTESIAN_POINT ( 'NONE',  ( -35.00000000000000000, 0.000000000000000000, 0.000000000000000000 ) ) ;
#48984=EDGE_CURVE ( 'NONE', #26657, #40821, #61392, .T. ) ;
#48986=VERTEX_POINT ( 'NONE', #41776 ) ;
#48987=EDGE_CURVE ( 'NONE', #17242, #17690, #59498, .T. ) ;
#48988=DIRECTION ( 'NONE',  ( 1.000000000000000000, 0.000000000000000000, -0.000000000000000000 ) ) ;
#48991=AXIS2_PLACEMENT_3D ( 'NONE', #3717, #31560, #16278 ) ;
#48993=ORIENTED_EDGE ( 'NONE', *, *, #36917, .F. ) ;
#48994=CARTESIAN_POINT ( 'NONE',  ( 37.00000000000000711, -8.954052073409666690, -9.076753354953966735 ) ) ;
#48995=FACE_OUTER_BOUND ( 'NONE', #50820, .T. ) ;
#48996=CARTESIAN_POINT ( 'NONE',  ( 27.62838931380291996, 25.00000000000000000, -3.066727421130092779 ) ) ;
#48997=CARTESIAN_POINT ( 'NONE',  ( 11.99083905025487340, -8.556418439408641774, -8.415045165346302980 ) ) ;
#48999=ADVANCED_FACE ( 'NONE', ( #62073 ), #51463, .T. ) ;
#49002=ORIENTED_EDGE ( 'NONE', *, *, #61162, .T. ) ;
#49003=CARTESIAN_POINT ( 'NONE',  ( -20.79170840334646542, 12.91784323155722980, -3.921648409140116698 ) ) ;
#49006=CYLINDRICAL_SURFACE ( 'NONE', #9679, 12.74999999999999822 ) ;
#49007=CARTESIAN_POINT ( 'NONE',  ( 35.00000000000000000, -6.303578524887018197, -10.42955799785318050 ) ) ;
#49008=DIRECTION ( 'NONE',  ( 1.000000000000000000, 0.000000000000000000, 0.000000000000000000 ) ) ;
#49010=CIRCLE ( 'NONE', #10758, 4.999999999999999112 ) ;
#49011=CARTESIAN_POINT ( 'NONE',  ( 35.00000000000000000, 10.64792938439763859, 5.927257550915197015 ) ) ;
#49014=LINE ( 'NONE', #14692, #18299 ) ;
#49015=ORIENTED_EDGE ( 'NONE', *, *, #48789, .F. ) ;
#49016=CARTESIAN_POINT ( 'NONE',  ( -4.975205859172449507, -1.416020129149132778, 13.42553116244733680 ) ) ;
#49017=EDGE_LOOP ( 'NONE', ( #45711, #8346, #25603, #14806 ) ) ;
#49018=EDGE_LOOP ( 'NONE', ( #16834, #28295, #46826, #8302 ) ) ;
#49019=DIRECTION ( 'NONE',  ( 1.000000000000000000, 0.000000000000000000, 0.000000000000000000 ) ) ;
#49021=LINE ( 'NONE', #7433, #42546 ) ;
#49024=CIRCLE ( 'NONE', #35156, 5.000000000000000888 ) ;
#49025=DIRECTION ( 'NONE',  ( -0.000000000000000000, -0.000000000000000000, -1.000000000000000000 ) ) ;
#49026=ADVANCED_FACE ( 'NONE', ( #30798, #41109, #36468, #46441, #15517, #890, #6545, #45788, #16523, #21164, #11514, #15195, #56778, #50781, #25498, #11201 ), #20524, .T. ) ;
#49027=CARTESIAN_POINT ( 'NONE',  ( -36.00000000000000711, -12.57916205664480103, -2.080187960898693511 ) ) ;
#49029=EDGE_CURVE ( 'NONE', #11975, #60850, #39314, .T. ) ;
#49030=ORIENTED_EDGE ( 'NONE', *, *, #37638, .F. ) ;
#49031=DIRECTION ( 'NONE',  ( 1.000000000000000000, 0.000000000000000000, -0.000000000000000000 ) ) ;
#49032=AXIS2_PLACEMENT_3D ( 'NONE', #4081, #2800, #3456 ) ;
#49034=CYLINDRICAL_SURFACE ( 'NONE', #58329, 12.18650000000000055 ) ;
#49035=VECTOR ( 'NONE', #45458, 1000.000000000000000 ) ;
#49036=EDGE_CURVE ( 'NONE', #53488, #61135, #13811, .T. ) ;
#49037=CARTESIAN_POINT ( 'NONE',  ( 35.00000000000000000, 11.44858830469736333, -2.627174906297124135 ) ) ;
#49038=CARTESIAN_POINT ( 'NONE',  ( -37.00000000000000711, 0.000000000000000000, 0.000000000000000000 ) ) ;
#49039=AXIS2_PLACEMENT_3D ( 'NONE', #53511, #47848, #17266 ) ;
#49041=CARTESIAN_POINT ( 'NONE',  ( 9.039992663053343591, 3.544502836495995624, -11.46723145265938371 ) ) ;
#49042=CIRCLE ( 'NONE', #15015, 12.74999999999999822 ) ;
#49043=AXIS2_PLACEMENT_3D ( 'NONE', #52502, #16248, #11577 ) ;
#49044=ADVANCED_FACE ( 'NONE', ( #43083 ), #62701, .T. ) ;
#49046=CARTESIAN_POINT ( 'NONE',  ( 9.687175622948609899, 11.98570860552671391, -0.5854820436212360146 ) ) ;
#49048=FACE_OUTER_BOUND ( 'NONE', #39241, .T. ) ;
#49050=CIRCLE ( 'NONE', #16126, 5.000000000000000000 ) ;
#49051=CIRCLE ( 'NONE', #60705, 12.18650000000000233 ) ;
#49052=CYLINDRICAL_SURFACE ( 'NONE', #34158, 12.74999999999999822 ) ;
#49054=ORIENTED_EDGE ( 'NONE', *, *, #25875, .F. ) ;
#49055=CARTESIAN_POINT ( 'NONE',  ( -16.98800322446194855, 2.922502605998049674, 13.17987020110344787 ) ) ;
#49056=CARTESIAN_POINT ( 'NONE',  ( -9.689264015130110153, -9.446331388885504055, -7.412799815278878768 ) ) ;
#49057=FACE_OUTER_BOUND ( 'NONE', #42263, .T. ) ;
#49058=ORIENTED_EDGE ( 'NONE', *, *, #39024, .F. ) ;
#49059=CARTESIAN_POINT ( 'NONE',  ( 23.30833610924781851, 11.22569009227929016, -7.505971052558499501 ) ) ;
#49062=EDGE_LOOP ( 'NONE', ( #9079, #20173, #63669, #26467 ) ) ;
#49063=DIRECTION ( 'NONE',  ( 0.000000000000000000, -0.07632122047555069122, 0.9970832820307048427 ) ) ;
#49064=AXIS2_PLACEMENT_3D ( 'NONE', #6074, #30991, #51303 ) ;
#49067=EDGE_LOOP ( 'NONE', ( #64355, #57986, #10184, #56003 ) ) ;
#49068=CIRCLE ( 'NONE', #31009, 12.18649999999999878 ) ;
#49069=EDGE_CURVE ( 'NONE', #7009, #7257, #27459, .T. ) ;
#49072=CYLINDRICAL_SURFACE ( 'NONE', #16300, 12.75000000000000178 ) ;
#49075=CARTESIAN_POINT ( 'NONE',  ( -25.54417658651491863, 25.00000000000000000, 11.22596262356930197 ) ) ;
#49076=CARTESIAN_POINT ( 'NONE',  ( -35.00000000000000000, 0.000000000000000000, 0.000000000000000000 ) ) ;
#49077=VERTEX_POINT ( 'NONE', #63359 ) ;
#49078=CYLINDRICAL_SURFACE ( 'NONE', #1214, 5.000000000000000888 ) ;
#49079=ORIENTED_EDGE ( 'NONE', *, *, #41196, .T. ) ;
#49081=VECTOR ( 'NONE', #35407, 1000.000000000000000 ) ;
#49082=ORIENTED_EDGE ( 'NONE', *, *, #14337, .F. ) ;
#49083=ORIENTED_EDGE ( 'NONE', *, *, #29888, .F. ) ;
#49084=CARTESIAN_POINT ( 'NONE',  ( -25.47089039327535787, 11.72955104421914641, 6.684715474021441395 ) ) ;
#49086=CARTESIAN_POINT ( 'NONE',  ( -25.32250750182991794, 7.778036012028926471, 11.03925478766256951 ) ) ;
#49087=DIRECTION ( 'NONE',  ( -1.000000000000000000, 0.000000000000000000, 0.000000000000000000 ) ) ;
#49088=DIRECTION ( 'NONE',  ( 0.000000000000000000, 0.9246979985058736418, 0.3807014730195186214 ) ) ;
#49089=CARTESIAN_POINT ( 'NONE',  ( -47.00000000000000711, 0.000000000000000000, 0.000000000000000000 ) ) ;
#49092=VERTEX_POINT ( 'NONE', #57407 ) ;
#49093=CARTESIAN_POINT ( 'NONE',  ( 11.92180594182149456, 0.08356320926551469297, 11.99997121442060077 ) ) ;
#49094=DIRECTION ( 'NONE',  ( 1.000000000000000000, 0.000000000000000000, -0.000000000000000000 ) ) ;
#49095=CYLINDRICAL_SURFACE ( 'NONE', #61913, 12.18649999999999878 ) ;
#49096=ORIENTED_EDGE ( 'NONE', *, *, #54618, .F. ) ;
#49098=VECTOR ( 'NONE', #18223, 1000.000000000000000 ) ;
#49099=DIRECTION ( 'NONE',  ( -1.000000000000000000, 0.000000000000000000, 0.000000000000000000 ) ) ;
#49101=CARTESIAN_POINT ( 'NONE',  ( -35.00000000000000000, 11.54110654723652196, -2.185196060783755279 ) ) ;
#49102=AXIS2_PLACEMENT_3D ( 'NONE', #27630, #47933, #29202 ) ;
#49104=CARTESIAN_POINT ( 'NONE',  ( -29.65843796945371125, -0.5587665441277258616, 13.49517765288613980 ) ) ;
#49106=CARTESIAN_POINT ( 'NONE',  ( -9.044148139924336860, 12.95551142774389319, -3.795959767731164725 ) ) ;
#49107=EDGE_CURVE ( 'NONE', #11130, #34336, #18493, .T. ) ;
#49108=ORIENTED_EDGE ( 'NONE', *, *, #60318, .F. ) ;
#49110=LINE ( 'NONE', #24456, #4117 ) ;
#49112=CARTESIAN_POINT ( 'NONE',  ( 35.00000000000000000, 4.705694406421931860E-17, -3.469127814946512892E-15 ) ) ;
#49113=AXIS2_PLACEMENT_3D ( 'NONE', #51453, #56072, #20174 ) ;
#49115=CARTESIAN_POINT ( 'NONE',  ( -37.00000000000000711, -11.32068061209291265, -5.865551165831199398 ) ) ;
#49116=EDGE_CURVE ( 'NONE', #31052, #35667, #53142, .T. ) ;
#49117=DIRECTION ( 'NONE',  ( 1.000000000000000000, 0.000000000000000000, 0.000000000000000000 ) ) ;
#49118=AXIS2_PLACEMENT_3D ( 'NONE', #56924, #1050, #45953 ) ;
#49119=LINE ( 'NONE', #20798, #26673 ) ;
#49120=DIRECTION ( 'NONE',  ( 0.000000000000000000, -0.01356324068817998940, 0.9999080150203990547 ) ) ;
#49121=CIRCLE ( 'NONE', #45925, 12.18650000000000233 ) ;
#49123=DIRECTION ( 'NONE',  ( 0.5702167306099040767, -0.8214942970785323872, 0.000000000000000000 ) ) ;
#49124=ADVANCED_FACE ( 'NONE', ( #27799 ), #22827, .T. ) ;
#49134=CARTESIAN_POINT ( 'NONE',  ( 29.72418321309294953, 10.03637985811942102, 9.031728217441806095 ) ) ;
#49136=VERTEX_POINT ( 'NONE', #52438 ) ;
#49139=CARTESIAN_POINT ( 'NONE',  ( 16.87411952752378852, -11.83808284204321204, 6.535263924872153574 ) ) ;
#49140=LINE ( 'NONE', #9506, #54080 ) ;
#49141=DIRECTION ( 'NONE',  ( 1.000000000000000000, 0.000000000000000000, 0.000000000000000000 ) ) ;
#49145=ORIENTED_EDGE ( 'NONE', *, *, #52298, .T. ) ;
#49146=DIRECTION ( 'NONE',  ( -1.000000000000000000, 0.000000000000000000, 0.000000000000000000 ) ) ;
#49152=DIRECTION ( 'NONE',  ( 0.000000000000000000, 0.01356324068817992175, -0.9999080150203990547 ) ) ;
#49153=CARTESIAN_POINT ( 'NONE',  ( -28.85619398320021745, 3.750539801530000439, -11.39883551934754280 ) ) ;
#49155=ORIENTED_EDGE ( 'NONE', *, *, #27254, .T. ) ;
#49156=VERTEX_POINT ( 'NONE', #60267 ) ;
#49157=CIRCLE ( 'NONE', #28969, 12.75000000000000178 ) ;
#49161=EDGE_CURVE ( 'NONE', #40614, #17964, #51009, .T. ) ;
#49162=CIRCLE ( 'NONE', #37455, 12.74999999999999822 ) ;
#49164=B_SPLINE_CURVE_WITH_KNOTS ( 'NONE', 3,
 ( #58306, #53323, #21759, #26395, #6787, #57001, #63273, #27062, #47355, #41691, #61980, #1796, #16436, #31696 ),
 .UNSPECIFIED., .F., .F.,
 ( 4, 2, 2, 2, 2, 2, 4 ),
 ( 3.035766082959412415E-18, 0.001898234031154803509, 0.002847351046732204179, 0.003796468062309605717, 0.004745585077887007688, 0.005694702093464407491, 0.007592936124619207097 ),
 .UNSPECIFIED. ) ;
#49168=VECTOR ( 'NONE', #63508, 1000.000000000000000 ) ;
#49171=EDGE_LOOP ( 'NONE', ( #40809, #31551, #44653, #60386, #49280, #12541 ) ) ;
#49173=ORIENTED_EDGE ( 'NONE', *, *, #11874, .F. ) ;
#49176=ORIENTED_EDGE ( 'NONE', *, *, #7260, .F. ) ;
#49180=CARTESIAN_POINT ( 'NONE',  ( -36.00000000000000711, -1.908798535168293897, -12.60630747491665282 ) ) ;
#49181=DIRECTION ( 'NONE',  ( 1.000000000000000000, 0.000000000000000000, 0.000000000000000000 ) ) ;
#49182=DIRECTION ( 'NONE',  ( 0.000000000000000000, -0.01356324068817991828, 0.9999080150203990547 ) ) ;
#49184=EDGE_CURVE ( 'NONE', #48271, #64858, #4773, .T. ) ;
#49188=EDGE_CURVE ( 'NONE', #64815, #57020, #7458, .T. ) ;
#49189=LINE ( 'NONE', #29842, #14073 ) ;
#49192=FACE_OUTER_BOUND ( 'NONE', #5200, .T. ) ;
#49195=CARTESIAN_POINT ( 'NONE',  ( -37.00000000000000711, -8.624332853796127907, 9.390600770287960586 ) ) ;
#49197=CARTESIAN_POINT ( 'NONE',  ( 26.08439714455133185, 25.00000000000000000, 3.743551691817327942 ) ) ;
#49198=VECTOR ( 'NONE', #11159, 1000.000000000000000 ) ;
#49199=VECTOR ( 'NONE', #5640, 1000.000000000000000 ) ;
#49200=VERTEX_POINT ( 'NONE', #5082 ) ;
#49201=ADVANCED_FACE ( 'NONE', ( #72 ), #20694, .T. ) ;
#49202=DIRECTION ( 'NONE',  ( 0.000000000000000000, 0.01356324068817998940, -0.9999080150203990547 ) ) ;
#49203=ORIENTED_EDGE ( 'NONE', *, *, #10824, .F. ) ;
#49205=FACE_OUTER_BOUND ( 'NONE', #58217, .T. ) ;
#49206=DIRECTION ( 'NONE',  ( 1.000000000000000000, 0.000000000000000000, 0.000000000000000000 ) ) ;
#49207=AXIS2_PLACEMENT_3D ( 'NONE', #64599, #19412, #40318 ) ;
#49208=CARTESIAN_POINT ( 'NONE',  ( -25.54417658651491863, -7.498517398407823720, 11.22596262356930197 ) ) ;
#49211=AXIS2_PLACEMENT_3D ( 'NONE', #15139, #20471, #56363 ) ;
#49213=DIRECTION ( 'NONE',  ( 0.000000000000000000, -0.01356324068817998940, 0.9999080150203990547 ) ) ;
#49214=CARTESIAN_POINT ( 'NONE',  ( 9.772191328647716446, 2.017934697571601710, 11.83060272079844388 ) ) ;
#49216=AXIS2_PLACEMENT_3D ( 'NONE', #44132, #27519, #7236 ) ;
#49219=VERTEX_POINT ( 'NONE', #15677 ) ;
#49222=VERTEX_POINT ( 'NONE', #10369 ) ;
#49223=DIRECTION ( 'NONE',  ( 0.000000000000000000, -0.4935949184179321825, 0.8696919319575150409 ) ) ;
#49227=ORIENTED_EDGE ( 'NONE', *, *, #16886, .T. ) ;
#49233=DIRECTION ( 'NONE',  ( 1.000000000000000000, 0.000000000000000000, 0.000000000000000000 ) ) ;
#49235=ORIENTED_EDGE ( 'NONE', *, *, #31161, .F. ) ;
#49238=VERTEX_POINT ( 'NONE', #55625 ) ;
#49239=ORIENTED_EDGE ( 'NONE', *, *, #6994, .T. ) ;
#49241=CIRCLE ( 'NONE', #58784, 4.999999999999999112 ) ;
#49243=DIRECTION ( 'NONE',  ( 1.000000000000000000, 0.000000000000000000, 0.000000000000000000 ) ) ;
#49245=ORIENTED_EDGE ( 'NONE', *, *, #65327, .T. ) ;
#49248=ORIENTED_EDGE ( 'NONE', *, *, #1761, .T. ) ;
#49253=CIRCLE ( 'NONE', #7842, 5.000000000000000000 ) ;
#49254=EDGE_LOOP ( 'NONE', ( #10373, #22150, #16568, #28275 ) ) ;
#49257=PRESENTATION_STYLE_ASSIGNMENT (( #53898 ) ) ;
#49258=ORIENTED_EDGE ( 'NONE', *, *, #18526, .F. ) ;
#49259=ORIENTED_EDGE ( 'NONE', *, *, #28615, .T. ) ;
#49260=ORIENTED_EDGE ( 'NONE', *, *, #45577, .F. ) ;
#49261=CARTESIAN_POINT ( 'NONE',  ( -35.00000000000000000, 0.000000000000000000, 0.000000000000000000 ) ) ;
#49262=VECTOR ( 'NONE', #60994, 1000.000000000000000 ) ;
#49265=EDGE_CURVE ( 'NONE', #61654, #26437, #31906, .T. ) ;
#49272=EDGE_CURVE ( 'NONE', #44677, #35395, #8511, .T. ) ;
#49273=VECTOR ( 'NONE', #23483, 1000.000000000000000 ) ;
#49274=CARTESIAN_POINT ( 'NONE',  ( -19.18766336847270182, -4.482615930790736058, -12.73550487531713493 ) ) ;
#49275=EDGE_CURVE ( 'NONE', #9298, #17535, #45677, .T. ) ;
#49277=CARTESIAN_POINT ( 'NONE',  ( 22.88594695219327235, -4.822122601967141264, 10.98850006195556261 ) ) ;
#49280=ORIENTED_EDGE ( 'NONE', *, *, #279, .T. ) ;
#49281=AXIS2_PLACEMENT_3D ( 'NONE', #29574, #45875, #50219 ) ;
#49283=EDGE_CURVE ( 'NONE', #61894, #16455, #54155, .T. ) ;
#49285=ORIENTED_EDGE ( 'NONE', *, *, #2249, .F. ) ;
#49286=EDGE_CURVE ( 'NONE', #54019, #18418, #46949, .T. ) ;
#49287=FACE_OUTER_BOUND ( 'NONE', #341, .T. ) ;
#49291=CARTESIAN_POINT ( 'NONE',  ( 11.87488961725744296, 11.87513487482758556, -1.734258419331586198 ) ) ;
#49292=ORIENTED_EDGE ( 'NONE', *, *, #4518, .F. ) ;
#49293=VECTOR ( 'NONE', #6029, 1000.000000000000000 ) ;
#49294=CIRCLE ( 'NONE', #5762, 12.75000000000000178 ) ;
#49295=CARTESIAN_POINT ( 'NONE',  ( -37.00000000000000711, 0.000000000000000000, 0.000000000000000000 ) ) ;
#49297=AXIS2_PLACEMENT_3D ( 'NONE', #42369, #27114, #11798 ) ;
#49298=EDGE_CURVE ( 'NONE', #45722, #8028, #61615, .T. ) ;
#49299=CARTESIAN_POINT ( 'NONE',  ( -35.00000000000000000, -11.80185301892984384, 4.824807283154076920 ) ) ;
#49301=AXIS2_PLACEMENT_3D ( 'NONE', #14473, #64050, #44740 ) ;
#49302=EDGE_CURVE ( 'NONE', #3960, #41521, #6217, .T. ) ;
#49303=CARTESIAN_POINT ( 'NONE',  ( -17.19821944094000088, -8.152051224790197281, 8.812769963160908659 ) ) ;
#49307=DIRECTION ( 'NONE',  ( 0.000000000000000000, 0.01356324068817998940, -0.9999080150203990547 ) ) ;
#49308=CARTESIAN_POINT ( 'NONE',  ( -35.00000000000000000, -1.738225594539906771, -12.63095688309030962 ) ) ;
#49309=CIRCLE ( 'NONE', #397, 5.000000000000000000 ) ;
#49310=AXIS2_PLACEMENT_3D ( 'NONE', #33183, #28851, #32834 ) ;
#49311=ORIENTED_EDGE ( 'NONE', *, *, #55147, .T. ) ;
#49313=VERTEX_POINT ( 'NONE', #11358 ) ;
#49316=LINE ( 'NONE', #63911, #61886 ) ;
#49317=AXIS2_PLACEMENT_3D ( 'NONE', #31171, #37459, #37120 ) ;
#49318=DIRECTION ( 'NONE',  ( 1.000000000000000000, 0.000000000000000000, 0.000000000000000000 ) ) ;
#49324=EDGE_CURVE ( 'NONE', #10957, #6586, #49963, .T. ) ;
#49325=EDGE_CURVE ( 'NONE', #30454, #36193, #58468, .T. ) ;
#49327=ORIENTED_EDGE ( 'NONE', *, *, #34452, .F. ) ;
#49329=DIRECTION ( 'NONE',  ( 0.000000000000000000, -0.01356324068817991828, 0.9999080150203990547 ) ) ;
#49336=CARTESIAN_POINT ( 'NONE',  ( -37.00000000000000711, 2.696588552979058750, 12.46157735505190267 ) ) ;
#49343=VECTOR ( 'NONE', #50437, 1000.000000000000000 ) ;
#49345=CARTESIAN_POINT ( 'NONE',  ( -37.00000000000000711, 0.000000000000000000, 0.000000000000000000 ) ) ;
#49346=CARTESIAN_POINT ( 'NONE',  ( -47.00000000000000711, 0.000000000000000000, 0.000000000000000000 ) ) ;
#49348=CARTESIAN_POINT ( 'NONE',  ( 35.00000000000000000, -11.05394794832825767, 5.130401251914841865 ) ) ;
#49350=EDGE_CURVE ( 'NONE', #51910, #55845, #36300, .T. ) ;
#49351=DIRECTION ( 'NONE',  ( -1.000000000000000000, 0.000000000000000000, 0.000000000000000000 ) ) ;
#49353=ORIENTED_EDGE ( 'NONE', *, *, #14335, .F. ) ;
#49354=ORIENTED_EDGE ( 'NONE', *, *, #41045, .F. ) ;
#49355=DIRECTION ( 'NONE',  ( 1.000000000000000000, 0.000000000000000000, 0.000000000000000000 ) ) ;
#49357=EDGE_CURVE ( 'NONE', #21596, #2479, #9584, .T. ) ;
#49358=ORIENTED_EDGE ( 'NONE', *, *, #21915, .F. ) ;
#49359=AXIS2_PLACEMENT_3D ( 'NONE', #21445, #52696, #26111 ) ;
#49361=DIRECTION ( 'NONE',  ( 1.000000000000000000, 0.000000000000000000, -0.000000000000000000 ) ) ;
#49364=DIRECTION ( 'NONE',  ( 1.000000000000000000, 0.000000000000000000, 0.000000000000000000 ) ) ;
#49366=LINE ( 'NONE', #39343, #23849 ) ;
#49367=( BOUNDED_CURVE ( )  B_SPLINE_CURVE ( 3, ( #36054, #16464, #62634, #11146 ),
 .UNSPECIFIED., .F., .F. ) 
 B_SPLINE_CURVE_WITH_KNOTS ( ( 4, 4 ),
 ( 4.423281819347653965, 4.457400363100178176 ),
 .UNSPECIFIED. ) 
 CURVE ( )  GEOMETRIC_REPRESENTATION_ITEM ( )  RATIONAL_B_SPLINE_CURVE ( ( 1.000000000000000000, 0.9999029961002143807, 0.9999029961002143807, 1.000000000000000000 ) ) 
 REPRESENTATION_ITEM ( '' )  );
#49368=VERTEX_POINT ( 'NONE', #6071 ) ;
#49369=CIRCLE ( 'NONE', #47223, 5.000000000000000888 ) ;
#49371=CARTESIAN_POINT ( 'NONE',  ( 37.00000000000000711, -1.171570255487531131, -11.68758509253248157 ) ) ;
#49373=DIRECTION ( 'NONE',  ( 0.000000000000000000, 0.01356324068817998940, -0.9999080150203990547 ) ) ;
#49374=ADVANCED_FACE ( 'NONE', ( #52608 ), #11677, .T. ) ;
#49375=ORIENTED_EDGE ( 'NONE', *, *, #47031, .T. ) ;
#49376=EDGE_CURVE ( 'NONE', #61981, #57557, #6384, .T. ) ;
#49380=CARTESIAN_POINT ( 'NONE',  ( -11.40165637462999904, -7.508992741355383416, 11.21895841913464409 ) ) ;
#49382=EDGE_CURVE ( 'NONE', #62542, #36458, #52099, .T. ) ;
#49383=DIRECTION ( 'NONE',  ( 0.000000000000000000, -0.7617968321374946061, -0.6478160128811869534 ) ) ;
#49385=DIRECTION ( 'NONE',  ( 0.000000000000000000, -0.01356324068818000848, 0.9999080150203990547 ) ) ;
#49386=CARTESIAN_POINT ( 'NONE',  ( -37.00000000000000711, 0.000000000000000000, 0.000000000000000000 ) ) ;
#49387=CYLINDRICAL_SURFACE ( 'NONE', #8827, 5.000000000000000888 ) ;
#49388=DIRECTION ( 'NONE',  ( 0.000000000000000000, -1.000000000000000000, 0.000000000000000000 ) ) ;
#49390=CIRCLE ( 'NONE', #52567, 5.000000000000000888 ) ;
#49391=ORIENTED_EDGE ( 'NONE', *, *, #21634, .F. ) ;
#49394=CARTESIAN_POINT ( 'NONE',  ( -17.29244623348158783, 2.525873743887551814, -11.73115347397429176 ) ) ;
#49395=EDGE_LOOP ( 'NONE', ( #3354, #3110, #1190, #19475 ) ) ;
#49396=LINE ( 'NONE', #29714, #40373 ) ;
#49397=CYLINDRICAL_SURFACE ( 'NONE', #10707, 12.18649999999999878 ) ;
#49399=VECTOR ( 'NONE', #59225, 1000.000000000000000 ) ;
#49401=CYLINDRICAL_SURFACE ( 'NONE', #38483, 5.000000000000000888 ) ;
#49402=AXIS2_PLACEMENT_3D ( 'NONE', #25093, #51020, #20757 ) ;
#49404=EDGE_LOOP ( 'NONE', ( #61632, #38515, #27573, #6353 ) ) ;
#49409=DIRECTION ( 'NONE',  ( 1.000000000000000000, 0.000000000000000000, 0.000000000000000000 ) ) ;
#49411=ORIENTED_EDGE ( 'NONE', *, *, #45355, .T. ) ;
#49413=VERTEX_POINT ( 'NONE', #37940 ) ;
#49414=DIRECTION ( 'NONE',  ( 0.000000000000000000, -0.01356324068817998940, 0.9999080150203990547 ) ) ;
#49418=CARTESIAN_POINT ( 'NONE',  ( -24.81333898230430535, 10.23818681080158655, 8.801029818708748564 ) ) ;
#49420=CARTESIAN_POINT ( 'NONE',  ( 37.00000000000000711, 9.908974237959730758, 6.307491713048920090 ) ) ;
#49421=AXIS2_PLACEMENT_3D ( 'NONE', #42268, #26349, #21023 ) ;
#49422=DIRECTION ( 'NONE',  ( 1.000000000000000000, -0.000000000000000000, 0.000000000000000000 ) ) ;
#49423=DIRECTION ( 'NONE',  ( 0.000000000000000000, -0.6269146997507876184, -0.7790879021242596014 ) ) ;
#49424=CARTESIAN_POINT ( 'NONE',  ( 35.00000000000000000, 8.573591947375318156, -8.029056188533719052 ) ) ;
#49425=EDGE_LOOP ( 'NONE', ( #63580, #5810, #536, #41220 ) ) ;
#49426=ORIENTED_EDGE ( 'NONE', *, *, #29862, .F. ) ;
#49433=ADVANCED_FACE ( 'NONE', ( #17679 ), #8034, .T. ) ;
#49435=DIRECTION ( 'NONE',  ( -1.000000000000000000, 0.000000000000000000, 0.000000000000000000 ) ) ;
#49436=CYLINDRICAL_SURFACE ( 'NONE', #48230, 12.74999999999999822 ) ;
#49437=VERTEX_POINT ( 'NONE', #38257 ) ;
#49438=AXIS2_PLACEMENT_3D ( 'NONE', #36592, #16637, #56893 ) ;
#49440=DIRECTION ( 'NONE',  ( -1.000000000000000000, -0.000000000000000000, 0.000000000000000000 ) ) ;
#49441=CARTESIAN_POINT ( 'NONE',  ( 37.00000000000000711, -9.390600770288051180, -8.624332853796024878 ) ) ;
#49443=ADVANCED_FACE ( 'NONE', ( #42933 ), #27980, .T. ) ;
#49444=AXIS2_PLACEMENT_3D ( 'NONE', #43400, #63677, #58742 ) ;
#49448=CARTESIAN_POINT ( 'NONE',  ( 7.290274017563119990, -6.630274286016201835, -11.76160339896002149 ) ) ;
#49449=FACE_OUTER_BOUND ( 'NONE', #40361, .T. ) ;
#49450=EDGE_CURVE ( 'NONE', #2058, #40710, #58233, .T. ) ;
#49452=CARTESIAN_POINT ( 'NONE',  ( -35.00000000000000000, -11.60979404548637461, 3.704519465651263221 ) ) ;
#49453=ORIENTED_EDGE ( 'NONE', *, *, #35330, .T. ) ;
#49455=CARTESIAN_POINT ( 'NONE',  ( 22.21053567399755124, 13.47268488964861000, -0.8606552803710473265 ) ) ;
#49457=EDGE_CURVE ( 'NONE', #16833, #55363, #35118, .T. ) ;
#49465=CARTESIAN_POINT ( 'NONE',  ( -8.333177752689428175, -1.918561656600153098, -13.36554899929619289 ) ) ;
#49466=CYLINDRICAL_SURFACE ( 'NONE', #18301, 12.74999999999999822 ) ;
#49467=DIRECTION ( 'NONE',  ( -1.000000000000000000, 0.000000000000000000, 0.000000000000000000 ) ) ;
#49469=CARTESIAN_POINT ( 'NONE',  ( -9.614904064140660012, -12.77521411685881425, -4.380909147133119852 ) ) ;
#49471=ORIENTED_EDGE ( 'NONE', *, *, #45102, .F. ) ;
#49474=CARTESIAN_POINT ( 'NONE',  ( -37.00000000000000711, 0.000000000000000000, 0.000000000000000000 ) ) ;
#49475=CARTESIAN_POINT ( 'NONE',  ( -37.00000000000000711, 3.093009498344089003, -11.78745411414836752 ) ) ;
#49477=DIRECTION ( 'NONE',  ( 0.000000000000000000, -0.01356324068817998940, 0.9999080150203990547 ) ) ;
#49480=CARTESIAN_POINT ( 'NONE',  ( 47.00000000000000711, 4.705694406421931860E-17, -3.469127814946512892E-15 ) ) ;
#49483=ORIENTED_EDGE ( 'NONE', *, *, #38765, .T. ) ;
#49486=DIRECTION ( 'NONE',  ( 1.000000000000000000, 0.000000000000000000, -0.000000000000000000 ) ) ;
#49488=DIRECTION ( 'NONE',  ( 1.000000000000000000, -0.000000000000000000, -0.000000000000000000 ) ) ;
#49489=VERTEX_POINT ( 'NONE', #22993 ) ;
#49490=CARTESIAN_POINT ( 'NONE',  ( 35.00000000000000000, 4.705694406421931860E-17, -3.469127814946512892E-15 ) ) ;
#49492=CARTESIAN_POINT ( 'NONE',  ( -35.00000000000000000, -11.02904044024211849, 4.041347439435823752 ) ) ;
#49493=ORIENTED_EDGE ( 'NONE', *, *, #59345, .T. ) ;
#49494=ORIENTED_EDGE ( 'NONE', *, *, #31128, .T. ) ;
#49498=ORIENTED_EDGE ( 'NONE', *, *, #40382, .F. ) ;
#49499=CARTESIAN_POINT ( 'NONE',  ( 4.040225803495397727, -10.40460620550539161, -5.985298750905354126 ) ) ;
#49500=VERTEX_POINT ( 'NONE', #38606 ) ;
#49501=CARTESIAN_POINT ( 'NONE',  ( 37.00000000000000711, -9.217970097227780713, -7.971186206369443639 ) ) ;
#49503=DIRECTION ( 'NONE',  ( 0.000000000000000000, 0.01356324068817998940, -0.9999080150203989437 ) ) ;
#49504=DIRECTION ( 'NONE',  ( -1.000000000000000000, 0.000000000000000000, 0.000000000000000000 ) ) ;
#49507=VERTEX_POINT ( 'NONE', #28959 ) ;
#49509=CARTESIAN_POINT ( 'NONE',  ( -16.60799812198239778, 7.628243526059563351, 9.263658496022879163 ) ) ;
#49510=CARTESIAN_POINT ( 'NONE',  ( -19.31247144139280181, -13.48787587759413142, -0.6540986653347018454 ) ) ;
#49511=CARTESIAN_POINT ( 'NONE',  ( 35.00000000000000000, 8.496612874013157679, -9.506317355798403312 ) ) ;
#49512=CARTESIAN_POINT ( 'NONE',  ( 35.00000000000000000, -3.704519465651390675, -11.60979404548633731 ) ) ;
#49514=CARTESIAN_POINT ( 'NONE',  ( -37.00000000000000711, 0.000000000000000000, 0.000000000000000000 ) ) ;
#49515=DIRECTION ( 'NONE',  ( 0.000000000000000000, -0.01356324068817998940, 0.9999080150203990547 ) ) ;
#49520=CIRCLE ( 'NONE', #45232, 12.74999999999999822 ) ;
#49521=AXIS2_PLACEMENT_3D ( 'NONE', #10738, #31027, #6754 ) ;
#49526=CARTESIAN_POINT ( 'NONE',  ( -35.00000000000000000, 10.14408668126213442, 5.921969905510389154 ) ) ;
#49528=ORIENTED_EDGE ( 'NONE', *, *, #12955, .F. ) ;
#49533=EDGE_CURVE ( 'NONE', #11516, #41856, #42530, .T. ) ;
#49536=VERTEX_POINT ( 'NONE', #60188 ) ;
#49537=DIRECTION ( 'NONE',  ( 1.000000000000000000, 0.000000000000000000, 0.000000000000000000 ) ) ;
#49538=ORIENTED_EDGE ( 'NONE', *, *, #25581, .F. ) ;
#49539=CYLINDRICAL_SURFACE ( 'NONE', #37864, 12.18650000000000055 ) ;
#49540=DIRECTION ( 'NONE',  ( 0.000000000000000000, -0.6478160128812003871, 0.7617968321374830598 ) ) ;
#49541=DIRECTION ( 'NONE',  ( 1.000000000000000000, -0.000000000000000000, -0.000000000000000000 ) ) ;
#49542=CARTESIAN_POINT ( 'NONE',  ( -29.68541646480307250, -2.175302793937436974, -13.34544795947793716 ) ) ;
#49546=EDGE_CURVE ( 'NONE', #6221, #61765, #16003, .T. ) ;
#49550=DIRECTION ( 'NONE',  ( 0.000000000000000000, -0.5472293298355156432, 0.8369827122275419473 ) ) ;
#49554=ORIENTED_EDGE ( 'NONE', *, *, #15098, .T. ) ;
#49555=ORIENTED_EDGE ( 'NONE', *, *, #55172, .F. ) ;
#49557=AXIS2_PLACEMENT_3D ( 'NONE', #48667, #53662, #8100 ) ;
#49558=DIRECTION ( 'NONE',  ( 0.000000000000000000, -0.01356324068817998073, 0.9999080150203990547 ) ) ;
#49562=CIRCLE ( 'NONE', #46372, 5.000000000000000888 ) ;
#49563=CARTESIAN_POINT ( 'NONE',  ( 3.347841273039249721, -10.61118957148187825, 25.00000000000000000 ) ) ;
#49565=ORIENTED_EDGE ( 'NONE', *, *, #63115, .T. ) ;
#49567=DIRECTION ( 'NONE',  ( 0.000000000000000000, -0.01356324068817992175, 0.9999080150203990547 ) ) ;
#49569=ORIENTED_EDGE ( 'NONE', *, *, #57575, .T. ) ;
#49570=ORIENTED_EDGE ( 'NONE', *, *, #51423, .T. ) ;
#49571=CARTESIAN_POINT ( 'NONE',  ( -35.00000000000000000, 0.000000000000000000, 0.000000000000000000 ) ) ;
#49572=VERTEX_POINT ( 'NONE', #54880 ) ;
#49573=EDGE_CURVE ( 'NONE', #49489, #21740, #13859, .T. ) ;
#49574=DIRECTION ( 'NONE',  ( -1.000000000000000000, 0.000000000000000000, 0.000000000000000000 ) ) ;
#49575=ORIENTED_EDGE ( 'NONE', *, *, #6039, .T. ) ;
#49576=EDGE_LOOP ( 'NONE', ( #28453, #56591, #62532, #43806 ) ) ;
#49577=VERTEX_POINT ( 'NONE', #59882 ) ;
#49578=CARTESIAN_POINT ( 'NONE',  ( -2.952869152607111136, 25.00000000000000000, 11.17020052527586138 ) ) ;
#49579=CARTESIAN_POINT ( 'NONE',  ( 35.00000000000000000, -10.42955799785315563, 6.303578524887051948 ) ) ;
#49580=CARTESIAN_POINT ( 'NONE',  ( 37.00000000000000711, 4.705694406421931860E-17, -3.469127814946512892E-15 ) ) ;
#49584=ORIENTED_EDGE ( 'NONE', *, *, #15174, .T. ) ;
#49586=CARTESIAN_POINT ( 'NONE',  ( -17.76813863392193582, -8.408734016395053246, -10.56536593579148153 ) ) ;
#49588=LINE ( 'NONE', #24295, #61506 ) ;
#49591=ORIENTED_EDGE ( 'NONE', *, *, #3897, .F. ) ;
#49596=FACE_OUTER_BOUND ( 'NONE', #12543, .T. ) ;
#49599=CARTESIAN_POINT ( 'NONE',  ( -35.00000000000000000, 9.621072037177116343, -8.366449238204259231 ) ) ;
#49603=AXIS2_PLACEMENT_3D ( 'NONE', #6382, #60931, #10694 ) ;
#49605=ADVANCED_FACE ( 'NONE', ( #4018 ), #4695, .T. ) ;
#49606=AXIS2_PLACEMENT_3D ( 'NONE', #54929, #55604, #25325 ) ;
#49611=CARTESIAN_POINT ( 'NONE',  ( -35.00000000000000000, 0.000000000000000000, 0.000000000000000000 ) ) ;
#49613=VERTEX_POINT ( 'NONE', #65488 ) ;
#49614=DIRECTION ( 'NONE',  ( 0.000000000000000000, 0.9903235168508544017, 0.1387779952735853917 ) ) ;
#49615=ADVANCED_FACE ( 'NONE', ( #44551 ), #60513, .T. ) ;
#49616=VERTEX_POINT ( 'NONE', #9986 ) ;
#49618=EDGE_CURVE ( 'NONE', #3042, #11376, #19311, .T. ) ;
#49622=EDGE_CURVE ( 'NONE', #22141, #12853, #25553, .T. ) ;
#49624=EDGE_LOOP ( 'NONE', ( #34901, #17399, #17952, #25577 ) ) ;
#49625=ORIENTED_EDGE ( 'NONE', *, *, #37664, .F. ) ;
#49626=LINE ( 'NONE', #64251, #51447 ) ;
#49628=EDGE_CURVE ( 'NONE', #58596, #22365, #61668, .T. ) ;
#49629=VERTEX_POINT ( 'NONE', #40910 ) ;
#49634=ORIENTED_EDGE ( 'NONE', *, *, #23022, .T. ) ;
#49635=CARTESIAN_POINT ( 'NONE',  ( 36.00000000000000711, -7.745827850123079727, -10.12742074351894317 ) ) ;
#49636=EDGE_CURVE ( 'NONE', #65189, #61311, #36168, .T. ) ;
#49639=CARTESIAN_POINT ( 'NONE',  ( 37.00000000000000711, 4.705694406421931860E-17, -3.469127814946512892E-15 ) ) ;
#49640=EDGE_LOOP ( 'NONE', ( #19203, #34880, #58042, #42114 ) ) ;
#49642=ORIENTED_EDGE ( 'NONE', *, *, #15462, .T. ) ;
#49644=ORIENTED_EDGE ( 'NONE', *, *, #55475, .F. ) ;
#49645=AXIS2_PLACEMENT_3D ( 'NONE', #37195, #37542, #51862 ) ;
#49646=DIRECTION ( 'NONE',  ( 1.000000000000000000, -0.000000000000000000, -0.000000000000000000 ) ) ;
#49647=DIRECTION ( 'NONE',  ( -1.000000000000000000, 0.000000000000000000, 0.000000000000000000 ) ) ;
#49648=DIRECTION ( 'NONE',  ( 1.000000000000000000, -0.000000000000000000, 0.000000000000000000 ) ) ;
#49649=CARTESIAN_POINT ( 'NONE',  ( 35.00000000000000000, 4.705694406421931860E-17, -3.469127814946512892E-15 ) ) ;
#49651=AXIS2_PLACEMENT_3D ( 'NONE', #30721, #20438, #4835 ) ;
#49653=CARTESIAN_POINT ( 'NONE',  ( -36.00000000000000711, -10.02106554660702997, -7.882940143791884680 ) ) ;
#49654=CARTESIAN_POINT ( 'NONE',  ( -36.00000000000000711, 8.830544224262947495, 9.196955404009329982 ) ) ;
#49655=ORIENTED_EDGE ( 'NONE', *, *, #15462, .F. ) ;
#49656=EDGE_CURVE ( 'NONE', #50600, #7923, #23476, .T. ) ;
#49657=ORIENTED_EDGE ( 'NONE', *, *, #49265, .T. ) ;
#49659=EDGE_LOOP ( 'NONE', ( #26084, #18635, #62248, #40587 ) ) ;
#49661=DIRECTION ( 'NONE',  ( 0.000000000000000000, 0.01356324068817998940, -0.9999080150203990547 ) ) ;
#49666=CARTESIAN_POINT ( 'NONE',  ( -35.00000000000000000, 0.000000000000000000, 0.000000000000000000 ) ) ;
#49669=CARTESIAN_POINT ( 'NONE',  ( -37.00000000000000711, 0.000000000000000000, 0.000000000000000000 ) ) ;
#49670=FACE_OUTER_BOUND ( 'NONE', #32853, .T. ) ;
#49673=AXIS2_PLACEMENT_3D ( 'NONE', #8993, #30567, #13964 ) ;
#49674=ADVANCED_FACE ( 'NONE', ( #347 ), #20625, .T. ) ;
#49675=CIRCLE ( 'NONE', #39075, 5.000000000000002665 ) ;
#49676=CARTESIAN_POINT ( 'NONE',  ( -11.27062903137229810, -6.186534743127487523, 12.00099709470298315 ) ) ;
#49681=DIRECTION ( 'NONE',  ( -1.000000000000000000, -0.000000000000000000, 0.000000000000000000 ) ) ;
#49682=CARTESIAN_POINT ( 'NONE',  ( 1.658631356726815387, 0.7601067232070346513, 11.97997174763777650 ) ) ;
#49685=CIRCLE ( 'NONE', #25228, 12.18650000000000233 ) ;
#49686=LINE ( 'NONE', #40684, #10811 ) ;
#49687=CARTESIAN_POINT ( 'NONE',  ( 35.00000000000000000, 11.56998259273182583, 3.827046518384956020 ) ) ;
#49688=ORIENTED_EDGE ( 'NONE', *, *, #53695, .T. ) ;
#49689=EDGE_CURVE ( 'NONE', #55692, #53292, #32990, .T. ) ;
#49690=CARTESIAN_POINT ( 'NONE',  ( 22.36482863261543486, 13.46837713145128923, -0.9234811557364158707 ) ) ;
#49694=CARTESIAN_POINT ( 'NONE',  ( 35.00000000000000000, -7.718225330433870823, -9.430788938294027091 ) ) ;
#49695=FACE_OUTER_BOUND ( 'NONE', #61081, .T. ) ;
#49698=ORIENTED_EDGE ( 'NONE', *, *, #4260, .F. ) ;
#49700=DIRECTION ( 'NONE',  ( 1.000000000000000000, 0.000000000000000000, -0.000000000000000000 ) ) ;
#49702=CARTESIAN_POINT ( 'NONE',  ( 18.84867683979355846, 5.944105725974518251, 12.12095735156415088 ) ) ;
#49703=DIRECTION ( 'NONE',  ( -0.000000000000000000, -0.000000000000000000, -1.000000000000000000 ) ) ;
#49710=ORIENTED_EDGE ( 'NONE', *, *, #21009, .F. ) ;
#49712=EDGE_CURVE ( 'NONE', #18784, #40821, #55922, .T. ) ;
#49713=ORIENTED_EDGE ( 'NONE', *, *, #30624, .F. ) ;
#49715=VERTEX_POINT ( 'NONE', #1331 ) ;
#49716=ORIENTED_EDGE ( 'NONE', *, *, #64705, .F. ) ;
#49720=DIRECTION ( 'NONE',  ( 0.3628680629012471792, -0.9318405276259971171, 0.000000000000000000 ) ) ;
#49721=CARTESIAN_POINT ( 'NONE',  ( 24.31148382840972033, -1.623357687012453088, 11.89098708344122812 ) ) ;
#49723=CARTESIAN_POINT ( 'NONE',  ( 6.812204945636112896, -4.138731716409435712, 25.00000000000000000 ) ) ;
#49724=EDGE_CURVE ( 'NONE', #59781, #16732, #21260, .T. ) ;
#49726=AXIS2_PLACEMENT_3D ( 'NONE', #47134, #16847, #37123 ) ;
#49728=VERTEX_POINT ( 'NONE', #57182 ) ;
#49729=CARTESIAN_POINT ( 'NONE',  ( -35.00000000000000000, 0.000000000000000000, 0.000000000000000000 ) ) ;
#49730=EDGE_CURVE ( 'NONE', #30664, #26254, #11610, .T. ) ;
#49731=CIRCLE ( 'NONE', #30581, 12.18649999999999878 ) ;
#49734=AXIS2_PLACEMENT_3D ( 'NONE', #26668, #46963, #1421 ) ;
#49738=CARTESIAN_POINT ( 'NONE',  ( -35.00000000000000000, -9.430788938294105250, 7.718225330433773124 ) ) ;
#49741=ORIENTED_EDGE ( 'NONE', *, *, #6747, .T. ) ;
#49744=CARTESIAN_POINT ( 'NONE',  ( 6.812204945636112896, -4.138731716409435712, -12.84993773446340803 ) ) ;
#49746=CARTESIAN_POINT ( 'NONE',  ( 3.347841273039249721, -10.61118957148187825, 25.00000000000000000 ) ) ;
#49748=VECTOR ( 'NONE', #53248, 1000.000000000000000 ) ;
#49749=CARTESIAN_POINT ( 'NONE',  ( 7.219696859909502606, -7.180886164847118280, -11.43374296297836779 ) ) ;
#49754=FACE_OUTER_BOUND ( 'NONE', #35574, .T. ) ;
#49755=CYLINDRICAL_SURFACE ( 'NONE', #64019, 4.999999999999999112 ) ;
#49756=EDGE_CURVE ( 'NONE', #63312, #8204, #58524, .T. ) ;
#49757=CARTESIAN_POINT ( 'NONE',  ( 35.00000000000000000, -12.09831040184922912, 1.463443770872898453 ) ) ;
#49758=AXIS2_PLACEMENT_3D ( 'NONE', #1244, #57419, #6230 ) ;
#49761=AXIS2_PLACEMENT_3D ( 'NONE', #28988, #34920, #9661 ) ;
#49762=AXIS2_PLACEMENT_3D ( 'NONE', #3531, #13461, #34071 ) ;
#49763=ORIENTED_EDGE ( 'NONE', *, *, #14413, .F. ) ;
#49764=CARTESIAN_POINT ( 'NONE',  ( -37.00000000000000711, 12.09831040184926287, -1.463443770872647542 ) ) ;
#49765=CARTESIAN_POINT ( 'NONE',  ( 47.00000000000000711, 4.705694406421931860E-17, -3.469127814946512892E-15 ) ) ;
#49768=DIRECTION ( 'NONE',  ( 0.000000000000000000, -0.01356324068817998940, 0.9999080150203990547 ) ) ;
#49769=CARTESIAN_POINT ( 'NONE',  ( -27.94693092740403273, -13.15284231573790130, -3.100845697411033441 ) ) ;
#49771=EDGE_CURVE ( 'NONE', #3400, #58711, #58161, .T. ) ;
#49772=CIRCLE ( 'NONE', #38081, 5.000000000000001776 ) ;
#49774=B_SPLINE_CURVE_WITH_KNOTS ( 'NONE', 3,
 ( #4900, #61072, #61377, #15819, #35769, #31138, #25162, #20171, #56068, #21146 ),
 .UNSPECIFIED., .F., .F.,
 ( 4, 2, 2, 2, 4 ),
 ( 0.006778809408328222152, 0.007562956181792331208, 0.008347102955256440263, 0.009131249728720550185, 0.009915396502184661842 ),
 .UNSPECIFIED. ) ;
#49776=FACE_OUTER_BOUND ( 'NONE', #49018, .T. ) ;
#49779=CARTESIAN_POINT ( 'NONE',  ( -2.952869152607111136, -4.384817011589735358, 11.17020052527586138 ) ) ;
#49780=CYLINDRICAL_SURFACE ( 'NONE', #35353, 12.75000000000000178 ) ;
#49781=DIRECTION ( 'NONE',  ( -1.000000000000000000, 0.000000000000000000, 0.000000000000000000 ) ) ;
#49783=CARTESIAN_POINT ( 'NONE',  ( 37.00000000000000711, -11.59605747147790211, -5.300372733891605570 ) ) ;
#49784=DIRECTION ( 'NONE',  ( -1.000000000000000000, 0.000000000000000000, -0.000000000000000000 ) ) ;
#49786=EDGE_LOOP ( 'NONE', ( #30473, #471, #47181, #37540 ) ) ;
#49789=ORIENTED_EDGE ( 'NONE', *, *, #57452, .T. ) ;
#49791=ADVANCED_FACE ( 'NONE', ( #37869 ), #17604, .T. ) ;
#49796=ORIENTED_EDGE ( 'NONE', *, *, #13653, .T. ) ;
#49797=CYLINDRICAL_SURFACE ( 'NONE', #3621, 4.999999999999999112 ) ;
#49802=EDGE_LOOP ( 'NONE', ( #4147, #58152, #13022, #52294 ) ) ;
#49805=CARTESIAN_POINT ( 'NONE',  ( 35.00000000000000000, 4.705694406421931860E-17, -3.469127814946512892E-15 ) ) ;
#49806=ORIENTED_EDGE ( 'NONE', *, *, #28150, .F. ) ;
#49808=ORIENTED_EDGE ( 'NONE', *, *, #36983, .T. ) ;
#49813=DIRECTION ( 'NONE',  ( 0.000000000000000000, 0.5472293298355273006, -0.8369827122275342868 ) ) ;
#49814=FACE_OUTER_BOUND ( 'NONE', #5467, .T. ) ;
#49816=ORIENTED_EDGE ( 'NONE', *, *, #12212, .T. ) ;
#49819=DIRECTION ( 'NONE',  ( 0.000000000000000000, -0.8827602140260265573, 0.4698238015817460256 ) ) ;
#49820=DIRECTION ( 'NONE',  ( 0.000000000000000000, -0.4380125133593848474, 0.8989688749565218906 ) ) ;
#49821=CARTESIAN_POINT ( 'NONE',  ( 12.64843508166302399, 11.70598649689469717, -6.727170912064254438 ) ) ;
#49823=CARTESIAN_POINT ( 'NONE',  ( 35.00000000000000000, 10.54834585426228877, 6.102719229070555862 ) ) ;
#49824=CARTESIAN_POINT ( 'NONE',  ( -35.00000000000000000, 0.000000000000000000, 0.000000000000000000 ) ) ;
#49827=ORIENTED_EDGE ( 'NONE', *, *, #56234, .F. ) ;
#49829=EDGE_CURVE ( 'NONE', #64891, #16581, #58493, .T. ) ;
#49830=EDGE_LOOP ( 'NONE', ( #57239, #6433, #10605, #4989 ) ) ;
#49831=DIRECTION ( 'NONE',  ( 0.000000000000000000, 0.01356324068817998940, -0.9999080150203990547 ) ) ;
#49833=DIRECTION ( 'NONE',  ( 1.000000000000000000, -0.000000000000000000, -0.000000000000000000 ) ) ;
#49837=CARTESIAN_POINT ( 'NONE',  ( -27.01437459610461644, 8.723448335974111956, -8.240233560378637634 ) ) ;
#49839=ADVANCED_FACE ( 'NONE', ( #57851 ), #7959, .T. ) ;
#49841=CARTESIAN_POINT ( 'NONE',  ( 35.00000000000000000, 12.49688848680883879, -2.527899948230684313 ) ) ;
#49842=AXIS2_PLACEMENT_3D ( 'NONE', #55889, #61512, #25623 ) ;
#49845=CIRCLE ( 'NONE', #11626, 4.999999999999999112 ) ;
#49846=CARTESIAN_POINT ( 'NONE',  ( 37.00000000000000711, 4.705694406421931860E-17, -3.469127814946512892E-15 ) ) ;
#49847=ORIENTED_EDGE ( 'NONE', *, *, #55303, .F. ) ;
#49849=DIRECTION ( 'NONE',  ( 0.000000000000000000, 0.01356324068817998940, -0.9999080150203989437 ) ) ;
#49850=EDGE_CURVE ( 'NONE', #60788, #32449, #57413, .T. ) ;
#49851=ADVANCED_FACE ( 'NONE', ( #7270 ), #22587, .T. ) ;
#49852=CARTESIAN_POINT ( 'NONE',  ( -2.532614230583026593, -7.965877694534051479, 10.89930238848911337 ) ) ;
#49853=EDGE_CURVE ( 'NONE', #40181, #51873, #64886, .T. ) ;
#49855=AXIS2_PLACEMENT_3D ( 'NONE', #53792, #52492, #13217 ) ;
#49856=ORIENTED_EDGE ( 'NONE', *, *, #59253, .T. ) ;
#49857=ORIENTED_EDGE ( 'NONE', *, *, #59741, .F. ) ;
#49860=CIRCLE ( 'NONE', #51962, 12.75000000000000178 ) ;
#49861=CARTESIAN_POINT ( 'NONE',  ( 35.00000000000000000, -4.603882218679472338, 10.80631716521671493 ) ) ;
#49862=LINE ( 'NONE', #45195, #18357 ) ;
#49867=DIRECTION ( 'NONE',  ( -1.000000000000000000, 0.000000000000000000, 0.000000000000000000 ) ) ;
#49868=VERTEX_POINT ( 'NONE', #3293 ) ;
#49870=VECTOR ( 'NONE', #32515, 1000.000000000000000 ) ;
#49872=B_SPLINE_CURVE_WITH_KNOTS ( 'NONE', 3,
 ( #56640, #6099, #17034, #15706, #41973, #36665, #57284, #21718, #56964, #10732, #29770, #37312, #41647, #11387, #768, #11706 ),
 .UNSPECIFIED., .F., .F.,
 ( 4, 2, 2, 2, 2, 2, 2, 4 ),
 ( 3.878959614448864246E-18, 0.002501164792002928683, 0.003751747188004390856, 0.005002329584005853029, 0.006252911980007317370, 0.007503494376008781712, 0.008754076772010246921, 0.01000465916801171126 ),
 .UNSPECIFIED. ) ;
#49874=EDGE_CURVE ( 'NONE', #15604, #45790, #19257, .T. ) ;
#49875=DIRECTION ( 'NONE',  ( 1.000000000000000000, 0.000000000000000000, 0.000000000000000000 ) ) ;
#49876=ORIENTED_EDGE ( 'NONE', *, *, #5488, .F. ) ;
#49877=EDGE_CURVE ( 'NONE', #2479, #12997, #8616, .T. ) ;
#49878=FACE_BOUND ( 'NONE', #19024, .T. ) ;
#49879=EDGE_LOOP ( 'NONE', ( #11687, #64827, #318, #32607 ) ) ;
#49880=CARTESIAN_POINT ( 'NONE',  ( -36.00000000000000711, 7.745827850123011338, 10.12742074351899468 ) ) ;
#49885=ORIENTED_EDGE ( 'NONE', *, *, #55336, .F. ) ;
#49891=ORIENTED_EDGE ( 'NONE', *, *, #65582, .T. ) ;
#49895=CIRCLE ( 'NONE', #2139, 12.75000000000000178 ) ;
#49897=CARTESIAN_POINT ( 'NONE',  ( 37.00000000000000711, 3.340853584269691368, 11.26103545359851665 ) ) ;
#49902=FACE_OUTER_BOUND ( 'NONE', #11826, .T. ) ;
#49903=DIRECTION ( 'NONE',  ( 1.000000000000000000, 0.000000000000000000, 0.000000000000000000 ) ) ;
#49904=ORIENTED_EDGE ( 'NONE', *, *, #20332, .T. ) ;
#49912=VECTOR ( 'NONE', #45345, 1000.000000000000000 ) ;
#49914=( BOUNDED_CURVE ( )  B_SPLINE_CURVE ( 3, ( #18975, #39571, #59874, #29582 ),
 .UNSPECIFIED., .F., .F. ) 
 B_SPLINE_CURVE_WITH_KNOTS ( ( 4, 4 ),
 ( 5.331207651931955560, 5.369882018696277015 ),
 .UNSPECIFIED. ) 
 CURVE ( )  GEOMETRIC_REPRESENTATION_ITEM ( )  RATIONAL_B_SPLINE_CURVE ( ( 1.000000000000000000, 0.9998753616634872277, 0.9998753616634872277, 1.000000000000000000 ) ) 
 REPRESENTATION_ITEM ( '' )  );
#49915=ORIENTED_EDGE ( 'NONE', *, *, #25509, .F. ) ;
#49917=DIRECTION ( 'NONE',  ( -1.000000000000000000, -0.000000000000000000, -0.000000000000000000 ) ) ;
#49919=CARTESIAN_POINT ( 'NONE',  ( -3.358052903796875377, 10.43609928815077126, 5.926952491707684345 ) ) ;
#49920=DIRECTION ( 'NONE',  ( 1.000000000000000000, 0.000000000000000000, 0.000000000000000000 ) ) ;
#49922=AXIS2_PLACEMENT_3D ( 'NONE', #2296, #38167, #23220 ) ;
#49923=DIRECTION ( 'NONE',  ( 0.000000000000000000, -0.2355298848897378339, -0.9718671068226493182 ) ) ;
#49927=DIRECTION ( 'NONE',  ( 1.000000000000000000, 0.000000000000000000, 0.000000000000000000 ) ) ;
#49929=EDGE_CURVE ( 'NONE', #56844, #58552, #36228, .T. ) ;
#49930=CARTESIAN_POINT ( 'NONE',  ( -36.00000000000000711, -8.830544224262881770, -9.196955404009390378 ) ) ;
#49931=DIRECTION ( 'NONE',  ( 0.000000000000000000, -0.01356324068817991828, 0.9999080150203990547 ) ) ;
#49932=AXIS2_PLACEMENT_3D ( 'NONE', #47627, #48957, #37966 ) ;
#49933=CIRCLE ( 'NONE', #21259, 5.000000000000000000 ) ;
#49934=EDGE_LOOP ( 'NONE', ( #61896, #29918, #55365, #52518 ) ) ;
#49935=CARTESIAN_POINT ( 'NONE',  ( 35.00000000000000000, 4.705694406421931860E-17, -3.469127814946512892E-15 ) ) ;
#49936=ORIENTED_EDGE ( 'NONE', *, *, #34613, .F. ) ;
#49938=PLANE ( 'NONE',  #9901 ) ;
#49939=CARTESIAN_POINT ( 'NONE',  ( -37.00000000000000711, 0.000000000000000000, 0.000000000000000000 ) ) ;
#49940=CARTESIAN_POINT ( 'NONE',  ( -36.00000000000000711, 12.71517666308949579, -0.9416912585473031783 ) ) ;
#49941=ORIENTED_EDGE ( 'NONE', *, *, #52766, .F. ) ;
#49942=EDGE_LOOP ( 'NONE', ( #25169, #37730, #57201, #18944 ) ) ;
#49943=ORIENTED_EDGE ( 'NONE', *, *, #63381, .F. ) ;
#49946=EDGE_CURVE ( 'NONE', #24268, #7657, #46996, .T. ) ;
#49947=CARTESIAN_POINT ( 'NONE',  ( -35.00000000000000000, 11.26103545359856106, -3.340853584269573684 ) ) ;
#49950=CARTESIAN_POINT ( 'NONE',  ( -36.00000000000000711, 12.38385022362082033, 3.033604067594622755 ) ) ;
#49951=CIRCLE ( 'NONE', #58456, 4.999999999999998224 ) ;
#49952=DIRECTION ( 'NONE',  ( -1.000000000000000000, -0.000000000000000000, 0.000000000000000000 ) ) ;
#49954=ORIENTED_EDGE ( 'NONE', *, *, #52505, .F. ) ;
#49955=PLANE ( 'NONE',  #55377 ) ;
#49957=DIRECTION ( 'NONE',  ( -1.000000000000000000, 0.000000000000000000, 0.000000000000000000 ) ) ;
#49958=CARTESIAN_POINT ( 'NONE',  ( 37.00000000000000711, 4.705694406421931860E-17, -3.469127814946512892E-15 ) ) ;
#49959=ORIENTED_EDGE ( 'NONE', *, *, #2492, .F. ) ;
#49960=CARTESIAN_POINT ( 'NONE',  ( -36.00000000000000711, 8.954052073409602741, 9.076753354954030684 ) ) ;
#49963=CIRCLE ( 'NONE', #21286, 12.74999999999999822 ) ;
#49967=CYLINDRICAL_SURFACE ( 'NONE', #37231, 5.000000000000000888 ) ;
#49969=EDGE_CURVE ( 'NONE', #14515, #6027, #54292, .T. ) ;
#49970=CARTESIAN_POINT ( 'NONE',  ( 35.00000000000000000, 4.705694406421931860E-17, -3.469127814946512892E-15 ) ) ;
#49971=CARTESIAN_POINT ( 'NONE',  ( -10.74958689447668014, -6.108794307151256042, -12.04558683403140940 ) ) ;
#49972=DIRECTION ( 'NONE',  ( 1.000000000000000000, 0.000000000000000000, -0.000000000000000000 ) ) ;
#49974=ORIENTED_EDGE ( 'NONE', *, *, #64560, .F. ) ;
#49975=AXIS2_PLACEMENT_3D ( 'NONE', #56776, #46767, #1228 ) ;
#49977=CARTESIAN_POINT ( 'NONE',  ( 13.35499959353619914, -12.72359730182141568, -4.517647836983113230 ) ) ;
#49984=CARTESIAN_POINT ( 'NONE',  ( -35.00000000000000000, -9.060822531526103063, 7.474872387600973944 ) ) ;
#49985=DIRECTION ( 'NONE',  ( 0.000000000000000000, -0.9987865678893281807, 0.04924826701373505311 ) ) ;
#49986=CARTESIAN_POINT ( 'NONE',  ( -37.00000000000000711, -0.4871980014162358152, 12.74068829017553739 ) ) ;
#49987=VECTOR ( 'NONE', #4294, 1000.000000000000000 ) ;
#49988=AXIS2_PLACEMENT_3D ( 'NONE', #34528, #64769, #43862 ) ;
#49990=FACE_OUTER_BOUND ( 'NONE', #24506, .T. ) ;
#49993=VERTEX_POINT ( 'NONE', #29207 ) ;
#49994=DIRECTION ( 'NONE',  ( -1.000000000000000000, -0.000000000000000000, 0.000000000000000000 ) ) ;
#49996=ADVANCED_FACE ( 'NONE', ( #60111 ), #44165, .T. ) ;
#49997=CARTESIAN_POINT ( 'NONE',  ( -35.00000000000000000, 7.717887834988368390, -8.854740511458771834 ) ) ;
#49998=EDGE_LOOP ( 'NONE', ( #4995, #35729, #15522, #33715 ) ) ;
#49999=AXIS2_PLACEMENT_3D ( 'NONE', #8408, #64902, #24041 ) ;
#50002=AXIS2_PLACEMENT_3D ( 'NONE', #56827, #36521, #37829 ) ;
#50003=CARTESIAN_POINT ( 'NONE',  ( -7.154245469367370269, -1.341795249608957130, 13.43334531127548281 ) ) ;
#50005=CYLINDRICAL_SURFACE ( 'NONE', #60718, 4.999999999999999112 ) ;
#50007=EDGE_LOOP ( 'NONE', ( #19195, #521, #65466, #14937 ) ) ;
#50010=CARTESIAN_POINT ( 'NONE',  ( 3.899688111913728772, 7.685012310942984648, 9.227363078734208912 ) ) ;
#50012=EDGE_CURVE ( 'NONE', #24413, #12853, #9888, .T. ) ;
#50013=DIRECTION ( 'NONE',  ( -0.000000000000000000, -1.000000000000000000, -0.000000000000000000 ) ) ;
#50014=CARTESIAN_POINT ( 'NONE',  ( 36.00000000000000711, -8.017674001891711200, 9.913596905230193101 ) ) ;
#50015=AXIS2_PLACEMENT_3D ( 'NONE', #9072, #49648, #65257 ) ;
#50016=ORIENTED_EDGE ( 'NONE', *, *, #22350, .T. ) ;
#50017=DIRECTION ( 'NONE',  ( -1.000000000000000000, 0.000000000000000000, -0.000000000000000000 ) ) ;
#50018=CARTESIAN_POINT ( 'NONE',  ( -9.257124744190798893, -8.325323762313093567, -8.651777918013287660 ) ) ;
#50021=DIRECTION ( 'NONE',  ( 1.000000000000000000, 0.000000000000000000, 0.000000000000000000 ) ) ;
#50022=AXIS2_PLACEMENT_3D ( 'NONE', #19443, #10107, #14102 ) ;
#50023=CARTESIAN_POINT ( 'NONE',  ( 36.00000000000000711, -12.31350058095520339, 3.307597835713371737 ) ) ;
#50024=ORIENTED_EDGE ( 'NONE', *, *, #31666, .F. ) ;
#50025=ORIENTED_EDGE ( 'NONE', *, *, #3424, .F. ) ;
#50026=VERTEX_POINT ( 'NONE', #20196 ) ;
#50027=VECTOR ( 'NONE', #25803, 1000.000000000000000 ) ;
#50028=VECTOR ( 'NONE', #28165, 1000.000000000000000 ) ;
#50031=DIRECTION ( 'NONE',  ( -1.000000000000000000, -0.000000000000000000, 0.000000000000000000 ) ) ;
#50033=CARTESIAN_POINT ( 'NONE',  ( 37.00000000000000711, 4.705694406421931860E-17, -3.469127814946512892E-15 ) ) ;
#50034=AXIS2_PLACEMENT_3D ( 'NONE', #19070, #2483, #64593 ) ;
#50036=CARTESIAN_POINT ( 'NONE',  ( 35.00000000000000000, 4.705694406421931860E-17, -3.469127814946512892E-15 ) ) ;
#50037=DIRECTION ( 'NONE',  ( 0.2180658516479614395, -0.9759340573753174652, 0.000000000000000000 ) ) ;
#50038=VERTEX_POINT ( 'NONE', #60770 ) ;
#50039=DIRECTION ( 'NONE',  ( -1.000000000000000000, 0.000000000000000000, -0.000000000000000000 ) ) ;
#50042=VERTEX_POINT ( 'NONE', #35488 ) ;
#50043=ORIENTED_EDGE ( 'NONE', *, *, #2408, .F. ) ;
#50047=DIRECTION ( 'NONE',  ( 0.000000000000000000, -0.9970832820307030664, -0.07632122047557565736 ) ) ;
#50049=AXIS2_PLACEMENT_3D ( 'NONE', #25302, #30, #54909 ) ;
#50051=CARTESIAN_POINT ( 'NONE',  ( 35.00000000000000000, 4.705694406421931860E-17, -3.469127814946512892E-15 ) ) ;
#50052=CARTESIAN_POINT ( 'NONE',  ( 35.00000000000000000, -11.90598845858536770, -4.561791185930372805 ) ) ;
#50053=CIRCLE ( 'NONE', #13902, 4.999999999999999112 ) ;
#50054=ORIENTED_EDGE ( 'NONE', *, *, #44712, .T. ) ;
#50055=AXIS2_PLACEMENT_3D ( 'NONE', #24048, #33366, #7772 ) ;
#50058=ORIENTED_EDGE ( 'NONE', *, *, #40785, .T. ) ;
#50059=AXIS2_PLACEMENT_3D ( 'NONE', #58979, #2796, #39307 ) ;
#50062=CARTESIAN_POINT ( 'NONE',  ( 35.00000000000000000, 11.37311665002363270, 2.936739658819908616 ) ) ;
#50064=CARTESIAN_POINT ( 'NONE',  ( 16.92262867437927198, -9.930101274560646729, 6.758629725180155035 ) ) ;
#50066=CARTESIAN_POINT ( 'NONE',  ( -11.40165637463000436, -7.508992741355388745, -9.360289953322599388 ) ) ;
#50069=ORIENTED_EDGE ( 'NONE', *, *, #32600, .T. ) ;
#50071=EDGE_LOOP ( 'NONE', ( #45205, #8124, #9427, #37963 ) ) ;
#50072=AXIS2_PLACEMENT_3D ( 'NONE', #12721, #2795, #38325 ) ;
#50073=AXIS2_PLACEMENT_3D ( 'NONE', #14580, #54851, #29555 ) ;
#50075=LINE ( 'NONE', #30745, #10496 ) ;
#50077=CARTESIAN_POINT ( 'NONE',  ( 37.00000000000000711, 8.352657516904789858, 8.258652103341336925 ) ) ;
#50078=CIRCLE ( 'NONE', #9716, 12.75000000000000178 ) ;
#50079=AXIS2_PLACEMENT_3D ( 'NONE', #5863, #4866, #26119 ) ;
#50081=DIRECTION ( 'NONE',  ( -1.000000000000000000, 0.000000000000000000, 0.000000000000000000 ) ) ;
#50082=EDGE_CURVE ( 'NONE', #29886, #48262, #3375, .T. ) ;
#50083=CARTESIAN_POINT ( 'NONE',  ( 7.118931388086720879, -4.897740429628226089, -12.58727760722467259 ) ) ;
#50084=ADVANCED_FACE ( 'NONE', ( #46451 ), #51130, .T. ) ;
#50085=CARTESIAN_POINT ( 'NONE',  ( -37.00000000000000711, 5.644643009979071202, 10.30098186818251982 ) ) ;
#50086=DIRECTION ( 'NONE',  ( 1.000000000000000000, 0.000000000000000000, 0.000000000000000000 ) ) ;
#50087=DIRECTION ( 'NONE',  ( -1.000000000000000000, -0.000000000000000000, 0.000000000000000000 ) ) ;
#50088=VERTEX_POINT ( 'NONE', #45803 ) ;
#50090=CARTESIAN_POINT ( 'NONE',  ( 17.27839441901508977, 12.20388373500084711, 5.771933972472493402 ) ) ;
#50091=LINE ( 'NONE', #49757, #20617 ) ;
#50092=EDGE_CURVE ( 'NONE', #42734, #52455, #33049, .T. ) ;
#50093=VECTOR ( 'NONE', #14766, 1000.000000000000000 ) ;
#50097=CARTESIAN_POINT ( 'NONE',  ( -28.12637923985837674, -10.04112151140785691, -6.578508732650774071 ) ) ;
#50099=ORIENTED_EDGE ( 'NONE', *, *, #38027, .T. ) ;
#50100=DIRECTION ( 'NONE',  ( 1.000000000000000000, 0.000000000000000000, 0.000000000000000000 ) ) ;
#50107=AXIS2_PLACEMENT_3D ( 'NONE', #20460, #55715, #51053 ) ;
#50108=DIRECTION ( 'NONE',  ( -0.000000000000000000, -0.000000000000000000, -1.000000000000000000 ) ) ;
#50109=CARTESIAN_POINT ( 'NONE',  ( -9.824684730204651828, -11.82156200828225145, -6.531049348231868557 ) ) ;
#50110=CARTESIAN_POINT ( 'NONE',  ( 35.00000000000000000, 1.488153103996963100, -11.65150730582935523 ) ) ;
#50111=EDGE_LOOP ( 'NONE', ( #4606, #64169, #12671, #13995, #6359, #9752 ) ) ;
#50113=AXIS2_PLACEMENT_3D ( 'NONE', #41713, #11141, #37714 ) ;
#50115=CARTESIAN_POINT ( 'NONE',  ( -17.47051625687515397, 7.643161633986498948, -11.12960797627961007 ) ) ;
#50116=CARTESIAN_POINT ( 'NONE',  ( 9.382205902475009296, 7.259643443602203483, -11.38652836844183369 ) ) ;
#50118=CARTESIAN_POINT ( 'NONE',  ( 35.00000000000000000, -11.70009620280412399, -1.039216533672868481 ) ) ;
#50119=FACE_OUTER_BOUND ( 'NONE', #2630, .T. ) ;
#50122=EDGE_LOOP ( 'NONE', ( #39009, #2059, #25431, #58136 ) ) ;
#50128=EDGE_CURVE ( 'NONE', #54202, #16892, #20535, .T. ) ;
#50129=AXIS2_PLACEMENT_3D ( 'NONE', #56870, #35234, #30573 ) ;
#50131=AXIS2_PLACEMENT_3D ( 'NONE', #4473, #50673, #29705 ) ;
#50132=ORIENTED_EDGE ( 'NONE', *, *, #49850, .F. ) ;
#50133=CARTESIAN_POINT ( 'NONE',  ( -35.00000000000000000, 12.01765980939845058, -2.021542716731266065 ) ) ;
#50134=CARTESIAN_POINT ( 'NONE',  ( 10.35219383903665857, 11.93001091997956919, -1.309405142360217544 ) ) ;
#50135=DIRECTION ( 'NONE',  ( 0.000000000000000000, 0.01356324068817998940, -0.9999080150203990547 ) ) ;
#50138=DIRECTION ( 'NONE',  ( 1.000000000000000000, 0.000000000000000000, 0.000000000000000000 ) ) ;
#50139=ADVANCED_FACE ( 'NONE', ( #11212 ), #31487, .T. ) ;
#50140=VERTEX_POINT ( 'NONE', #46780 ) ;
#50143=AXIS2_PLACEMENT_3D ( 'NONE', #44983, #34008, #4093 ) ;
#50144=DIRECTION ( 'NONE',  ( -1.000000000000000000, -0.000000000000000000, 0.000000000000000000 ) ) ;
#50146=AXIS2_PLACEMENT_3D ( 'NONE', #63567, #8072, #18386 ) ;
#50149=EDGE_CURVE ( 'NONE', #26657, #64905, #53798, .T. ) ;
#50153=CARTESIAN_POINT ( 'NONE',  ( -17.96188634106787063, 6.007102645581881895, 10.39092871488517389 ) ) ;
#50156=EDGE_CURVE ( 'NONE', #4686, #23899, #42572, .T. ) ;
#50157=CARTESIAN_POINT ( 'NONE',  ( 35.00000000000000000, 8.258652103341434625, -8.352657516904704593 ) ) ;
#50159=CARTESIAN_POINT ( 'NONE',  ( 23.75066733795811658, -3.115628287466211344, 13.13955084818059404 ) ) ;
#50160=CARTESIAN_POINT ( 'NONE',  ( -35.00000000000000000, 12.16632754454237819, -0.7008968033237440443 ) ) ;
#50161=CYLINDRICAL_SURFACE ( 'NONE', #33393, 12.18649999999999878 ) ;
#50163=ORIENTED_EDGE ( 'NONE', *, *, #9030, .T. ) ;
#50164=CARTESIAN_POINT ( 'NONE',  ( -17.08774245407508019, 7.933722547746723919, -9.005484594861211889 ) ) ;
#50165=CIRCLE ( 'NONE', #21489, 12.75000000000000178 ) ;
#50167=DIRECTION ( 'NONE',  ( 1.000000000000000000, 0.000000000000000000, 0.000000000000000000 ) ) ;
#50169=ADVANCED_FACE ( 'NONE', ( #21855 ), #31795, .T. ) ;
#50170=DIRECTION ( 'NONE',  ( -1.000000000000000000, 0.000000000000000000, 0.000000000000000000 ) ) ;
#50171=DIRECTION ( 'NONE',  ( 0.000000000000000000, -0.01356324068817991828, 0.9999080150203990547 ) ) ;
#50172=CARTESIAN_POINT ( 'NONE',  ( 35.00000000000000000, 8.235637554476779698, 9.733281772932071974 ) ) ;
#50173=EDGE_CURVE ( 'NONE', #43014, #36640, #51109, .T. ) ;
#50177=CARTESIAN_POINT ( 'NONE',  ( 10.28253184321369140, 1.474010143406270679, 11.91011122907010922 ) ) ;
#50179=EDGE_CURVE ( 'NONE', #44827, #55595, #22418, .T. ) ;
#50180=AXIS2_PLACEMENT_3D ( 'NONE', #19107, #28750, #23787 ) ;
#50181=CIRCLE ( 'NONE', #62880, 5.000000000000000000 ) ;
#50183=DIRECTION ( 'NONE',  ( -1.000000000000000000, -0.000000000000000000, -0.000000000000000000 ) ) ;
#50184=ORIENTED_EDGE ( 'NONE', *, *, #33585, .F. ) ;
#50187=ORIENTED_EDGE ( 'NONE', *, *, #20161, .F. ) ;
#50188=DIRECTION ( 'NONE',  ( -1.000000000000000000, -0.000000000000000000, 0.000000000000000000 ) ) ;
#50191=VECTOR ( 'NONE', #41099, 1000.000000000000000 ) ;
#50192=CYLINDRICAL_SURFACE ( 'NONE', #53263, 5.000000000000002665 ) ;
#50197=ORIENTED_EDGE ( 'NONE', *, *, #387, .F. ) ;
#50198=CYLINDRICAL_SURFACE ( 'NONE', #24532, 5.000000000000000888 ) ;
#50199=CARTESIAN_POINT ( 'NONE',  ( 37.00000000000000711, 4.705694406421931860E-17, -3.469127814946512892E-15 ) ) ;
#50200=AXIS2_PLACEMENT_3D ( 'NONE', #65472, #60492, #19935 ) ;
#50201=CARTESIAN_POINT ( 'NONE',  ( 35.00000000000000000, -9.926225166346981155, 6.280308599560240346 ) ) ;
#50202=LINE ( 'NONE', #19923, #36437 ) ;
#50203=CARTESIAN_POINT ( 'NONE',  ( 35.00000000000000000, 4.705694406421931860E-17, -3.469127814946512892E-15 ) ) ;
#50204=AXIS2_PLACEMENT_3D ( 'NONE', #53155, #3630, #43484 ) ;
#50205=LINE ( 'NONE', #28033, #32786 ) ;
#50207=ORIENTED_EDGE ( 'NONE', *, *, #61651, .T. ) ;
#50215=AXIS2_PLACEMENT_3D ( 'NONE', #17189, #37465, #62090 ) ;
#50216=DIRECTION ( 'NONE',  ( -0.6334066780386838902, 0.000000000000000000, -0.7738190875236917732 ) ) ;
#50219=DIRECTION ( 'NONE',  ( 0.000000000000000000, -0.01356324068817998767, 0.9999080150203990547 ) ) ;
#50220=CARTESIAN_POINT ( 'NONE',  ( 37.00000000000000711, 4.705694406421931860E-17, -3.469127814946512892E-15 ) ) ;
#50221=FACE_OUTER_BOUND ( 'NONE', #484, .T. ) ;
#50222=CARTESIAN_POINT ( 'NONE',  ( 6.320217901527452220, -9.250799897007995654, 7.654551209031711601 ) ) ;
#50223=EDGE_LOOP ( 'NONE', ( #29031, #23488, #38630, #10455 ) ) ;
#50225=CARTESIAN_POINT ( 'NONE',  ( -36.00000000000000711, 12.46157735505193109, -2.696588552978925524 ) ) ;
#50226=ORIENTED_EDGE ( 'NONE', *, *, #57277, .T. ) ;
#50228=EDGE_LOOP ( 'NONE', ( #3595, #50471, #26965, #54543 ) ) ;
#50230=EDGE_CURVE ( 'NONE', #45140, #62469, #1891, .T. ) ;
#50232=ORIENTED_EDGE ( 'NONE', *, *, #64302, .T. ) ;
#50233=VERTEX_POINT ( 'NONE', #7189 ) ;
#50234=CARTESIAN_POINT ( 'NONE',  ( -36.00000000000000711, 0.4871980014163243000, -12.74068829017553561 ) ) ;
#50236=CARTESIAN_POINT ( 'NONE',  ( 35.00000000000000000, -10.80631716521670427, -4.603882218679513194 ) ) ;
#50237=CARTESIAN_POINT ( 'NONE',  ( -37.00000000000000711, 5.927257550915472351, -10.64792938439748937 ) ) ;
#50238=VERTEX_POINT ( 'NONE', #53082 ) ;
#50239=CARTESIAN_POINT ( 'NONE',  ( -35.00000000000000000, -1.791059740004510070, 12.05416472667165273 ) ) ;
#50240=ORIENTED_EDGE ( 'NONE', *, *, #48689, .T. ) ;
#50241=CYLINDRICAL_SURFACE ( 'NONE', #64606, 12.18649999999999878 ) ;
#50243=EDGE_CURVE ( 'NONE', #57170, #5815, #28832, .T. ) ;
#50244=ORIENTED_EDGE ( 'NONE', *, *, #39001, .F. ) ;
#50246=AXIS2_PLACEMENT_3D ( 'NONE', #5524, #21107, #41384 ) ;
#50252=ORIENTED_EDGE ( 'NONE', *, *, #17449, .T. ) ;
#50254=CARTESIAN_POINT ( 'NONE',  ( -37.00000000000000711, -11.86701198550358427, 2.772148766916072926 ) ) ;
#50256=FACE_OUTER_BOUND ( 'NONE', #40808, .T. ) ;
#50257=DIRECTION ( 'NONE',  ( 1.000000000000000000, 0.000000000000000000, 0.000000000000000000 ) ) ;
#50258=CARTESIAN_POINT ( 'NONE',  ( -37.00000000000000711, 0.000000000000000000, 0.000000000000000000 ) ) ;
#50261=DIRECTION ( 'NONE',  ( 0.000000000000000000, 0.3807014730195152907, -0.9246979985058750851 ) ) ;
#50264=EDGE_CURVE ( 'NONE', #37599, #45626, #22159, .T. ) ;
#50266=EDGE_CURVE ( 'NONE', #34038, #10268, #38100, .T. ) ;
#50271=LINE ( 'NONE', #49930, #52736 ) ;
#50273=CIRCLE ( 'NONE', #37481, 5.000000000000000000 ) ;
#50274=CIRCLE ( 'NONE', #13096, 12.74999999999999822 ) ;
#50277=EDGE_CURVE ( 'NONE', #21283, #3374, #40502, .T. ) ;
#50279=LINE ( 'NONE', #34619, #39527 ) ;
#50280=EDGE_LOOP ( 'NONE', ( #17055, #36617, #48429, #29786 ) ) ;
#50284=AXIS2_PLACEMENT_3D ( 'NONE', #47232, #15945, #56544 ) ;
#50287=EDGE_LOOP ( 'NONE', ( #10894, #3137, #24864, #60832 ) ) ;
#50288=AXIS2_PLACEMENT_3D ( 'NONE', #1358, #41901, #50907 ) ;
#50289=VERTEX_POINT ( 'NONE', #43760 ) ;
#50290=ORIENTED_EDGE ( 'NONE', *, *, #25982, .F. ) ;
#50291=CARTESIAN_POINT ( 'NONE',  ( -10.90165637462999904, -7.508992741355383416, -9.360289953322597611 ) ) ;
#50294=VERTEX_POINT ( 'NONE', #57765 ) ;
#50295=DIRECTION ( 'NONE',  ( 1.000000000000000000, 0.000000000000000000, 0.000000000000000000 ) ) ;
#50296=CARTESIAN_POINT ( 'NONE',  ( 35.00000000000000000, 4.705694406421931860E-17, -3.469127814946512892E-15 ) ) ;
#50298=EDGE_CURVE ( 'NONE', #15913, #45235, #64942, .T. ) ;
#50300=CARTESIAN_POINT ( 'NONE',  ( 35.00000000000000000, -9.060822531525994705, 7.474872387601095625 ) ) ;
#50301=AXIS2_PLACEMENT_3D ( 'NONE', #19651, #39909, #60191 ) ;
#50303=CYLINDRICAL_SURFACE ( 'NONE', #10111, 6.595312090839647645 ) ;
#50304=CARTESIAN_POINT ( 'NONE',  ( 35.00000000000000000, 11.39945968423471356, -5.710938531231753323 ) ) ;
#50306=CARTESIAN_POINT ( 'NONE',  ( -36.00000000000000711, 11.01837265713082203, -6.415447294506590126 ) ) ;
#50308=CYLINDRICAL_SURFACE ( 'NONE', #33710, 4.999999999999999112 ) ;
#50309=ORIENTED_EDGE ( 'NONE', *, *, #37159, .F. ) ;
#50310=CARTESIAN_POINT ( 'NONE',  ( -29.14105348823734687, 1.985002961251433051, -11.86469874868790519 ) ) ;
#50312=DIRECTION ( 'NONE',  ( 1.000000000000000000, -0.000000000000000000, 0.000000000000000000 ) ) ;
#50313=DIRECTION ( 'NONE',  ( -1.000000000000000000, 0.000000000000000000, 0.000000000000000000 ) ) ;
#50315=CIRCLE ( 'NONE', #2571, 4.999999999999999112 ) ;
#50316=DIRECTION ( 'NONE',  ( -1.000000000000000000, -0.000000000000000000, -0.000000000000000000 ) ) ;
#50319=LINE ( 'NONE', #25346, #10943 ) ;
#50321=ORIENTED_EDGE ( 'NONE', *, *, #53318, .T. ) ;
#50323=( BOUNDED_CURVE ( )  B_SPLINE_CURVE ( 3, ( #49208, #3664, #63471, #17942 ),
 .UNSPECIFIED., .F., .F. ) 
 B_SPLINE_CURVE_WITH_KNOTS ( ( 4, 4 ),
 ( 3.730491548985638506, 3.779698989410085197 ),
 .UNSPECIFIED. ) 
 CURVE ( )  GEOMETRIC_REPRESENTATION_ITEM ( )  RATIONAL_B_SPLINE_CURVE ( ( 1.000000000000000000, 0.9997982291625954199, 0.9997982291625954199, 1.000000000000000000 ) ) 
 REPRESENTATION_ITEM ( '' )  );
#50325=CARTESIAN_POINT ( 'NONE',  ( 12.10998784662220729, -10.46621227226782835, -8.526922110106905706 ) ) ;
#50326=ORIENTED_EDGE ( 'NONE', *, *, #47180, .T. ) ;
#50327=ADVANCED_FACE ( 'NONE', ( #28458 ), #48760, .T. ) ;
#50328=VECTOR ( 'NONE', #25293, 1000.000000000000000 ) ;
#50329=ORIENTED_EDGE ( 'NONE', *, *, #40282, .F. ) ;
#50331=AXIS2_PLACEMENT_3D ( 'NONE', #21423, #36384, #6141 ) ;
#50332=DIRECTION ( 'NONE',  ( 0.000000000000000000, 0.5243256840888561587, 0.8515178078024868702 ) ) ;
#50333=CARTESIAN_POINT ( 'NONE',  ( -35.00000000000000000, 10.80478261802190154, -5.636262487437199376 ) ) ;
#50335=LINE ( 'NONE', #4785, #63522 ) ;
#50336=EDGE_CURVE ( 'NONE', #17474, #17695, #24134, .T. ) ;
#50337=CIRCLE ( 'NONE', #29097, 12.18650000000000055 ) ;
#50338=CYLINDRICAL_SURFACE ( 'NONE', #19192, 12.75000000000000178 ) ;
#50339=DIRECTION ( 'NONE',  ( -1.000000000000000000, -0.000000000000000000, 0.000000000000000000 ) ) ;
#50340=ORIENTED_EDGE ( 'NONE', *, *, #50456, .T. ) ;
#50343=DIRECTION ( 'NONE',  ( 0.4622435816439414147, -0.000000000000000000, 0.8867529933577789070 ) ) ;
#50346=VECTOR ( 'NONE', #55735, 1000.000000000000000 ) ;
#50348=CIRCLE ( 'NONE', #29069, 12.75000000000000178 ) ;
#50351=DIRECTION ( 'NONE',  ( 0.000000000000000000, -0.1740410799127686259, -0.9847383929261604996 ) ) ;
#50355=FACE_OUTER_BOUND ( 'NONE', #56225, .T. ) ;
#50356=CARTESIAN_POINT ( 'NONE',  ( 3.780834652287974773, 8.352030633203074927, 8.616471685210687070 ) ) ;
#50358=CIRCLE ( 'NONE', #34434, 5.000000000000000888 ) ;
#50359=DIRECTION ( 'NONE',  ( 0.000000000000000000, 0.01356324068817992175, -0.9999080150203990547 ) ) ;
#50364=CARTESIAN_POINT ( 'NONE',  ( 37.00000000000000711, -4.074242145636093326, -12.08151691381188719 ) ) ;
#50366=CARTESIAN_POINT ( 'NONE',  ( 21.63471773768895190, 12.68614566336015947, -4.633447873545391893 ) ) ;
#50367=DIRECTION ( 'NONE',  ( -1.000000000000000000, 0.000000000000000000, -0.000000000000000000 ) ) ;
#50368=ORIENTED_EDGE ( 'NONE', *, *, #45260, .F. ) ;
#50371=ORIENTED_EDGE ( 'NONE', *, *, #32404, .T. ) ;
#50373=DIRECTION ( 'NONE',  ( 1.000000000000000000, -0.000000000000000000, 0.000000000000000000 ) ) ;
#50375=CARTESIAN_POINT ( 'NONE',  ( -35.00000000000000000, 0.000000000000000000, 0.000000000000000000 ) ) ;
#50377=EDGE_CURVE ( 'NONE', #36681, #53717, #58621, .T. ) ;
#50380=CARTESIAN_POINT ( 'NONE',  ( -37.00000000000000711, -6.753013023069787124, 10.14433819232432477 ) ) ;
#50381=ORIENTED_EDGE ( 'NONE', *, *, #18479, .F. ) ;
#50382=EDGE_CURVE ( 'NONE', #57089, #19062, #8669, .T. ) ;
#50384=ORIENTED_EDGE ( 'NONE', *, *, #62965, .F. ) ;
#50386=VECTOR ( 'NONE', #20052, 1000.000000000000000 ) ;
#50387=ORIENTED_EDGE ( 'NONE', *, *, #24873, .T. ) ;
#50388=EDGE_LOOP ( 'NONE', ( #17989, #40774, #6049, #37108 ) ) ;
#50391=VECTOR ( 'NONE', #11274, 1000.000000000000000 ) ;
#50395=CARTESIAN_POINT ( 'NONE',  ( -19.02967556479663713, 11.99999999999999645, 1.585036030062028271E-15 ) ) ;
#50397=VERTEX_POINT ( 'NONE', #20124 ) ;
#50399=DIRECTION ( 'NONE',  ( 0.000000000000000000, 0.01356324068817998940, -0.9999080150203990547 ) ) ;
#50400=ORIENTED_EDGE ( 'NONE', *, *, #48586, .F. ) ;
#50401=ADVANCED_FACE ( 'NONE', ( #4526 ), #3558, .T. ) ;
#50402=ORIENTED_EDGE ( 'NONE', *, *, #31797, .T. ) ;
#50403=FACE_OUTER_BOUND ( 'NONE', #42949, .T. ) ;
#50406=CARTESIAN_POINT ( 'NONE',  ( 18.68377751299183132, 2.160179296860150977, 11.81608574661026978 ) ) ;
#50408=CARTESIAN_POINT ( 'NONE',  ( -11.08198513529404394, -5.470473237785703269, -10.68265194728579282 ) ) ;
#50409=AXIS2_PLACEMENT_3D ( 'NONE', #61838, #36579, #56881 ) ;
#50414=CIRCLE ( 'NONE', #59953, 12.74999999999999822 ) ;
#50419=AXIS2_PLACEMENT_3D ( 'NONE', #55384, #25790, #15137 ) ;
#50420=LINE ( 'NONE', #56365, #63818 ) ;
#50423=VERTEX_POINT ( 'NONE', #29437 ) ;
#50424=VECTOR ( 'NONE', #20283, 1000.000000000000000 ) ;
#50425=CARTESIAN_POINT ( 'NONE',  ( 35.00000000000000000, 7.499679039484058229, -9.040300684349723781 ) ) ;
#50426=CARTESIAN_POINT ( 'NONE',  ( 17.70433014606954103, 10.91857155134370494, 7.947521937489286259 ) ) ;
#50427=CARTESIAN_POINT ( 'NONE',  ( 35.00000000000000000, 10.92721691015455754, -4.309077947445693724 ) ) ;
#50428=CIRCLE ( 'NONE', #30243, 12.18650000000000055 ) ;
#50430=DIRECTION ( 'NONE',  ( -1.000000000000000000, 0.000000000000000000, 0.000000000000000000 ) ) ;
#50431=CYLINDRICAL_SURFACE ( 'NONE', #8582, 4.999999999999999112 ) ;
#50432=VERTEX_POINT ( 'NONE', #49738 ) ;
#50436=ORIENTED_EDGE ( 'NONE', *, *, #49, .F. ) ;
#50437=DIRECTION ( 'NONE',  ( -1.000000000000000000, 0.000000000000000000, 0.000000000000000000 ) ) ;
#50440=CARTESIAN_POINT ( 'NONE',  ( -35.00000000000000000, 3.827046518385245122, -11.56998259273173701 ) ) ;
#50442=ORIENTED_EDGE ( 'NONE', *, *, #6322, .T. ) ;
#50443=CARTESIAN_POINT ( 'NONE',  ( 37.00000000000000711, 10.91536515067648239, 4.339012074899986970 ) ) ;
#50444=CIRCLE ( 'NONE', #9037, 12.18650000000000233 ) ;
#50445=ADVANCED_FACE ( 'NONE', ( #3874 ), #4181, .T. ) ;
#50447=ORIENTED_EDGE ( 'NONE', *, *, #53812, .F. ) ;
#50448=DIRECTION ( 'NONE',  ( -1.000000000000000000, 0.000000000000000000, -0.000000000000000000 ) ) ;
#50450=LINE ( 'NONE', #25481, #59825 ) ;
#50451=CARTESIAN_POINT ( 'NONE',  ( 9.169146324975033124, 6.964048800780563653, -11.57111712795824587 ) ) ;
#50452=CARTESIAN_POINT ( 'NONE',  ( -37.00000000000000711, -1.262958560998674429, -12.12087942037211086 ) ) ;
#50454=DIRECTION ( 'NONE',  ( -1.000000000000000000, 0.000000000000000000, 0.000000000000000000 ) ) ;
#50456=EDGE_CURVE ( 'NONE', #63705, #38749, #60044, .T. ) ;
#50459=CARTESIAN_POINT ( 'NONE',  ( -35.00000000000000000, -11.74614673114904129, -0.01609748574457297438 ) ) ;
#50460=VERTEX_POINT ( 'NONE', #29754 ) ;
#50463=EDGE_CURVE ( 'NONE', #15694, #61226, #65155, .T. ) ;
#50465=VERTEX_POINT ( 'NONE', #10149 ) ;
#50466=FACE_OUTER_BOUND ( 'NONE', #41683, .T. ) ;
#50467=CIRCLE ( 'NONE', #3778, 4.999999999999999112 ) ;
#50468=DIRECTION ( 'NONE',  ( -1.000000000000000000, 0.000000000000000000, 0.000000000000000000 ) ) ;
#50469=CARTESIAN_POINT ( 'NONE',  ( 24.19770493339638406, 1.945095382686029550, 13.36407410745160540 ) ) ;
#50470=ADVANCED_FACE ( 'NONE', ( #52032 ), #5511, .T. ) ;
#50471=ORIENTED_EDGE ( 'NONE', *, *, #46318, .T. ) ;
#50472=VERTEX_POINT ( 'NONE', #56351 ) ;
#50474=VERTEX_POINT ( 'NONE', #831 ) ;
#50476=DIRECTION ( 'NONE',  ( -1.000000000000000000, 0.000000000000000000, 0.000000000000000000 ) ) ;
#50478=CIRCLE ( 'NONE', #38788, 5.000000000000000000 ) ;
#50481=CARTESIAN_POINT ( 'NONE',  ( -35.00000000000000000, 0.000000000000000000, 0.000000000000000000 ) ) ;
#50482=ADVANCED_FACE ( 'NONE', ( #10799 ), #31089, .T. ) ;
#50484=ORIENTED_EDGE ( 'NONE', *, *, #57734, .F. ) ;
#50486=EDGE_CURVE ( 'NONE', #2113, #38173, #5173, .T. ) ;
#50488=CARTESIAN_POINT ( 'NONE',  ( -37.00000000000000711, -2.936739658819952581, 11.37311665002362560 ) ) ;
#50489=LINE ( 'NONE', #19884, #25388 ) ;
#50490=DIRECTION ( 'NONE',  ( 0.3628680629012471792, -0.9318405276259971171, 0.000000000000000000 ) ) ;
#50491=CARTESIAN_POINT ( 'NONE',  ( 35.00000000000000000, 4.705694406421931860E-17, -3.469127814946512892E-15 ) ) ;
#50492=FACE_OUTER_BOUND ( 'NONE', #28316, .T. ) ;
#50493=CARTESIAN_POINT ( 'NONE',  ( -37.00000000000000711, 2.021542716731397071, 12.01765980939842748 ) ) ;
#50494=CIRCLE ( 'NONE', #34563, 12.18649999999999878 ) ;
#50495=ORIENTED_EDGE ( 'NONE', *, *, #49730, .T. ) ;
#50496=DIRECTION ( 'NONE',  ( 1.000000000000000000, 0.000000000000000000, -0.000000000000000000 ) ) ;
#50498=ORIENTED_EDGE ( 'NONE', *, *, #23444, .F. ) ;
#50499=CYLINDRICAL_SURFACE ( 'NONE', #22201, 12.74999999999999822 ) ;
#50500=DIRECTION ( 'NONE',  ( 0.000000000000000000, 0.01356324068817992175, -0.9999080150203990547 ) ) ;
#50501=CARTESIAN_POINT ( 'NONE',  ( -17.88545287150297014, 6.217808922599323829, -11.98485482592045237 ) ) ;
#50503=CARTESIAN_POINT ( 'NONE',  ( -37.00000000000000711, -9.321877890560388735, -7.146664589318012517 ) ) ;
#50507=CARTESIAN_POINT ( 'NONE',  ( -37.00000000000000711, -5.273331777780412288, 10.49591321039678959 ) ) ;
#50508=CARTESIAN_POINT ( 'NONE',  ( 36.00000000000000711, 12.02534193257720574, -4.237174932027271801 ) ) ;
#50509=EDGE_CURVE ( 'NONE', #13166, #38215, #37371, .T. ) ;
#50510=CARTESIAN_POINT ( 'NONE',  ( -17.56786360922926349, -5.609040142167114773, 10.61363638985786473 ) ) ;
#50515=ORIENTED_EDGE ( 'NONE', *, *, #64602, .T. ) ;
#50516=CARTESIAN_POINT ( 'NONE',  ( 35.00000000000000000, 4.705694406421931860E-17, -3.469127814946512892E-15 ) ) ;
#50517=LINE ( 'NONE', #302, #54375 ) ;
#50518=ADVANCED_FACE ( 'NONE', ( #15774 ), #36730, .T. ) ;
#50521=AXIS2_PLACEMENT_3D ( 'NONE', #23299, #33273, #38592 ) ;
#50523=ORIENTED_EDGE ( 'NONE', *, *, #40239, .F. ) ;
#50524=VERTEX_POINT ( 'NONE', #31722 ) ;
#50526=ORIENTED_EDGE ( 'NONE', *, *, #2765, .F. ) ;
#50530=CARTESIAN_POINT ( 'NONE',  ( -27.31123137524929234, 10.57279367158373162, -8.394978051634899074 ) ) ;
#50531=FACE_OUTER_BOUND ( 'NONE', #54956, .T. ) ;
#50532=CARTESIAN_POINT ( 'NONE',  ( -11.35685066047967062, -8.377133794443500037, 10.59944628267702527 ) ) ;
#50537=CARTESIAN_POINT ( 'NONE',  ( -9.144366736240645110, -11.10870866445312544, -4.554380859875097443 ) ) ;
#50538=ORIENTED_EDGE ( 'NONE', *, *, #26123, .F. ) ;
#50540=DIRECTION ( 'NONE',  ( -1.000000000000000000, 0.000000000000000000, 0.000000000000000000 ) ) ;
#50542=DIRECTION ( 'NONE',  ( -1.000000000000000000, 0.000000000000000000, 0.000000000000000000 ) ) ;
#50544=CARTESIAN_POINT ( 'NONE',  ( 37.00000000000000711, 5.391785509271111110, 10.43555801961468887 ) ) ;
#50545=DIRECTION ( 'NONE',  ( -1.000000000000000000, 0.000000000000000000, 0.000000000000000000 ) ) ;
#50549=EDGE_LOOP ( 'NONE', ( #13443, #3094, #34715, #7770 ) ) ;
#50550=ORIENTED_EDGE ( 'NONE', *, *, #62667, .F. ) ;
#50552=EDGE_CURVE ( 'NONE', #65779, #61418, #21437, .T. ) ;
#50554=DIRECTION ( 'NONE',  ( 0.000000000000000000, -0.01356324068817998940, 0.9999080150203990547 ) ) ;
#50557=ORIENTED_EDGE ( 'NONE', *, *, #23742, .F. ) ;
#50558=EDGE_CURVE ( 'NONE', #40917, #30330, #62814, .T. ) ;
#50562=DIRECTION ( 'NONE',  ( 0.000000000000000000, -0.01356324068817998940, 0.9999080150203990547 ) ) ;
#50563=DIRECTION ( 'NONE',  ( -1.000000000000000000, 0.000000000000000000, 0.000000000000000000 ) ) ;
#50564=ORIENTED_EDGE ( 'NONE', *, *, #33348, .F. ) ;
#50565=CIRCLE ( 'NONE', #3862, 4.999999999999999112 ) ;
#50566=EDGE_CURVE ( 'NONE', #38541, #25992, #5849, .T. ) ;
#50569=AXIS2_PLACEMENT_3D ( 'NONE', #19758, #21036, #5116 ) ;
#50571=CARTESIAN_POINT ( 'NONE',  ( -17.19065538327509657, 2.658487034042159802, 13.23633903133955414 ) ) ;
#50573=EDGE_CURVE ( 'NONE', #19083, #11411, #7627, .T. ) ;
#50575=CARTESIAN_POINT ( 'NONE',  ( 35.00000000000000000, 8.366449238204499039, 9.621072037176897851 ) ) ;
#50576=CARTESIAN_POINT ( 'NONE',  ( 28.91776584869966626, 9.508282570375039100, 7.334618107890905847 ) ) ;
#50578=CIRCLE ( 'NONE', #6993, 4.999999999999999112 ) ;
#50581=EDGE_LOOP ( 'NONE', ( #3100, #45369, #11094, #55632, #19656, #2946 ) ) ;
#50582=DIRECTION ( 'NONE',  ( -1.000000000000000000, 0.000000000000000000, 0.000000000000000000 ) ) ;
#50583=CARTESIAN_POINT ( 'NONE',  ( -37.00000000000000711, 9.677500615117999416, -6.657191900728212985 ) ) ;
#50584=DIRECTION ( 'NONE',  ( 0.000000000000000000, -0.01356324068817998940, 0.9999080150203990547 ) ) ;
#50585=DIRECTION ( 'NONE',  ( -1.000000000000000000, 0.000000000000000000, 0.000000000000000000 ) ) ;
#50588=CARTESIAN_POINT ( 'NONE',  ( 35.00000000000000000, 4.705694406421931860E-17, -3.469127814946512892E-15 ) ) ;
#50590=DIRECTION ( 'NONE',  ( 0.000000000000000000, 0.3554799084908970563, 0.9346839223284539866 ) ) ;
#50592=ADVANCED_FACE ( 'NONE', ( #42343 ), #42674, .T. ) ;
#50594=LINE ( 'NONE', #54908, #2010 ) ;
#50595=CARTESIAN_POINT ( 'NONE',  ( -36.00000000000000711, -6.265926637539413591, -11.10408318471066380 ) ) ;
#50596=CARTESIAN_POINT ( 'NONE',  ( 35.00000000000000000, 4.705694406421931860E-17, -3.469127814946512892E-15 ) ) ;
#50598=EDGE_CURVE ( 'NONE', #52926, #38497, #27397, .T. ) ;
#50600=VERTEX_POINT ( 'NONE', #43675 ) ;
#50601=AXIS2_PLACEMENT_3D ( 'NONE', #28019, #33963, #54615 ) ;
#50602=VERTEX_POINT ( 'NONE', #17443 ) ;
#50603=DIRECTION ( 'NONE',  ( 0.000000000000000000, 0.01356324068818000848, -0.9999080150203990547 ) ) ;
#50604=CARTESIAN_POINT ( 'NONE',  ( 35.00000000000000000, 11.16627499335655216, 3.645068577060061266 ) ) ;
#50608=EDGE_CURVE ( 'NONE', #23216, #29886, #53287, .T. ) ;
#50609=ORIENTED_EDGE ( 'NONE', *, *, #17032, .F. ) ;
#50610=VERTEX_POINT ( 'NONE', #62979 ) ;
#50611=B_SPLINE_CURVE_WITH_KNOTS ( 'NONE', 3,
 ( #24764, #19783, #40039, #45361, #15099, #40706, #35376, #25409, #25749, #14753, #45689, #492, #35030, #55345, #31057, #9783, #5820, #55684, #10121, #21065, #30399, #60998 ),
 .UNSPECIFIED., .F., .F.,
 ( 4, 2, 2, 2, 2, 2, 2, 2, 2, 2, 4 ),
 ( 0.000000000000000000, 0.001195189350898897109, 0.002390378701797794218, 0.003585568052696691543, 0.004780757403595588435, 0.005378352079045037315, 0.005975946754494486195, 0.006573541429943933340, 0.007171136105393381352, 0.008366325456292272172, 0.009561514807191164728 ),
 .UNSPECIFIED. ) ;
#50612=CARTESIAN_POINT ( 'NONE',  ( 29.45729197154192747, -9.438926003476494131, 7.413919495756846167 ) ) ;
#50613=CYLINDRICAL_SURFACE ( 'NONE', #55479, 12.75000000000000178 ) ;
#50614=ORIENTED_EDGE ( 'NONE', *, *, #6621, .F. ) ;
#50615=CARTESIAN_POINT ( 'NONE',  ( -37.00000000000000711, 12.46157735505193109, -2.696588552978925524 ) ) ;
#50616=DIRECTION ( 'NONE',  ( -1.000000000000000000, -0.000000000000000000, 0.000000000000000000 ) ) ;
#50618=ORIENTED_EDGE ( 'NONE', *, *, #41903, .F. ) ;
#50621=CARTESIAN_POINT ( 'NONE',  ( 37.00000000000000711, 4.705694406421931860E-17, -3.469127814946512892E-15 ) ) ;
#50625=ORIENTED_EDGE ( 'NONE', *, *, #39669, .T. ) ;
#50626=DIRECTION ( 'NONE',  ( 0.000000000000000000, 0.01356324068817998940, -0.9999080150203990547 ) ) ;
#50627=ORIENTED_EDGE ( 'NONE', *, *, #55231, .F. ) ;
#50628=CARTESIAN_POINT ( 'NONE',  ( 35.00000000000000000, -10.99909370905160699, -5.246972444133983338 ) ) ;
#50629=ADVANCED_FACE ( 'NONE', ( #37044 ), #7793, .T. ) ;
#50630=CYLINDRICAL_SURFACE ( 'NONE', #3313, 12.18650000000000055 ) ;
#50635=DIRECTION ( 'NONE',  ( 1.000000000000000000, 0.000000000000000000, -0.000000000000000000 ) ) ;
#50636=CARTESIAN_POINT ( 'NONE',  ( 11.38817443037663679, 0.2421923074375172957, 11.99781792006712955 ) ) ;
#50639=CARTESIAN_POINT ( 'NONE',  ( 5.736444914132059480, -9.902886448537387309, 9.181108836895850445 ) ) ;
#50640=ORIENTED_EDGE ( 'NONE', *, *, #62040, .T. ) ;
#50642=DIRECTION ( 'NONE',  ( 0.000000000000000000, -0.07632122047557186872, 0.9970832820307033995 ) ) ;
#50646=B_SPLINE_CURVE_WITH_KNOTS ( 'NONE', 3,
 ( #11195, #17500, #16178, #16827, #51770, #26812, #41427, #61720, #6212, #1225 ),
 .UNSPECIFIED., .F., .F.,
 ( 4, 2, 2, 2, 4 ),
 ( 4.336808689942017736E-19, 0.0006730921559986501133, 0.001346184311997299793, 0.002019276467995947087, 0.002692368623994594382 ),
 .UNSPECIFIED. ) ;
#50647=EDGE_CURVE ( 'NONE', #33925, #16732, #26750, .T. ) ;
#50648=ORIENTED_EDGE ( 'NONE', *, *, #61380, .F. ) ;
#50651=CARTESIAN_POINT ( 'NONE',  ( 37.00000000000000711, 4.705694406421931860E-17, -3.469127814946512892E-15 ) ) ;
#50652=CIRCLE ( 'NONE', #21962, 5.000000000000000000 ) ;
#50654=FACE_OUTER_BOUND ( 'NONE', #25221, .T. ) ;
#50657=ORIENTED_EDGE ( 'NONE', *, *, #12887, .F. ) ;
#50659=DIRECTION ( 'NONE',  ( 0.8867529933577789070, 0.000000000000000000, -0.4622435816439414147 ) ) ;
#50661=ORIENTED_EDGE ( 'NONE', *, *, #46263, .F. ) ;
#50664=EDGE_CURVE ( 'NONE', #21253, #37151, #1822, .T. ) ;
#50668=ORIENTED_EDGE ( 'NONE', *, *, #12029, .F. ) ;
#50669=DIRECTION ( 'NONE',  ( -1.000000000000000000, 0.000000000000000000, 0.000000000000000000 ) ) ;
#50671=DIRECTION ( 'NONE',  ( -1.000000000000000000, 0.000000000000000000, 0.000000000000000000 ) ) ;
#50672=EDGE_CURVE ( 'NONE', #52930, #40729, #6589, .T. ) ;
#50673=DIRECTION ( 'NONE',  ( -1.000000000000000000, 0.000000000000000000, 0.000000000000000000 ) ) ;
#50675=ORIENTED_EDGE ( 'NONE', *, *, #55953, .F. ) ;
#50676=AXIS2_PLACEMENT_3D ( 'NONE', #54667, #35325, #10074 ) ;
#50677=CARTESIAN_POINT ( 'NONE',  ( -35.00000000000000000, 12.18359334611896472, 0.2661492558803780772 ) ) ;
#50678=CARTESIAN_POINT ( 'NONE',  ( 3.441679217059768980, 6.045329562784094612, -10.36821124058885424 ) ) ;
#50679=ORIENTED_EDGE ( 'NONE', *, *, #16143, .T. ) ;
#50680=CARTESIAN_POINT ( 'NONE',  ( 11.92331831525852159, 0.08325394350958797984, 13.49997450358961792 ) ) ;
#50682=ORIENTED_EDGE ( 'NONE', *, *, #12080, .T. ) ;
#50683=EDGE_CURVE ( 'NONE', #22894, #4994, #48373, .T. ) ;
#50684=EDGE_CURVE ( 'NONE', #48941, #53899, #52252, .T. ) ;
#50685=ORIENTED_EDGE ( 'NONE', *, *, #42349, .T. ) ;
#50687=ORIENTED_EDGE ( 'NONE', *, *, #31911, .F. ) ;
#50688=EDGE_CURVE ( 'NONE', #37930, #10044, #60730, .T. ) ;
#50691=CARTESIAN_POINT ( 'NONE',  ( 37.00000000000000711, 12.16893194857555116, 3.805206332242343059 ) ) ;
#50692=FACE_OUTER_BOUND ( 'NONE', #37690, .T. ) ;
#50697=CARTESIAN_POINT ( 'NONE',  ( 35.00000000000000000, 4.705694406421931860E-17, -3.469127814946512892E-15 ) ) ;
#50699=VERTEX_POINT ( 'NONE', #22765 ) ;
#50700=CARTESIAN_POINT ( 'NONE',  ( 35.00000000000000000, 4.705694406421931860E-17, -3.469127814946512892E-15 ) ) ;
#50703=ORIENTED_EDGE ( 'NONE', *, *, #50664, .F. ) ;
#50704=ORIENTED_EDGE ( 'NONE', *, *, #6976, .T. ) ;
#50708=CARTESIAN_POINT ( 'NONE',  ( 47.00000000000000711, 4.705694406421931860E-17, -3.469127814946512892E-15 ) ) ;
#50714=VERTEX_POINT ( 'NONE', #23750 ) ;
#50717=VERTEX_POINT ( 'NONE', #30022 ) ;
#50718=DIRECTION ( 'NONE',  ( -1.000000000000000000, -1.836970198721029688E-16, 0.000000000000000000 ) ) ;
#50719=CYLINDRICAL_SURFACE ( 'NONE', #41615, 12.18649999999999878 ) ;
#50720=DIRECTION ( 'NONE',  ( -1.000000000000000000, 0.000000000000000000, 0.000000000000000000 ) ) ;
#50723=CIRCLE ( 'NONE', #40064, 12.75000000000000178 ) ;
#50724=CARTESIAN_POINT ( 'NONE',  ( 35.00000000000000000, 8.551552972817191289, 8.052525312709789773 ) ) ;
#50725=CARTESIAN_POINT ( 'NONE',  ( -35.00000000000000000, 12.01765980939845058, -2.021542716731266065 ) ) ;
#50726=VECTOR ( 'NONE', #13266, 1000.000000000000000 ) ;
#50727=ORIENTED_EDGE ( 'NONE', *, *, #2098, .F. ) ;
#50731=AXIS2_PLACEMENT_3D ( 'NONE', #42759, #6228, #26490 ) ;
#50733=CARTESIAN_POINT ( 'NONE',  ( 6.433569295279546907, -8.070817871543312094, 8.888545806055137888 ) ) ;
#50734=DIRECTION ( 'NONE',  ( 1.000000000000000000, 0.000000000000000000, 0.000000000000000000 ) ) ;
#50735=CIRCLE ( 'NONE', #1893, 4.999999999999999112 ) ;
#50736=EDGE_CURVE ( 'NONE', #50472, #11758, #62856, .T. ) ;
#50739=DIRECTION ( 'NONE',  ( -1.000000000000000000, 0.000000000000000000, 0.000000000000000000 ) ) ;
#50740=ORIENTED_EDGE ( 'NONE', *, *, #47652, .T. ) ;
#50742=CARTESIAN_POINT ( 'NONE',  ( 17.48655162378398131, 11.52771039025705591, 7.062232779588992315 ) ) ;
#50744=EDGE_CURVE ( 'NONE', #59777, #39315, #19411, .T. ) ;
#50747=EDGE_LOOP ( 'NONE', ( #42558, #41919, #63375, #37884 ) ) ;
#50749=CARTESIAN_POINT ( 'NONE',  ( 26.34661844826604593, 13.08594712317291986, 3.317828791472332117 ) ) ;
#50755=CARTESIAN_POINT ( 'NONE',  ( -37.00000000000000711, 11.60979404548639948, -3.704519465651187282 ) ) ;
#50756=VERTEX_POINT ( 'NONE', #24720 ) ;
#50758=AXIS2_PLACEMENT_3D ( 'NONE', #15922, #36557, #46860 ) ;
#50759=CARTESIAN_POINT ( 'NONE',  ( 37.00000000000000711, 3.805206332242470957, -12.16893194857551563 ) ) ;
#50760=ORIENTED_EDGE ( 'NONE', *, *, #35602, .T. ) ;
#50761=DIRECTION ( 'NONE',  ( -1.000000000000000000, 0.000000000000000000, 0.000000000000000000 ) ) ;
#50763=CIRCLE ( 'NONE', #8286, 12.18649999999999878 ) ;
#50764=CARTESIAN_POINT ( 'NONE',  ( -18.58686583997247155, 5.151216734910867068, -12.47858029384659417 ) ) ;
#50765=DIRECTION ( 'NONE',  ( 0.000000000000000000, 0.01356324068817998940, -0.9999080150203990547 ) ) ;
#50766=DIRECTION ( 'NONE',  ( -1.000000000000000000, 0.000000000000000000, -0.000000000000000000 ) ) ;
#50767=DIRECTION ( 'NONE',  ( 0.000000000000000000, 0.01356324068817998940, -0.9999080150203990547 ) ) ;
#50768=CARTESIAN_POINT ( 'NONE',  ( 37.00000000000000711, 4.705694406421931860E-17, -3.469127814946512892E-15 ) ) ;
#50769=AXIS2_PLACEMENT_3D ( 'NONE', #13091, #33372, #53672 ) ;
#50772=VERTEX_POINT ( 'NONE', #49986 ) ;
#50778=ORIENTED_EDGE ( 'NONE', *, *, #19410, .T. ) ;
#50779=DIRECTION ( 'NONE',  ( 0.000000000000000000, -0.9467777615094536969, -0.3218879778916073908 ) ) ;
#50780=CARTESIAN_POINT ( 'NONE',  ( 12.83590194764781778, 10.34016517225328080, -6.102282133837778844 ) ) ;
#50781=FACE_BOUND ( 'NONE', #10719, .T. ) ;
#50782=ORIENTED_EDGE ( 'NONE', *, *, #58004, .T. ) ;
#50783=EDGE_LOOP ( 'NONE', ( #39208, #26086, #5176, #4634 ) ) ;
#50784=DIRECTION ( 'NONE',  ( 0.000000000000000000, -0.8515178078024813191, 0.5243256840888652626 ) ) ;
#50785=ORIENTED_EDGE ( 'NONE', *, *, #59116, .F. ) ;
#50788=CARTESIAN_POINT ( 'NONE',  ( -37.00000000000000711, -10.12742074351902311, 7.745827850122975811 ) ) ;
#50789=CARTESIAN_POINT ( 'NONE',  ( -35.00000000000000000, -11.38112321385052716, 2.905556151562584954 ) ) ;
#50790=ADVANCED_FACE ( 'NONE', ( #28712 ), #50338, .T. ) ;
#50792=CARTESIAN_POINT ( 'NONE',  ( 6.361445718264521432, -4.355102044641763648, -12.77822703589027320 ) ) ;
#50793=LINE ( 'NONE', #39828, #43971 ) ;
#50798=CARTESIAN_POINT ( 'NONE',  ( 35.00000000000000000, 11.54110654723649176, -2.185196060783925809 ) ) ;
#50799=CARTESIAN_POINT ( 'NONE',  ( 12.84739494846498786, 12.07655647595275994, -6.046275926700755754 ) ) ;
#50800=FACE_OUTER_BOUND ( 'NONE', #5889, .T. ) ;
#50802=DIRECTION ( 'NONE',  ( 1.000000000000000000, -0.000000000000000000, 0.000000000000000000 ) ) ;
#50803=DIRECTION ( 'NONE',  ( 0.000000000000000000, 0.5767582926624970074, 0.8169148498130275327 ) ) ;
#50804=CIRCLE ( 'NONE', #39111, 5.000000000000001776 ) ;
#50805=ADVANCED_FACE ( 'NONE', ( #33702 ), #59004, .T. ) ;
#50806=ORIENTED_EDGE ( 'NONE', *, *, #21254, .F. ) ;
#50807=CARTESIAN_POINT ( 'NONE',  ( 35.00000000000000000, -11.47561260193572963, 5.556331110570524423 ) ) ;
#50808=CIRCLE ( 'NONE', #33794, 12.18650000000000055 ) ;
#50809=VECTOR ( 'NONE', #4502, 1000.000000000000000 ) ;
#50810=EDGE_CURVE ( 'NONE', #43258, #30430, #3482, .T. ) ;
#50813=CARTESIAN_POINT ( 'NONE',  ( 37.00000000000000711, -1.738225594540086405, -12.63095688309028652 ) ) ;
#50814=DIRECTION ( 'NONE',  ( -1.000000000000000000, 0.000000000000000000, 0.000000000000000000 ) ) ;
#50818=ADVANCED_FACE ( 'NONE', ( #9090 ), #29372, .T. ) ;
#50820=EDGE_LOOP ( 'NONE', ( #51349, #43765, #14565, #42943 ) ) ;
#50821=CARTESIAN_POINT ( 'NONE',  ( 47.00000000000000711, 4.705694406421931860E-17, -3.469127814946512892E-15 ) ) ;
#50822=CARTESIAN_POINT ( 'NONE',  ( -30.01168020819624616, -3.375037589979597463, -11.52238638448564600 ) ) ;
#50824=CIRCLE ( 'NONE', #3043, 5.000000000000000888 ) ;
#50825=DIRECTION ( 'NONE',  ( 1.000000000000000000, -0.000000000000000000, 0.000000000000000000 ) ) ;
#50828=CARTESIAN_POINT ( 'NONE',  ( -18.01507738101584621, -4.918977875164763702, 10.94647906529714732 ) ) ;
#50830=ORIENTED_EDGE ( 'NONE', *, *, #34589, .F. ) ;
#50831=EDGE_CURVE ( 'NONE', #5805, #17595, #54243, .T. ) ;
#50832=CARTESIAN_POINT ( 'NONE',  ( -37.00000000000000711, -4.732539170486343316, 11.23004253107762906 ) ) ;
#50833=ORIENTED_EDGE ( 'NONE', *, *, #60208, .T. ) ;
#50838=AXIS2_PLACEMENT_3D ( 'NONE', #47546, #1682, #42197 ) ;
#50839=VERTEX_POINT ( 'NONE', #61581 ) ;
#50840=ORIENTED_EDGE ( 'NONE', *, *, #34750, .T. ) ;
#50842=EDGE_CURVE ( 'NONE', #44156, #34336, #10466, .T. ) ;
#50843=VERTEX_POINT ( 'NONE', #36318 ) ;
#50844=DIRECTION ( 'NONE',  ( -1.000000000000000000, 0.000000000000000000, -0.000000000000000000 ) ) ;
#50845=CARTESIAN_POINT ( 'NONE',  ( -18.49080574448724690, 11.99999999999999645, 2.510045011421233839E-15 ) ) ;
#50848=AXIS2_PLACEMENT_3D ( 'NONE', #32050, #47045, #17094 ) ;
#50851=DIRECTION ( 'NONE',  ( -0.02770351589312032917, 0.9996161839461982224, 0.000000000000000000 ) ) ;
#50854=ORIENTED_EDGE ( 'NONE', *, *, #6400, .T. ) ;
#50855=CARTESIAN_POINT ( 'NONE',  ( 35.00000000000000000, -4.426194442447322075, -11.35427606708804937 ) ) ;
#50859=FACE_OUTER_BOUND ( 'NONE', #40409, .T. ) ;
#50860=ORIENTED_EDGE ( 'NONE', *, *, #20659, .F. ) ;
#50861=CIRCLE ( 'NONE', #1873, 4.999999999999999112 ) ;
#50862=PLANE ( 'NONE',  #31211 ) ;
#50863=CARTESIAN_POINT ( 'NONE',  ( 6.788880239637845371, -6.730272244910862511, -11.70889290456736909 ) ) ;
#50867=VERTEX_POINT ( 'NONE', #443 ) ;
#50868=VECTOR ( 'NONE', #15532, 1000.000000000000000 ) ;
#50870=ORIENTED_EDGE ( 'NONE', *, *, #55425, .F. ) ;
#50871=CARTESIAN_POINT ( 'NONE',  ( -35.00000000000000000, -3.645068577060105230, 11.16627499335654150 ) ) ;
#50872=ORIENTED_EDGE ( 'NONE', *, *, #63432, .F. ) ;
#50873=VERTEX_POINT ( 'NONE', #15049 ) ;
#50878=ADVANCED_FACE ( 'NONE', ( #21354 ), #40657, .T. ) ;
#50880=DIRECTION ( 'NONE',  ( 0.000000000000000000, -1.000000000000000000, 0.000000000000000000 ) ) ;
#50882=ORIENTED_EDGE ( 'NONE', *, *, #18439, .T. ) ;
#50883=CARTESIAN_POINT ( 'NONE',  ( -21.17861794710831091, 25.00000000000000000, -3.604945070120774808 ) ) ;
#50885=ORIENTED_EDGE ( 'NONE', *, *, #3872, .F. ) ;
#50888=CARTESIAN_POINT ( 'NONE',  ( 36.00000000000000711, 5.865551165831078606, -11.32068061209297483 ) ) ;
#50889=CARTESIAN_POINT ( 'NONE',  ( 35.00000000000000000, 4.705694406421931860E-17, -3.469127814946512892E-15 ) ) ;
#50890=FACE_OUTER_BOUND ( 'NONE', #58105, .T. ) ;
#50891=CIRCLE ( 'NONE', #37050, 12.18649999999999878 ) ;
#50892=EDGE_CURVE ( 'NONE', #40209, #26482, #10386, .T. ) ;
#50894=CARTESIAN_POINT ( 'NONE',  ( 35.00000000000000000, -3.340853584269612764, -11.26103545359855040 ) ) ;
#50895=AXIS2_PLACEMENT_3D ( 'NONE', #8594, #53841, #17929 ) ;
#50896=EDGE_LOOP ( 'NONE', ( #64416, #52182, #44229, #65427 ) ) ;
#50898=DIRECTION ( 'NONE',  ( 0.000000000000000000, 0.2960891610144441022, 0.9551603052523500725 ) ) ;
#50903=CARTESIAN_POINT ( 'NONE',  ( 35.00000000000000000, 2.544412758415841580, -11.91791701451267471 ) ) ;
#50905=CARTESIAN_POINT ( 'NONE',  ( -35.00000000000000000, -8.052525312709946093, 8.551552972817052733 ) ) ;
#50907=DIRECTION ( 'NONE',  ( 0.000000000000000000, -0.07632122047557189648, 0.9970832820307033995 ) ) ;
#50908=LINE ( 'NONE', #30937, #26356 ) ;
#50909=AXIS2_PLACEMENT_3D ( 'NONE', #33158, #58797, #13215 ) ;
#50910=AXIS2_PLACEMENT_3D ( 'NONE', #48803, #37499, #3254 ) ;
#50914=EDGE_CURVE ( 'NONE', #9977, #22363, #31006, .T. ) ;
#50918=DIRECTION ( 'NONE',  ( -1.000000000000000000, 0.000000000000000000, 0.000000000000000000 ) ) ;
#50920=AXIS2_PLACEMENT_3D ( 'NONE', #8023, #48581, #42919 ) ;
#50922=VERTEX_POINT ( 'NONE', #41298 ) ;
#50923=EDGE_CURVE ( 'NONE', #35283, #10110, #11261, .T. ) ;
#50928=ADVANCED_FACE ( 'NONE', ( #50654 ), #13895, .T. ) ;
#50930=VERTEX_POINT ( 'NONE', #38192 ) ;
#50931=ORIENTED_EDGE ( 'NONE', *, *, #48735, .F. ) ;
#50932=ORIENTED_EDGE ( 'NONE', *, *, #64705, .T. ) ;
#50936=ORIENTED_EDGE ( 'NONE', *, *, #3021, .T. ) ;
#50937=DIRECTION ( 'NONE',  ( 0.000000000000000000, -0.01356324068817992175, 0.9999080150203990547 ) ) ;
#50944=DIRECTION ( 'NONE',  ( 1.000000000000000000, 0.000000000000000000, 0.000000000000000000 ) ) ;
#50945=VERTEX_POINT ( 'NONE', #8277 ) ;
#50946=CARTESIAN_POINT ( 'NONE',  ( -19.47984447937493613, -1.416020129149132334, 25.00000000000000000 ) ) ;
#50947=EDGE_LOOP ( 'NONE', ( #36139, #45377, #21365, #24283 ) ) ;
#50948=CARTESIAN_POINT ( 'NONE',  ( -37.00000000000000711, 1.286231064351496922, -12.68495603654570481 ) ) ;
#50949=ORIENTED_EDGE ( 'NONE', *, *, #57931, .T. ) ;
#50950=CARTESIAN_POINT ( 'NONE',  ( 12.10998784662220729, -8.443435280036764468, -8.526922110106905706 ) ) ;
#50951=AXIS2_PLACEMENT_3D ( 'NONE', #57228, #11655, #21970 ) ;
#50954=DIRECTION ( 'NONE',  ( 1.000000000000000000, 0.000000000000000000, 0.000000000000000000 ) ) ;
#50956=CARTESIAN_POINT ( 'NONE',  ( 36.00000000000000711, 12.74921544981111055, -0.1414404973752615424 ) ) ;
#50959=CARTESIAN_POINT ( 'NONE',  ( -35.00000000000000000, -8.017674001891851532, 9.913596905230086520 ) ) ;
#50960=LINE ( 'NONE', #61251, #26775 ) ;
#50961=ORIENTED_EDGE ( 'NONE', *, *, #65228, .T. ) ;
#50963=CYLINDRICAL_SURFACE ( 'NONE', #22622, 5.000000000000000888 ) ;
#50964=ORIENTED_EDGE ( 'NONE', *, *, #37336, .T. ) ;
#50965=CARTESIAN_POINT ( 'NONE',  ( 11.83609954913792883, -13.39357575799777145, -1.699053554970645363 ) ) ;
#50966=ORIENTED_EDGE ( 'NONE', *, *, #22895, .F. ) ;
#50968=ORIENTED_EDGE ( 'NONE', *, *, #41754, .F. ) ;
#50972=VECTOR ( 'NONE', #5991, 1000.000000000000000 ) ;
#50973=DIRECTION ( 'NONE',  ( -1.000000000000000000, 0.000000000000000000, 0.000000000000000000 ) ) ;
#50976=ADVANCED_FACE ( 'NONE', ( #58169 ), #12590, .T. ) ;
#50977=ORIENTED_EDGE ( 'NONE', *, *, #53310, .T. ) ;
#50978=CARTESIAN_POINT ( 'NONE',  ( -17.15262702242703341, -7.064764427389573775, -9.706288918837138624 ) ) ;
#50979=VERTEX_POINT ( 'NONE', #7970 ) ;
#50985=CIRCLE ( 'NONE', #44587, 12.18649999999999878 ) ;
#50989=VERTEX_POINT ( 'NONE', #64442 ) ;
#50994=AXIS2_PLACEMENT_3D ( 'NONE', #44138, #9203, #19537 ) ;
#50996=EDGE_CURVE ( 'NONE', #7257, #62589, #38309, .T. ) ;
#50997=DIRECTION ( 'NONE',  ( 1.000000000000000000, -0.000000000000000000, 0.000000000000000000 ) ) ;
#50998=CYLINDRICAL_SURFACE ( 'NONE', #40413, 13.50000000000000178 ) ;
#50999=AXIS2_PLACEMENT_3D ( 'NONE', #64084, #29175, #23869 ) ;
#51000=ORIENTED_EDGE ( 'NONE', *, *, #44789, .T. ) ;
#51001=DIRECTION ( 'NONE',  ( 1.000000000000000000, 0.000000000000000000, 0.000000000000000000 ) ) ;
#51004=ORIENTED_EDGE ( 'NONE', *, *, #46490, .F. ) ;
#51005=EDGE_CURVE ( 'NONE', #13375, #62432, #29808, .T. ) ;
#51007=CARTESIAN_POINT ( 'NONE',  ( 35.00000000000000000, 4.705694406421931860E-17, -3.469127814946512892E-15 ) ) ;
#51008=ORIENTED_EDGE ( 'NONE', *, *, #52660, .F. ) ;
#51009=CIRCLE ( 'NONE', #24, 12.18649999999999878 ) ;
#51013=DIRECTION ( 'NONE',  ( 0.000000000000000000, 0.01356324068817998940, -0.9999080150203990547 ) ) ;
#51014=DIRECTION ( 'NONE',  ( 0.000000000000000000, 0.01356324068817991828, -0.9999080150203990547 ) ) ;
#51016=AXIS2_PLACEMENT_3D ( 'NONE', #20029, #53976, #29661 ) ;
#51017=CARTESIAN_POINT ( 'NONE',  ( 8.982479512971032420, 5.162787350578708967, 10.83868146673709276 ) ) ;
#51018=DIRECTION ( 'NONE',  ( 0.000000000000000000, 0.000000000000000000, -1.000000000000000000 ) ) ;
#51020=DIRECTION ( 'NONE',  ( 1.000000000000000000, 0.000000000000000000, 0.000000000000000000 ) ) ;
#51022=ORIENTED_EDGE ( 'NONE', *, *, #59830, .F. ) ;
#51023=CARTESIAN_POINT ( 'NONE',  ( -36.00000000000000711, 12.21925492305362226, 3.640372113593595138 ) ) ;
#51024=CIRCLE ( 'NONE', #2170, 12.74999999999999822 ) ;
#51025=ORIENTED_EDGE ( 'NONE', *, *, #2124, .F. ) ;
#51028=ORIENTED_EDGE ( 'NONE', *, *, #61367, .F. ) ;
#51031=CARTESIAN_POINT ( 'NONE',  ( -35.00000000000000000, 5.672855678558835102, -10.28547182238001767 ) ) ;
#51034=AXIS2_PLACEMENT_3D ( 'NONE', #59563, #64531, #44258 ) ;
#51035=AXIS2_PLACEMENT_3D ( 'NONE', #19323, #44250, #59234 ) ;
#51037=CIRCLE ( 'NONE', #22339, 12.75000000000000178 ) ;
#51040=VERTEX_POINT ( 'NONE', #18913 ) ;
#51041=EDGE_CURVE ( 'NONE', #16656, #16455, #29520, .T. ) ;
#51042=EDGE_LOOP ( 'NONE', ( #51242, #55160, #58830, #45354 ) ) ;
#51043=FACE_OUTER_BOUND ( 'NONE', #8026, .T. ) ;
#51044=ORIENTED_EDGE ( 'NONE', *, *, #9899, .F. ) ;
#51047=CARTESIAN_POINT ( 'NONE',  ( -17.29244623348158783, 2.525873743887551814, 25.00000000000000000 ) ) ;
#51048=DIRECTION ( 'NONE',  ( 1.000000000000000000, 0.000000000000000000, -0.000000000000000000 ) ) ;
#51049=DIRECTION ( 'NONE',  ( -1.000000000000000000, -1.836970198721029688E-16, -0.000000000000000000 ) ) ;
#51052=AXIS2_PLACEMENT_3D ( 'NONE', #12469, #33091, #12803 ) ;
#51053=DIRECTION ( 'NONE',  ( 0.000000000000000000, -0.01356324068817998940, 0.9999080150203990547 ) ) ;
#51054=AXIS2_PLACEMENT_3D ( 'NONE', #31181, #57113, #47143 ) ;
#51056=ORIENTED_EDGE ( 'NONE', *, *, #40656, .T. ) ;
#51057=ORIENTED_EDGE ( 'NONE', *, *, #65440, .T. ) ;
#51058=VECTOR ( 'NONE', #40828, 1000.000000000000000 ) ;
#51059=CARTESIAN_POINT ( 'NONE',  ( 35.00000000000000000, 4.705694406421931860E-17, -3.469127814946512892E-15 ) ) ;
#51060=EDGE_CURVE ( 'NONE', #57376, #17810, #19573, .T. ) ;
#51063=CARTESIAN_POINT ( 'NONE',  ( -2.665275975174092871, -8.247467911538802099, 10.69349901239360001 ) ) ;
#51064=EDGE_CURVE ( 'NONE', #23892, #40032, #30504, .T. ) ;
#51065=CARTESIAN_POINT ( 'NONE',  ( 6.774697637567625996, -5.779741746118725487, 10.51838463467937856 ) ) ;
#51066=CYLINDRICAL_SURFACE ( 'NONE', #49211, 5.000000000000000888 ) ;
#51067=CARTESIAN_POINT ( 'NONE',  ( -35.00000000000000000, 0.000000000000000000, 0.000000000000000000 ) ) ;
#51068=CARTESIAN_POINT ( 'NONE',  ( 3.158320548757213686, 2.992226752387131761, -11.62285000527830192 ) ) ;
#51070=AXIS2_PLACEMENT_3D ( 'NONE', #3848, #59046, #13455 ) ;
#51071=VERTEX_POINT ( 'NONE', #60779 ) ;
#51073=DIRECTION ( 'NONE',  ( 0.000000000000000000, 0.01356324068817998940, -0.9999080150203990547 ) ) ;
#51074=DIRECTION ( 'NONE',  ( 0.000000000000000000, -0.01356324068817998940, 0.9999080150203990547 ) ) ;
#51076=AXIS2_PLACEMENT_3D ( 'NONE', #59026, #8138, #44667 ) ;
#51078=CIRCLE ( 'NONE', #7535, 12.75000000000000178 ) ;
#51079=ADVANCED_FACE ( 'NONE', ( #24883 ), #29846, .T. ) ;
#51081=CARTESIAN_POINT ( 'NONE',  ( -37.00000000000000711, 1.903127969211188653, 11.59095880812009227 ) ) ;
#51083=ORIENTED_EDGE ( 'NONE', *, *, #46689, .F. ) ;
#51085=CARTESIAN_POINT ( 'NONE',  ( 28.03536240197431439, 12.64334364039261693, 4.746761413380614414 ) ) ;
#51087=ORIENTED_EDGE ( 'NONE', *, *, #16997, .T. ) ;
#51089=DIRECTION ( 'NONE',  ( 0.000000000000000000, -0.01356324068817992175, 0.9999080150203990547 ) ) ;
#51090=DIRECTION ( 'NONE',  ( 1.000000000000000000, 0.000000000000000000, -0.000000000000000000 ) ) ;
#51092=ORIENTED_EDGE ( 'NONE', *, *, #5579, .F. ) ;
#51094=AXIS2_PLACEMENT_3D ( 'NONE', #18887, #24189, #29818 ) ;
#51097=CIRCLE ( 'NONE', #53230, 12.18650000000000233 ) ;
#51098=FACE_OUTER_BOUND ( 'NONE', #31977, .T. ) ;
#51103=DIRECTION ( 'NONE',  ( 0.000000000000000000, 0.01356324068817998940, -0.9999080150203990547 ) ) ;
#51104=AXIS2_PLACEMENT_3D ( 'NONE', #48899, #32909, #53223 ) ;
#51105=CARTESIAN_POINT ( 'NONE',  ( -37.00000000000000711, 0.000000000000000000, 0.000000000000000000 ) ) ;
#51106=CARTESIAN_POINT ( 'NONE',  ( -35.00000000000000000, 4.339012074900111315, -10.91536515067643620 ) ) ;
#51108=DIRECTION ( 'NONE',  ( 0.000000000000000000, 0.8515178078024849828, -0.5243256840888593784 ) ) ;
#51109=CIRCLE ( 'NONE', #59594, 12.75000000000000178 ) ;
#51110=ORIENTED_EDGE ( 'NONE', *, *, #29081, .T. ) ;
#51112=CARTESIAN_POINT ( 'NONE',  ( 3.291290029914074378, 8.250315036047103590, -10.68561190601526079 ) ) ;
#51113=CARTESIAN_POINT ( 'NONE',  ( -37.00000000000000711, 4.561791185930588632, -11.90598845858528776 ) ) ;
#51115=ORIENTED_EDGE ( 'NONE', *, *, #57795, .F. ) ;
#51118=CARTESIAN_POINT ( 'NONE',  ( 37.00000000000000711, -11.72397916322011824, 0.7214809346829776926 ) ) ;
#51120=ORIENTED_EDGE ( 'NONE', *, *, #35659, .F. ) ;
#51121=CARTESIAN_POINT ( 'NONE',  ( 29.22851443451641984, -10.03996910372599238, 9.034550257766868597 ) ) ;
#51122=CIRCLE ( 'NONE', #37290, 12.18649999999999878 ) ;
#51123=ORIENTED_EDGE ( 'NONE', *, *, #55385, .T. ) ;
#51124=CARTESIAN_POINT ( 'NONE',  ( 22.02159064219758022, -11.31093606971245791, -4.012113827732382454 ) ) ;
#51125=CYLINDRICAL_SURFACE ( 'NONE', #15072, 12.75000000000000178 ) ;
#51126=DIRECTION ( 'NONE',  ( -1.000000000000000000, 0.000000000000000000, -0.000000000000000000 ) ) ;
#51128=AXIS2_PLACEMENT_3D ( 'NONE', #57637, #61954, #62265 ) ;
#51129=AXIS2_PLACEMENT_3D ( 'NONE', #3572, #29449, #13816 ) ;
#51130=CYLINDRICAL_SURFACE ( 'NONE', #10740, 5.000000000000000888 ) ;
#51132=CARTESIAN_POINT ( 'NONE',  ( 37.00000000000000711, 4.705694406421931860E-17, -3.469127814946512892E-15 ) ) ;
#51135=ORIENTED_EDGE ( 'NONE', *, *, #16035, .F. ) ;
#51137=CARTESIAN_POINT ( 'NONE',  ( 24.73935261814495590, 8.970571808567301630, -7.973448879465720118 ) ) ;
#51138=EDGE_CURVE ( 'NONE', #39393, #40131, #15214, .T. ) ;
#51141=DIRECTION ( 'NONE',  ( 0.000000000000000000, 0.01356324068817992175, -0.9999080150203990547 ) ) ;
#51143=DIRECTION ( 'NONE',  ( 0.000000000000000000, 0.4935949184179200810, -0.8696919319575219243 ) ) ;
#51145=CARTESIAN_POINT ( 'NONE',  ( -35.00000000000000000, 11.61976888909158490, 3.827969819614505997 ) ) ;
#51146=CIRCLE ( 'NONE', #61801, 12.75000000000000178 ) ;
#51147=EDGE_CURVE ( 'NONE', #19224, #37445, #51217, .T. ) ;
#51148=AXIS2_PLACEMENT_3D ( 'NONE', #30374, #50669, #35675 ) ;
#51149=EDGE_LOOP ( 'NONE', ( #31203, #56851, #37739, #30744 ) ) ;
#51150=CARTESIAN_POINT ( 'NONE',  ( 35.00000000000000000, 4.705694406421931860E-17, -3.469127814946512892E-15 ) ) ;
#51151=CIRCLE ( 'NONE', #23513, 12.75000000000000178 ) ;
#51155=AXIS2_PLACEMENT_3D ( 'NONE', #23802, #55013, #19117 ) ;
#51158=ORIENTED_EDGE ( 'NONE', *, *, #42596, .T. ) ;
#51159=DIRECTION ( 'NONE',  ( 1.000000000000000000, 0.000000000000000000, 0.000000000000000000 ) ) ;
#51160=CARTESIAN_POINT ( 'NONE',  ( 35.00000000000000000, 2.021542716731571154, 12.01765980939839196 ) ) ;
#51161=AXIS2_PLACEMENT_3D ( 'NONE', #26757, #47052, #12109 ) ;
#51163=DIRECTION ( 'NONE',  ( 1.000000000000000000, 0.000000000000000000, 0.000000000000000000 ) ) ;
#51164=EDGE_CURVE ( 'NONE', #36886, #24124, #65736, .T. ) ;
#51165=CARTESIAN_POINT ( 'NONE',  ( 10.47324744292499510, 7.645705331602621335, -11.12856369570244830 ) ) ;
#51166=VECTOR ( 'NONE', #1888, 1000.000000000000000 ) ;
#51167=CARTESIAN_POINT ( 'NONE',  ( -35.00000000000000000, -12.71517666308948513, 0.9416912585473978803 ) ) ;
#51168=ORIENTED_EDGE ( 'NONE', *, *, #45580, .T. ) ;
#51169=LINE ( 'NONE', #30851, #15846 ) ;
#51171=ORIENTED_EDGE ( 'NONE', *, *, #59038, .F. ) ;
#51172=AXIS2_PLACEMENT_3D ( 'NONE', #32648, #39876, #63571 ) ;
#51174=LINE ( 'NONE', #37155, #22515 ) ;
#51175=CARTESIAN_POINT ( 'NONE',  ( 35.00000000000000000, 11.72195762423409704, 0.7536123767498881243 ) ) ;
#51176=CARTESIAN_POINT ( 'NONE',  ( 35.00000000000000000, 11.78745411414844035, 3.093009498343795460 ) ) ;
#51178=VECTOR ( 'NONE', #57724, 1000.000000000000000 ) ;
#51179=CIRCLE ( 'NONE', #36297, 12.75000000000000178 ) ;
#51181=EDGE_LOOP ( 'NONE', ( #18017, #30612, #33878, #42592 ) ) ;
#51182=VERTEX_POINT ( 'NONE', #9238 ) ;
#51183=CARTESIAN_POINT ( 'NONE',  ( -29.72940237447408762, 1.708107138515393864, 11.88595848903394092 ) ) ;
#51184=ORIENTED_EDGE ( 'NONE', *, *, #48222, .F. ) ;
#51187=DIRECTION ( 'NONE',  ( 0.000000000000000000, 0.000000000000000000, -1.000000000000000000 ) ) ;
#51189=CARTESIAN_POINT ( 'NONE',  ( -35.00000000000000000, 8.839356091080043498, 8.389074212634319849 ) ) ;
#51190=CARTESIAN_POINT ( 'NONE',  ( -35.00000000000000000, -8.029056188533626681, -8.573591947375405198 ) ) ;
#51191=EDGE_LOOP ( 'NONE', ( #28913, #11761, #34915, #30874 ) ) ;
#51193=EDGE_LOOP ( 'NONE', ( #60150, #50340, #7782, #16028 ) ) ;
#51194=CARTESIAN_POINT ( 'NONE',  ( 8.937200413559436285, 4.816788486362209021, 12.61660635838017797 ) ) ;
#51195=CIRCLE ( 'NONE', #2352, 12.74999999999999822 ) ;
#51197=CIRCLE ( 'NONE', #15048, 12.75000000000000178 ) ;
#51199=ORIENTED_EDGE ( 'NONE', *, *, #49850, .T. ) ;
#51201=AXIS2_PLACEMENT_3D ( 'NONE', #19426, #34375, #49383 ) ;
#51203=EDGE_LOOP ( 'NONE', ( #9015, #10862, #31600, #37775 ) ) ;
#51204=CARTESIAN_POINT ( 'NONE',  ( 37.00000000000000711, -4.400442035670863561, 11.96656215839372983 ) ) ;
#51205=EDGE_CURVE ( 'NONE', #44528, #55692, #44659, .T. ) ;
#51208=CARTESIAN_POINT ( 'NONE',  ( 7.301893923874954062, -6.385938209748294625, 10.16239020806034432 ) ) ;
#51209=ORIENTED_EDGE ( 'NONE', *, *, #42029, .F. ) ;
#51211=VERTEX_POINT ( 'NONE', #14864 ) ;
#51213=ADVANCED_FACE ( 'NONE', ( #274 ), #35152, .T. ) ;
#51216=ORIENTED_EDGE ( 'NONE', *, *, #5099, .F. ) ;
#51217=CIRCLE ( 'NONE', #55308, 12.18650000000000055 ) ;
#51221=LINE ( 'NONE', #21256, #6084 ) ;
#51222=CYLINDRICAL_SURFACE ( 'NONE', #50129, 12.74999999999999822 ) ;
#51227=DIRECTION ( 'NONE',  ( -0.6334066780386838902, 0.000000000000000000, -0.7738190875236917732 ) ) ;
#51229=ORIENTED_EDGE ( 'NONE', *, *, #46880, .F. ) ;
#51230=CARTESIAN_POINT ( 'NONE',  ( 37.00000000000000711, 4.705694406421931860E-17, -3.469127814946512892E-15 ) ) ;
#51232=DIRECTION ( 'NONE',  ( 1.000000000000000000, 0.000000000000000000, -0.000000000000000000 ) ) ;
#51233=CARTESIAN_POINT ( 'NONE',  ( -27.46772105850581980, 13.11490794829154005, -3.249960617400303509 ) ) ;
#51234=CARTESIAN_POINT ( 'NONE',  ( 29.12484106848172161, 5.686051718212023154, 10.57743981609822903 ) ) ;
#51236=CIRCLE ( 'NONE', #36340, 12.75000000000000178 ) ;
#51238=VECTOR ( 'NONE', #34822, 1000.000000000000000 ) ;
#51240=CARTESIAN_POINT ( 'NONE',  ( -37.00000000000000711, 12.14284015767850100, 1.030638227056609679 ) ) ;
#51242=ORIENTED_EDGE ( 'NONE', *, *, #33124, .F. ) ;
#51246=CARTESIAN_POINT ( 'NONE',  ( -35.00000000000000000, -9.896810808925444292, 7.110831038798244741 ) ) ;
#51248=DIRECTION ( 'NONE',  ( 1.000000000000000000, 0.000000000000000000, 0.000000000000000000 ) ) ;
#51249=LINE ( 'NONE', #10322, #50328 ) ;
#51250=CARTESIAN_POINT ( 'NONE',  ( 21.76150723431516454, 10.89040160248869960, -5.054754920142551455 ) ) ;
#51252=CIRCLE ( 'NONE', #59723, 5.000000000000001776 ) ;
#51255=VECTOR ( 'NONE', #48195, 1000.000000000000000 ) ;
#51256=CYLINDRICAL_SURFACE ( 'NONE', #44517, 5.000000000000000888 ) ;
#51259=DIRECTION ( 'NONE',  ( -1.000000000000000000, 0.000000000000000000, 0.000000000000000000 ) ) ;
#51263=CYLINDRICAL_SURFACE ( 'NONE', #40592, 15.00000000000000000 ) ;
#51266=CARTESIAN_POINT ( 'NONE',  ( -2.952869152607111136, 7.581333670610111319, 11.17020052527586138 ) ) ;
#51269=AXIS2_PLACEMENT_3D ( 'NONE', #50604, #14655, #19999 ) ;
#51270=CIRCLE ( 'NONE', #45942, 5.000000000000000888 ) ;
#51271=ORIENTED_EDGE ( 'NONE', *, *, #58759, .T. ) ;
#51272=ORIENTED_EDGE ( 'NONE', *, *, #32366, .T. ) ;
#51277=EDGE_CURVE ( 'NONE', #23800, #36879, #10088, .T. ) ;
#51279=FACE_OUTER_BOUND ( 'NONE', #28217, .T. ) ;
#51280=CYLINDRICAL_SURFACE ( 'NONE', #13024, 12.18649999999999878 ) ;
#51282=( BOUNDED_CURVE ( )  B_SPLINE_CURVE ( 3, ( #32948, #3059, #23321, #3733 ),
 .UNSPECIFIED., .F., .F. ) 
 B_SPLINE_CURVE_WITH_KNOTS ( ( 4, 4 ),
 ( 5.358943115472171392, 5.400987736605186385 ),
 .UNSPECIFIED. ) 
 CURVE ( )  GEOMETRIC_REPRESENTATION_ITEM ( )  RATIONAL_B_SPLINE_CURVE ( ( 1.000000000000000000, 0.9998526929113126238, 0.9998526929113126238, 1.000000000000000000 ) ) 
 REPRESENTATION_ITEM ( '' )  );
#51284=EDGE_CURVE ( 'NONE', #36860, #32235, #15998, .T. ) ;
#51289=EDGE_CURVE ( 'NONE', #60763, #64737, #53190, .T. ) ;
#51290=VERTEX_POINT ( 'NONE', #26504 ) ;
#51295=CARTESIAN_POINT ( 'NONE',  ( -37.00000000000000711, 0.000000000000000000, 0.000000000000000000 ) ) ;
#51296=VECTOR ( 'NONE', #20591, 1000.000000000000000 ) ;
#51297=DIRECTION ( 'NONE',  ( -1.000000000000000000, -0.000000000000000000, -0.000000000000000000 ) ) ;
#51299=DIRECTION ( 'NONE',  ( 1.000000000000000000, -0.000000000000000000, 0.000000000000000000 ) ) ;
#51300=EDGE_CURVE ( 'NONE', #21470, #22647, #2258, .T. ) ;
#51301=DIRECTION ( 'NONE',  ( 1.000000000000000000, 0.000000000000000000, -0.000000000000000000 ) ) ;
#51302=CARTESIAN_POINT ( 'NONE',  ( 9.088549504245943211, 6.815555982525443923, -9.878547223985661319 ) ) ;
#51303=DIRECTION ( 'NONE',  ( 0.000000000000000000, -0.9937233664769749009, 0.1118654143051720229 ) ) ;
#51304=EDGE_LOOP ( 'NONE', ( #11741, #13769, #15491, #64226 ) ) ;
#51305=CARTESIAN_POINT ( 'NONE',  ( -37.00000000000000711, 10.14433819232434253, 6.753013023069750709 ) ) ;
#51306=ORIENTED_EDGE ( 'NONE', *, *, #56208, .F. ) ;
#51309=CIRCLE ( 'NONE', #4593, 4.999999999999999112 ) ;
#51310=DIRECTION ( 'NONE',  ( -1.000000000000000000, 0.000000000000000000, 0.000000000000000000 ) ) ;
#51311=ORIENTED_EDGE ( 'NONE', *, *, #7691, .F. ) ;
#51314=CARTESIAN_POINT ( 'NONE',  ( 35.00000000000000000, -6.036400161834636791, -10.07641281632175634 ) ) ;
#51315=FACE_OUTER_BOUND ( 'NONE', #13616, .T. ) ;
#51316=CARTESIAN_POINT ( 'NONE',  ( 35.00000000000000000, -5.814360711498364864, -10.70999494708490829 ) ) ;
#51317=ORIENTED_EDGE ( 'NONE', *, *, #11714, .T. ) ;
#51318=DIRECTION ( 'NONE',  ( 1.000000000000000000, -0.000000000000000000, 0.000000000000000000 ) ) ;
#51319=ADVANCED_FACE ( 'NONE', ( #10890 ), #51487, .T. ) ;
#51320=ORIENTED_EDGE ( 'NONE', *, *, #36603, .T. ) ;
#51322=EDGE_CURVE ( 'NONE', #17416, #9772, #21186, .T. ) ;
#51323=FACE_OUTER_BOUND ( 'NONE', #62839, .T. ) ;
#51324=CARTESIAN_POINT ( 'NONE',  ( -37.00000000000000711, 0.000000000000000000, 0.000000000000000000 ) ) ;
#51325=EDGE_LOOP ( 'NONE', ( #53597, #36794, #29719, #60560 ) ) ;
#51326=AXIS2_PLACEMENT_3D ( 'NONE', #58547, #17967, #53561 ) ;
#51328=CARTESIAN_POINT ( 'NONE',  ( -35.00000000000000000, -11.65150730582933392, -1.488153103997089888 ) ) ;
#51329=AXIS2_PLACEMENT_3D ( 'NONE', #3018, #23279, #49550 ) ;
#51331=LINE ( 'NONE', #40998, #52178 ) ;
#51333=CARTESIAN_POINT ( 'NONE',  ( 9.883521448361594963, 7.802028015148476214, 11.02197474982682124 ) ) ;
#51340=CARTESIAN_POINT ( 'NONE',  ( -16.78077304548816429, 7.535057906616318135, 11.20259948750489976 ) ) ;
#51341=CARTESIAN_POINT ( 'NONE',  ( 17.36552780755588543, -11.88930279851165928, 6.437067910676037563 ) ) ;
#51342=AXIS2_PLACEMENT_3D ( 'NONE', #59280, #23372, #12390 ) ;
#51343=ORIENTED_EDGE ( 'NONE', *, *, #30588, .F. ) ;
#51346=CYLINDRICAL_SURFACE ( 'NONE', #14083, 12.18650000000000055 ) ;
#51347=AXIS2_PLACEMENT_3D ( 'NONE', #25946, #60859, #36219 ) ;
#51349=ORIENTED_EDGE ( 'NONE', *, *, #42329, .F. ) ;
#51350=CARTESIAN_POINT ( 'NONE',  ( -17.68824251889582655, 2.869235522687681339, 11.65378641629914647 ) ) ;
#51351=LINE ( 'NONE', #31677, #187 ) ;
#51353=ADVANCED_FACE ( 'NONE', ( #48995 ), #3452, .T. ) ;
#51354=ORIENTED_EDGE ( 'NONE', *, *, #65168, .T. ) ;
#51355=ORIENTED_EDGE ( 'NONE', *, *, #31828, .F. ) ;
#51356=CARTESIAN_POINT ( 'NONE',  ( 145.1370849898475797, 3.309064568108273190E-14, 0.000000000000000000 ) ) ;
#51357=VECTOR ( 'NONE', #54952, 1000.000000000000000 ) ;
#51359=ORIENTED_EDGE ( 'NONE', *, *, #31378, .T. ) ;
#51362=CARTESIAN_POINT ( 'NONE',  ( -35.00000000000000000, -8.235637554476575417, -9.733281772932249609 ) ) ;
#51363=DIRECTION ( 'NONE',  ( 1.000000000000000000, -0.000000000000000000, 0.000000000000000000 ) ) ;
#51368=ORIENTED_EDGE ( 'NONE', *, *, #49573, .F. ) ;
#51369=B_SPLINE_CURVE_WITH_KNOTS ( 'NONE', 3,
 ( #34221, #65134, #49542, #55157 ),
 .UNSPECIFIED., .F., .F.,
 ( 4, 4 ),
 ( 0.000000000000000000, 0.002277974501771297573 ),
 .UNSPECIFIED. ) ;
#51373=AXIS2_PLACEMENT_3D ( 'NONE', #65513, #5699, #50261 ) ;
#51376=AXIS2_PLACEMENT_3D ( 'NONE', #18422, #58991, #13402 ) ;
#51380=CIRCLE ( 'NONE', #36494, 5.000000000000000888 ) ;
#51381=LINE ( 'NONE', #22067, #35384 ) ;
#51382=ORIENTED_EDGE ( 'NONE', *, *, #53609, .F. ) ;
#51383=DIRECTION ( 'NONE',  ( 1.000000000000000000, -0.000000000000000000, 0.000000000000000000 ) ) ;
#51385=ORIENTED_EDGE ( 'NONE', *, *, #28156, .T. ) ;
#51390=AXIS2_PLACEMENT_3D ( 'NONE', #46553, #25960, #20640 ) ;
#51391=ADVANCED_FACE ( 'NONE', ( #43988 ), #64262, .T. ) ;
#51392=ORIENTED_EDGE ( 'NONE', *, *, #38434, .T. ) ;
#51396=DIRECTION ( 'NONE',  ( 1.000000000000000000, 0.000000000000000000, 0.000000000000000000 ) ) ;
#51397=CARTESIAN_POINT ( 'NONE',  ( 17.53254851291653438, -7.812843716768262503, 9.123340610460312305 ) ) ;
#51398=EDGE_CURVE ( 'NONE', #26437, #22263, #22732, .T. ) ;
#51399=VECTOR ( 'NONE', #144, 1000.000000000000000 ) ;
#51401=EDGE_CURVE ( 'NONE', #60526, #45531, #38366, .T. ) ;
#51402=DIRECTION ( 'NONE',  ( 1.000000000000000000, 0.000000000000000000, 0.000000000000000000 ) ) ;
#51403=CIRCLE ( 'NONE', #63042, 12.18649999999999878 ) ;
#51405=VECTOR ( 'NONE', #36124, 1000.000000000000000 ) ;
#51406=EDGE_CURVE ( 'NONE', #26022, #43321, #19250, .T. ) ;
#51410=DIRECTION ( 'NONE',  ( 0.000000000000000000, -0.01356324068817998940, 0.9999080150203990547 ) ) ;
#51413=CARTESIAN_POINT ( 'NONE',  ( 35.00000000000000000, -11.73463472867578083, -3.287724142101374092 ) ) ;
#51414=CARTESIAN_POINT ( 'NONE',  ( 3.986618437605343512, 6.992948023114762712, -9.794201124374950496 ) ) ;
#51416=ORIENTED_EDGE ( 'NONE', *, *, #41297, .T. ) ;
#51417=AXIS2_PLACEMENT_3D ( 'NONE', #65695, #9858, #14822 ) ;
#51420=CIRCLE ( 'NONE', #11058, 5.000000000000000888 ) ;
#51422=AXIS2_PLACEMENT_3D ( 'NONE', #37405, #31114, #6843 ) ;
#51423=EDGE_CURVE ( 'NONE', #23040, #6900, #54287, .T. ) ;
#51425=LINE ( 'NONE', #5537, #50027 ) ;
#51426=CIRCLE ( 'NONE', #1497, 12.75000000000000178 ) ;
#51427=ORIENTED_EDGE ( 'NONE', *, *, #4328, .F. ) ;
#51428=CARTESIAN_POINT ( 'NONE',  ( -17.36985044138108947, -8.809625639090254978, -10.23436652272288505 ) ) ;
#51431=VERTEX_POINT ( 'NONE', #23625 ) ;
#51432=CARTESIAN_POINT ( 'NONE',  ( -37.00000000000000711, -8.954052073409537016, -9.076753354954096409 ) ) ;
#51433=CARTESIAN_POINT ( 'NONE',  ( -37.00000000000000711, 7.817492529713987004, -9.348667969174327297 ) ) ;
#51434=AXIS2_PLACEMENT_3D ( 'NONE', #56716, #41717, #10800 ) ;
#51436=DIRECTION ( 'NONE',  ( 1.000000000000000000, -0.000000000000000000, 0.000000000000000000 ) ) ;
#51437=VERTEX_POINT ( 'NONE', #63501 ) ;
#51438=CARTESIAN_POINT ( 'NONE',  ( 35.00000000000000000, -10.91536515067650903, -4.339012074899918581 ) ) ;
#51439=VECTOR ( 'NONE', #48341, 1000.000000000000000 ) ;
#51440=CYLINDRICAL_SURFACE ( 'NONE', #36107, 5.000000000000000888 ) ;
#51441=ORIENTED_EDGE ( 'NONE', *, *, #8111, .F. ) ;
#51442=FACE_OUTER_BOUND ( 'NONE', #21542, .T. ) ;
#51443=FACE_OUTER_BOUND ( 'NONE', #48194, .T. ) ;
#51444=CARTESIAN_POINT ( 'NONE',  ( -35.00000000000000000, 0.000000000000000000, 0.000000000000000000 ) ) ;
#51445=DIRECTION ( 'NONE',  ( 1.000000000000000000, -0.000000000000000000, 0.000000000000000000 ) ) ;
#51446=CARTESIAN_POINT ( 'NONE',  ( -9.721193118338453232, 9.581699509156610617, -7.227512093013982231 ) ) ;
#51447=VECTOR ( 'NONE', #4067, 1000.000000000000000 ) ;
#51450=ORIENTED_EDGE ( 'NONE', *, *, #37587, .T. ) ;
#51452=ORIENTED_EDGE ( 'NONE', *, *, #52702, .F. ) ;
#51453=CARTESIAN_POINT ( 'NONE',  ( -35.00000000000000000, -8.573591947375380329, 8.029056188533655103 ) ) ;
#51454=EDGE_LOOP ( 'NONE', ( #19120, #46849, #32494, #32308 ) ) ;
#51457=DIRECTION ( 'NONE',  ( 0.000000000000000000, -0.8009703041134103030, -0.5987040770935764256 ) ) ;
#51458=CIRCLE ( 'NONE', #41835, 5.000000000000000888 ) ;
#51459=CYLINDRICAL_SURFACE ( 'NONE', #1257, 4.999999999999999112 ) ;
#51460=EDGE_LOOP ( 'NONE', ( #57116, #52361, #21325, #54559 ) ) ;
#51461=CYLINDRICAL_SURFACE ( 'NONE', #15960, 4.999999999999999112 ) ;
#51462=DIRECTION ( 'NONE',  ( 0.000000000000000000, -0.01356324068817992175, 0.9999080150203990547 ) ) ;
#51463=CYLINDRICAL_SURFACE ( 'NONE', #28689, 4.999999999999998224 ) ;
#51466=CARTESIAN_POINT ( 'NONE',  ( -8.891032880924177206, 25.00000000000000000, -3.860857758255646921 ) ) ;
#51467=AXIS2_PLACEMENT_3D ( 'NONE', #52661, #32017, #1786 ) ;
#51468=AXIS2_PLACEMENT_3D ( 'NONE', #36080, #22117, #11170 ) ;
#51470=CYLINDRICAL_SURFACE ( 'NONE', #38050, 12.75000000000000178 ) ;
#51472=CARTESIAN_POINT ( 'NONE',  ( -35.00000000000000000, 3.614449339633491576, 11.17622378668007777 ) ) ;
#51475=DIRECTION ( 'NONE',  ( 1.000000000000000000, 0.000000000000000000, 0.000000000000000000 ) ) ;
#51478=EDGE_CURVE ( 'NONE', #3297, #25143, #13944, .T. ) ;
#51480=EDGE_LOOP ( 'NONE', ( #21487, #7084, #49698, #26902 ) ) ;
#51482=EDGE_CURVE ( 'NONE', #21758, #47524, #40443, .T. ) ;
#51483=CARTESIAN_POINT ( 'NONE',  ( 21.94787173280690240, 11.49320247778055837, -3.471189377931829245 ) ) ;
#51484=CARTESIAN_POINT ( 'NONE',  ( -27.25047371082987624, 12.34411773464382023, 5.468532507261041786 ) ) ;
#51485=CARTESIAN_POINT ( 'NONE',  ( 35.00000000000000000, 4.705694406421931860E-17, -3.469127814946512892E-15 ) ) ;
#51486=CARTESIAN_POINT ( 'NONE',  ( -2.816255946208524374, 7.711081843936713476, 11.08213906273406657 ) ) ;
#51487=CYLINDRICAL_SURFACE ( 'NONE', #63799, 4.999999999999999112 ) ;
#51488=DIRECTION ( 'NONE',  ( 0.000000000000000000, 0.6269146997507987207, 0.7790879021242504976 ) ) ;
#51490=CIRCLE ( 'NONE', #46159, 12.75000000000000178 ) ;
#51491=VERTEX_POINT ( 'NONE', #58211 ) ;
#51492=ORIENTED_EDGE ( 'NONE', *, *, #59003, .T. ) ;
#51493=CARTESIAN_POINT ( 'NONE',  ( -36.00000000000000711, -3.307597835713157242, -12.31350058095526911 ) ) ;
#51495=( BOUNDED_CURVE ( )  B_SPLINE_CURVE ( 3, ( #65088, #15206, #15528, #30179 ),
 .UNSPECIFIED., .F., .F. ) 
 B_SPLINE_CURVE_WITH_KNOTS ( ( 4, 4 ),
 ( 2.185177278367677278, 2.228289365106483899 ),
 .UNSPECIFIED. ) 
 CURVE ( )  GEOMETRIC_REPRESENTATION_ITEM ( )  RATIONAL_B_SPLINE_CURVE ( ( 1.000000000000000000, 0.9998451183288734612, 0.9998451183288734612, 1.000000000000000000 ) ) 
 REPRESENTATION_ITEM ( '' )  );
#51505=CARTESIAN_POINT ( 'NONE',  ( 8.990732662897594096, 5.150069606959243096, -12.48035402102856217 ) ) ;
#51506=EDGE_CURVE ( 'NONE', #64097, #54202, #20291, .T. ) ;
#51508=VERTEX_POINT ( 'NONE', #64181 ) ;
#51509=DIRECTION ( 'NONE',  ( -1.000000000000000000, 0.000000000000000000, 0.000000000000000000 ) ) ;
#51510=ORIENTED_EDGE ( 'NONE', *, *, #53472, .T. ) ;
#51511=CARTESIAN_POINT ( 'NONE',  ( -37.00000000000000711, 4.400442035671113139, -11.96656215839364457 ) ) ;
#51514=CIRCLE ( 'NONE', #63166, 5.000000000000000888 ) ;
#51515=CYLINDRICAL_SURFACE ( 'NONE', #17959, 4.999999999999999112 ) ;
#51516=DIRECTION ( 'NONE',  ( 1.000000000000000000, 0.000000000000000000, 0.000000000000000000 ) ) ;
#51517=ORIENTED_EDGE ( 'NONE', *, *, #62290, .F. ) ;
#51525=LINE ( 'NONE', #40186, #35182 ) ;
#51527=CARTESIAN_POINT ( 'NONE',  ( -35.00000000000000000, 0.000000000000000000, 0.000000000000000000 ) ) ;
#51529=CARTESIAN_POINT ( 'NONE',  ( -5.883084918421578990, -0.9869286070152175627, 11.95978564732913974 ) ) ;
#51530=ORIENTED_EDGE ( 'NONE', *, *, #41222, .F. ) ;
#51531=ADVANCED_FACE ( 'NONE', ( #33908 ), #18653, .T. ) ;
#51532=EDGE_CURVE ( 'NONE', #27983, #23644, #28933, .T. ) ;
#51534=ORIENTED_EDGE ( 'NONE', *, *, #46840, .T. ) ;
#51537=CARTESIAN_POINT ( 'NONE',  ( 21.90174657591892071, -13.47998113580522528, -0.7349207973210680755 ) ) ;
#51538=DIRECTION ( 'NONE',  ( -1.000000000000000000, 0.000000000000000000, 0.000000000000000000 ) ) ;
#51539=ORIENTED_EDGE ( 'NONE', *, *, #11386, .T. ) ;
#51542=FACE_OUTER_BOUND ( 'NONE', #61469, .T. ) ;
#51547=VERTEX_POINT ( 'NONE', #60829 ) ;
#51548=CARTESIAN_POINT ( 'NONE',  ( -35.00000000000000000, 0.000000000000000000, 0.000000000000000000 ) ) ;
#51549=ORIENTED_EDGE ( 'NONE', *, *, #1635, .F. ) ;
#51550=DIRECTION ( 'NONE',  ( 0.000000000000000000, -0.01356324068817998940, 0.9999080150203990547 ) ) ;
#51551=ORIENTED_EDGE ( 'NONE', *, *, #4975, .T. ) ;
#51552=ORIENTED_EDGE ( 'NONE', *, *, #2328, .F. ) ;
#51553=ORIENTED_EDGE ( 'NONE', *, *, #36841, .F. ) ;
#51555=ADVANCED_FACE ( 'NONE', ( #54860 ), #4669, .T. ) ;
#51557=AXIS2_PLACEMENT_3D ( 'NONE', #17367, #47620, #31650 ) ;
#51559=DIRECTION ( 'NONE',  ( -1.000000000000000000, 0.000000000000000000, 0.000000000000000000 ) ) ;
#51563=DIRECTION ( 'NONE',  ( 0.000000000000000000, 0.7617968321374901652, 0.6478160128811921714 ) ) ;
#51565=CARTESIAN_POINT ( 'NONE',  ( 2.798553295784531159, 25.00000000000000000, 7.462808788758677814 ) ) ;
#51567=CARTESIAN_POINT ( 'NONE',  ( 29.19404894130743600, 6.482428994453312221, 10.10898271525048386 ) ) ;
#51569=EDGE_CURVE ( 'NONE', #40556, #32142, #36224, .T. ) ;
#51572=VERTEX_POINT ( 'NONE', #39556 ) ;
#51576=CARTESIAN_POINT ( 'NONE',  ( -37.00000000000000711, 0.000000000000000000, 0.000000000000000000 ) ) ;
#51579=FACE_OUTER_BOUND ( 'NONE', #24611, .T. ) ;
#51580=CARTESIAN_POINT ( 'NONE',  ( -36.00000000000000711, -7.745827850122939395, -10.12742074351904975 ) ) ;
#51582=LINE ( 'NONE', #6992, #41246 ) ;
#51583=AXIS2_PLACEMENT_3D ( 'NONE', #39232, #28943, #12991 ) ;
#51587=CARTESIAN_POINT ( 'NONE',  ( -37.00000000000000711, 4.983891302653582933, 11.73555825188278590 ) ) ;
#51588=CARTESIAN_POINT ( 'NONE',  ( -18.49080574448680991, -12.00000000000057909, -4.407108900774715188E-13 ) ) ;
#51589=PLANE ( 'NONE',  #31184 ) ;
#51590=VECTOR ( 'NONE', #45168, 1000.000000000000000 ) ;
#51591=EDGE_CURVE ( 'NONE', #52926, #46774, #55546, .T. ) ;
#51593=ORIENTED_EDGE ( 'NONE', *, *, #3144, .F. ) ;
#51596=CARTESIAN_POINT ( 'NONE',  ( -29.92777678363736626, -3.750539801530011985, 25.00000000000000000 ) ) ;
#51597=B_SPLINE_CURVE_WITH_KNOTS ( 'NONE', 3,
 ( #53217, #42219, #16652, #36923, #2362, #32574 ),
 .UNSPECIFIED., .F., .F.,
 ( 4, 2, 4 ),
 ( 0.005162059057943477365, 0.006293711021387341994, 0.007425362984831206624 ),
 .UNSPECIFIED. ) ;
#51600=EDGE_CURVE ( 'NONE', #43974, #31785, #60166, .T. ) ;
#51601=ORIENTED_EDGE ( 'NONE', *, *, #11386, .F. ) ;
#51602=EDGE_LOOP ( 'NONE', ( #35563, #43147, #59984, #59447 ) ) ;
#51604=LINE ( 'NONE', #62521, #30202 ) ;
#51605=DIRECTION ( 'NONE',  ( 0.000000000000000000, -0.01356324068817992175, 0.9999080150203990547 ) ) ;
#51607=CARTESIAN_POINT ( 'NONE',  ( -17.32524154617501821, 3.215141440730553413, -11.56265422116751296 ) ) ;
#51608=CYLINDRICAL_SURFACE ( 'NONE', #7714, 5.000000000000000888 ) ;
#51610=CIRCLE ( 'NONE', #60084, 12.18650000000000055 ) ;
#51613=DIRECTION ( 'NONE',  ( 1.000000000000000000, 0.000000000000000000, 0.000000000000000000 ) ) ;
#51614=ORIENTED_EDGE ( 'NONE', *, *, #592, .T. ) ;
#51616=VERTEX_POINT ( 'NONE', #14590 ) ;
#51617=CARTESIAN_POINT ( 'NONE',  ( -35.00000000000000000, 12.42372387097882402, 2.865935305911668785 ) ) ;
#51619=CARTESIAN_POINT ( 'NONE',  ( -36.00000000000000711, 11.39945968423479883, -5.710938531231587234 ) ) ;
#51620=CIRCLE ( 'NONE', #38890, 5.000000000000000888 ) ;
#51623=CARTESIAN_POINT ( 'NONE',  ( 35.00000000000000000, -9.493370459201747380, -6.917234959366797220 ) ) ;
#51625=DIRECTION ( 'NONE',  ( 0.000000000000000000, -0.9467777615094538080, -0.3218879778916074463 ) ) ;
#51626=DIRECTION ( 'NONE',  ( 0.000000000000000000, -0.9718671068226484300, 0.2355298848897411923 ) ) ;
#51628=CARTESIAN_POINT ( 'NONE',  ( 6.916391019076965740, -8.217520853910727396, 10.71822957364710760 ) ) ;
#51629=ORIENTED_EDGE ( 'NONE', *, *, #31465, .T. ) ;
#51630=CARTESIAN_POINT ( 'NONE',  ( -37.00000000000000711, -11.44858830469742017, 2.627174906296871448 ) ) ;
#51631=ORIENTED_EDGE ( 'NONE', *, *, #48769, .F. ) ;
#51632=CARTESIAN_POINT ( 'NONE',  ( -35.00000000000000000, -7.379373053628940582, 10.39746860227888092 ) ) ;
#51633=CARTESIAN_POINT ( 'NONE',  ( 35.00000000000000000, 4.824807283154291859, 11.80185301892974969 ) ) ;
#51634=ADVANCED_FACE ( 'NONE', ( #34867 ), #4982, .T. ) ;
#51636=CARTESIAN_POINT ( 'NONE',  ( -37.00000000000000711, -7.882940143791846488, 10.02106554660705839 ) ) ;
#51639=DIRECTION ( 'NONE',  ( 0.000000000000000000, 0.8369827122275325104, 0.5472293298355301872 ) ) ;
#51640=EDGE_CURVE ( 'NONE', #28779, #53475, #7560, .T. ) ;
#51643=CARTESIAN_POINT ( 'NONE',  ( 47.00000000000000711, 4.705694406421931860E-17, -3.469127814946512892E-15 ) ) ;
#51644=ORIENTED_EDGE ( 'NONE', *, *, #32847, .T. ) ;
#51647=DIRECTION ( 'NONE',  ( -1.000000000000000000, 0.000000000000000000, 0.000000000000000000 ) ) ;
#51649=CARTESIAN_POINT ( 'NONE',  ( 37.00000000000000711, 11.50504120060948487, 4.018060380616274685 ) ) ;
#51650=EDGE_CURVE ( 'NONE', #12997, #29569, #32431, .T. ) ;
#51651=AXIS2_PLACEMENT_3D ( 'NONE', #49970, #51942, #47289 ) ;
#51652=CIRCLE ( 'NONE', #43121, 12.75000000000000178 ) ;
#51653=EDGE_CURVE ( 'NONE', #31409, #46540, #37270, .T. ) ;
#51656=EDGE_CURVE ( 'NONE', #37945, #40578, #23473, .T. ) ;
#51657=CARTESIAN_POINT ( 'NONE',  ( 37.00000000000000711, 3.640372113593552061, -12.21925492305363647 ) ) ;
#51658=CARTESIAN_POINT ( 'NONE',  ( 8.437200413559441614, 4.476360154859203355, 12.73625532737111143 ) ) ;
#51660=CARTESIAN_POINT ( 'NONE',  ( -35.00000000000000000, 1.286231064351496034, -12.68495603654570303 ) ) ;
#51664=VERTEX_POINT ( 'NONE', #48415 ) ;
#51665=CARTESIAN_POINT ( 'NONE',  ( -17.57519261785461850, 6.782244033140607087, 11.67428159032847645 ) ) ;
#51666=CARTESIAN_POINT ( 'NONE',  ( 6.574848435243071165, -7.682001007202829079, 11.10271414525420575 ) ) ;
#51667=( BOUNDED_CURVE ( )  B_SPLINE_CURVE ( 3, ( #4992, #45528, #45216, #65476 ),
 .UNSPECIFIED., .F., .F. ) 
 B_SPLINE_CURVE_WITH_KNOTS ( ( 4, 4 ),
 ( 1.062823956857581464, 1.069007632545065700 ),
 .UNSPECIFIED. ) 
 CURVE ( )  GEOMETRIC_REPRESENTATION_ITEM ( )  RATIONAL_B_SPLINE_CURVE ( ( 1.000000000000000000, 0.9999968135154544413, 0.9999968135154544413, 1.000000000000000000 ) ) 
 REPRESENTATION_ITEM ( '' )  );
#51668=ORIENTED_EDGE ( 'NONE', *, *, #31987, .T. ) ;
#51669=CARTESIAN_POINT ( 'NONE',  ( -37.00000000000000711, 10.68873102412852560, -6.950793414699682593 ) ) ;
#51670=EDGE_CURVE ( 'NONE', #38324, #32833, #45975, .T. ) ;
#51671=CARTESIAN_POINT ( 'NONE',  ( -17.83419946441818027, -9.720786832536937538, 25.00000000000000000 ) ) ;
#51672=CARTESIAN_POINT ( 'NONE',  ( -9.464296738015105959, 10.76059690970763505, -8.161180804017673651 ) ) ;
#51673=VERTEX_POINT ( 'NONE', #63345 ) ;
#51674=DIRECTION ( 'NONE',  ( 0.000000000000000000, -0.8827602140260366603, 0.4698238015817268187 ) ) ;
#51675=ORIENTED_EDGE ( 'NONE', *, *, #33821, .T. ) ;
#51677=EDGE_LOOP ( 'NONE', ( #10915, #17972, #25764, #337 ) ) ;
#51679=CARTESIAN_POINT ( 'NONE',  ( -35.00000000000000000, -12.17626345777664021, 0.4993900848166987760 ) ) ;
#51680=ORIENTED_EDGE ( 'NONE', *, *, #60786, .F. ) ;
#51682=CARTESIAN_POINT ( 'NONE',  ( -25.27109080293329413, -9.776000194394919518, 6.961263260165105216 ) ) ;
#51684=CARTESIAN_POINT ( 'NONE',  ( 37.00000000000000711, -1.908798535168467536, -12.60630747491662618 ) ) ;
#51685=CARTESIAN_POINT ( 'NONE',  ( -37.00000000000000711, 10.42955799785328708, -6.303578524886837009 ) ) ;
#51686=VERTEX_POINT ( 'NONE', #15586 ) ;
#51687=CARTESIAN_POINT ( 'NONE',  ( 37.00000000000000711, 7.608228585767871976, 10.23119532541064203 ) ) ;
#51689=CARTESIAN_POINT ( 'NONE',  ( -35.00000000000000000, 11.74614673114903951, 0.01609748574465447862 ) ) ;
#51690=FACE_OUTER_BOUND ( 'NONE', #17974, .T. ) ;
#51695=VERTEX_POINT ( 'NONE', #47432 ) ;
#51697=AXIS2_PLACEMENT_3D ( 'NONE', #27978, #11676, #37621 ) ;
#51698=DIRECTION ( 'NONE',  ( 0.000000000000000000, 0.3807014730195219521, -0.9246979985058723095 ) ) ;
#51700=DIRECTION ( 'NONE',  ( -1.000000000000000000, 0.000000000000000000, 0.000000000000000000 ) ) ;
#51701=ORIENTED_EDGE ( 'NONE', *, *, #358, .T. ) ;
#51702=FACE_OUTER_BOUND ( 'NONE', #26008, .T. ) ;
#51704=CYLINDRICAL_SURFACE ( 'NONE', #57974, 5.000000000000000888 ) ;
#51706=ORIENTED_EDGE ( 'NONE', *, *, #30663, .F. ) ;
#51707=ORIENTED_EDGE ( 'NONE', *, *, #64842, .F. ) ;
#51708=DIRECTION ( 'NONE',  ( -1.000000000000000000, 0.000000000000000000, 0.000000000000000000 ) ) ;
#51710=ORIENTED_EDGE ( 'NONE', *, *, #47251, .T. ) ;
#51713=CARTESIAN_POINT ( 'NONE',  ( 37.00000000000000711, 2.346765782874432382, -11.95840593935202278 ) ) ;
#51716=EDGE_CURVE ( 'NONE', #19597, #2444, #5446, .T. ) ;
#51718=DIRECTION ( 'NONE',  ( -0.2415534870330798278, 0.000000000000000000, 0.9703875065674330003 ) ) ;
#51719=ORIENTED_EDGE ( 'NONE', *, *, #60208, .F. ) ;
#51721=DIRECTION ( 'NONE',  ( -1.000000000000000000, -0.000000000000000000, 0.000000000000000000 ) ) ;
#51725=CIRCLE ( 'NONE', #10313, 4.999999999999998224 ) ;
#51726=CARTESIAN_POINT ( 'NONE',  ( 35.00000000000000000, 2.216820770815085773, -11.53507381115584529 ) ) ;
#51728=CARTESIAN_POINT ( 'NONE',  ( 3.627734094270521403, 4.214566690872760368, -11.24377562339657999 ) ) ;
#51729=CARTESIAN_POINT ( 'NONE',  ( 11.38592777356517871, 0.2429536942619314188, -11.99780484965632077 ) ) ;
#51730=EDGE_CURVE ( 'NONE', #2297, #24257, #8610, .T. ) ;
#51732=LINE ( 'NONE', #47399, #19576 ) ;
#51733=CARTESIAN_POINT ( 'NONE',  ( -47.00000000000000711, 0.000000000000000000, 0.000000000000000000 ) ) ;
#51734=DIRECTION ( 'NONE',  ( 0.000000000000000000, -0.01356324068817998940, 0.9999080150203990547 ) ) ;
#51736=CIRCLE ( 'NONE', #8198, 12.75000000000000178 ) ;
#51737=CARTESIAN_POINT ( 'NONE',  ( 9.778943843942252911, 2.009314548101766462, -13.35093242851569784 ) ) ;
#51740=CARTESIAN_POINT ( 'NONE',  ( -35.00000000000000000, 10.07641281632186114, -6.036400161834460043 ) ) ;
#51741=CYLINDRICAL_SURFACE ( 'NONE', #14221, 12.18649999999999878 ) ;
#51744=ORIENTED_EDGE ( 'NONE', *, *, #58418, .F. ) ;
#51746=CARTESIAN_POINT ( 'NONE',  ( -17.58536674675198341, 6.767421432155036776, -9.911758545779559171 ) ) ;
#51747=CARTESIAN_POINT ( 'NONE',  ( 37.00000000000000711, 4.705694406421931860E-17, -3.469127814946512892E-15 ) ) ;
#51748=ADVANCED_FACE ( 'NONE', ( #18497 ), #49078, .T. ) ;
#51750=ORIENTED_EDGE ( 'NONE', *, *, #13172, .F. ) ;
#51754=ORIENTED_EDGE ( 'NONE', *, *, #6642, .F. ) ;
#51755=ADVANCED_FACE ( 'NONE', ( #13459 ), #39389, .T. ) ;
#51756=DIRECTION ( 'NONE',  ( 0.000000000000000000, -0.01356324068817998940, 0.9999080150203990547 ) ) ;
#51757=LINE ( 'NONE', #16503, #2239 ) ;
#51758=CARTESIAN_POINT ( 'NONE',  ( 35.00000000000000000, -12.71517666308947092, 0.9416912585475696318 ) ) ;
#51759=CARTESIAN_POINT ( 'NONE',  ( -3.347463755625758264, -12.75767721842421665, 4.430665912812002283 ) ) ;
#51760=CARTESIAN_POINT ( 'NONE',  ( -9.264327559741124318, 8.341203664785947325, -8.636428847717205315 ) ) ;
#51761=EDGE_CURVE ( 'NONE', #30430, #50238, #23519, .T. ) ;
#51763=LINE ( 'NONE', #45774, #28672 ) ;
#51764=ORIENTED_EDGE ( 'NONE', *, *, #24533, .T. ) ;
#51765=ORIENTED_EDGE ( 'NONE', *, *, #46475, .T. ) ;
#51766=CARTESIAN_POINT ( 'NONE',  ( 24.89709673309864257, -0.9453300160761306525, -11.96437408882576925 ) ) ;
#51767=ORIENTED_EDGE ( 'NONE', *, *, #52516, .F. ) ;
#51770=CARTESIAN_POINT ( 'NONE',  ( -17.71793285162545928, 3.743050124886382335, 11.40313316626405182 ) ) ;
#51771=CARTESIAN_POINT ( 'NONE',  ( 35.00000000000000000, -7.882940143791697274, 10.02106554660716853 ) ) ;
#51772=ORIENTED_EDGE ( 'NONE', *, *, #26860, .T. ) ;
#51774=CYLINDRICAL_SURFACE ( 'NONE', #24097, 5.000000000000000888 ) ;
#51775=CARTESIAN_POINT ( 'NONE',  ( -35.00000000000000000, 0.000000000000000000, 0.000000000000000000 ) ) ;
#51777=ORIENTED_EDGE ( 'NONE', *, *, #34994, .F. ) ;
#51778=CARTESIAN_POINT ( 'NONE',  ( 29.03109630806826758, -11.07829921360117353, 7.725641260898457041 ) ) ;
#51780=CARTESIAN_POINT ( 'NONE',  ( 21.94670809694110147, -11.54116911556738145, -3.292040187117030392 ) ) ;
#51781=AXIS2_PLACEMENT_3D ( 'NONE', #58081, #62082, #31486 ) ;
#51785=EDGE_CURVE ( 'NONE', #62115, #49238, #4500, .T. ) ;
#51786=DIRECTION ( 'NONE',  ( -1.000000000000000000, 0.000000000000000000, 0.000000000000000000 ) ) ;
#51787=CARTESIAN_POINT ( 'NONE',  ( 36.00000000000000711, -10.84030624090611283, -6.711949091238110121 ) ) ;
#51789=LINE ( 'NONE', #61406, #1514 ) ;
#51791=CYLINDRICAL_SURFACE ( 'NONE', #1878, 12.18650000000000055 ) ;
#51793=CARTESIAN_POINT ( 'NONE',  ( 37.00000000000000711, 4.705694406421931860E-17, -3.469127814946512892E-15 ) ) ;
#51794=CARTESIAN_POINT ( 'NONE',  ( 37.00000000000000711, 6.303578524887092804, 10.42955799785312898 ) ) ;
#51795=LINE ( 'NONE', #20545, #22289 ) ;
#51797=EDGE_CURVE ( 'NONE', #14607, #45697, #5502, .T. ) ;
#51800=VERTEX_POINT ( 'NONE', #9133 ) ;
#51801=EDGE_CURVE ( 'NONE', #40209, #9770, #45826, .T. ) ;
#51802=CARTESIAN_POINT ( 'NONE',  ( -37.00000000000000711, 9.430788938294160317, -7.718225330433705622 ) ) ;
#51803=VERTEX_POINT ( 'NONE', #13779 ) ;
#51807=DIRECTION ( 'NONE',  ( 0.000000000000000000, -1.000000000000000000, 0.000000000000000000 ) ) ;
#51808=EDGE_CURVE ( 'NONE', #59054, #65435, #29416, .T. ) ;
#51809=ORIENTED_EDGE ( 'NONE', *, *, #44579, .F. ) ;
#51811=CARTESIAN_POINT ( 'NONE',  ( 36.00000000000000711, 10.68873102412842435, -6.950793414699834472 ) ) ;
#51814=CIRCLE ( 'NONE', #46483, 12.74999999999999822 ) ;
#51818=VERTEX_POINT ( 'NONE', #9444 ) ;
#51819=ORIENTED_EDGE ( 'NONE', *, *, #60065, .F. ) ;
#51820=CARTESIAN_POINT ( 'NONE',  ( -37.00000000000000711, -10.92721691015459307, 4.309077947445612899 ) ) ;
#51821=CARTESIAN_POINT ( 'NONE',  ( 29.51976981715666781, -4.571419055710073565, 11.09513982864076276 ) ) ;
#51823=AXIS2_PLACEMENT_3D ( 'NONE', #24064, #63296, #28074 ) ;
#51825=CARTESIAN_POINT ( 'NONE',  ( 35.00000000000000000, 4.705694406421931860E-17, -3.469127814946512892E-15 ) ) ;
#51826=ADVANCED_FACE ( 'NONE', ( #29108 ), #3852, .T. ) ;
#51827=ORIENTED_EDGE ( 'NONE', *, *, #18675, .F. ) ;
#51828=VECTOR ( 'NONE', #7771, 1000.000000000000000 ) ;
#51829=ORIENTED_EDGE ( 'NONE', *, *, #47239, .F. ) ;
#51830=CARTESIAN_POINT ( 'NONE',  ( -30.17816725640874154, -0.9612562749268102058, 11.96359558481438157 ) ) ;
#51831=ADVANCED_FACE ( 'NONE', ( #18141 ), #38413, .T. ) ;
#51834=DIRECTION ( 'NONE',  ( 0.000000000000000000, 0.3218879778915972878, -0.9467777615094571386 ) ) ;
#51835=DIRECTION ( 'NONE',  ( 0.000000000000000000, -0.01356324068818000328, 0.9999080150203990547 ) ) ;
#51837=DIRECTION ( 'NONE',  ( 0.000000000000000000, -0.01356324068817998940, 0.9999080150203990547 ) ) ;
#51838=ADVANCED_FACE ( 'NONE', ( #31060 ), #60328, .T. ) ;
#51841=ORIENTED_EDGE ( 'NONE', *, *, #63381, .T. ) ;
#51842=CARTESIAN_POINT ( 'NONE',  ( -9.340346724179731552, -10.24301314885845571, -6.263313883498242696 ) ) ;
#51844=CARTESIAN_POINT ( 'NONE',  ( -9.044048956294592045, 11.38398270688161595, -3.796001806769623066 ) ) ;
#51845=CARTESIAN_POINT ( 'NONE',  ( 36.00000000000000711, -3.307597835713331325, -12.31350058095522293 ) ) ;
#51846=ORIENTED_EDGE ( 'NONE', *, *, #21248, .F. ) ;
#51847=DIRECTION ( 'NONE',  ( -1.000000000000000000, 0.000000000000000000, 0.000000000000000000 ) ) ;
#51851=CARTESIAN_POINT ( 'NONE',  ( -36.00000000000000711, 1.457575200925721237, -12.66641127287624435 ) ) ;
#51855=CARTESIAN_POINT ( 'NONE',  ( 3.222831877979512871, 4.636616073543464722, 12.68534664307357396 ) ) ;
#51857=FACE_OUTER_BOUND ( 'NONE', #19600, .T. ) ;
#51858=ORIENTED_EDGE ( 'NONE', *, *, #36253, .T. ) ;
#51859=ORIENTED_EDGE ( 'NONE', *, *, #12887, .T. ) ;
#51861=DIRECTION ( 'NONE',  ( -1.000000000000000000, 0.000000000000000000, -0.000000000000000000 ) ) ;
#51862=DIRECTION ( 'NONE',  ( 0.000000000000000000, -1.000000000000000000, 0.000000000000000000 ) ) ;
#51863=AXIS2_PLACEMENT_3D ( 'NONE', #2659, #18902, #22920 ) ;
#51867=CYLINDRICAL_SURFACE ( 'NONE', #58212, 5.000000000000000000 ) ;
#51869=CARTESIAN_POINT ( 'NONE',  ( -47.00000000000000711, 0.000000000000000000, 0.000000000000000000 ) ) ;
#51872=CIRCLE ( 'NONE', #14709, 4.999999999999999112 ) ;
#51873=VERTEX_POINT ( 'NONE', #56683 ) ;
#51874=( BOUNDED_CURVE ( )  B_SPLINE_CURVE ( 3, ( #65789, #36196, #14925, #35218 ),
 .UNSPECIFIED., .F., .F. ) 
 B_SPLINE_CURVE_WITH_KNOTS ( ( 4, 4 ),
 ( 4.370225155591277222, 4.394090018125422326 ),
 .UNSPECIFIED. ) 
 CURVE ( )  GEOMETRIC_REPRESENTATION_ITEM ( )  RATIONAL_B_SPLINE_CURVE ( ( 1.000000000000000000, 0.9999525395911521564, 0.9999525395911521564, 1.000000000000000000 ) ) 
 REPRESENTATION_ITEM ( '' )  );
#51875=DIRECTION ( 'NONE',  ( 0.000000000000000000, -0.01356324068817991828, 0.9999080150203990547 ) ) ;
#51880=DIRECTION ( 'NONE',  ( -1.000000000000000000, 0.000000000000000000, 0.000000000000000000 ) ) ;
#51881=FACE_OUTER_BOUND ( 'NONE', #6408, .T. ) ;
#51882=EDGE_CURVE ( 'NONE', #44077, #58033, #29917, .T. ) ;
#51884=EDGE_LOOP ( 'NONE', ( #53362, #27461, #17424, #51272 ) ) ;
#51886=VERTEX_POINT ( 'NONE', #45692 ) ;
#51887=DIRECTION ( 'NONE',  ( 0.000000000000000000, 0.9105187689795940509, -0.4134677391718546424 ) ) ;
#51891=CARTESIAN_POINT ( 'NONE',  ( -35.00000000000000000, -12.14284015767849390, -1.030638227056693834 ) ) ;
#51892=ADVANCED_FACE ( 'NONE', ( #25096 ), #46040, .T. ) ;
#51893=EDGE_CURVE ( 'NONE', #27609, #54327, #11116, .T. ) ;
#51894=ORIENTED_EDGE ( 'NONE', *, *, #22925, .F. ) ;
#51896=DIRECTION ( 'NONE',  ( 0.000000000000000000, -0.7617968321374811724, -0.6478160128812026075 ) ) ;
#51898=CARTESIAN_POINT ( 'NONE',  ( 21.49227063098244628, 11.34819223667060406, -3.922596895461145650 ) ) ;
#51899=CARTESIAN_POINT ( 'NONE',  ( 21.97974065927837017, -13.30026544007890266, -2.341972921265582208 ) ) ;
#51900=ADVANCED_FACE ( 'NONE', ( #61313 ), #20099, .T. ) ;
#51904=CIRCLE ( 'NONE', #62453, 5.000000000000000888 ) ;
#51905=CARTESIAN_POINT ( 'NONE',  ( -37.00000000000000711, 11.23004253107764505, 4.732539170486304236 ) ) ;
#51906=DIRECTION ( 'NONE',  ( 0.000000000000000000, 0.01356324068817998940, -0.9999080150203990547 ) ) ;
#51907=DIRECTION ( 'NONE',  ( -1.000000000000000000, 0.000000000000000000, 0.000000000000000000 ) ) ;
#51908=ADVANCED_FACE ( 'NONE', ( #26085 ), #495, .T. ) ;
#51909=CIRCLE ( 'NONE', #60375, 12.74999999999999822 ) ;
#51910=VERTEX_POINT ( 'NONE', #41029 ) ;
#51911=ADVANCED_FACE ( 'NONE', ( #15102 ), #14756, .T. ) ;
#51912=VECTOR ( 'NONE', #16322, 1000.000000000000000 ) ;
#51916=DIRECTION ( 'NONE',  ( 0.000000000000000000, -0.04924826701375289995, -0.9987865678893274035 ) ) ;
#51917=AXIS2_PLACEMENT_3D ( 'NONE', #25606, #3, #35241 ) ;
#51919=ORIENTED_EDGE ( 'NONE', *, *, #1136, .T. ) ;
#51921=AXIS2_PLACEMENT_3D ( 'NONE', #50157, #56798, #4612 ) ;
#51922=ORIENTED_EDGE ( 'NONE', *, *, #7585, .T. ) ;
#51923=DIRECTION ( 'NONE',  ( 1.000000000000000000, 0.000000000000000000, 0.000000000000000000 ) ) ;
#51925=VERTEX_POINT ( 'NONE', #55348 ) ;
#51926=EDGE_CURVE ( 'NONE', #47572, #31395, #2319, .T. ) ;
#51927=CARTESIAN_POINT ( 'NONE',  ( -17.97366836756218689, 4.334172528176946315, -11.19214901861635170 ) ) ;
#51929=ORIENTED_EDGE ( 'NONE', *, *, #58622, .F. ) ;
#51932=CARTESIAN_POINT ( 'NONE',  ( 24.43856487734552019, -2.854323001380032032, 11.65700061237547658 ) ) ;
#51933=ORIENTED_EDGE ( 'NONE', *, *, #5187, .F. ) ;
#51934=CARTESIAN_POINT ( 'NONE',  ( -37.00000000000000711, 8.352657516904674395, 8.258652103341463047 ) ) ;
#51936=CARTESIAN_POINT ( 'NONE',  ( 35.00000000000000000, 4.705694406421931860E-17, -3.469127814946512892E-15 ) ) ;
#51940=CARTESIAN_POINT ( 'NONE',  ( 36.00000000000000711, 11.59605747147793942, 5.300372733891517640 ) ) ;
#51942=DIRECTION ( 'NONE',  ( 1.000000000000000000, 0.000000000000000000, 0.000000000000000000 ) ) ;
#51943=CARTESIAN_POINT ( 'NONE',  ( 9.953255994279757601, 1.096471986029277312, 11.95103177947028605 ) ) ;
#51944=CYLINDRICAL_SURFACE ( 'NONE', #34499, 13.50000000000000178 ) ;
#51946=EDGE_LOOP ( 'NONE', ( #1576, #51754, #42262, #63714 ) ) ;
#51947=DIRECTION ( 'NONE',  ( -1.000000000000000000, 0.000000000000000000, 0.000000000000000000 ) ) ;
#51948=EDGE_CURVE ( 'NONE', #32729, #19643, #803, .T. ) ;
#51950=CIRCLE ( 'NONE', #24302, 5.000000000000000888 ) ;
#51952=EDGE_LOOP ( 'NONE', ( #51441, #26867, #7245, #3460 ) ) ;
#51953=CARTESIAN_POINT ( 'NONE',  ( -17.49435431676402786, 7.621753754644457146, 9.270964220055409655 ) ) ;
#51954=DIRECTION ( 'NONE',  ( -1.000000000000000000, -0.000000000000000000, -0.000000000000000000 ) ) ;
#51955=DIRECTION ( 'NONE',  ( 0.000000000000000000, -0.01356324068817998940, 0.9999080150203990547 ) ) ;
#51957=AXIS2_PLACEMENT_3D ( 'NONE', #19839, #38816, #19178 ) ;
#51962=AXIS2_PLACEMENT_3D ( 'NONE', #6268, #61133, #56128 ) ;
#51963=ORIENTED_EDGE ( 'NONE', *, *, #8732, .F. ) ;
#51965=LINE ( 'NONE', #52933, #63191 ) ;
#51966=DIRECTION ( 'NONE',  ( -1.000000000000000000, 0.000000000000000000, 0.000000000000000000 ) ) ;
#51967=EDGE_CURVE ( 'NONE', #23545, #16620, #7096, .T. ) ;
#51968=ORIENTED_EDGE ( 'NONE', *, *, #48956, .F. ) ;
#51969=VECTOR ( 'NONE', #24072, 1000.000000000000000 ) ;
#51971=EDGE_CURVE ( 'NONE', #26131, #22816, #52348, .T. ) ;
#51972=LINE ( 'NONE', #62255, #7438 ) ;
#51973=LINE ( 'NONE', #61179, #16127 ) ;
#51974=CARTESIAN_POINT ( 'NONE',  ( 37.00000000000000711, 11.74614673114903773, 0.01609748574448878478 ) ) ;
#51975=CARTESIAN_POINT ( 'NONE',  ( 35.00000000000000000, 0.7536123767498499326, -11.72195762423410414 ) ) ;
#51976=DIRECTION ( 'NONE',  ( -0.8867529933577791290, 0.000000000000000000, -0.4622435816439406930 ) ) ;
#51980=AXIS2_PLACEMENT_3D ( 'NONE', #54432, #18541, #9173 ) ;
#51981=ORIENTED_EDGE ( 'NONE', *, *, #48789, .T. ) ;
#51983=DIRECTION ( 'NONE',  ( -0.7290028908350527637, 0.000000000000000000, 0.6845106172691086677 ) ) ;
#51984=ORIENTED_EDGE ( 'NONE', *, *, #11308, .F. ) ;
#51985=CYLINDRICAL_SURFACE ( 'NONE', #2585, 4.094603870727468120 ) ;
#51986=CARTESIAN_POINT ( 'NONE',  ( 0.6844764289427172077, 0.5169738502507784661, -11.99252702960889927 ) ) ;
#51988=DIRECTION ( 'NONE',  ( 1.000000000000000000, 0.000000000000000000, -0.000000000000000000 ) ) ;
#51989=ORIENTED_EDGE ( 'NONE', *, *, #7728, .F. ) ;
#51991=EDGE_LOOP ( 'NONE', ( #37643, #6786, #31144, #30335 ) ) ;
#51992=ORIENTED_EDGE ( 'NONE', *, *, #34746, .F. ) ;
#51993=CIRCLE ( 'NONE', #16961, 5.000000000000001776 ) ;
#51994=EDGE_CURVE ( 'NONE', #42367, #43621, #49164, .T. ) ;
#51996=VERTEX_POINT ( 'NONE', #17069 ) ;
#51997=CARTESIAN_POINT ( 'NONE',  ( -25.16596872619400216, -6.639998712458014651, 10.00200833204654494 ) ) ;
#52000=DIRECTION ( 'NONE',  ( 0.000000000000000000, 0.000000000000000000, -1.000000000000000000 ) ) ;
#52001=ORIENTED_EDGE ( 'NONE', *, *, #45424, .T. ) ;
#52005=DIRECTION ( 'NONE',  ( 0.000000000000000000, 0.01356324068817998940, -0.9999080150203989437 ) ) ;
#52006=ORIENTED_EDGE ( 'NONE', *, *, #57277, .F. ) ;
#52007=CARTESIAN_POINT ( 'NONE',  ( -35.00000000000000000, -11.16627499335652374, -3.645068577060142978 ) ) ;
#52008=ORIENTED_EDGE ( 'NONE', *, *, #45656, .F. ) ;
#52009=LINE ( 'NONE', #41352, #1977 ) ;
#52010=AXIS2_PLACEMENT_3D ( 'NONE', #65160, #45527, #30886 ) ;
#52011=VERTEX_POINT ( 'NONE', #6451 ) ;
#52013=DIRECTION ( 'NONE',  ( -0.000000000000000000, -0.000000000000000000, -1.000000000000000000 ) ) ;
#52014=DIRECTION ( 'NONE',  ( 1.000000000000000000, 0.000000000000000000, 0.000000000000000000 ) ) ;
#52015=ORIENTED_EDGE ( 'NONE', *, *, #36622, .T. ) ;
#52019=B_SPLINE_CURVE_WITH_KNOTS ( 'NONE', 3,
 ( #50950, #20028, #60261, #65558, #40293, #15364, #5399, #29999, #20351, #40633, #56248, #64909, #34965, #24354, #35637, #19390, #55271, #34649, #39655, #59957, #54945, #9374, #29659, #52604, #26010, #46605 ),
 .UNSPECIFIED., .F., .F.,
 ( 4, 2, 2, 2, 2, 2, 2, 2, 2, 2, 2, 2, 4 ),
 ( 7.152448122690996019E-18, 0.001355494837136931013, 0.002033242255705391098, 0.002710989674273851183, 0.004066484511410767451, 0.004744231929979227103, 0.005421979348547687622, 0.006099726767116149875, 0.006777474185684612996, 0.007455221604253076118, 0.008132969022821540106, 0.009488463859958469818, 0.01084395869709539779 ),
 .UNSPECIFIED. ) ;
#52020=VERTEX_POINT ( 'NONE', #22736 ) ;
#52021=EDGE_CURVE ( 'NONE', #29441, #65378, #12397, .T. ) ;
#52024=VERTEX_POINT ( 'NONE', #22060 ) ;
#52026=ORIENTED_EDGE ( 'NONE', *, *, #52569, .F. ) ;
#52027=DIRECTION ( 'NONE',  ( 1.000000000000000000, 0.000000000000000000, -0.000000000000000000 ) ) ;
#52028=CARTESIAN_POINT ( 'NONE',  ( 35.00000000000000000, 2.185196060784047045, 11.54110654723646157 ) ) ;
#52031=CARTESIAN_POINT ( 'NONE',  ( -37.00000000000000711, -5.927257550915394191, 10.64792938439753378 ) ) ;
#52032=FACE_OUTER_BOUND ( 'NONE', #25022, .T. ) ;
#52034=VECTOR ( 'NONE', #2980, 1000.000000000000000 ) ;
#52035=ADVANCED_FACE ( 'NONE', ( #52978 ), #17744, .T. ) ;
#52037=ORIENTED_EDGE ( 'NONE', *, *, #53318, .F. ) ;
#52040=CARTESIAN_POINT ( 'NONE',  ( -4.023342348990911255, -9.886260852804344523, 6.816691047944269499 ) ) ;
#52043=CARTESIAN_POINT ( 'NONE',  ( -35.00000000000000000, 0.000000000000000000, 0.000000000000000000 ) ) ;
#52044=EDGE_CURVE ( 'NONE', #30121, #48464, #12726, .T. ) ;
#52045=( BOUNDED_CURVE ( )  B_SPLINE_CURVE ( 3, ( #43723, #64004, #18487, #38743 ),
 .UNSPECIFIED., .F., .F. ) 
 B_SPLINE_CURVE_WITH_KNOTS ( ( 4, 4 ),
 ( 1.841109206681600385, 1.865537793031380120 ),
 .UNSPECIFIED. ) 
 CURVE ( )  GEOMETRIC_REPRESENTATION_ITEM ( )  RATIONAL_B_SPLINE_CURVE ( ( 1.000000000000000000, 0.9999502709656691302, 0.9999502709656691302, 1.000000000000000000 ) ) 
 REPRESENTATION_ITEM ( '' )  );
#52048=ORIENTED_EDGE ( 'NONE', *, *, #65519, .T. ) ;
#52051=CARTESIAN_POINT ( 'NONE',  ( -25.54417658651491863, 4.240019242199842608, 11.22596262356930197 ) ) ;
#52056=VERTEX_POINT ( 'NONE', #62289 ) ;
#52057=DIRECTION ( 'NONE',  ( -1.000000000000000000, -0.000000000000000000, 0.000000000000000000 ) ) ;
#52058=CARTESIAN_POINT ( 'NONE',  ( 2.354167843600960097, -6.278647867796540716, 25.00000000000000000 ) ) ;
#52059=CARTESIAN_POINT ( 'NONE',  ( -27.19357181888462094, -12.48377454417556542, 5.138615876886901468 ) ) ;
#52060=ORIENTED_EDGE ( 'NONE', *, *, #63777, .T. ) ;
#52062=DIRECTION ( 'NONE',  ( 1.000000000000000000, 0.000000000000000000, 0.000000000000000000 ) ) ;
#52064=CARTESIAN_POINT ( 'NONE',  ( 35.00000000000000000, -6.280308599560208371, -9.926225166347007800 ) ) ;
#52065=ORIENTED_EDGE ( 'NONE', *, *, #1952, .F. ) ;
#52067=ADVANCED_FACE ( 'NONE', ( #16744 ), #11426, .T. ) ;
#52068=AXIS2_PLACEMENT_3D ( 'NONE', #31830, #52145, #1613 ) ;
#52069=CIRCLE ( 'NONE', #12793, 12.18649999999999878 ) ;
#52072=DIRECTION ( 'NONE',  ( -1.000000000000000000, 0.000000000000000000, 0.000000000000000000 ) ) ;
#52076=CARTESIAN_POINT ( 'NONE',  ( 10.48620311856346454, 8.250315036047107142, 25.00000000000000000 ) ) ;
#52077=CARTESIAN_POINT ( 'NONE',  ( 35.00000000000000000, 11.17622378668006355, -3.614449339633533764 ) ) ;
#52079=ORIENTED_EDGE ( 'NONE', *, *, #40871, .F. ) ;
#52081=VERTEX_POINT ( 'NONE', #32359 ) ;
#52083=ORIENTED_EDGE ( 'NONE', *, *, #48152, .T. ) ;
#52084=LINE ( 'NONE', #32436, #18838 ) ;
#52085=VECTOR ( 'NONE', #63271, 1000.000000000000000 ) ;
#52086=ADVANCED_FACE ( 'NONE', ( #62953 ), #37017, .T. ) ;
#52089=EDGE_LOOP ( 'NONE', ( #32986, #48905, #52340, #58630 ) ) ;
#52090=CARTESIAN_POINT ( 'NONE',  ( -35.00000000000000000, 12.12087942037211263, -1.262958560998631796 ) ) ;
#52091=DIRECTION ( 'NONE',  ( -1.000000000000000000, 0.000000000000000000, 0.000000000000000000 ) ) ;
#52094=VERTEX_POINT ( 'NONE', #39650 ) ;
#52095=ORIENTED_EDGE ( 'NONE', *, *, #29704, .T. ) ;
#52099=CIRCLE ( 'NONE', #23424, 12.74999999999999822 ) ;
#52100=DIRECTION ( 'NONE',  ( 1.000000000000000000, -0.000000000000000000, 0.000000000000000000 ) ) ;
#52102=CARTESIAN_POINT ( 'NONE',  ( 35.00000000000000000, -10.64792938439759595, -5.927257550915285833 ) ) ;
#52106=ADVANCED_FACE ( 'NONE', ( #54646 ), #63594, .F. ) ;
#52107=CARTESIAN_POINT ( 'NONE',  ( 36.00000000000000711, -12.57916205664482767, -2.080187960898522537 ) ) ;
#52109=ORIENTED_EDGE ( 'NONE', *, *, #1173, .T. ) ;
#52112=ORIENTED_EDGE ( 'NONE', *, *, #48685, .F. ) ;
#52113=CIRCLE ( 'NONE', #54260, 12.74999999999999822 ) ;
#52114=FACE_OUTER_BOUND ( 'NONE', #56261, .T. ) ;
#52118=DIRECTION ( 'NONE',  ( -1.000000000000000000, 0.000000000000000000, 0.000000000000000000 ) ) ;
#52121=VERTEX_POINT ( 'NONE', #58983 ) ;
#52122=CIRCLE ( 'NONE', #33020, 4.999999999999999112 ) ;
#52123=CIRCLE ( 'NONE', #60611, 5.000000000000001776 ) ;
#52124=ORIENTED_EDGE ( 'NONE', *, *, #3565, .F. ) ;
#52125=VECTOR ( 'NONE', #62354, 1000.000000000000000 ) ;
#52126=DIRECTION ( 'NONE',  ( 1.000000000000000000, -0.000000000000000000, 0.000000000000000000 ) ) ;
#52128=ORIENTED_EDGE ( 'NONE', *, *, #2604, .F. ) ;
#52129=AXIS2_PLACEMENT_3D ( 'NONE', #22835, #62080, #37113 ) ;
#52131=DIRECTION ( 'NONE',  ( 0.000000000000000000, -0.01356324068817992175, 0.9999080150203990547 ) ) ;
#52133=LINE ( 'NONE', #1603, #62804 ) ;
#52134=LINE ( 'NONE', #31818, #31778 ) ;
#52137=CARTESIAN_POINT ( 'NONE',  ( 35.00000000000000000, 4.339012074899953220, -10.91536515067649660 ) ) ;
#52139=DIRECTION ( 'NONE',  ( -1.000000000000000000, -1.836970198721029688E-16, 0.000000000000000000 ) ) ;
#52140=VECTOR ( 'NONE', #27536, 1000.000000000000000 ) ;
#52141=AXIS2_PLACEMENT_3D ( 'NONE', #33626, #27002, #47298 ) ;
#52142=AXIS2_PLACEMENT_3D ( 'NONE', #23679, #18698, #38956 ) ;
#52144=AXIS2_PLACEMENT_3D ( 'NONE', #37156, #31838, #6601 ) ;
#52145=DIRECTION ( 'NONE',  ( 1.000000000000000000, 0.000000000000000000, 0.000000000000000000 ) ) ;
#52147=VECTOR ( 'NONE', #12471, 1000.000000000000000 ) ;
#52149=ORIENTED_EDGE ( 'NONE', *, *, #1173, .F. ) ;
#52154=CYLINDRICAL_SURFACE ( 'NONE', #43701, 12.18649999999999878 ) ;
#52156=ORIENTED_EDGE ( 'NONE', *, *, #22188, .T. ) ;
#52157=VERTEX_POINT ( 'NONE', #13077 ) ;
#52159=ORIENTED_EDGE ( 'NONE', *, *, #50092, .T. ) ;
#52160=CARTESIAN_POINT ( 'NONE',  ( 3.403981455603509065, 7.616542962421854135, 9.282725052014482614 ) ) ;
#52162=DIRECTION ( 'NONE',  ( -1.000000000000000000, 0.000000000000000000, 0.000000000000000000 ) ) ;
#52163=CARTESIAN_POINT ( 'NONE',  ( -37.00000000000000711, 0.000000000000000000, 0.000000000000000000 ) ) ;
#52168=VERTEX_POINT ( 'NONE', #34333 ) ;
#52169=AXIS2_PLACEMENT_3D ( 'NONE', #132, #40028, #5127 ) ;
#52170=EDGE_CURVE ( 'NONE', #12280, #3409, #3369, .T. ) ;
#52174=CARTESIAN_POINT ( 'NONE',  ( -37.00000000000000711, 8.624332853796195408, -9.390600770287900190 ) ) ;
#52175=CARTESIAN_POINT ( 'NONE',  ( 21.59694336868049902, -12.74990532528425291, -4.441854890391109478 ) ) ;
#52177=CARTESIAN_POINT ( 'NONE',  ( 37.00000000000000711, 4.705694406421931860E-17, -3.469127814946512892E-15 ) ) ;
#52178=VECTOR ( 'NONE', #61279, 1000.000000000000000 ) ;
#52180=ADVANCED_FACE ( 'NONE', ( #44302 ), #39311, .T. ) ;
#52181=CARTESIAN_POINT ( 'NONE',  ( 35.00000000000000000, -9.677500615117850202, 6.657191900728419043 ) ) ;
#52182=ORIENTED_EDGE ( 'NONE', *, *, #29161, .T. ) ;
#52183=DIRECTION ( 'NONE',  ( 1.000000000000000000, -0.000000000000000000, -0.000000000000000000 ) ) ;
#52185=DIRECTION ( 'NONE',  ( -1.000000000000000000, -0.000000000000000000, 0.000000000000000000 ) ) ;
#52188=CARTESIAN_POINT ( 'NONE',  ( 3.435435718939642946, 5.961994453915724357, 12.11397542276001538 ) ) ;
#52189=EDGE_CURVE ( 'NONE', #49613, #30052, #61552, .T. ) ;
#52190=EDGE_LOOP ( 'NONE', ( #27286, #16367 ) ) ;
#52191=VERTEX_POINT ( 'NONE', #24690 ) ;
#52192=EDGE_LOOP ( 'NONE', ( #51000, #6450, #37792, #45764 ) ) ;
#52194=CIRCLE ( 'NONE', #6574, 12.18650000000000055 ) ;
#52196=CYLINDRICAL_SURFACE ( 'NONE', #49645, 13.50000000000000178 ) ;
#52197=VECTOR ( 'NONE', #57884, 1000.000000000000000 ) ;
#52199=DIRECTION ( 'NONE',  ( 1.000000000000000000, -0.000000000000000000, -0.000000000000000000 ) ) ;
#52200=DIRECTION ( 'NONE',  ( 0.000000000000000000, 0.01356324068817992175, -0.9999080150203990547 ) ) ;
#52201=ORIENTED_EDGE ( 'NONE', *, *, #20140, .T. ) ;
#52203=VERTEX_POINT ( 'NONE', #40628 ) ;
#52204=CYLINDRICAL_SURFACE ( 'NONE', #5063, 4.999999999999999112 ) ;
#52205=ADVANCED_FACE ( 'NONE', ( #15665 ), #25666, .T. ) ;
#52207=AXIS2_PLACEMENT_3D ( 'NONE', #37691, #2460, #57320 ) ;
#52209=EDGE_CURVE ( 'NONE', #49715, #2584, #53008, .T. ) ;
#52210=CYLINDRICAL_SURFACE ( 'NONE', #20128, 4.999999999999999112 ) ;
#52213=DIRECTION ( 'NONE',  ( 0.000000000000000000, -1.000000000000000000, 0.000000000000000000 ) ) ;
#52216=DIRECTION ( 'NONE',  ( 0.000000000000000000, 0.7617968321374855023, 0.6478160128811973895 ) ) ;
#52218=AXIS2_PLACEMENT_3D ( 'NONE', #36119, #61733, #55782 ) ;
#52223=EDGE_CURVE ( 'NONE', #27379, #23284, #730, .T. ) ;
#52224=CIRCLE ( 'NONE', #42486, 4.999999999999999112 ) ;
#52225=CARTESIAN_POINT ( 'NONE',  ( 35.00000000000000000, -5.644643009979139592, -10.30098186818248074 ) ) ;
#52228=VERTEX_POINT ( 'NONE', #14677 ) ;
#52229=CARTESIAN_POINT ( 'NONE',  ( -35.00000000000000000, 1.903127969211188653, 11.59095880812009227 ) ) ;
#52231=CARTESIAN_POINT ( 'NONE',  ( 21.44135743879865430, 11.69231880031143866, -2.731539164460570657 ) ) ;
#52232=DIRECTION ( 'NONE',  ( 1.000000000000000000, 0.000000000000000000, 0.000000000000000000 ) ) ;
#52233=CIRCLE ( 'NONE', #30938, 5.000000000000000000 ) ;
#52234=CIRCLE ( 'NONE', #23550, 12.74999999999999822 ) ;
#52238=LINE ( 'NONE', #57552, #43674 ) ;
#52239=CIRCLE ( 'NONE', #9774, 5.000000000000001776 ) ;
#52240=EDGE_CURVE ( 'NONE', #50233, #57324, #45960, .T. ) ;
#52241=ORIENTED_EDGE ( 'NONE', *, *, #30449, .F. ) ;
#52242=AXIS2_PLACEMENT_3D ( 'NONE', #17540, #33785, #7541 ) ;
#52248=DIRECTION ( 'NONE',  ( 0.000000000000000000, 0.01356324068817991828, -0.9999080150203990547 ) ) ;
#52249=AXIS2_PLACEMENT_3D ( 'NONE', #64501, #53239, #23303 ) ;
#52252=CIRCLE ( 'NONE', #23582, 5.000000000000000888 ) ;
#52255=ORIENTED_EDGE ( 'NONE', *, *, #58570, .F. ) ;
#52256=CARTESIAN_POINT ( 'NONE',  ( -35.00000000000000000, 6.946017217729938409, 10.01317267707888981 ) ) ;
#52257=CARTESIAN_POINT ( 'NONE',  ( 37.00000000000000711, -11.86701198550353986, 2.772148766916240348 ) ) ;
#52258=EDGE_LOOP ( 'NONE', ( #45046, #45210, #22642, #54888 ) ) ;
#52259=CARTESIAN_POINT ( 'NONE',  ( -17.60261755426340713, 3.558939319148466396, -11.46150330649539306 ) ) ;
#52260=AXIS2_PLACEMENT_3D ( 'NONE', #47691, #12104, #41371 ) ;
#52261=CARTESIAN_POINT ( 'NONE',  ( 145.1370849898475797, 3.309064568108273190E-14, 0.000000000000000000 ) ) ;
#52262=ORIENTED_EDGE ( 'NONE', *, *, #31647, .F. ) ;
#52265=DIRECTION ( 'NONE',  ( -1.000000000000000000, 0.000000000000000000, 0.000000000000000000 ) ) ;
#52267=EDGE_LOOP ( 'NONE', ( #57165, #28892, #62485, #35739 ) ) ;
#52268=DIRECTION ( 'NONE',  ( 1.000000000000000000, 0.000000000000000000, 0.000000000000000000 ) ) ;
#52269=EDGE_CURVE ( 'NONE', #48664, #37930, #20021, .T. ) ;
#52271=CARTESIAN_POINT ( 'NONE',  ( 35.00000000000000000, -12.16893194857552452, -3.805206332242430101 ) ) ;
#52272=VECTOR ( 'NONE', #18875, 1000.000000000000000 ) ;
#52273=CARTESIAN_POINT ( 'NONE',  ( -17.67260731600310208, -7.949547442848166945, 10.91509878626014540 ) ) ;
#52274=EDGE_CURVE ( 'NONE', #29168, #13166, #5738, .T. ) ;
#52276=CYLINDRICAL_SURFACE ( 'NONE', #31539, 4.999999999999999112 ) ;
#52277=CIRCLE ( 'NONE', #4470, 12.18650000000000055 ) ;
#52279=CYLINDRICAL_SURFACE ( 'NONE', #30370, 4.999999999999999112 ) ;
#52280=AXIS2_PLACEMENT_3D ( 'NONE', #20207, #15218, #54821 ) ;
#52281=DIRECTION ( 'NONE',  ( 1.000000000000000000, 0.000000000000000000, 0.000000000000000000 ) ) ;
#52283=CARTESIAN_POINT ( 'NONE',  ( 9.188001832116450274, 6.971707373100242577, -9.768769640225654527 ) ) ;
#52285=CARTESIAN_POINT ( 'NONE',  ( -35.00000000000000000, -2.772148766916031182, -11.86701198550359315 ) ) ;
#52286=ORIENTED_EDGE ( 'NONE', *, *, #152, .T. ) ;
#52290=DIRECTION ( 'NONE',  ( 0.000000000000000000, 0.3218879778915972878, -0.9467777615094571386 ) ) ;
#52294=ORIENTED_EDGE ( 'NONE', *, *, #60960, .T. ) ;
#52295=AXIS2_PLACEMENT_3D ( 'NONE', #34129, #64390, #25149 ) ;
#52297=LINE ( 'NONE', #6737, #3548 ) ;
#52298=EDGE_CURVE ( 'NONE', #10001, #10138, #55457, .T. ) ;
#52302=DIRECTION ( 'NONE',  ( -1.000000000000000000, 0.000000000000000000, 0.000000000000000000 ) ) ;
#52303=ADVANCED_FACE ( 'NONE', ( #60253 ), #45609, .T. ) ;
#52304=CARTESIAN_POINT ( 'NONE',  ( -35.00000000000000000, -5.921969905510425569, 10.14408668126211488 ) ) ;
#52305=ORIENTED_EDGE ( 'NONE', *, *, #23954, .F. ) ;
#52311=FACE_OUTER_BOUND ( 'NONE', #3732, .T. ) ;
#52312=DIRECTION ( 'NONE',  ( -1.000000000000000000, -0.000000000000000000, 0.000000000000000000 ) ) ;
#52314=CARTESIAN_POINT ( 'NONE',  ( 35.00000000000000000, -7.251710744571640888, -9.240395740215610942 ) ) ;
#52316=LINE ( 'NONE', #41654, #56637 ) ;
#52317=VECTOR ( 'NONE', #5381, 1000.000000000000000 ) ;
#52318=AXIS2_PLACEMENT_3D ( 'NONE', #2997, #38553, #8951 ) ;
#52321=CARTESIAN_POINT ( 'NONE',  ( -18.08686583997218733, 5.370770984569721129, 12.38794726521413736 ) ) ;
#52323=ADVANCED_FACE ( 'NONE', ( #10358 ), #61239, .T. ) ;
#52324=VERTEX_POINT ( 'NONE', #11034 ) ;
#52325=LINE ( 'NONE', #6764, #9849 ) ;
#52327=ORIENTED_EDGE ( 'NONE', *, *, #26203, .F. ) ;
#52330=CARTESIAN_POINT ( 'NONE',  ( -35.00000000000000000, 5.391785509270962784, 10.43555801961477236 ) ) ;
#52332=ORIENTED_EDGE ( 'NONE', *, *, #46864, .F. ) ;
#52336=CYLINDRICAL_SURFACE ( 'NONE', #52509, 5.000000000000000888 ) ;
#52338=CARTESIAN_POINT ( 'NONE',  ( 22.88594695219327235, -4.822122601967141264, -12.60940655271284427 ) ) ;
#52339=DIRECTION ( 'NONE',  ( 1.000000000000000000, 0.000000000000000000, 0.000000000000000000 ) ) ;
#52340=ORIENTED_EDGE ( 'NONE', *, *, #28314, .F. ) ;
#52341=VECTOR ( 'NONE', #58216, 1000.000000000000000 ) ;
#52342=CARTESIAN_POINT ( 'NONE',  ( 29.03457606387295087, 7.862146963512124387, 10.97436308512422265 ) ) ;
#52346=CARTESIAN_POINT ( 'NONE',  ( -24.39341069969850295, 9.142292985779414849, 7.776119890389081135 ) ) ;
#52347=VERTEX_POINT ( 'NONE', #52900 ) ;
#52348=LINE ( 'NONE', #33010, #58615 ) ;
#52349=EDGE_CURVE ( 'NONE', #12370, #45713, #42666, .T. ) ;
#52350=ORIENTED_EDGE ( 'NONE', *, *, #54866, .F. ) ;
#52352=ORIENTED_EDGE ( 'NONE', *, *, #462, .F. ) ;
#52353=CARTESIAN_POINT ( 'NONE',  ( 21.65883687731333751, -11.04763598250161749, -4.689338699165349844 ) ) ;
#52354=DIRECTION ( 'NONE',  ( 0.000000000000000000, -0.04924826701373159060, -0.9987865678893284027 ) ) ;
#52358=DIRECTION ( 'NONE',  ( 0.000000000000000000, -0.01356324068817998940, 0.9999080150203990547 ) ) ;
#52359=CARTESIAN_POINT ( 'NONE',  ( -37.00000000000000711, 0.000000000000000000, 0.000000000000000000 ) ) ;
#52361=ORIENTED_EDGE ( 'NONE', *, *, #36230, .T. ) ;
#52362=VERTEX_POINT ( 'NONE', #46937 ) ;
#52363=CARTESIAN_POINT ( 'NONE',  ( -35.00000000000000000, 2.185196060783882288, 11.54110654723649709 ) ) ;
#52364=EDGE_LOOP ( 'NONE', ( #46268, #5316, #22297, #4111 ) ) ;
#52365=ORIENTED_EDGE ( 'NONE', *, *, #52021, .F. ) ;
#52366=DIRECTION ( 'NONE',  ( 0.000000000000000000, 0.3218879778915905154, -0.9467777615094595811 ) ) ;
#52367=VECTOR ( 'NONE', #36865, 1000.000000000000000 ) ;
#52368=CARTESIAN_POINT ( 'NONE',  ( 35.00000000000000000, 4.705694406421931860E-17, -3.469127814946512892E-15 ) ) ;
#52369=CARTESIAN_POINT ( 'NONE',  ( 35.00000000000000000, -11.66953048682396954, 3.511814412392239682 ) ) ;
#52371=CYLINDRICAL_SURFACE ( 'NONE', #44388, 12.18649999999999878 ) ;
#52372=EDGE_CURVE ( 'NONE', #4532, #33015, #2363, .T. ) ;
#52373=AXIS2_PLACEMENT_3D ( 'NONE', #27837, #58780, #43114 ) ;
#52376=DIRECTION ( 'NONE',  ( 1.000000000000000000, -0.000000000000000000, 0.000000000000000000 ) ) ;
#52377=EDGE_LOOP ( 'NONE', ( #19996, #33667, #16559, #1744 ) ) ;
#52380=CARTESIAN_POINT ( 'NONE',  ( 35.00000000000000000, 11.73808581813437080, -0.4353888892050498116 ) ) ;
#52381=EDGE_CURVE ( 'NONE', #63113, #64447, #22299, .T. ) ;
#52382=CIRCLE ( 'NONE', #21571, 12.74999999999999822 ) ;
#52383=CYLINDRICAL_SURFACE ( 'NONE', #56595, 12.75000000000000178 ) ;
#52386=CARTESIAN_POINT ( 'NONE',  ( 8.810907765906716094, 2.660651897896487483, -11.70423931794396211 ) ) ;
#52389=CARTESIAN_POINT ( 'NONE',  ( -37.00000000000000711, 0.9416912585474421782, 12.71517666308948513 ) ) ;
#52391=CARTESIAN_POINT ( 'NONE',  ( -17.54726996257253191, -12.93490414535027710, 3.865003848717349033 ) ) ;
#52392=CARTESIAN_POINT ( 'NONE',  ( -24.84400141115547456, 8.878028940934107993, 8.075574810441137785 ) ) ;
#52393=CARTESIAN_POINT ( 'NONE',  ( -24.79772874291392526, -10.35329051066264761, 8.670239208206227843 ) ) ;
#52395=ORIENTED_EDGE ( 'NONE', *, *, #45056, .T. ) ;
#52396=DIRECTION ( 'NONE',  ( 0.000000000000000000, -0.9999080150203989437, -0.01356324068819032662 ) ) ;
#52397=CARTESIAN_POINT ( 'NONE',  ( -2.532614230583023041, 12.88560382747354005, 4.026315189028235153 ) ) ;
#52398=CARTESIAN_POINT ( 'NONE',  ( -8.891032880924177206, 25.00000000000000000, -3.860857758255646921 ) ) ;
#52401=ADVANCED_FACE ( 'NONE', ( #11351 ), #41933, .T. ) ;
#52403=CARTESIAN_POINT ( 'NONE',  ( -35.00000000000000000, -12.05416472667164207, -1.791059740004549372 ) ) ;
#52407=VERTEX_POINT ( 'NONE', #62871 ) ;
#52409=AXIS2_PLACEMENT_3D ( 'NONE', #63636, #65598, #9756 ) ;
#52411=EDGE_CURVE ( 'NONE', #4408, #47167, #7665, .T. ) ;
#52412=DIRECTION ( 'NONE',  ( 1.000000000000000000, 0.000000000000000000, 0.000000000000000000 ) ) ;
#52413=ORIENTED_EDGE ( 'NONE', *, *, #54572, .F. ) ;
#52416=DIRECTION ( 'NONE',  ( 1.000000000000000000, 0.000000000000000000, 0.000000000000000000 ) ) ;
#52417=CARTESIAN_POINT ( 'NONE',  ( -3.460650213238962269, -8.804360588126725062, 10.24121041136440802 ) ) ;
#52419=CIRCLE ( 'NONE', #51390, 5.000000000000000888 ) ;
#52424=EDGE_CURVE ( 'NONE', #34070, #34540, #42923, .T. ) ;
#52425=EDGE_CURVE ( 'NONE', #54245, #26733, #31012, .T. ) ;
#52427=DIRECTION ( 'NONE',  ( 0.000000000000000000, 0.01356324068817998940, -0.9999080150203990547 ) ) ;
#52428=CIRCLE ( 'NONE', #50288, 12.18650000000000055 ) ;
#52429=ORIENTED_EDGE ( 'NONE', *, *, #17635, .F. ) ;
#52432=CIRCLE ( 'NONE', #45010, 12.18649999999999878 ) ;
#52433=CARTESIAN_POINT ( 'NONE',  ( -2.952869152607106251, 11.39722960915212724, 3.755417052241485365 ) ) ;
#52434=DIRECTION ( 'NONE',  ( 0.000000000000000000, 0.7617968321374899432, 0.6478160128811920604 ) ) ;
#52436=AXIS2_PLACEMENT_3D ( 'NONE', #48342, #33352, #7759 ) ;
#52437=FACE_OUTER_BOUND ( 'NONE', #64923, .T. ) ;
#52438=CARTESIAN_POINT ( 'NONE',  ( -35.00000000000000000, 8.534258022646220354, -8.699265615722891809 ) ) ;
#52439=ORIENTED_EDGE ( 'NONE', *, *, #53787, .T. ) ;
#52441=ORIENTED_EDGE ( 'NONE', *, *, #11242, .F. ) ;
#52442=CARTESIAN_POINT ( 'NONE',  ( 29.20601902130347227, -10.31618498597828371, 8.717929643690714769 ) ) ;
#52443=ORIENTED_EDGE ( 'NONE', *, *, #63516, .F. ) ;
#52444=DIRECTION ( 'NONE',  ( 1.000000000000000000, 0.000000000000000000, 0.000000000000000000 ) ) ;
#52445=LINE ( 'NONE', #16531, #33026 ) ;
#52446=CARTESIAN_POINT ( 'NONE',  ( 9.042193032038563061, 3.535237157306648115, 13.03118443932375925 ) ) ;
#52452=VERTEX_POINT ( 'NONE', #6709 ) ;
#52455=VERTEX_POINT ( 'NONE', #26986 ) ;
#52458=AXIS2_PLACEMENT_3D ( 'NONE', #43807, #64086, #29475 ) ;
#52459=CARTESIAN_POINT ( 'NONE',  ( -9.036293593347389574, 11.24548700741398477, -4.203574557735506367 ) ) ;
#52460=DIRECTION ( 'NONE',  ( -1.000000000000000000, 0.000000000000000000, 0.000000000000000000 ) ) ;
#52462=CARTESIAN_POINT ( 'NONE',  ( -35.00000000000000000, 0.000000000000000000, 0.000000000000000000 ) ) ;
#52463=EDGE_LOOP ( 'NONE', ( #62954, #59833, #29684, #32638 ) ) ;
#52464=VECTOR ( 'NONE', #31751, 1000.000000000000000 ) ;
#52468=ORIENTED_EDGE ( 'NONE', *, *, #16873, .T. ) ;
#52469=DIRECTION ( 'NONE',  ( 1.000000000000000000, 0.000000000000000000, 0.000000000000000000 ) ) ;
#52470=DIRECTION ( 'NONE',  ( 0.000000000000000000, 0.3554799084908968343, 0.9346839223284540976 ) ) ;
#52471=AXIS2_PLACEMENT_3D ( 'NONE', #34447, #4194, #64682 ) ;
#52472=DIRECTION ( 'NONE',  ( 0.000000000000000000, 0.9551603052523468529, -0.2960891610144545938 ) ) ;
#52474=EDGE_LOOP ( 'NONE', ( #24616, #41422, #37001, #33530 ) ) ;
#52476=DIRECTION ( 'NONE',  ( -1.000000000000000000, -0.000000000000000000, 0.000000000000000000 ) ) ;
#52479=AXIS2_PLACEMENT_3D ( 'NONE', #11912, #52514, #6946 ) ;
#52480=EDGE_CURVE ( 'NONE', #54776, #39567, #62531, .T. ) ;
#52482=CARTESIAN_POINT ( 'NONE',  ( 3.780834652287974773, 8.352030633203080257, 10.60629927458383115 ) ) ;
#52483=ORIENTED_EDGE ( 'NONE', *, *, #13190, .F. ) ;
#52485=AXIS2_PLACEMENT_3D ( 'NONE', #3876, #25123, #19485 ) ;
#52489=CARTESIAN_POINT ( 'NONE',  ( 10.75853767213705225, 7.830989516993144051, -10.99661780661415733 ) ) ;
#52490=DIRECTION ( 'NONE',  ( -1.000000000000000000, 0.000000000000000000, 0.000000000000000000 ) ) ;
#52492=DIRECTION ( 'NONE',  ( -1.000000000000000000, 0.000000000000000000, -0.000000000000000000 ) ) ;
#52494=VECTOR ( 'NONE', #51954, 1000.000000000000000 ) ;
#52495=VERTEX_POINT ( 'NONE', #54562 ) ;
#52496=EDGE_CURVE ( 'NONE', #32830, #35021, #27832, .T. ) ;
#52497=VERTEX_POINT ( 'NONE', #64195 ) ;
#52499=VERTEX_POINT ( 'NONE', #12644 ) ;
#52502=CARTESIAN_POINT ( 'NONE',  ( -37.00000000000000711, 0.000000000000000000, 0.000000000000000000 ) ) ;
#52504=DIRECTION ( 'NONE',  ( 0.000000000000000000, -0.01356324068817991828, 0.9999080150203990547 ) ) ;
#52505=EDGE_CURVE ( 'NONE', #35632, #33360, #61814, .T. ) ;
#52507=CARTESIAN_POINT ( 'NONE',  ( -20.79170840334646542, 12.91784323155722980, -3.921648409140116698 ) ) ;
#52508=ORIENTED_EDGE ( 'NONE', *, *, #2841, .F. ) ;
#52509=AXIS2_PLACEMENT_3D ( 'NONE', #2449, #22051, #21405 ) ;
#52511=CIRCLE ( 'NONE', #25969, 12.18649999999999878 ) ;
#52512=DIRECTION ( 'NONE',  ( -1.000000000000000000, 0.000000000000000000, 0.000000000000000000 ) ) ;
#52514=DIRECTION ( 'NONE',  ( 1.000000000000000000, -0.000000000000000000, 0.000000000000000000 ) ) ;
#52516=EDGE_CURVE ( 'NONE', #32335, #51910, #18310, .T. ) ;
#52518=ORIENTED_EDGE ( 'NONE', *, *, #7054, .T. ) ;
#52520=CARTESIAN_POINT ( 'NONE',  ( -35.00000000000000000, 11.05394794832836780, -5.130401251914613603 ) ) ;
#52521=CARTESIAN_POINT ( 'NONE',  ( 36.00000000000000711, -6.265926637539571686, -11.10408318471057498 ) ) ;
#52525=CARTESIAN_POINT ( 'NONE',  ( 3.117994775788107020, 4.258268480479466156, 12.81686186562924057 ) ) ;
#52526=VERTEX_POINT ( 'NONE', #58569 ) ;
#52527=VERTEX_POINT ( 'NONE', #7684 ) ;
#52528=AXIS2_PLACEMENT_3D ( 'NONE', #33041, #12423, #22767 ) ;
#52529=VERTEX_POINT ( 'NONE', #12994 ) ;
#52532=CIRCLE ( 'NONE', #21766, 5.000000000000000888 ) ;
#52535=DIRECTION ( 'NONE',  ( 1.000000000000000000, 0.000000000000000000, 0.000000000000000000 ) ) ;
#52540=DIRECTION ( 'NONE',  ( 0.000000000000000000, 0.01356324068817998940, -0.9999080150203989437 ) ) ;
#52545=DIRECTION ( 'NONE',  ( 0.000000000000000000, -0.01356324068817998940, 0.9999080150203990547 ) ) ;
#52546=CARTESIAN_POINT ( 'NONE',  ( -36.00000000000000711, 0.1414404973752139416, 12.74921544981111232 ) ) ;
#52548=AXIS2_PLACEMENT_3D ( 'NONE', #36896, #1675, #52213 ) ;
#52549=VERTEX_POINT ( 'NONE', #18667 ) ;
#52550=CARTESIAN_POINT ( 'NONE',  ( -36.00000000000000711, -11.47561260193580956, 5.556331110570368992 ) ) ;
#52556=DIRECTION ( 'NONE',  ( -1.000000000000000000, -0.000000000000000000, 0.000000000000000000 ) ) ;
#52559=AXIS2_PLACEMENT_3D ( 'NONE', #25656, #5060, #50937 ) ;
#52560=ADVANCED_FACE ( 'NONE', ( #8991 ), #29274, .T. ) ;
#52563=DIRECTION ( 'NONE',  ( 0.000000000000000000, -0.01356324068817998940, 0.9999080150203990547 ) ) ;
#52565=EDGE_CURVE ( 'NONE', #20824, #38497, #2918, .T. ) ;
#52567=AXIS2_PLACEMENT_3D ( 'NONE', #25449, #9480, #4863 ) ;
#52569=EDGE_CURVE ( 'NONE', #4335, #18175, #14718, .T. ) ;
#52572=CARTESIAN_POINT ( 'NONE',  ( -37.00000000000000711, -12.54989509947649573, -2.250029553613892563 ) ) ;
#52575=VERTEX_POINT ( 'NONE', #4997 ) ;
#52577=FACE_OUTER_BOUND ( 'NONE', #15653, .T. ) ;
#52579=EDGE_CURVE ( 'NONE', #65758, #19449, #19300, .T. ) ;
#52580=FACE_OUTER_BOUND ( 'NONE', #19748, .T. ) ;
#52581=EDGE_LOOP ( 'NONE', ( #35785, #22829, #19768, #32011 ) ) ;
#52584=ORIENTED_EDGE ( 'NONE', *, *, #49324, .T. ) ;
#52587=AXIS2_PLACEMENT_3D ( 'NONE', #14400, #10724, #39685 ) ;
#52588=CARTESIAN_POINT ( 'NONE',  ( -35.00000000000000000, -11.35427606708809556, 4.426194442447198618 ) ) ;
#52590=EDGE_CURVE ( 'NONE', #21600, #51800, #9781, .T. ) ;
#52592=ADVANCED_FACE ( 'NONE', ( #25255 ), #9621, .T. ) ;
#52598=ORIENTED_EDGE ( 'NONE', *, *, #14772, .F. ) ;
#52599=EDGE_CURVE ( 'NONE', #42626, #21283, #28879, .T. ) ;
#52600=CARTESIAN_POINT ( 'NONE',  ( -35.00000000000000000, -1.262958560998674429, -12.12087942037211086 ) ) ;
#52602=COLOUR_RGB ( '', 0.72549020, 0.75294118, 0.79215686) ;
#52604=CARTESIAN_POINT ( 'NONE',  ( 10.56078269551218085, -11.97184738340593846, -0.8518863164657939357 ) ) ;
#52605=CARTESIAN_POINT ( 'NONE',  ( -19.62362846926599147, -4.052573403833378052, 11.29610975316521504 ) ) ;
#52606=DIRECTION ( 'NONE',  ( 1.000000000000000000, 0.000000000000000000, -0.000000000000000000 ) ) ;
#52608=FACE_OUTER_BOUND ( 'NONE', #57474, .T. ) ;
#52610=CARTESIAN_POINT ( 'NONE',  ( 6.646157311995629868, -5.064915162312895625, -10.88629149749473157 ) ) ;
#52611=ORIENTED_EDGE ( 'NONE', *, *, #59871, .F. ) ;
#52613=ORIENTED_EDGE ( 'NONE', *, *, #2350, .T. ) ;
#52614=CYLINDRICAL_SURFACE ( 'NONE', #65645, 12.18650000000000055 ) ;
#52619=DIRECTION ( 'NONE',  ( 1.000000000000000000, 0.000000000000000000, 0.000000000000000000 ) ) ;
#52621=ORIENTED_EDGE ( 'NONE', *, *, #19984, .T. ) ;
#52623=ORIENTED_EDGE ( 'NONE', *, *, #36524, .T. ) ;
#52628=DIRECTION ( 'NONE',  ( -1.000000000000000000, 0.000000000000000000, -0.000000000000000000 ) ) ;
#52630=CARTESIAN_POINT ( 'NONE',  ( 35.00000000000000000, 11.29812557209481483, 3.213188559034117819 ) ) ;
#52633=DIRECTION ( 'NONE',  ( 0.000000000000000000, -0.01356324068817999114, 0.9999080150203989437 ) ) ;
#52634=AXIS2_PLACEMENT_3D ( 'NONE', #31900, #16953, #57204 ) ;
#52636=CARTESIAN_POINT ( 'NONE',  ( -35.00000000000000000, -11.65150730582933392, -1.488153103997089888 ) ) ;
#52638=CARTESIAN_POINT ( 'NONE',  ( 35.00000000000000000, -10.14433819232439049, -6.753013023069681431 ) ) ;
#52639=ADVANCED_FACE ( 'NONE', ( #29580 ), #54871, .T. ) ;
#52640=DIRECTION ( 'NONE',  ( 0.000000000000000000, -0.4698238015817237101, -0.8827602140260384367 ) ) ;
#52642=CARTESIAN_POINT ( 'NONE',  ( 47.00000000000000711, 4.705694406421931860E-17, -3.469127814946512892E-15 ) ) ;
#52645=VERTEX_POINT ( 'NONE', #9293 ) ;
#52647=CARTESIAN_POINT ( 'NONE',  ( -35.00000000000000000, 7.094637218249357780, 10.59380114696472397 ) ) ;
#52650=CARTESIAN_POINT ( 'NONE',  ( -4.975205859172449507, -1.416020129149132778, -13.42553116244733680 ) ) ;
#52651=VERTEX_POINT ( 'NONE', #65796 ) ;
#52652=DIRECTION ( 'NONE',  ( -1.000000000000000000, -0.000000000000000000, -0.000000000000000000 ) ) ;
#52654=CARTESIAN_POINT ( 'NONE',  ( -29.43980975494970309, -3.641506875706030488, 25.00000000000000000 ) ) ;
#52655=ORIENTED_EDGE ( 'NONE', *, *, #64087, .T. ) ;
#52656=ORIENTED_EDGE ( 'NONE', *, *, #46782, .F. ) ;
#52658=DIRECTION ( 'NONE',  ( -1.000000000000000000, -1.836970198721029688E-16, 0.000000000000000000 ) ) ;
#52660=EDGE_CURVE ( 'NONE', #61666, #30718, #35865, .T. ) ;
#52661=CARTESIAN_POINT ( 'NONE',  ( 35.00000000000000000, -10.49591321039684289, -5.273331777780305707 ) ) ;
#52663=CARTESIAN_POINT ( 'NONE',  ( 22.68159425457230682, -4.559965384753717821, -12.70733236524612764 ) ) ;
#52665=ORIENTED_EDGE ( 'NONE', *, *, #53993, .F. ) ;
#52666=CARTESIAN_POINT ( 'NONE',  ( -4.975205859172452172, -1.416020129149132778, -11.91616074890918675 ) ) ;
#52669=CARTESIAN_POINT ( 'NONE',  ( 12.47628546223243617, 0.000000000000000000, -13.50000000000000178 ) ) ;
#52670=VERTEX_POINT ( 'NONE', #19639 ) ;
#52671=EDGE_CURVE ( 'NONE', #59777, #34070, #57689, .T. ) ;
#52675=VERTEX_POINT ( 'NONE', #47205 ) ;
#52676=CARTESIAN_POINT ( 'NONE',  ( 24.82652845881425208, -8.390869743685021476, -8.578654028722157321 ) ) ;
#52678=FACE_OUTER_BOUND ( 'NONE', #22021, .T. ) ;
#52679=EDGE_LOOP ( 'NONE', ( #24548, #38909, #5468, #9693 ) ) ;
#52680=DIRECTION ( 'NONE',  ( 1.000000000000000000, -0.000000000000000000, 0.000000000000000000 ) ) ;
#52681=CARTESIAN_POINT ( 'NONE',  ( -37.00000000000000711, 5.273331777780488672, -10.49591321039675229 ) ) ;
#52682=DIRECTION ( 'NONE',  ( 0.000000000000000000, -0.01356324068817998940, 0.9999080150203990547 ) ) ;
#52683=ORIENTED_EDGE ( 'NONE', *, *, #29888, .T. ) ;
#52684=VERTEX_POINT ( 'NONE', #31868 ) ;
#52685=DIRECTION ( 'NONE',  ( 1.000000000000000000, 0.000000000000000000, -0.000000000000000000 ) ) ;
#52686=VERTEX_POINT ( 'NONE', #26905 ) ;
#52687=ORIENTED_EDGE ( 'NONE', *, *, #1449, .F. ) ;
#52688=CYLINDRICAL_SURFACE ( 'NONE', #52973, 12.74999999999999822 ) ;
#52689=CARTESIAN_POINT ( 'NONE',  ( 37.00000000000000711, -3.827046518385000429, 11.56998259273181162 ) ) ;
#52690=DIRECTION ( 'NONE',  ( 1.000000000000000000, 0.000000000000000000, -0.000000000000000000 ) ) ;
#52692=CYLINDRICAL_SURFACE ( 'NONE', #43351, 12.74999999999999822 ) ;
#52694=ADVANCED_FACE ( 'NONE', ( #62457 ), #41194, .T. ) ;
#52696=DIRECTION ( 'NONE',  ( 1.000000000000000000, -0.000000000000000000, 0.000000000000000000 ) ) ;
#52698=CIRCLE ( 'NONE', #37818, 12.18650000000000233 ) ;
#52699=ORIENTED_EDGE ( 'NONE', *, *, #25059, .T. ) ;
#52700=CARTESIAN_POINT ( 'NONE',  ( -37.00000000000000711, 11.80185301892987582, -4.824807283153995208 ) ) ;
#52702=EDGE_CURVE ( 'NONE', #886, #37463, #16203, .T. ) ;
#52704=CARTESIAN_POINT ( 'NONE',  ( 47.00000000000000711, 4.705694406421931860E-17, -3.469127814946512892E-15 ) ) ;
#52706=CYLINDRICAL_SURFACE ( 'NONE', #6501, 12.75000000000000178 ) ;
#52707=CARTESIAN_POINT ( 'NONE',  ( 10.09531169970623488, 1.650681656277897869, -11.88740217892082995 ) ) ;
#52708=EDGE_CURVE ( 'NONE', #30956, #2445, #19403, .T. ) ;
#52709=EDGE_CURVE ( 'NONE', #32709, #45989, #57502, .T. ) ;
#52710=ORIENTED_EDGE ( 'NONE', *, *, #56280, .T. ) ;
#52711=FACE_OUTER_BOUND ( 'NONE', #62278, .T. ) ;
#52715=EDGE_CURVE ( 'NONE', #36890, #52926, #23714, .T. ) ;
#52716=DIRECTION ( 'NONE',  ( -1.000000000000000000, 0.000000000000000000, 0.000000000000000000 ) ) ;
#52717=DIRECTION ( 'NONE',  ( 0.000000000000000000, 0.01356324068817998940, -0.9999080150203990547 ) ) ;
#52719=CARTESIAN_POINT ( 'NONE',  ( -35.00000000000000000, -4.237620530777717498, -11.42599468261433771 ) ) ;
#52720=CARTESIAN_POINT ( 'NONE',  ( -27.46687570686240676, -13.11534287648462360, -3.247842855528481731 ) ) ;
#52725=CYLINDRICAL_SURFACE ( 'NONE', #21348, 5.000000000000000888 ) ;
#52726=ORIENTED_EDGE ( 'NONE', *, *, #55672, .T. ) ;
#52728=ADVANCED_FACE ( 'NONE', ( #20920 ), #37188, .T. ) ;
#52729=VECTOR ( 'NONE', #63657, 1000.000000000000000 ) ;
#52732=EDGE_CURVE ( 'NONE', #63997, #36620, #14062, .T. ) ;
#52733=DIRECTION ( 'NONE',  ( 0.000000000000000000, 0.8369827122275362852, 0.5472293298355244140 ) ) ;
#52734=DIRECTION ( 'NONE',  ( 1.000000000000000000, 0.000000000000000000, -0.000000000000000000 ) ) ;
#52735=DIRECTION ( 'NONE',  ( 0.000000000000000000, 0.01356324068817998940, -0.9999080150203990547 ) ) ;
#52736=VECTOR ( 'NONE', #39941, 1000.000000000000000 ) ;
#52739=CARTESIAN_POINT ( 'NONE',  ( 35.00000000000000000, -7.376655759824808811, 9.700295462048739381 ) ) ;
#52740=CARTESIAN_POINT ( 'NONE',  ( -2.812344914800139151, 12.94091111974183050, 3.845999582511304027 ) ) ;
#52742=CARTESIAN_POINT ( 'NONE',  ( 9.775898761646960367, 6.948960757856110781, 11.57769295466150083 ) ) ;
#52745=ORIENTED_EDGE ( 'NONE', *, *, #17642, .T. ) ;
#52747=FACE_OUTER_BOUND ( 'NONE', #38958, .T. ) ;
#52751=CARTESIAN_POINT ( 'NONE',  ( 37.00000000000000711, 7.971186206369473837, -9.217970097227755844 ) ) ;
#52752=ORIENTED_EDGE ( 'NONE', *, *, #36722, .T. ) ;
#52753=CARTESIAN_POINT ( 'NONE',  ( -24.55403303652017399, -6.841724855681644790, 9.860983143791417049 ) ) ;
#52754=DIRECTION ( 'NONE',  ( 1.000000000000000000, -0.000000000000000000, -0.000000000000000000 ) ) ;
#52755=VERTEX_POINT ( 'NONE', #31554 ) ;
#52756=VERTEX_POINT ( 'NONE', #16603 ) ;
#52758=ORIENTED_EDGE ( 'NONE', *, *, #63633, .T. ) ;
#52759=DIRECTION ( 'NONE',  ( 0.000000000000000000, 0.3218879778915904044, -0.9467777615094594701 ) ) ;
#52760=CARTESIAN_POINT ( 'NONE',  ( -10.90165637463012516, -7.508992741355087652, 9.360289953322833867 ) ) ;
#52766=EDGE_CURVE ( 'NONE', #46638, #2528, #63992, .T. ) ;
#52768=CARTESIAN_POINT ( 'NONE',  ( 37.00000000000000711, 4.705694406421931860E-17, -3.469127814946512892E-15 ) ) ;
#52769=ORIENTED_EDGE ( 'NONE', *, *, #61158, .F. ) ;
#52770=CARTESIAN_POINT ( 'NONE',  ( -36.00000000000000711, -12.42372387097880626, -2.865935305911760267 ) ) ;
#52771=CARTESIAN_POINT ( 'NONE',  ( -9.274221350650309503, -12.48030023152219670, -5.158876694329755708 ) ) ;
#52773=CARTESIAN_POINT ( 'NONE',  ( -37.00000000000000711, 11.39945968423479883, -5.710938531231588122 ) ) ;
#52774=VERTEX_POINT ( 'NONE', #13251 ) ;
#52776=EDGE_CURVE ( 'NONE', #31867, #22729, #42710, .T. ) ;
#52779=ORIENTED_EDGE ( 'NONE', *, *, #11581, .T. ) ;
#52781=LINE ( 'NONE', #27491, #33539 ) ;
#52783=DIRECTION ( 'NONE',  ( -1.000000000000000000, 0.000000000000000000, 0.000000000000000000 ) ) ;
#52786=DIRECTION ( 'NONE',  ( 1.000000000000000000, 0.000000000000000000, -0.000000000000000000 ) ) ;
#52791=EDGE_LOOP ( 'NONE', ( #8295, #53075, #19183, #38 ) ) ;
#52793=ORIENTED_EDGE ( 'NONE', *, *, #2651, .T. ) ;
#52794=CYLINDRICAL_SURFACE ( 'NONE', #18534, 12.18649999999999878 ) ;
#52795=CARTESIAN_POINT ( 'NONE',  ( 35.00000000000000000, -11.30684963584392477, -4.545979934229371189 ) ) ;
#52797=FACE_OUTER_BOUND ( 'NONE', #45524, .T. ) ;
#52798=CARTESIAN_POINT ( 'NONE',  ( 35.00000000000000000, -9.908974237959688125, -6.307491713048997362 ) ) ;
#52799=EDGE_CURVE ( 'NONE', #46276, #55675, #15143, .T. ) ;
#52800=ORIENTED_EDGE ( 'NONE', *, *, #20493, .T. ) ;
#52801=EDGE_LOOP ( 'NONE', ( #47698, #1844, #56704, #44328 ) ) ;
#52804=CARTESIAN_POINT ( 'NONE',  ( 0.6825652211286046267, 0.5155054322761191132, 11.99253999668229653 ) ) ;
#52808=DIRECTION ( 'NONE',  ( -1.000000000000000000, 0.000000000000000000, 0.000000000000000000 ) ) ;
#52810=DIRECTION ( 'NONE',  ( 1.000000000000000000, 0.000000000000000000, 0.000000000000000000 ) ) ;
#52812=ORIENTED_EDGE ( 'NONE', *, *, #9137, .F. ) ;
#52814=EDGE_LOOP ( 'NONE', ( #4969, #5485, #7606, #24766 ) ) ;
#52815=CIRCLE ( 'NONE', #23064, 5.000000000000000888 ) ;
#52817=CARTESIAN_POINT ( 'NONE',  ( 35.00000000000000000, 4.705694406421931860E-17, -3.469127814946512892E-15 ) ) ;
#52819=CARTESIAN_POINT ( 'NONE',  ( 8.621148270653568702, 25.00000000000000000, -5.251012286260225537 ) ) ;
#52820=AXIS2_PLACEMENT_3D ( 'NONE', #4000, #19291, #5222 ) ;
#52821=CARTESIAN_POINT ( 'NONE',  ( 35.00000000000000000, 4.705694406421931860E-17, -3.469127814946512892E-15 ) ) ;
#52822=ORIENTED_EDGE ( 'NONE', *, *, #53823, .T. ) ;
#52824=( BOUNDED_CURVE ( )  B_SPLINE_CURVE ( 3, ( #42963, #63900, #58616, #17710 ),
 .UNSPECIFIED., .F., .F. ) 
 B_SPLINE_CURVE_WITH_KNOTS ( ( 4, 4 ),
 ( 1.252925267387246189, 1.274022647499400307 ),
 .UNSPECIFIED. ) 
 CURVE ( )  GEOMETRIC_REPRESENTATION_ITEM ( )  RATIONAL_B_SPLINE_CURVE ( ( 1.000000000000000000, 0.9999629087233127267, 0.9999629087233127267, 1.000000000000000000 ) ) 
 REPRESENTATION_ITEM ( '' )  );
#52825=LINE ( 'NONE', #16266, #12682 ) ;
#52826=CARTESIAN_POINT ( 'NONE',  ( -36.00000000000000711, -5.865551165831157654, 11.32068061209293219 ) ) ;
#52827=ORIENTED_EDGE ( 'NONE', *, *, #28482, .T. ) ;
#52828=VERTEX_POINT ( 'NONE', #13555 ) ;
#52829=CARTESIAN_POINT ( 'NONE',  ( 3.417879546546324310, 5.772183446363515991, 12.20553527385939141 ) ) ;
#52830=ORIENTED_EDGE ( 'NONE', *, *, #12305, .F. ) ;
#52833=ORIENTED_EDGE ( 'NONE', *, *, #4909, .T. ) ;
#52838=DIRECTION ( 'NONE',  ( 0.000000000000000000, -0.3218879778916040602, 0.9467777615094549182 ) ) ;
#52840=CARTESIAN_POINT ( 'NONE',  ( 35.00000000000000000, 6.036400161834703404, 10.07641281632170838 ) ) ;
#52841=DIRECTION ( 'NONE',  ( -1.000000000000000000, -0.000000000000000000, 0.000000000000000000 ) ) ;
#52842=EDGE_CURVE ( 'NONE', #33705, #63532, #20427, .T. ) ;
#52844=DIRECTION ( 'NONE',  ( -1.000000000000000000, 0.000000000000000000, 0.000000000000000000 ) ) ;
#52845=DIRECTION ( 'NONE',  ( -1.000000000000000000, -0.000000000000000000, 0.000000000000000000 ) ) ;
#52846=EDGE_CURVE ( 'NONE', #58393, #33730, #12913, .T. ) ;
#52849=CARTESIAN_POINT ( 'NONE',  ( 47.00000000000000711, 4.705694406421931860E-17, -3.469127814946512892E-15 ) ) ;
#52851=AXIS2_PLACEMENT_3D ( 'NONE', #23305, #37617, #12646 ) ;
#52852=ORIENTED_EDGE ( 'NONE', *, *, #35123, .T. ) ;
#52853=EDGE_CURVE ( 'NONE', #36890, #56049, #17593, .T. ) ;
#52855=CIRCLE ( 'NONE', #31615, 4.999999999999999112 ) ;
#52856=ORIENTED_EDGE ( 'NONE', *, *, #12653, .F. ) ;
#52857=EDGE_CURVE ( 'NONE', #49536, #9428, #22575, .T. ) ;
#52858=CYLINDRICAL_SURFACE ( 'NONE', #50838, 5.000000000000000888 ) ;
#52861=CARTESIAN_POINT ( 'NONE',  ( -25.86628395826706850, 25.00000000000000000, 10.84354029019568522 ) ) ;
#52865=CARTESIAN_POINT ( 'NONE',  ( -36.00000000000000711, 12.49688848680888142, -2.527899948230499572 ) ) ;
#52866=DIRECTION ( 'NONE',  ( 1.000000000000000000, 0.000000000000000000, -0.000000000000000000 ) ) ;
#52867=CIRCLE ( 'NONE', #24183, 12.18650000000000055 ) ;
#52868=CARTESIAN_POINT ( 'NONE',  ( -4.050859062405498534, 11.17340644476572109, 7.587242358561010924 ) ) ;
#52870=EDGE_CURVE ( 'NONE', #853, #49572, #58709, .T. ) ;
#52874=DIRECTION ( 'NONE',  ( 0.000000000000000000, 0.000000000000000000, -1.000000000000000000 ) ) ;
#52875=EDGE_LOOP ( 'NONE', ( #33787, #36746, #39598, #56512 ) ) ;
#52876=CARTESIAN_POINT ( 'NONE',  ( 37.00000000000000711, 4.705694406421931860E-17, -3.469127814946512892E-15 ) ) ;
#52877=ORIENTED_EDGE ( 'NONE', *, *, #38585, .T. ) ;
#52878=CARTESIAN_POINT ( 'NONE',  ( -18.37106647529896719, 3.948826690502797998, 11.33420767669607443 ) ) ;
#52880=LINE ( 'NONE', #2705, #45994 ) ;
#52883=ORIENTED_EDGE ( 'NONE', *, *, #43284, .T. ) ;
#52886=DIRECTION ( 'NONE',  ( 1.000000000000000000, 0.000000000000000000, 0.000000000000000000 ) ) ;
#52888=LINE ( 'NONE', #7321, #18336 ) ;
#52891=DIRECTION ( 'NONE',  ( -1.000000000000000000, 0.000000000000000000, 0.000000000000000000 ) ) ;
#52893=ORIENTED_EDGE ( 'NONE', *, *, #14998, .T. ) ;
#52895=CARTESIAN_POINT ( 'NONE',  ( 35.00000000000000000, -11.32068061209299081, -5.865551165831040414 ) ) ;
#52896=CARTESIAN_POINT ( 'NONE',  ( 24.83648533618617193, -1.531185848485796530, 11.90359809980858330 ) ) ;
#52899=AXIS2_PLACEMENT_3D ( 'NONE', #3472, #3134, #59301 ) ;
#52900=CARTESIAN_POINT ( 'NONE',  ( 35.00000000000000000, 11.78977382767499549, -4.245927698352105928 ) ) ;
#52903=CARTESIAN_POINT ( 'NONE',  ( 8.460324815083970051, 3.946969223371512125, -12.91307448586167617 ) ) ;
#52905=CIRCLE ( 'NONE', #16776, 5.000000000000000000 ) ;
#52908=CARTESIAN_POINT ( 'NONE',  ( -35.00000000000000000, -6.036400161834495570, -10.07641281632183983 ) ) ;
#52909=DIRECTION ( 'NONE',  ( -1.000000000000000000, 0.000000000000000000, -0.000000000000000000 ) ) ;
#52912=DIRECTION ( 'NONE',  ( 0.000000000000000000, 0.01356324068817992175, -0.9999080150203990547 ) ) ;
#52914=ORIENTED_EDGE ( 'NONE', *, *, #9296, .F. ) ;
#52915=CARTESIAN_POINT ( 'NONE',  ( 35.00000000000000000, 10.68873102412842258, -6.950793414699832695 ) ) ;
#52916=ORIENTED_EDGE ( 'NONE', *, *, #52223, .T. ) ;
#52919=DIRECTION ( 'NONE',  ( 1.000000000000000000, 0.000000000000000000, 0.000000000000000000 ) ) ;
#52921=ORIENTED_EDGE ( 'NONE', *, *, #27101, .F. ) ;
#52922=CARTESIAN_POINT ( 'NONE',  ( -18.12908327424137767, 6.849030978105520973, 9.857092249840578191 ) ) ;
#52925=ORIENTED_EDGE ( 'NONE', *, *, #561, .T. ) ;
#52926=VERTEX_POINT ( 'NONE', #12566 ) ;
#52930=VERTEX_POINT ( 'NONE', #53820 ) ;
#52931=EDGE_CURVE ( 'NONE', #16286, #12785, #49121, .T. ) ;
#52933=CARTESIAN_POINT ( 'NONE',  ( -35.00000000000000000, 9.821084925794572484, 7.215058775251292467 ) ) ;
#52935=FACE_OUTER_BOUND ( 'NONE', #820, .T. ) ;
#52937=DIRECTION ( 'NONE',  ( 0.000000000000000000, 0.01356324068817992175, -0.9999080150203990547 ) ) ;
#52940=AXIS2_PLACEMENT_3D ( 'NONE', #13289, #39856, #18289 ) ;
#52943=DIRECTION ( 'NONE',  ( 0.000000000000000000, -0.9987865678893271815, 0.04924826701375695226 ) ) ;
#52945=CARTESIAN_POINT ( 'NONE',  ( 22.62448365577994736, 12.20317485621798781, -5.782486214010236658 ) ) ;
#52946=DIRECTION ( 'NONE',  ( 0.000000000000000000, 0.01356324068817300540, -0.9999080150203989437 ) ) ;
#52947=CARTESIAN_POINT ( 'NONE',  ( 35.00000000000000000, 11.13736569743274174, -4.946702696913213515 ) ) ;
#52951=EDGE_LOOP ( 'NONE', ( #13975, #30785, #65038, #47358 ) ) ;
#52954=ORIENTED_EDGE ( 'NONE', *, *, #33030, .T. ) ;
#52956=CARTESIAN_POINT ( 'NONE',  ( -35.00000000000000000, -2.220215194441821360, -11.98254675519230794 ) ) ;
#52957=ORIENTED_EDGE ( 'NONE', *, *, #65306, .T. ) ;
#52959=VERTEX_POINT ( 'NONE', #55106 ) ;
#52964=EDGE_CURVE ( 'NONE', #57074, #15972, #1363, .T. ) ;
#52965=VECTOR ( 'NONE', #54256, 1000.000000000000000 ) ;
#52967=CYLINDRICAL_SURFACE ( 'NONE', #51467, 4.999999999999998224 ) ;
#52968=DIRECTION ( 'NONE',  ( -1.000000000000000000, 0.000000000000000000, 0.000000000000000000 ) ) ;
#52969=DIRECTION ( 'NONE',  ( 0.000000000000000000, 0.7381862504171926576, -0.6745969609292690183 ) ) ;
#52971=VERTEX_POINT ( 'NONE', #20529 ) ;
#52972=DIRECTION ( 'NONE',  ( 0.000000000000000000, -0.01356324068817991828, 0.9999080150203990547 ) ) ;
#52973=AXIS2_PLACEMENT_3D ( 'NONE', #32686, #37038, #11444 ) ;
#52976=CARTESIAN_POINT ( 'NONE',  ( -27.45775109278351067, -11.83395752356219255, -1.989333891161980894 ) ) ;
#52977=ORIENTED_EDGE ( 'NONE', *, *, #1005, .F. ) ;
#52978=FACE_OUTER_BOUND ( 'NONE', #1743, .T. ) ;
#52981=EDGE_CURVE ( 'NONE', #58976, #2866, #10209, .T. ) ;
#52983=CYLINDRICAL_SURFACE ( 'NONE', #9178, 5.000000000000000888 ) ;
#52984=LINE ( 'NONE', #7102, #2409 ) ;
#52985=AXIS2_PLACEMENT_3D ( 'NONE', #36123, #16843, #31796 ) ;
#52986=CARTESIAN_POINT ( 'NONE',  ( 35.00000000000000000, 12.63095688309028830, -1.738225594540042884 ) ) ;
#52987=ORIENTED_EDGE ( 'NONE', *, *, #40924, .F. ) ;
#52988=DIRECTION ( 'NONE',  ( 0.000000000000000000, 0.01356324068817991828, -0.9999080150203990547 ) ) ;
#52991=CARTESIAN_POINT ( 'NONE',  ( 13.39599373663352466, 12.21273670597637384, -5.770182307986416070 ) ) ;
#52992=ORIENTED_EDGE ( 'NONE', *, *, #44023, .T. ) ;
#52993=AXIS2_PLACEMENT_3D ( 'NONE', #27027, #62258, #11709 ) ;
#52994=VERTEX_POINT ( 'NONE', #24197 ) ;
#52995=DIRECTION ( 'NONE',  ( 1.000000000000000000, 0.000000000000000000, 0.000000000000000000 ) ) ;
#52997=AXIS2_PLACEMENT_3D ( 'NONE', #51230, #41880, #57190 ) ;
#52999=ORIENTED_EDGE ( 'NONE', *, *, #52842, .T. ) ;
#53000=DIRECTION ( 'NONE',  ( -1.000000000000000000, 0.000000000000000000, -0.000000000000000000 ) ) ;
#53001=DIRECTION ( 'NONE',  ( 0.000000000000000000, -0.8169148498130338609, 0.5767582926624880146 ) ) ;
#53003=DIRECTION ( 'NONE',  ( -1.000000000000000000, -1.836970198721029688E-16, -0.000000000000000000 ) ) ;
#53005=CYLINDRICAL_SURFACE ( 'NONE', #33763, 13.50000000000000178 ) ;
#53007=DIRECTION ( 'NONE',  ( 1.000000000000000000, 0.000000000000000000, 0.000000000000000000 ) ) ;
#53008=( BOUNDED_CURVE ( )  B_SPLINE_CURVE ( 3, ( #5070, #46289, #5394, #35301 ),
 .UNSPECIFIED., .F., .F. ) 
 B_SPLINE_CURVE_WITH_KNOTS ( ( 4, 4 ),
 ( 2.503486317769501479, 2.552693758193947282 ),
 .UNSPECIFIED. ) 
 CURVE ( )  GEOMETRIC_REPRESENTATION_ITEM ( )  RATIONAL_B_SPLINE_CURVE ( ( 1.000000000000000000, 0.9997982291625954199, 0.9997982291625954199, 1.000000000000000000 ) ) 
 REPRESENTATION_ITEM ( '' )  );
#53011=DIRECTION ( 'NONE',  ( -1.000000000000000000, 0.000000000000000000, 0.000000000000000000 ) ) ;
#53015=AXIS2_PLACEMENT_3D ( 'NONE', #4041, #49920, #64534 ) ;
#53016=CYLINDRICAL_SURFACE ( 'NONE', #41722, 12.18650000000000055 ) ;
#53017=EDGE_CURVE ( 'NONE', #43073, #47572, #2412, .T. ) ;
#53018=CARTESIAN_POINT ( 'NONE',  ( -35.00000000000000000, 4.041347439435861943, 11.02904044024210428 ) ) ;
#53019=ADVANCED_FACE ( 'NONE', ( #254 ), #4595, .T. ) ;
#53020=DIRECTION ( 'NONE',  ( -0.000000000000000000, -0.000000000000000000, -1.000000000000000000 ) ) ;
#53027=CYLINDRICAL_SURFACE ( 'NONE', #53206, 5.000000000000000888 ) ;
#53028=AXIS2_PLACEMENT_3D ( 'NONE', #41480, #61776, #36517 ) ;
#53029=ORIENTED_EDGE ( 'NONE', *, *, #61771, .T. ) ;
#53030=CARTESIAN_POINT ( 'NONE',  ( 18.82996414057443957, -4.825507986298288365, 10.99672610388072869 ) ) ;
#53034=ORIENTED_EDGE ( 'NONE', *, *, #52776, .F. ) ;
#53037=ORIENTED_EDGE ( 'NONE', *, *, #48896, .T. ) ;
#53038=AXIS2_PLACEMENT_3D ( 'NONE', #50220, #10280, #4677 ) ;
#53040=CARTESIAN_POINT ( 'NONE',  ( 35.00000000000000000, 4.705694406421931860E-17, -3.469127814946512892E-15 ) ) ;
#53041=EDGE_CURVE ( 'NONE', #26195, #8028, #3933, .T. ) ;
#53044=FACE_OUTER_BOUND ( 'NONE', #7738, .T. ) ;
#53046=CYLINDRICAL_SURFACE ( 'NONE', #30413, 12.75000000000000178 ) ;
#53047=LINE ( 'NONE', #33737, #31200 ) ;
#53048=LINE ( 'NONE', #32739, #85 ) ;
#53049=CARTESIAN_POINT ( 'NONE',  ( 37.00000000000000711, -9.321877890560486435, -7.146664589317880178 ) ) ;
#53050=CARTESIAN_POINT ( 'NONE',  ( -37.00000000000000711, -3.213188559034318992, 11.29812557209475798 ) ) ;
#53051=CARTESIAN_POINT ( 'NONE',  ( -35.00000000000000000, -12.18632975068352842, -0.06441628369849203284 ) ) ;
#53052=ORIENTED_EDGE ( 'NONE', *, *, #60136, .F. ) ;
#53054=ORIENTED_EDGE ( 'NONE', *, *, #58476, .T. ) ;
#53055=CARTESIAN_POINT ( 'NONE',  ( 23.48656543641403971, 2.894652911351478064, -11.64991943752887416 ) ) ;
#53059=FACE_OUTER_BOUND ( 'NONE', #45245, .T. ) ;
#53061=DIRECTION ( 'NONE',  ( -1.000000000000000000, -0.000000000000000000, -0.000000000000000000 ) ) ;
#53063=CIRCLE ( 'NONE', #10721, 12.18650000000000233 ) ;
#53066=VERTEX_POINT ( 'NONE', #61396 ) ;
#53068=VECTOR ( 'NONE', #20544, 1000.000000000000000 ) ;
#53069=DIRECTION ( 'NONE',  ( 1.000000000000000000, 0.000000000000000000, 0.000000000000000000 ) ) ;
#53071=ORIENTED_EDGE ( 'NONE', *, *, #24613, .T. ) ;
#53074=EDGE_CURVE ( 'NONE', #57088, #50922, #56060, .T. ) ;
#53075=ORIENTED_EDGE ( 'NONE', *, *, #61568, .F. ) ;
#53077=CYLINDRICAL_SURFACE ( 'NONE', #63826, 4.500030059823568074 ) ;
#53078=CARTESIAN_POINT ( 'NONE',  ( 12.27828125814611226, 0.5230329997979927814, 13.48988865648588664 ) ) ;
#53079=EDGE_CURVE ( 'NONE', #21538, #51040, #30016, .T. ) ;
#53081=CIRCLE ( 'NONE', #24396, 5.000000000000000888 ) ;
#53082=CARTESIAN_POINT ( 'NONE',  ( 35.00000000000000000, 0.7008968033240532414, 12.16632754454235332 ) ) ;
#53084=LINE ( 'NONE', #48763, #33336 ) ;
#53085=AXIS2_PLACEMENT_3D ( 'NONE', #6279, #41838, #31844 ) ;
#53086=ORIENTED_EDGE ( 'NONE', *, *, #52870, .F. ) ;
#53089=DIRECTION ( 'NONE',  ( 0.000000000000000000, -0.1387779952735886391, 0.9903235168508540687 ) ) ;
#53090=FACE_OUTER_BOUND ( 'NONE', #13710, .T. ) ;
#53091=LINE ( 'NONE', #7530, #55199 ) ;
#53092=AXIS2_PLACEMENT_3D ( 'NONE', #6632, #26901, #47202 ) ;
#53093=CARTESIAN_POINT ( 'NONE',  ( 29.20115507325780513, 4.760464791327699174, 11.01582872674790714 ) ) ;
#53094=ADVANCED_FACE ( 'NONE', ( #20846 ), #56422, .T. ) ;
#53095=EDGE_LOOP ( 'NONE', ( #15338, #58937, #18215, #43436 ) ) ;
#53099=ORIENTED_EDGE ( 'NONE', *, *, #5519, .F. ) ;
#53102=EDGE_CURVE ( 'NONE', #33298, #44156, #26173, .T. ) ;
#53106=ORIENTED_EDGE ( 'NONE', *, *, #42480, .T. ) ;
#53107=DIRECTION ( 'NONE',  ( 0.000000000000000000, 0.01356324068817992522, -0.9999080150203990547 ) ) ;
#53108=CARTESIAN_POINT ( 'NONE',  ( -37.00000000000000711, 0.000000000000000000, 0.000000000000000000 ) ) ;
#53110=FACE_OUTER_BOUND ( 'NONE', #12379, .T. ) ;
#53113=CARTESIAN_POINT ( 'NONE',  ( 26.34661844826604593, 25.00000000000000000, 3.317828791472333005 ) ) ;
#53114=DIRECTION ( 'NONE',  ( 1.000000000000000000, 0.000000000000000000, 0.000000000000000000 ) ) ;
#53115=ORIENTED_EDGE ( 'NONE', *, *, #24719, .T. ) ;
#53117=DIRECTION ( 'NONE',  ( 1.000000000000000000, 0.000000000000000000, 0.000000000000000000 ) ) ;
#53120=CARTESIAN_POINT ( 'NONE',  ( -9.039297670793269290, -2.446522702784146741, -13.27730549576870978 ) ) ;
#53122=CARTESIAN_POINT ( 'NONE',  ( 37.00000000000000711, -0.1414404973753014549, -12.74921544981111055 ) ) ;
#53124=CARTESIAN_POINT ( 'NONE',  ( 35.00000000000000000, 4.705694406421931860E-17, -3.469127814946512892E-15 ) ) ;
#53125=CIRCLE ( 'NONE', #16996, 12.18650000000000055 ) ;
#53127=ORIENTED_EDGE ( 'NONE', *, *, #56669, .T. ) ;
#53129=ORIENTED_EDGE ( 'NONE', *, *, #45323, .T. ) ;
#53130=CIRCLE ( 'NONE', #50999, 12.18650000000000055 ) ;
#53133=DIRECTION ( 'NONE',  ( 0.000000000000000000, 0.01356324068817998940, -0.9999080150203990547 ) ) ;
#53134=CARTESIAN_POINT ( 'NONE',  ( 35.00000000000000000, -11.44858830469738109, 2.627174906297032209 ) ) ;
#53140=VERTEX_POINT ( 'NONE', #27804 ) ;
#53141=CARTESIAN_POINT ( 'NONE',  ( 35.00000000000000000, 1.771820996347156507, -11.61175578952786935 ) ) ;
#53142=CIRCLE ( 'NONE', #29762, 5.000000000000000888 ) ;
#53143=ORIENTED_EDGE ( 'NONE', *, *, #6039, .F. ) ;
#53144=( NAMED_UNIT ( * ) PLANE_ANGLE_UNIT ( ) SI_UNIT ( $, .RADIAN. ) );
#53146=CARTESIAN_POINT ( 'NONE',  ( 17.48690873012385438, 10.08597650261509671, 8.981318438147098959 ) ) ;
#53148=CARTESIAN_POINT ( 'NONE',  ( -35.00000000000000000, -5.130401251914653571, -11.05394794832835359 ) ) ;
#53149=VERTEX_POINT ( 'NONE', #43750 ) ;
#53150=FACE_OUTER_BOUND ( 'NONE', #21167, .T. ) ;
#53151=DIRECTION ( 'NONE',  ( 0.000000000000000000, -0.2006870767258747135, 0.9796553971857772103 ) ) ;
#53154=ORIENTED_EDGE ( 'NONE', *, *, #27600, .T. ) ;
#53155=CARTESIAN_POINT ( 'NONE',  ( -35.00000000000000000, -0.7536123767499333104, 11.72195762423409704 ) ) ;
#53156=ORIENTED_EDGE ( 'NONE', *, *, #61473, .T. ) ;
#53158=VERTEX_POINT ( 'NONE', #42752 ) ;
#53159=CARTESIAN_POINT ( 'NONE',  ( -35.00000000000000000, 0.000000000000000000, 0.000000000000000000 ) ) ;
#53161=ORIENTED_EDGE ( 'NONE', *, *, #19608, .F. ) ;
#53165=AXIS2_PLACEMENT_3D ( 'NONE', #19261, #19596, #39858 ) ;
#53166=FACE_BOUND ( 'NONE', #16490, .T. ) ;
#53167=CIRCLE ( 'NONE', #2177, 4.999999999999999112 ) ;
#53170=CIRCLE ( 'NONE', #59521, 12.74999999999999822 ) ;
#53171=CARTESIAN_POINT ( 'NONE',  ( 35.00000000000000000, -12.18359334611896294, -0.2661492558802951991 ) ) ;
#53172=EDGE_LOOP ( 'NONE', ( #54869, #28951, #4124, #15519 ) ) ;
#53173=CARTESIAN_POINT ( 'NONE',  ( -35.00000000000000000, -4.426194442447158650, -11.35427606708811155 ) ) ;
#53175=CARTESIAN_POINT ( 'NONE',  ( 37.00000000000000711, -9.752226076388938125, -6.547236723513990775 ) ) ;
#53176=DIRECTION ( 'NONE',  ( 0.000000000000000000, 0.01356324068817998940, -0.9999080150203990547 ) ) ;
#53177=CARTESIAN_POINT ( 'NONE',  ( 29.51976981715666781, 4.571419055710094881, 11.09513982864076276 ) ) ;
#53178=DIRECTION ( 'NONE',  ( 0.000000000000000000, 0.7617968321374900542, 0.6478160128811920604 ) ) ;
#53180=CARTESIAN_POINT ( 'NONE',  ( -35.00000000000000000, 9.060822531526156354, -7.474872387600913548 ) ) ;
#53182=AXIS2_PLACEMENT_3D ( 'NONE', #63591, #48003, #12077 ) ;
#53184=ORIENTED_EDGE ( 'NONE', *, *, #45109, .F. ) ;
#53189=FACE_OUTER_BOUND ( 'NONE', #2396, .T. ) ;
#53190=CIRCLE ( 'NONE', #12826, 5.000000000000000888 ) ;
#53192=LINE ( 'NONE', #7639, #29641 ) ;
#53194=CARTESIAN_POINT ( 'NONE',  ( -35.00000000000000000, 0.000000000000000000, 0.000000000000000000 ) ) ;
#53195=CARTESIAN_POINT ( 'NONE',  ( 35.00000000000000000, 2.220215194442072271, 11.98254675519225287 ) ) ;
#53199=EDGE_CURVE ( 'NONE', #62291, #50465, #19439, .T. ) ;
#53202=EDGE_LOOP ( 'NONE', ( #43874, #54546, #40977, #9773 ) ) ;
#53203=CARTESIAN_POINT ( 'NONE',  ( 36.00000000000000711, -10.12742074351890764, 7.745827850123114366 ) ) ;
#53204=DIRECTION ( 'NONE',  ( -1.000000000000000000, 0.000000000000000000, -0.000000000000000000 ) ) ;
#53205=CARTESIAN_POINT ( 'NONE',  ( 35.00000000000000000, 4.705694406421931860E-17, -3.469127814946512892E-15 ) ) ;
#53206=AXIS2_PLACEMENT_3D ( 'NONE', #7462, #42056, #1843 ) ;
#53208=ORIENTED_EDGE ( 'NONE', *, *, #25982, .T. ) ;
#53209=CARTESIAN_POINT ( 'NONE',  ( -35.00000000000000000, -5.636262487437237567, -10.80478261802188023 ) ) ;
#53210=ADVANCED_FACE ( 'NONE', ( #44082 ), #12490, .T. ) ;
#53216=CARTESIAN_POINT ( 'NONE',  ( -36.00000000000000711, -8.954052073409537016, -9.076753354954096409 ) ) ;
#53217=CARTESIAN_POINT ( 'NONE',  ( -29.68541646480307250, -1.416020129149132334, 13.42553116244733680 ) ) ;
#53220=ORIENTED_EDGE ( 'NONE', *, *, #19749, .T. ) ;
#53221=VERTEX_POINT ( 'NONE', #58402 ) ;
#53222=ORIENTED_EDGE ( 'NONE', *, *, #49350, .F. ) ;
#53223=DIRECTION ( 'NONE',  ( 0.000000000000000000, -0.2006870767258747135, 0.9796553971857772103 ) ) ;
#53225=CIRCLE ( 'NONE', #33039, 12.74999999999999822 ) ;
#53226=CARTESIAN_POINT ( 'NONE',  ( 47.00000000000000711, 4.705694406421931860E-17, -3.469127814946512892E-15 ) ) ;
#53227=ADVANCED_FACE ( 'NONE', ( #37448 ), #49095, .T. ) ;
#53228=ORIENTED_EDGE ( 'NONE', *, *, #37073, .T. ) ;
#53229=DIRECTION ( 'NONE',  ( 0.000000000000000000, -0.01356324068817998940, 0.9999080150203990547 ) ) ;
#53230=AXIS2_PLACEMENT_3D ( 'NONE', #51576, #6985, #27258 ) ;
#53233=DIRECTION ( 'NONE',  ( -1.000000000000000000, 0.000000000000000000, 0.000000000000000000 ) ) ;
#53236=ORIENTED_EDGE ( 'NONE', *, *, #38834, .T. ) ;
#53238=VERTEX_POINT ( 'NONE', #48754 ) ;
#53239=DIRECTION ( 'NONE',  ( -1.000000000000000000, -0.000000000000000000, 0.000000000000000000 ) ) ;
#53240=ORIENTED_EDGE ( 'NONE', *, *, #48313, .F. ) ;
#53242=CARTESIAN_POINT ( 'NONE',  ( 35.00000000000000000, 9.040300684349800164, 7.499679039483956977 ) ) ;
#53244=AXIS2_PLACEMENT_3D ( 'NONE', #56431, #25856, #26492 ) ;
#53247=CARTESIAN_POINT ( 'NONE',  ( 35.00000000000000000, 9.040300684349800164, 7.499679039483956977 ) ) ;
#53248=DIRECTION ( 'NONE',  ( 1.000000000000000000, -0.000000000000000000, -0.000000000000000000 ) ) ;
#53251=CARTESIAN_POINT ( 'NONE',  ( -27.22418447007674658, -9.103645632685440248, -7.837741149085147185 ) ) ;
#53253=CARTESIAN_POINT ( 'NONE',  ( 37.00000000000000711, 6.657191900728455458, 9.677500615117825333 ) ) ;
#53255=DIRECTION ( 'NONE',  ( -1.000000000000000000, -1.836970198721029688E-16, 0.000000000000000000 ) ) ;
#53258=ORIENTED_EDGE ( 'NONE', *, *, #37931, .T. ) ;
#53259=CARTESIAN_POINT ( 'NONE',  ( -16.85489546068752276, 8.063588271002045005, 8.887448980655202391 ) ) ;
#53262=ORIENTED_EDGE ( 'NONE', *, *, #28869, .F. ) ;
#53263=AXIS2_PLACEMENT_3D ( 'NONE', #40515, #60812, #45187 ) ;
#53264=AXIS2_PLACEMENT_3D ( 'NONE', #51726, #11153, #15785 ) ;
#53266=VERTEX_POINT ( 'NONE', #63049 ) ;
#53267=LINE ( 'NONE', #43591, #10975 ) ;
#53269=CARTESIAN_POINT ( 'NONE',  ( -37.00000000000000711, 0.000000000000000000, 0.000000000000000000 ) ) ;
#53270=DIRECTION ( 'NONE',  ( 0.000000000000000000, -0.01356324068817998940, 0.9999080150203990547 ) ) ;
#53271=CARTESIAN_POINT ( 'NONE',  ( -2.532614230583026593, -7.965877694534051479, 10.89930238848911337 ) ) ;
#53272=CARTESIAN_POINT ( 'NONE',  ( -35.00000000000000000, 0.000000000000000000, 0.000000000000000000 ) ) ;
#53273=EDGE_LOOP ( 'NONE', ( #3789, #7932, #12659, #57635 ) ) ;
#53275=AXIS2_PLACEMENT_3D ( 'NONE', #37440, #37774, #54057 ) ;
#53276=EDGE_CURVE ( 'NONE', #1074, #31673, #23721, .T. ) ;
#53277=AXIS2_PLACEMENT_3D ( 'NONE', #47632, #62916, #8716 ) ;
#53281=VECTOR ( 'NONE', #10436, 1000.000000000000000 ) ;
#53282=CARTESIAN_POINT ( 'NONE',  ( 21.94459801178244618, 13.23030893428817123, -2.711026448255508647 ) ) ;
#53285=DIRECTION ( 'NONE',  ( -1.000000000000000000, 0.000000000000000000, 0.000000000000000000 ) ) ;
#53287=CIRCLE ( 'NONE', #3423, 12.75000000000000178 ) ;
#53289=ORIENTED_EDGE ( 'NONE', *, *, #46835, .T. ) ;
#53290=CARTESIAN_POINT ( 'NONE',  ( 12.63125402411999154, -9.907883201068845125, -6.772782016156807749 ) ) ;
#53291=VECTOR ( 'NONE', #6556, 1000.000000000000000 ) ;
#53292=VERTEX_POINT ( 'NONE', #7182 ) ;
#53293=DIRECTION ( 'NONE',  ( 0.9996161839461982224, 0.02770351589312032917, -0.000000000000000000 ) ) ;
#53297=VERTEX_POINT ( 'NONE', #47762 ) ;
#53298=VECTOR ( 'NONE', #38149, 1000.000000000000000 ) ;
#53299=DIRECTION ( 'NONE',  ( 1.000000000000000000, -0.000000000000000000, 0.000000000000000000 ) ) ;
#53302=DIRECTION ( 'NONE',  ( -1.000000000000000000, -1.836970198721029688E-16, -0.000000000000000000 ) ) ;
#53303=EDGE_LOOP ( 'NONE', ( #50618, #59288, #65157, #6087 ) ) ;
#53305=CARTESIAN_POINT ( 'NONE',  ( -10.60768675312085385, -9.408818418401033057, -7.467076076499517434 ) ) ;
#53308=AXIS2_PLACEMENT_3D ( 'NONE', #27234, #21609, #57513 ) ;
#53309=AXIS2_PLACEMENT_3D ( 'NONE', #33969, #54281, #32640 ) ;
#53310=EDGE_CURVE ( 'NONE', #6736, #19313, #28981, .T. ) ;
#53311=EDGE_LOOP ( 'NONE', ( #5299, #3353, #9540, #64783 ) ) ;
#53312=FACE_OUTER_BOUND ( 'NONE', #58150, .T. ) ;
#53313=CARTESIAN_POINT ( 'NONE',  ( 3.924654796536142243, 7.659842019319547113, 11.15136974237303669 ) ) ;
#53314=CARTESIAN_POINT ( 'NONE',  ( -37.00000000000000711, 7.215058775251399936, -9.821084925794492548 ) ) ;
#53316=ORIENTED_EDGE ( 'NONE', *, *, #19483, .T. ) ;
#53318=EDGE_CURVE ( 'NONE', #30510, #44234, #51309, .T. ) ;
#53320=CARTESIAN_POINT ( 'NONE',  ( -29.66395171513434548, -2.175773247908486141, -11.80721667090971749 ) ) ;
#53323=CARTESIAN_POINT ( 'NONE',  ( -27.75148563095054044, 11.73923255623741824, -2.552824637849768763 ) ) ;
#53325=CARTESIAN_POINT ( 'NONE',  ( -17.54726996257253191, 12.93490414535030020, 3.865003848717349033 ) ) ;
#53326=ORIENTED_EDGE ( 'NONE', *, *, #13311, .F. ) ;
#53327=CARTESIAN_POINT ( 'NONE',  ( 36.00000000000000711, -11.24036214326524608, -6.018036132182126963 ) ) ;
#53329=FACE_OUTER_BOUND ( 'NONE', #10314, .T. ) ;
#53331=CARTESIAN_POINT ( 'NONE',  ( -2.672122885467083986, 11.33640012973147293, 3.936387307894332110 ) ) ;
#53332=DIRECTION ( 'NONE',  ( -0.5551681190699946367, -0.8317381556525372810, 0.000000000000000000 ) ) ;
#53333=CARTESIAN_POINT ( 'NONE',  ( 37.00000000000000711, 4.705694406421931860E-17, -3.469127814946512892E-15 ) ) ;
#53337=ORIENTED_EDGE ( 'NONE', *, *, #13505, .T. ) ;
#53340=AXIS2_PLACEMENT_3D ( 'NONE', #63518, #53896, #33277 ) ;
#53341=EDGE_CURVE ( 'NONE', #17810, #26482, #32136, .T. ) ;
#53343=DIRECTION ( 'NONE',  ( 0.000000000000000000, -0.9796553971857763221, -0.2006870767258792099 ) ) ;
#53344=DIRECTION ( 'NONE',  ( 0.000000000000000000, 0.01356324068817998940, -0.9999080150203989437 ) ) ;
#53345=FACE_OUTER_BOUND ( 'NONE', #12900, .T. ) ;
#53347=DIRECTION ( 'NONE',  ( -1.000000000000000000, -0.000000000000000000, -0.000000000000000000 ) ) ;
#53348=CARTESIAN_POINT ( 'NONE',  ( -37.00000000000000711, -10.91536515067645041, -4.339012074900068683 ) ) ;
#53349=LINE ( 'NONE', #28716, #20662 ) ;
#53354=AXIS2_PLACEMENT_3D ( 'NONE', #35459, #60087, #51103 ) ;
#53355=CIRCLE ( 'NONE', #21504, 5.000000000000000888 ) ;
#53358=DIRECTION ( 'NONE',  ( -1.000000000000000000, 0.000000000000000000, 0.000000000000000000 ) ) ;
#53359=CIRCLE ( 'NONE', #24677, 5.000000000000000000 ) ;
#53361=CARTESIAN_POINT ( 'NONE',  ( 37.00000000000000711, -2.527899948230726057, -12.49688848680883346 ) ) ;
#53362=ORIENTED_EDGE ( 'NONE', *, *, #16533, .T. ) ;
#53363=DIRECTION ( 'NONE',  ( 0.000000000000000000, 0.01356324068817998940, -0.9999080150203990547 ) ) ;
#53364=DIRECTION ( 'NONE',  ( 0.000000000000000000, -0.01356324068817999114, 0.9999080150203989437 ) ) ;
#53366=EDGE_CURVE ( 'NONE', #64499, #22968, #45628, .T. ) ;
#53368=AXIS2_PLACEMENT_3D ( 'NONE', #53141, #43148, #63426 ) ;
#53370=EDGE_CURVE ( 'NONE', #18752, #38246, #15682, .T. ) ;
#53371=FACE_OUTER_BOUND ( 'NONE', #36175, .T. ) ;
#53372=CARTESIAN_POINT ( 'NONE',  ( -25.21046028333935496, -11.50704267535209269, 7.061154338470299940 ) ) ;
#53375=CARTESIAN_POINT ( 'NONE',  ( 35.00000000000000000, -8.366449238204431538, -9.621072037176965353 ) ) ;
#53378=DIRECTION ( 'NONE',  ( -1.000000000000000000, 0.000000000000000000, 0.000000000000000000 ) ) ;
#53379=ORIENTED_EDGE ( 'NONE', *, *, #32131, .T. ) ;
#53380=FACE_OUTER_BOUND ( 'NONE', #31845, .T. ) ;
#53381=CARTESIAN_POINT ( 'NONE',  ( 0.2851083653049504285, -0.4107471485392698018, 25.00000000000000000 ) ) ;
#53383=ORIENTED_EDGE ( 'NONE', *, *, #35018, .T. ) ;
#53384=ORIENTED_EDGE ( 'NONE', *, *, #10252, .F. ) ;
#53385=DIRECTION ( 'NONE',  ( 0.000000000000000000, 0.6745969609292609137, 0.7381862504172000961 ) ) ;
#53386=ORIENTED_EDGE ( 'NONE', *, *, #19065, .T. ) ;
#53387=DIRECTION ( 'NONE',  ( -1.000000000000000000, 0.000000000000000000, -0.000000000000000000 ) ) ;
#53388=CYLINDRICAL_SURFACE ( 'NONE', #25106, 5.000000000000000888 ) ;
#53389=CARTESIAN_POINT ( 'NONE',  ( -35.00000000000000000, -1.791059740004510070, 12.05416472667165273 ) ) ;
#53390=LINE ( 'NONE', #39382, #37236 ) ;
#53391=DIRECTION ( 'NONE',  ( 0.000000000000000000, -0.8696919319575130425, -0.4935949184179355131 ) ) ;
#53392=EDGE_CURVE ( 'NONE', #50038, #49437, #13796, .T. ) ;
#53393=DIRECTION ( 'NONE',  ( -1.000000000000000000, 0.000000000000000000, 0.000000000000000000 ) ) ;
#53394=DIRECTION ( 'NONE',  ( 1.000000000000000000, 0.000000000000000000, -0.000000000000000000 ) ) ;
#53395=VERTEX_POINT ( 'NONE', #31330 ) ;
#53399=AXIS2_PLACEMENT_3D ( 'NONE', #54992, #14096, #20407 ) ;
#53400=DIRECTION ( 'NONE',  ( 0.000000000000000000, -0.1387779952735679057, 0.9903235168508568442 ) ) ;
#53401=ORIENTED_EDGE ( 'NONE', *, *, #26617, .F. ) ;
#53402=CIRCLE ( 'NONE', #5616, 5.000000000000000888 ) ;
#53405=CARTESIAN_POINT ( 'NONE',  ( -24.80814996009129203, 10.56471359980137592, 8.406295728485659424 ) ) ;
#53406=ADVANCED_FACE ( 'NONE', ( #45309 ), #20040, .T. ) ;
#53408=CIRCLE ( 'NONE', #47051, 12.18650000000000055 ) ;
#53409=CARTESIAN_POINT ( 'NONE',  ( -24.47664113409060604, 11.24033395140356184, 7.479490891548917553 ) ) ;
#53410=VECTOR ( 'NONE', #8390, 1000.000000000000000 ) ;
#53413=EDGE_CURVE ( 'NONE', #16590, #40228, #59373, .T. ) ;
#53414=CARTESIAN_POINT ( 'NONE',  ( -36.00000000000000711, 12.57916205664481346, 2.080187960898606470 ) ) ;
#53417=FACE_OUTER_BOUND ( 'NONE', #21977, .T. ) ;
#53420=ORIENTED_EDGE ( 'NONE', *, *, #10070, .F. ) ;
#53421=ORIENTED_EDGE ( 'NONE', *, *, #42113, .T. ) ;
#53422=EDGE_CURVE ( 'NONE', #13725, #55868, #25794, .T. ) ;
#53423=DIRECTION ( 'NONE',  ( -1.000000000000000000, 0.000000000000000000, -0.000000000000000000 ) ) ;
#53424=VERTEX_POINT ( 'NONE', #10065 ) ;
#53425=AXIS2_PLACEMENT_3D ( 'NONE', #59910, #34609, #25294 ) ;
#53426=FACE_OUTER_BOUND ( 'NONE', #40725, .T. ) ;
#53427=CARTESIAN_POINT ( 'NONE',  ( -37.00000000000000711, -7.561043153947899498, -9.557269938331636183 ) ) ;
#53432=CARTESIAN_POINT ( 'NONE',  ( 37.00000000000000711, 4.705694406421931860E-17, -3.469127814946512892E-15 ) ) ;
#53434=EDGE_LOOP ( 'NONE', ( #51744, #26949, #57436, #12488 ) ) ;
#53435=DIRECTION ( 'NONE',  ( 0.000000000000000000, 0.8827602140260332186, -0.4698238015817332580 ) ) ;
#53436=ORIENTED_EDGE ( 'NONE', *, *, #45974, .F. ) ;
#53437=VECTOR ( 'NONE', #16188, 1000.000000000000000 ) ;
#53442=ORIENTED_EDGE ( 'NONE', *, *, #54524, .T. ) ;
#53444=ORIENTED_EDGE ( 'NONE', *, *, #2894, .T. ) ;
#53446=DIRECTION ( 'NONE',  ( 0.000000000000000000, -0.9246979985058763063, -0.3807014730195119601 ) ) ;
#53449=VERTEX_POINT ( 'NONE', #51305 ) ;
#53450=VECTOR ( 'NONE', #16249, 1000.000000000000000 ) ;
#53453=ADVANCED_FACE ( 'NONE', ( #45976 ), #50963, .T. ) ;
#53456=AXIS2_PLACEMENT_3D ( 'NONE', #28734, #58699, #63984 ) ;
#53457=AXIS2_PLACEMENT_3D ( 'NONE', #58205, #47262, #27598 ) ;
#53459=CARTESIAN_POINT ( 'NONE',  ( -36.00000000000000711, 1.908798535168378274, 12.60630747491664039 ) ) ;
#53461=CARTESIAN_POINT ( 'NONE',  ( 37.00000000000000711, 4.705694406421931860E-17, -3.469127814946512892E-15 ) ) ;
#53463=CIRCLE ( 'NONE', #58792, 5.000000000000000888 ) ;
#53466=CARTESIAN_POINT ( 'NONE',  ( -17.97127638550377782, 4.326068679718637178, -12.78996018384692590 ) ) ;
#53467=FACE_OUTER_BOUND ( 'NONE', #38168, .T. ) ;
#53471=CARTESIAN_POINT ( 'NONE',  ( -35.00000000000000000, 0.3025107581132838175, -11.74226168163341377 ) ) ;
#53472=EDGE_CURVE ( 'NONE', #7657, #55501, #7036, .T. ) ;
#53474=AXIS2_PLACEMENT_3D ( 'NONE', #21223, #16247, #36531 ) ;
#53475=VERTEX_POINT ( 'NONE', #52915 ) ;
#53476=FACE_OUTER_BOUND ( 'NONE', #60272, .T. ) ;
#53477=ORIENTED_EDGE ( 'NONE', *, *, #24483, .T. ) ;
#53479=DIRECTION ( 'NONE',  ( 0.000000000000000000, -0.01356324068817998940, 0.9999080150203990547 ) ) ;
#53480=AXIS2_PLACEMENT_3D ( 'NONE', #60323, #46033, #65620 ) ;
#53481=CARTESIAN_POINT ( 'NONE',  ( 35.00000000000000000, -11.61976888909157246, -3.827969819614423841 ) ) ;
#53482=DIRECTION ( 'NONE',  ( -1.000000000000000000, 0.000000000000000000, 0.000000000000000000 ) ) ;
#53484=AXIS2_PLACEMENT_3D ( 'NONE', #44554, #38940, #4021 ) ;
#53487=ORIENTED_EDGE ( 'NONE', *, *, #22925, .T. ) ;
#53488=VERTEX_POINT ( 'NONE', #62233 ) ;
#53490=ORIENTED_EDGE ( 'NONE', *, *, #41921, .T. ) ;
#53491=EDGE_CURVE ( 'NONE', #17535, #39390, #1412, .T. ) ;
#53494=VECTOR ( 'NONE', #2643, 1000.000000000000000 ) ;
#53495=EDGE_CURVE ( 'NONE', #26254, #22685, #57658, .T. ) ;
#53496=DIRECTION ( 'NONE',  ( -1.000000000000000000, 0.000000000000000000, -0.000000000000000000 ) ) ;
#53497=ORIENTED_EDGE ( 'NONE', *, *, #5702, .T. ) ;
#53501=VERTEX_POINT ( 'NONE', #27984 ) ;
#53502=ORIENTED_EDGE ( 'NONE', *, *, #12662, .F. ) ;
#53504=CARTESIAN_POINT ( 'NONE',  ( 37.00000000000000711, -9.493370459201747380, -6.917234959366797220 ) ) ;
#53506=CIRCLE ( 'NONE', #54544, 12.74999999999999822 ) ;
#53507=CYLINDRICAL_SURFACE ( 'NONE', #59909, 13.50000000000000178 ) ;
#53508=AXIS2_PLACEMENT_3D ( 'NONE', #39738, #40370, #56331 ) ;
#53511=CARTESIAN_POINT ( 'NONE',  ( 35.00000000000000000, 4.705694406421931860E-17, -3.469127814946512892E-15 ) ) ;
#53514=CARTESIAN_POINT ( 'NONE',  ( -35.00000000000000000, -4.986700593229626222, -10.63508530065527147 ) ) ;
#53516=DIRECTION ( 'NONE',  ( -1.000000000000000000, 0.000000000000000000, -0.000000000000000000 ) ) ;
#53517=EDGE_CURVE ( 'NONE', #13636, #24509, #26998, .T. ) ;
#53519=ORIENTED_EDGE ( 'NONE', *, *, #4053, .F. ) ;
#53520=VECTOR ( 'NONE', #58442, 1000.000000000000000 ) ;
#53521=DIRECTION ( 'NONE',  ( 0.000000000000000000, -0.01356324068817998940, 0.9999080150203990547 ) ) ;
#53522=AXIS2_PLACEMENT_3D ( 'NONE', #26275, #61505, #52216 ) ;
#53527=AXIS2_PLACEMENT_3D ( 'NONE', #46308, #21007, #61914 ) ;
#53528=CARTESIAN_POINT ( 'NONE',  ( -35.00000000000000000, 10.14408668126213442, 5.921969905510389154 ) ) ;
#53530=CARTESIAN_POINT ( 'NONE',  ( -7.181456785175555524, 25.00000000000000000, -10.45493698471458188 ) ) ;
#53531=CIRCLE ( 'NONE', #33328, 12.74999999999999822 ) ;
#53532=ORIENTED_EDGE ( 'NONE', *, *, #20528, .F. ) ;
#53533=CYLINDRICAL_SURFACE ( 'NONE', #13146, 4.999999999999999112 ) ;
#53536=DIRECTION ( 'NONE',  ( 1.000000000000000000, 0.000000000000000000, 0.000000000000000000 ) ) ;
#53538=AXIS2_PLACEMENT_3D ( 'NONE', #18260, #33848, #33207 ) ;
#53540=CARTESIAN_POINT ( 'NONE',  ( -10.90165637462999904, -7.508992741355384304, 11.21895841913464587 ) ) ;
#53544=CARTESIAN_POINT ( 'NONE',  ( -37.00000000000000711, 7.376655759825023750, -9.700295462048581285 ) ) ;
#53546=CARTESIAN_POINT ( 'NONE',  ( -18.11311222685468891, -13.11907746847522205, 3.257880281090000718 ) ) ;
#53552=ADVANCED_FACE ( 'NONE', ( #42582 ), #17684, .T. ) ;
#53554=AXIS2_PLACEMENT_3D ( 'NONE', #46562, #59120, #64397 ) ;
#53555=EDGE_CURVE ( 'NONE', #16089, #12285, #62884, .T. ) ;
#53557=DIRECTION ( 'NONE',  ( -1.000000000000000000, 0.000000000000000000, 0.000000000000000000 ) ) ;
#53558=ORIENTED_EDGE ( 'NONE', *, *, #28053, .F. ) ;
#53559=CARTESIAN_POINT ( 'NONE',  ( -35.00000000000000000, 1.591260454995410578, -12.08216339958899077 ) ) ;
#53561=DIRECTION ( 'NONE',  ( 0.000000000000000000, 0.01356324068817998940, -0.9999080150203990547 ) ) ;
#53564=ORIENTED_EDGE ( 'NONE', *, *, #56528, .F. ) ;
#53566=VERTEX_POINT ( 'NONE', #22671 ) ;
#53569=EDGE_CURVE ( 'NONE', #7570, #49200, #30050, .T. ) ;
#53570=AXIS2_PLACEMENT_3D ( 'NONE', #34635, #49952, #24681 ) ;
#53571=DIRECTION ( 'NONE',  ( 0.000000000000000000, 0.01356324068817998940, -0.9999080150203990547 ) ) ;
#53572=ORIENTED_EDGE ( 'NONE', *, *, #46854, .T. ) ;
#53577=CIRCLE ( 'NONE', #10031, 5.000000000000000000 ) ;
#53580=ORIENTED_EDGE ( 'NONE', *, *, #42539, .F. ) ;
#53581=VERTEX_POINT ( 'NONE', #57596 ) ;
#53582=CARTESIAN_POINT ( 'NONE',  ( -1.734723475976807094E-15, -3.469446951953614189E-15, 12.00000000000000178 ) ) ;
#53583=EDGE_LOOP ( 'NONE', ( #35463, #41659, #23001, #14693 ) ) ;
#53584=FILL_AREA_STYLE_COLOUR ( '', #54036 ) ;
#53585=ORIENTED_EDGE ( 'NONE', *, *, #23596, .T. ) ;
#53586=VECTOR ( 'NONE', #42437, 1000.000000000000000 ) ;
#53588=CARTESIAN_POINT ( 'NONE',  ( -35.00000000000000000, -11.59095880812009582, 1.903127969211145132 ) ) ;
#53590=AXIS2_PLACEMENT_3D ( 'NONE', #14865, #64761, #35153 ) ;
#53591=LINE ( 'NONE', #28300, #49748 ) ;
#53593=CARTESIAN_POINT ( 'NONE',  ( -35.00000000000000000, 7.215058775251398160, -9.821084925794490772 ) ) ;
#53594=CARTESIAN_POINT ( 'NONE',  ( 6.548939983325835712, -7.784018732717215450, -9.141476843261248320 ) ) ;
#53595=ORIENTED_EDGE ( 'NONE', *, *, #4484, .F. ) ;
#53597=ORIENTED_EDGE ( 'NONE', *, *, #5905, .F. ) ;
#53599=DIRECTION ( 'NONE',  ( 0.000000000000000000, -0.01356324068817992175, 0.9999080150203990547 ) ) ;
#53600=CIRCLE ( 'NONE', #36590, 12.18650000000000233 ) ;
#53601=ORIENTED_EDGE ( 'NONE', *, *, #60332, .F. ) ;
#53608=DIRECTION ( 'NONE',  ( -1.000000000000000000, -0.000000000000000000, 0.000000000000000000 ) ) ;
#53609=EDGE_CURVE ( 'NONE', #24621, #30317, #8801, .T. ) ;
#53610=ORIENTED_EDGE ( 'NONE', *, *, #3077, .T. ) ;
#53611=CARTESIAN_POINT ( 'NONE',  ( -28.85619398320021745, 3.750539801530000439, 12.96855624952675612 ) ) ;
#53615=CARTESIAN_POINT ( 'NONE',  ( -17.65546883943164147, -7.074198755462914434, 9.697947387155558374 ) ) ;
#53618=FACE_OUTER_BOUND ( 'NONE', #60572, .T. ) ;
#53620=ADVANCED_FACE ( 'NONE', ( #37629 ), #57926, .T. ) ;
#53627=CARTESIAN_POINT ( 'NONE',  ( 4.364872672758343342, -10.79984456430371864, -5.233809610475972818 ) ) ;
#53631=CARTESIAN_POINT ( 'NONE',  ( 12.86999076135267117, -11.06020008475422145, -4.659701079214955577 ) ) ;
#53632=ORIENTED_EDGE ( 'NONE', *, *, #12744, .T. ) ;
#53636=EDGE_LOOP ( 'NONE', ( #3116, #56596, #64936, #29092 ) ) ;
#53637=CARTESIAN_POINT ( 'NONE',  ( -35.00000000000000000, 11.32068061209295529, 5.865551165831117686 ) ) ;
#53638=DIRECTION ( 'NONE',  ( 0.000000000000000000, -0.01356324068817991828, 0.9999080150203990547 ) ) ;
#53640=CIRCLE ( 'NONE', #19655, 5.000000000000000000 ) ;
#53642=ORIENTED_EDGE ( 'NONE', *, *, #379, .T. ) ;
#53646=CARTESIAN_POINT ( 'NONE',  ( 35.00000000000000000, -4.018060380616318206, 11.50504120060946533 ) ) ;
#53648=DIRECTION ( 'NONE',  ( -1.000000000000000000, -0.000000000000000000, 0.000000000000000000 ) ) ;
#53649=CARTESIAN_POINT ( 'NONE',  ( -37.00000000000000711, -5.015831474386382105, 10.62137734850266391 ) ) ;
#53651=AXIS2_PLACEMENT_3D ( 'NONE', #61514, #56553, #21284 ) ;
#53653=DIRECTION ( 'NONE',  ( 0.000000000000000000, -0.01356324068817991828, 0.9999080150203990547 ) ) ;
#53654=CYLINDRICAL_SURFACE ( 'NONE', #27109, 5.000000000000000888 ) ;
#53655=CARTESIAN_POINT ( 'NONE',  ( -24.35981274529309815, 7.722558591804820516, 9.187561872115383110 ) ) ;
#53656=ORIENTED_EDGE ( 'NONE', *, *, #4136, .F. ) ;
#53658=EDGE_LOOP ( 'NONE', ( #33679, #51320, #51894, #33423 ) ) ;
#53659=DIRECTION ( 'NONE',  ( 0.000000000000000000, 0.5472293298355215274, -0.8369827122275381726 ) ) ;
#53660=EDGE_CURVE ( 'NONE', #31648, #51996, #55609, .T. ) ;
#53661=ORIENTED_EDGE ( 'NONE', *, *, #1605, .F. ) ;
#53662=DIRECTION ( 'NONE',  ( -1.000000000000000000, 0.000000000000000000, -0.000000000000000000 ) ) ;
#53663=DIRECTION ( 'NONE',  ( 0.000000000000000000, -0.01356324068817998940, 0.9999080150203990547 ) ) ;
#53664=CIRCLE ( 'NONE', #24986, 5.000000000000000888 ) ;
#53665=CARTESIAN_POINT ( 'NONE',  ( 47.00000000000000711, 4.705694406421931860E-17, -3.469127814946512892E-15 ) ) ;
#53666=DIRECTION ( 'NONE',  ( 0.000000000000000000, -0.9718671068226485410, 0.2355298848897412756 ) ) ;
#53668=CARTESIAN_POINT ( 'NONE',  ( 35.00000000000000000, 11.47758908105697806, 2.497432891016712286 ) ) ;
#53669=CARTESIAN_POINT ( 'NONE',  ( -9.813495697803759299, -4.010685208788737022, -12.89544212305399462 ) ) ;
#53671=EDGE_LOOP ( 'NONE', ( #15835, #23291, #27637, #60561, #6577, #15606, #15347, #38300, #51199, #3693, #3054, #54417, #53610, #18250, #11033, #12950, #60153, #58280, #9988, #7685, #55141, #35304, #22978, #34512, #43026, #7276, #52305, #64907, #63750, #49856, #30630, #27925, #51668, #99, #7950, #17597, #952, #8095, #13602, #15105, #19377, #49002, #28417, #58685, #34699, #37460, #30143, #50016, #43391, #4501, #15132, #32022, #46491, #27388, #25307, #34980, #60069, #5902, #18406, #10051, #1866, #8231, #47024, #61702, #47719, #8479, #36473, #54902, #21070, #49483, #24875, #53673, #21050, #49145, #13255, #55437, #5487, #10600, #50740, #22177, #47730, #53497, #26675, #32924, #10151, #41553, #30031, #27413, #22514, #38498, #1912, #29885, #29945, #28383, #19297, #4675, #36844, #6354, #27916, #47895, #2781, #53873, #7946, #41524, #65227, #46855, #35022, #3516, #65000, #61969, #18462, #16921, #5129, #44489, #24440, #4749, #50550, #39570, #1152, #55709, #38620, #28812, #59898, #3659, #43088, #51772, #20943, #9975, #42214, #6598, #43564, #30226, #43134, #30392, #53386, #39623, #24607, #13382, #52999, #53071, #19948, #61152, #54661, #43858, #15220, #44544, #1219, #15687, #64888, #25921, #38932, #61225, #11987, #11832, #6206, #25892, #18893, #27634, #23654, #8320, #33267, #61359, #54716, #4592, #3692, #7195, #36673, #54981, #21665, #2196, #55045, #28949, #51552, #47210, #47787, #45310, #22213, #60001, #42581, #38472, #32369, #21886, #56301, #64250, #22290, #54204, #42969, #16728, #24827, #28966, #31969, #32343, #9215, #22072, #3133, #8173, #11515, #28274, #7650, #4745, #17135, #48104, #33135, #55376, #38754, #27213, #23224, #47683, #20231, #5697, #46124, #55645, #802, #42290, #63427, #61099, #40522, #41307, #3947, #56751, #17409, #29930, #5742, #15106, #20100, #8441, #4517, #36428, #17071, #37892, #21709, #55834, #12571, #6483, #33518, #50682, #49713, #10271, #30763, #60465, #16818, #7416, #13439, #41015, #16938, #33507, #14186, #6742, #19709, #13874, #48004, #24323, #33095, #47581, #46422, #41927, #11601, #5090, #19559, #1333, #14114, #18683, #56297, #18700, #26497, #19867, #23381, #20089, #22724, #17207, #55216, #4095, #30858, #18716, #6137, #27542, #62217, #20127, #50840, #8729, #8810, #61787, #49227, #28310, #12228, #10524, #62552, #59095, #37370, #59216, #50977, #6664, #37846, #43538, #30729, #57563, #60687, #9910, #6997, #20020, #64672, #13633, #32839, #35864, #1857, #50226, #48069, #53746, #14608, #54294, #55850, #8568, #39851, #28935, #41864, #52877, #1700, #37133, #47592, #22833, #54825, #49082, #63093, #4367, #6685, #4001, #29577, #8990, #20142, #27317, #48538, #43459, #26060, #38260, #8750, #42597, #56552, #55412, #9183, #21614, #31616, #46709, #30813, #54805, #65, #48678, #6565, #15256, #38058, #35851, #43016, #2116, #50625, #36217, #30909, #55824, #28977, #44694, #6096, #16081, #30069, #51057, #17028, #55706, #25413, #11472, #8588, #40043, #53490, #6280, #14074, #57507, #55321, #16435, #1996, #20671, #7674, #60944, #46688, #59325, #53572, #11540, #20574, #19552, #41291, #25651, #65470, #717, #13012, #2694, #17716, #61014, #46771, #52095, #37596, #53674, #13919, #31299, #22987, #46469, #30058, #15351, #12483, #7600, #5049 ) ) ;
#53672=DIRECTION ( 'NONE',  ( 0.000000000000000000, 0.01356324068817998940, -0.9999080150203989437 ) ) ;
#53673=ORIENTED_EDGE ( 'NONE', *, *, #7991, .T. ) ;
#53674=ORIENTED_EDGE ( 'NONE', *, *, #15300, .T. ) ;
#53676=DIRECTION ( 'NONE',  ( 1.000000000000000000, 0.000000000000000000, 0.000000000000000000 ) ) ;
#53679=CARTESIAN_POINT ( 'NONE',  ( 29.51976981715666781, 25.00000000000000000, 11.09513982864076276 ) ) ;
#53680=DIRECTION ( 'NONE',  ( 1.000000000000000000, 0.000000000000000000, 0.000000000000000000 ) ) ;
#53683=FACE_OUTER_BOUND ( 'NONE', #27514, .T. ) ;
#53684=ADVANCED_FACE ( 'NONE', ( #43578 ), #33292, .T. ) ;
#53687=DIRECTION ( 'NONE',  ( 0.000000000000000000, 0.9999080150203989437, 0.01356324068818348313 ) ) ;
#53688=EDGE_CURVE ( 'NONE', #39957, #57971, #17352, .T. ) ;
#53689=CARTESIAN_POINT ( 'NONE',  ( -35.00000000000000000, 0.000000000000000000, 0.000000000000000000 ) ) ;
#53690=FACE_OUTER_BOUND ( 'NONE', #46005, .T. ) ;
#53691=DIRECTION ( 'NONE',  ( 1.000000000000000000, -0.000000000000000000, 0.000000000000000000 ) ) ;
#53692=ADVANCED_FACE ( 'NONE', ( #13649 ), #43253, .T. ) ;
#53693=VECTOR ( 'NONE', #31107, 1000.000000000000000 ) ;
#53695=EDGE_CURVE ( 'NONE', #8085, #31867, #53909, .T. ) ;
#53696=CARTESIAN_POINT ( 'NONE',  ( 9.769972995331128729, 2.020868073575773138, -11.83009605721721158 ) ) ;
#53697=ORIENTED_EDGE ( 'NONE', *, *, #60046, .T. ) ;
#53698=CARTESIAN_POINT ( 'NONE',  ( 37.00000000000000711, 2.627174906297071733, 11.44858830469737221 ) ) ;
#53699=LINE ( 'NONE', #13117, #47383 ) ;
#53700=CYLINDRICAL_SURFACE ( 'NONE', #12041, 12.74999999999999822 ) ;
#53702=EDGE_CURVE ( 'NONE', #16286, #57171, #33296, .T. ) ;
#53703=CARTESIAN_POINT ( 'NONE',  ( -35.00000000000000000, 1.488153103997124971, -11.65150730582933036 ) ) ;
#53704=CARTESIAN_POINT ( 'NONE',  ( 35.00000000000000000, 12.31350058095522826, -3.307597835713290024 ) ) ;
#53705=ORIENTED_EDGE ( 'NONE', *, *, #28219, .T. ) ;
#53706=CARTESIAN_POINT ( 'NONE',  ( -18.08686583997218733, 5.151216734910788908, 12.47858029384653733 ) ) ;
#53708=CARTESIAN_POINT ( 'NONE',  ( 35.00000000000000000, -11.86701198550353986, 2.772148766916240348 ) ) ;
#53709=ORIENTED_EDGE ( 'NONE', *, *, #38405, .T. ) ;
#53710=B_SPLINE_CURVE_WITH_KNOTS ( 'NONE', 3,
 ( #22034, #42288, #17390, #17045, #37324, #12054, #62926, #32641, #7385, #47976, #22710, #64167, #18638, #51666, #38900, #6109, #26368, #54844, #64475, #13927, #9265, #4964 ),
 .UNSPECIFIED., .F., .F.,
 ( 4, 2, 2, 2, 2, 2, 2, 2, 2, 2, 4 ),
 ( 3.903127820947815962E-18, 0.001139938506664698757, 0.001709907759997047159, 0.002279877013329395779, 0.003419815519994091283, 0.004559754026658787221, 0.005129723279991135407, 0.005699692533323483593, 0.006839631039988181699, 0.007979569546652876336, 0.009119508053317574442 ),
 .UNSPECIFIED. ) ;
#53711=CARTESIAN_POINT ( 'NONE',  ( 37.00000000000000711, 4.705694406421931860E-17, -3.469127814946512892E-15 ) ) ;
#53714=VERTEX_POINT ( 'NONE', #3053 ) ;
#53716=CIRCLE ( 'NONE', #10167, 4.999999999999999112 ) ;
#53717=VERTEX_POINT ( 'NONE', #8678 ) ;
#53718=DIRECTION ( 'NONE',  ( 0.000000000000000000, 0.2006870767258819854, -0.9796553971857756560 ) ) ;
#53720=DIRECTION ( 'NONE',  ( -1.000000000000000000, 0.000000000000000000, 0.000000000000000000 ) ) ;
#53721=DIRECTION ( 'NONE',  ( 0.000000000000000000, -0.5243256840888622650, -0.8515178078024832065 ) ) ;
#53722=FACE_OUTER_BOUND ( 'NONE', #38755, .T. ) ;
#53727=EDGE_LOOP ( 'NONE', ( #31869, #43830, #35477, #5992 ) ) ;
#53728=DIRECTION ( 'NONE',  ( 1.000000000000000000, 0.000000000000000000, 0.000000000000000000 ) ) ;
#53730=ORIENTED_EDGE ( 'NONE', *, *, #20552, .F. ) ;
#53731=CARTESIAN_POINT ( 'NONE',  ( -18.35026244561209552, 6.405804631758845069, 11.88625230963459067 ) ) ;
#53733=DIRECTION ( 'NONE',  ( -0.8867529933577791290, 0.000000000000000000, -0.4622435816439406930 ) ) ;
#53736=VECTOR ( 'NONE', #12736, 1000.000000000000000 ) ;
#53737=DIRECTION ( 'NONE',  ( -1.000000000000000000, 0.000000000000000000, -0.000000000000000000 ) ) ;
#53738=DIRECTION ( 'NONE',  ( 1.000000000000000000, -0.000000000000000000, -0.000000000000000000 ) ) ;
#53740=CIRCLE ( 'NONE', #44182, 12.18650000000000055 ) ;
#53741=CARTESIAN_POINT ( 'NONE',  ( -37.00000000000000711, -2.497432891016921008, 11.47758908105693720 ) ) ;
#53746=ORIENTED_EDGE ( 'NONE', *, *, #23337, .T. ) ;
#53747=DIRECTION ( 'NONE',  ( 1.000000000000000000, -0.000000000000000000, 0.000000000000000000 ) ) ;
#53751=CYLINDRICAL_SURFACE ( 'NONE', #33719, 4.999999999999999112 ) ;
#53755=LINE ( 'NONE', #8190, #49273 ) ;
#53756=ORIENTED_EDGE ( 'NONE', *, *, #37083, .T. ) ;
#53757=DIRECTION ( 'NONE',  ( 0.000000000000000000, 0.01356324068817998940, -0.9999080150203990547 ) ) ;
#53758=EDGE_CURVE ( 'NONE', #50610, #58860, #35238, .T. ) ;
#53761=DIRECTION ( 'NONE',  ( -0.000000000000000000, -0.000000000000000000, -1.000000000000000000 ) ) ;
#53763=CARTESIAN_POINT ( 'NONE',  ( 37.00000000000000711, 1.286231064351313735, -12.68495603654572257 ) ) ;
#53765=CARTESIAN_POINT ( 'NONE',  ( -28.19149199850170717, 12.81122912241742995, -4.268081906603431896 ) ) ;
#53766=EDGE_LOOP ( 'NONE', ( #6791, #12073, #21102, #5969 ) ) ;
#53767=CARTESIAN_POINT ( 'NONE',  ( 6.593984040184932560, -8.829533010771809742, -10.21404802089835151 ) ) ;
#53768=EDGE_CURVE ( 'NONE', #8663, #13128, #15299, .T. ) ;
#53771=FACE_OUTER_BOUND ( 'NONE', #38222, .T. ) ;
#53772=EDGE_CURVE ( 'NONE', #17578, #52527, #41208, .T. ) ;
#53776=DIRECTION ( 'NONE',  ( 0.000000000000000000, 0.01356324068817998940, -0.9999080150203989437 ) ) ;
#53778=ADVANCED_FACE ( 'NONE', ( #30906 ), #14948, .T. ) ;
#53782=CARTESIAN_POINT ( 'NONE',  ( -28.25057532999396059, -10.95459410115464216, -4.908922407349892936 ) ) ;
#53783=AXIS2_PLACEMENT_3D ( 'NONE', #29077, #9107, #33403 ) ;
#53784=VERTEX_POINT ( 'NONE', #20629 ) ;
#53787=EDGE_CURVE ( 'NONE', #15089, #18204, #35414, .T. ) ;
#53788=ORIENTED_EDGE ( 'NONE', *, *, #32069, .F. ) ;
#53790=DIRECTION ( 'NONE',  ( 1.000000000000000000, 0.000000000000000000, 0.000000000000000000 ) ) ;
#53791=DIRECTION ( 'NONE',  ( -1.000000000000000000, -0.000000000000000000, 0.000000000000000000 ) ) ;
#53792=CARTESIAN_POINT ( 'NONE',  ( -35.00000000000000000, 0.000000000000000000, 0.000000000000000000 ) ) ;
#53798=( BOUNDED_CURVE ( )  B_SPLINE_CURVE ( 3, ( #41788, #41120, #56092, #62083 ),
 .UNSPECIFIED., .F., .F. ) 
 B_SPLINE_CURVE_WITH_KNOTS ( ( 4, 4 ),
 ( 1.491236873172884225, 1.527413679725934559 ),
 .UNSPECIFIED. ) 
 CURVE ( )  GEOMETRIC_REPRESENTATION_ITEM ( )  RATIONAL_B_SPLINE_CURVE ( ( 1.000000000000000000, 0.9998909395293115177, 0.9998909395293115177, 1.000000000000000000 ) ) 
 REPRESENTATION_ITEM ( '' )  );
#53799=CARTESIAN_POINT ( 'NONE',  ( -35.00000000000000000, -0.06441628369844946966, 12.18632975068352842 ) ) ;
#53802=CYLINDRICAL_SURFACE ( 'NONE', #61839, 4.999999999999999112 ) ;
#53803=CARTESIAN_POINT ( 'NONE',  ( 35.00000000000000000, 5.672855678558685888, -10.28547182238010116 ) ) ;
#53805=VERTEX_POINT ( 'NONE', #25269 ) ;
#53806=ORIENTED_EDGE ( 'NONE', *, *, #56212, .T. ) ;
#53807=CARTESIAN_POINT ( 'NONE',  ( -17.63946288578489430, -7.321399697264532769, -9.512743050931277367 ) ) ;
#53812=EDGE_CURVE ( 'NONE', #22263, #26214, #48176, .T. ) ;
#53813=CARTESIAN_POINT ( 'NONE',  ( 35.00000000000000000, 7.817492529713852889, -9.348667969174437431 ) ) ;
#53818=ORIENTED_EDGE ( 'NONE', *, *, #65123, .F. ) ;
#53819=VERTEX_POINT ( 'NONE', #61184 ) ;
#53820=CARTESIAN_POINT ( 'NONE',  ( -37.00000000000000711, 4.545979934229579023, -11.30684963584384306 ) ) ;
#53822=CARTESIAN_POINT ( 'NONE',  ( 37.00000000000000711, 4.705694406421931860E-17, -3.469127814946512892E-15 ) ) ;
#53823=EDGE_CURVE ( 'NONE', #33456, #10138, #9934, .T. ) ;
#53824=VERTEX_POINT ( 'NONE', #56182 ) ;
#53825=VECTOR ( 'NONE', #41614, 1000.000000000000000 ) ;
#53828=DIRECTION ( 'NONE',  ( 0.000000000000000000, -0.01356324068817992175, 0.9999080150203990547 ) ) ;
#53830=CARTESIAN_POINT ( 'NONE',  ( -47.00000000000000711, 0.000000000000000000, 0.000000000000000000 ) ) ;
#53832=EDGE_CURVE ( 'NONE', #24551, #43237, #60919, .T. ) ;
#53834=DIRECTION ( 'NONE',  ( 0.000000000000000000, -0.5987040770935737610, 0.8009703041134123014 ) ) ;
#53836=CARTESIAN_POINT ( 'NONE',  ( -37.00000000000000711, -12.49688848680886011, 2.527899948230591942 ) ) ;
#53837=CYLINDRICAL_SURFACE ( 'NONE', #8932, 5.000000000000000888 ) ;
#53838=DIRECTION ( 'NONE',  ( 1.000000000000000000, 0.000000000000000000, 0.000000000000000000 ) ) ;
#53839=EDGE_CURVE ( 'NONE', #8090, #10925, #7808, .T. ) ;
#53840=DIRECTION ( 'NONE',  ( -1.000000000000000000, 0.000000000000000000, 0.000000000000000000 ) ) ;
#53841=DIRECTION ( 'NONE',  ( 1.000000000000000000, 0.000000000000000000, 0.000000000000000000 ) ) ;
#53843=DIRECTION ( 'NONE',  ( -1.000000000000000000, 0.000000000000000000, 0.000000000000000000 ) ) ;
#53845=DIRECTION ( 'NONE',  ( 1.000000000000000000, 0.000000000000000000, 0.000000000000000000 ) ) ;
#53846=ORIENTED_EDGE ( 'NONE', *, *, #38489, .T. ) ;
#53849=CARTESIAN_POINT ( 'NONE',  ( 35.00000000000000000, -11.74226168163341555, -0.3025107581130825896 ) ) ;
#53851=DIRECTION ( 'NONE',  ( 0.000000000000000000, 0.01356324068817998940, -0.9999080150203989437 ) ) ;
#53854=VERTEX_POINT ( 'NONE', #50239 ) ;
#53855=DIRECTION ( 'NONE',  ( 0.000000000000000000, -0.01356324068817992175, 0.9999080150203990547 ) ) ;
#53857=DIRECTION ( 'NONE',  ( 1.000000000000000000, 0.000000000000000000, -0.000000000000000000 ) ) ;
#53859=EDGE_CURVE ( 'NONE', #37516, #23486, #19489, .T. ) ;
#53862=CIRCLE ( 'NONE', #25172, 5.000000000000000888 ) ;
#53865=EDGE_CURVE ( 'NONE', #3409, #26770, #26920, .T. ) ;
#53867=CARTESIAN_POINT ( 'NONE',  ( -16.98800322446194855, 2.922502605998049674, 25.00000000000000000 ) ) ;
#53868=CIRCLE ( 'NONE', #26237, 5.000000000000000000 ) ;
#53869=ORIENTED_EDGE ( 'NONE', *, *, #29896, .T. ) ;
#53870=CIRCLE ( 'NONE', #19916, 5.000000000000000000 ) ;
#53871=ORIENTED_EDGE ( 'NONE', *, *, #46571, .T. ) ;
#53872=DIRECTION ( 'NONE',  ( -0.000000000000000000, -0.000000000000000000, -1.000000000000000000 ) ) ;
#53873=ORIENTED_EDGE ( 'NONE', *, *, #58267, .T. ) ;
#53874=DIRECTION ( 'NONE',  ( 1.000000000000000000, 0.000000000000000000, 0.000000000000000000 ) ) ;
#53875=CARTESIAN_POINT ( 'NONE',  ( 37.00000000000000711, 11.16627499335655216, 3.645068577060061266 ) ) ;
#53879=VERTEX_POINT ( 'NONE', #21933 ) ;
#53880=VERTEX_POINT ( 'NONE', #17608 ) ;
#53884=CARTESIAN_POINT ( 'NONE',  ( 35.00000000000000000, 12.14284015767851166, 1.030638227056429157 ) ) ;
#53885=ADVANCED_FACE ( 'NONE', ( #16937 ), #57518, .T. ) ;
#53887=DIRECTION ( 'NONE',  ( 0.000000000000000000, -0.01356324068817999287, 0.9999080150203990547 ) ) ;
#53895=ORIENTED_EDGE ( 'NONE', *, *, #18166, .T. ) ;
#53896=DIRECTION ( 'NONE',  ( 1.000000000000000000, 0.000000000000000000, -0.000000000000000000 ) ) ;
#53898=SURFACE_STYLE_USAGE ( .BOTH. , #23974 ) ;
#53899=VERTEX_POINT ( 'NONE', #46538 ) ;
#53900=EDGE_CURVE ( 'NONE', #49500, #43816, #12268, .T. ) ;
#53903=DIRECTION ( 'NONE',  ( -1.000000000000000000, 0.000000000000000000, 0.000000000000000000 ) ) ;
#53905=CARTESIAN_POINT ( 'NONE',  ( -35.00000000000000000, -11.53507381115581687, -2.216820770815207897 ) ) ;
#53907=DIRECTION ( 'NONE',  ( 0.000000000000000000, -0.01356324068817991828, 0.9999080150203990547 ) ) ;
#53908=EDGE_LOOP ( 'NONE', ( #4499, #64457, #41961, #60668 ) ) ;
#53909=LINE ( 'NONE', #13335, #42821 ) ;
#53911=DIRECTION ( 'NONE',  ( 0.3771207168306929813, -0.000000000000000000, 0.9261641133930337277 ) ) ;
#53914=ORIENTED_EDGE ( 'NONE', *, *, #25476, .F. ) ;
#53920=EDGE_CURVE ( 'NONE', #32028, #43145, #39797, .T. ) ;
#53922=VERTEX_POINT ( 'NONE', #6967 ) ;
#53925=VERTEX_POINT ( 'NONE', #21613 ) ;
#53926=LINE ( 'NONE', #19000, #35950 ) ;
#53927=DIRECTION ( 'NONE',  ( -1.000000000000000000, 0.000000000000000000, 0.000000000000000000 ) ) ;
#53929=CARTESIAN_POINT ( 'NONE',  ( -35.00000000000000000, 6.711949091238296639, -10.84030624090599559 ) ) ;
#53930=DIRECTION ( 'NONE',  ( 0.000000000000000000, 0.2355298848897516562, 0.9718671068226459875 ) ) ;
#53931=VERTEX_POINT ( 'NONE', #6317 ) ;
#53932=CYLINDRICAL_SURFACE ( 'NONE', #24267, 12.18649999999999878 ) ;
#53934=EDGE_CURVE ( 'NONE', #41081, #58777, #7273, .T. ) ;
#53937=DIRECTION ( 'NONE',  ( -1.000000000000000000, -0.000000000000000000, 0.000000000000000000 ) ) ;
#53938=DIRECTION ( 'NONE',  ( -1.000000000000000000, -1.836970198721029688E-16, -0.000000000000000000 ) ) ;
#53940=CARTESIAN_POINT ( 'NONE',  ( 3.663374565622874890, -11.05180360393428884, -4.676830153586281291 ) ) ;
#53942=AXIS2_PLACEMENT_3D ( 'NONE', #41525, #16606, #22828 ) ;
#53943=VERTEX_POINT ( 'NONE', #62165 ) ;
#53944=CARTESIAN_POINT ( 'NONE',  ( 12.91062684683197936, -10.80902803636823251, -5.215964072882972147 ) ) ;
#53945=CIRCLE ( 'NONE', #27399, 4.999999999999999112 ) ;
#53946=ORIENTED_EDGE ( 'NONE', *, *, #56721, .F. ) ;
#53952=CARTESIAN_POINT ( 'NONE',  ( 22.78386511336923093, 3.290201280387628824, -13.09362067330721757 ) ) ;
#53954=VERTEX_POINT ( 'NONE', #17271 ) ;
#53955=VERTEX_POINT ( 'NONE', #42506 ) ;
#53956=CARTESIAN_POINT ( 'NONE',  ( 29.71064890353178711, -9.099148391133041969, 9.982812328254121681 ) ) ;
#53958=ORIENTED_EDGE ( 'NONE', *, *, #8774, .F. ) ;
#53959=DIRECTION ( 'NONE',  ( -1.000000000000000000, 0.000000000000000000, 0.000000000000000000 ) ) ;
#53960=CARTESIAN_POINT ( 'NONE',  ( 3.916028893512121467, 5.727067861402937332, 12.22698748357986531 ) ) ;
#53961=CARTESIAN_POINT ( 'NONE',  ( 35.00000000000000000, -8.295159312811920316, -8.927548052240867449 ) ) ;
#53963=EDGE_CURVE ( 'NONE', #44463, #13725, #21264, .T. ) ;
#53964=ORIENTED_EDGE ( 'NONE', *, *, #41196, .F. ) ;
#53965=DIRECTION ( 'NONE',  ( 0.000000000000000000, -0.6478160128811839558, 0.7617968321374970486 ) ) ;
#53969=ORIENTED_EDGE ( 'NONE', *, *, #6342, .T. ) ;
#53972=DIRECTION ( 'NONE',  ( 0.000000000000000000, -0.8696919319575238116, -0.4935949184179166949 ) ) ;
#53973=ORIENTED_EDGE ( 'NONE', *, *, #7077, .F. ) ;
#53974=DIRECTION ( 'NONE',  ( 0.000000000000000000, -0.01356324068817999114, 0.9999080150203989437 ) ) ;
#53975=DIRECTION ( 'NONE',  ( 0.000000000000000000, -0.9105187689795998240, 0.4134677391718418193 ) ) ;
#53976=DIRECTION ( 'NONE',  ( 1.000000000000000000, 0.000000000000000000, 0.000000000000000000 ) ) ;
#53978=EDGE_CURVE ( 'NONE', #23142, #43264, #10990, .T. ) ;
#53980=CARTESIAN_POINT ( 'NONE',  ( -37.00000000000000711, 11.70009620280411688, 1.039216533672945753 ) ) ;
#53982=ORIENTED_EDGE ( 'NONE', *, *, #52599, .F. ) ;
#53984=DIRECTION ( 'NONE',  ( 1.000000000000000000, 0.000000000000000000, 0.000000000000000000 ) ) ;
#53989=FACE_OUTER_BOUND ( 'NONE', #23898, .T. ) ;
#53990=CARTESIAN_POINT ( 'NONE',  ( -35.00000000000000000, -12.60630747491664572, 1.908798535168333643 ) ) ;
#53993=EDGE_CURVE ( 'NONE', #40032, #22062, #24801, .T. ) ;
#53995=DIRECTION ( 'NONE',  ( -1.000000000000000000, -0.000000000000000000, 0.000000000000000000 ) ) ;
#53996=LINE ( 'NONE', #49027, #31247 ) ;
#53997=VECTOR ( 'NONE', #51163, 1000.000000000000000 ) ;
#53998=VECTOR ( 'NONE', #54714, 1000.000000000000000 ) ;
#53999=( BOUNDED_CURVE ( )  B_SPLINE_CURVE ( 3, ( #29338, #34953, #8743, #13705 ),
 .UNSPECIFIED., .F., .F. ) 
 B_SPLINE_CURVE_WITH_KNOTS ( ( 4, 4 ),
 ( 5.154908875633210208, 5.200862432538539082 ),
 .UNSPECIFIED. ) 
 CURVE ( )  GEOMETRIC_REPRESENTATION_ITEM ( )  RATIONAL_B_SPLINE_CURVE ( ( 1.000000000000000000, 0.9998240302925252010, 0.9998240302925252010, 1.000000000000000000 ) ) 
 REPRESENTATION_ITEM ( '' )  );
#54001=CARTESIAN_POINT ( 'NONE',  ( 37.00000000000000711, 2.544412758415841136, -11.91791701451267471 ) ) ;
#54003=AXIS2_PLACEMENT_3D ( 'NONE', #29289, #45549, #29595 ) ;
#54005=CIRCLE ( 'NONE', #20005, 5.000000000000000888 ) ;
#54007=CARTESIAN_POINT ( 'NONE',  ( -17.71317172853720479, -11.35466418304648251, 3.882258812239222312 ) ) ;
#54009=DIRECTION ( 'NONE',  ( -1.000000000000000000, 0.000000000000000000, 0.000000000000000000 ) ) ;
#54010=CARTESIAN_POINT ( 'NONE',  ( -8.245440395195840821, -2.472445095731639508, 13.27222751525900435 ) ) ;
#54012=CARTESIAN_POINT ( 'NONE',  ( -37.00000000000000711, 6.018036132182325026, -11.24036214326513949 ) ) ;
#54014=DIRECTION ( 'NONE',  ( 0.000000000000000000, -0.01356324068817992175, 0.9999080150203990547 ) ) ;
#54015=ADVANCED_FACE ( 'NONE', ( #48846 ), #8587, .T. ) ;
#54017=CARTESIAN_POINT ( 'NONE',  ( -27.45775109278350712, 13.35262336282554152, -1.989333891161978674 ) ) ;
#54019=VERTEX_POINT ( 'NONE', #58162 ) ;
#54020=AXIS2_PLACEMENT_3D ( 'NONE', #1156, #1504, #52366 ) ;
#54021=CARTESIAN_POINT ( 'NONE',  ( -17.16525335255839835, 3.058555645758342934, 13.14970181877596822 ) ) ;
#54022=CYLINDRICAL_SURFACE ( 'NONE', #25781, 4.999999999999999112 ) ;
#54023=CARTESIAN_POINT ( 'NONE',  ( 35.00000000000000000, 6.946017217730082294, 10.01317267707878500 ) ) ;
#54027=VERTEX_POINT ( 'NONE', #29210 ) ;
#54029=FACE_OUTER_BOUND ( 'NONE', #50549, .T. ) ;
#54030=CIRCLE ( 'NONE', #39161, 5.000000000000001776 ) ;
#54031=ORIENTED_EDGE ( 'NONE', *, *, #1671, .F. ) ;
#54032=DIRECTION ( 'NONE',  ( -0.000000000000000000, -1.000000000000000000, -0.000000000000000000 ) ) ;
#54034=VECTOR ( 'NONE', #63557, 1000.000000000000000 ) ;
#54036=COLOUR_RGB ( '', 0.72549020, 0.75294118, 0.79215686) ;
#54040=CARTESIAN_POINT ( 'NONE',  ( -18.08686583997218378, 5.151216734910788908, 25.00000000000000000 ) ) ;
#54042=AXIS2_PLACEMENT_3D ( 'NONE', #58498, #12930, #53521 ) ;
#54045=DIRECTION ( 'NONE',  ( -1.000000000000000000, 0.000000000000000000, -0.000000000000000000 ) ) ;
#54046=EDGE_LOOP ( 'NONE', ( #23553, #37295, #21245, #53106 ) ) ;
#54050=ORIENTED_EDGE ( 'NONE', *, *, #50377, .F. ) ;
#54051=CARTESIAN_POINT ( 'NONE',  ( 37.00000000000000711, -2.627174906296994905, -11.44858830469739530 ) ) ;
#54053=LINE ( 'NONE', #44072, #10960 ) ;
#54054=EDGE_CURVE ( 'NONE', #37251, #15685, #38860, .T. ) ;
#54055=CARTESIAN_POINT ( 'NONE',  ( 23.76437454561591522, 1.692121138565719107, 11.88453119584711182 ) ) ;
#54056=CARTESIAN_POINT ( 'NONE',  ( 35.00000000000000000, 4.705694406421931860E-17, -3.469127814946512892E-15 ) ) ;
#54057=DIRECTION ( 'NONE',  ( 0.000000000000000000, 0.1740410799127543318, 0.9847383929261630531 ) ) ;
#54059=DIRECTION ( 'NONE',  ( 0.000000000000000000, 0.01356324068817992175, -0.9999080150203990547 ) ) ;
#54061=LINE ( 'NONE', #8834, #16768 ) ;
#54062=CARTESIAN_POINT ( 'NONE',  ( 35.00000000000000000, 4.705694406421931860E-17, -3.469127814946512892E-15 ) ) ;
#54066=DIRECTION ( 'NONE',  ( 0.000000000000000000, 0.01356324068817998940, -0.9999080150203990547 ) ) ;
#54069=CARTESIAN_POINT ( 'NONE',  ( 29.19808783025697352, 7.805332973316867040, 11.01506521398891891 ) ) ;
#54070=DIRECTION ( 'NONE',  ( -1.000000000000000000, 0.000000000000000000, -0.000000000000000000 ) ) ;
#54072=CIRCLE ( 'NONE', #40236, 12.18650000000000055 ) ;
#54073=EDGE_CURVE ( 'NONE', #4699, #416, #38613, .T. ) ;
#54074=LINE ( 'NONE', #48447, #30153 ) ;
#54075=ORIENTED_EDGE ( 'NONE', *, *, #42094, .F. ) ;
#54076=ORIENTED_EDGE ( 'NONE', *, *, #10824, .T. ) ;
#54078=CARTESIAN_POINT ( 'NONE',  ( -37.00000000000000711, 0.000000000000000000, 0.000000000000000000 ) ) ;
#54079=DIRECTION ( 'NONE',  ( -1.000000000000000000, -0.000000000000000000, 0.000000000000000000 ) ) ;
#54080=VECTOR ( 'NONE', #13523, 1000.000000000000000 ) ;
#54082=DIRECTION ( 'NONE',  ( -1.000000000000000000, 0.000000000000000000, 0.000000000000000000 ) ) ;
#54084=CARTESIAN_POINT ( 'NONE',  ( 4.231238796982053962, -10.86860989014256518, -8.012325656740021174 ) ) ;
#54087=DIRECTION ( 'NONE',  ( 0.000000000000000000, 0.01356324068817998940, -0.9999080150203990547 ) ) ;
#54093=EDGE_CURVE ( 'NONE', #34672, #35595, #40689, .T. ) ;
#54095=CARTESIAN_POINT ( 'NONE',  ( -17.71314213125380377, -12.92974920937838057, 3.882255733911256890 ) ) ;
#54098=CYLINDRICAL_SURFACE ( 'NONE', #29057, 4.999999999999999112 ) ;
#54100=VERTEX_POINT ( 'NONE', #64125 ) ;
#54102=LINE ( 'NONE', #8541, #10822 ) ;
#54103=CYLINDRICAL_SURFACE ( 'NONE', #25399, 6.342778212674966554 ) ;
#54105=CARTESIAN_POINT ( 'NONE',  ( -14.29135464769095520, 7.782112657557433089, 9.134479874907178498 ) ) ;
#54106=CIRCLE ( 'NONE', #17994, 5.000000000000001776 ) ;
#54107=ADVANCED_FACE ( 'NONE', ( #54488 ), #18903, .T. ) ;
#54108=DIRECTION ( 'NONE',  ( 0.000000000000000000, 0.01356324068818000328, -0.9999080150203990547 ) ) ;
#54114=AXIS2_PLACEMENT_3D ( 'NONE', #23410, #29685, #54342 ) ;
#54117=DIRECTION ( 'NONE',  ( 0.000000000000000000, 0.9970832820307041766, 0.07632122047556146038 ) ) ;
#54118=DIRECTION ( 'NONE',  ( 0.000000000000000000, 0.01356324068817998940, -0.9999080150203990547 ) ) ;
#54120=EDGE_CURVE ( 'NONE', #32235, #39817, #3643, .T. ) ;
#54121=ORIENTED_EDGE ( 'NONE', *, *, #15182, .F. ) ;
#54123=EDGE_LOOP ( 'NONE', ( #12320, #50727, #18302, #26512 ) ) ;
#54126=CARTESIAN_POINT ( 'NONE',  ( -37.00000000000000711, -11.13736569743278082, 4.946702696913133579 ) ) ;
#54127=AXIS2_PLACEMENT_3D ( 'NONE', #29560, #49867, #60482 ) ;
#54131=AXIS2_PLACEMENT_3D ( 'NONE', #60640, #65608, #25391 ) ;
#54132=VERTEX_POINT ( 'NONE', #53171 ) ;
#54133=CARTESIAN_POINT ( 'NONE',  ( -35.00000000000000000, 0.000000000000000000, 0.000000000000000000 ) ) ;
#54137=VERTEX_POINT ( 'NONE', #45150 ) ;
#54138=ORIENTED_EDGE ( 'NONE', *, *, #45922, .T. ) ;
#54139=CARTESIAN_POINT ( 'NONE',  ( -37.00000000000000711, -11.72195762423409349, -0.7536123767499773862 ) ) ;
#54140=DIRECTION ( 'NONE',  ( 0.000000000000000000, -0.01356324068817991828, 0.9999080150203990547 ) ) ;
#54144=DIRECTION ( 'NONE',  ( 0.000000000000000000, -0.01356324068817991828, 0.9999080150203990547 ) ) ;
#54145=DIRECTION ( 'NONE',  ( 1.000000000000000000, 0.000000000000000000, -0.000000000000000000 ) ) ;
#54147=DIRECTION ( 'NONE',  ( -1.000000000000000000, -0.000000000000000000, 0.000000000000000000 ) ) ;
#54149=ADVANCED_FACE ( 'NONE', ( #49814 ), #4263, .T. ) ;
#54151=VERTEX_POINT ( 'NONE', #20538 ) ;
#54154=EDGE_CURVE ( 'NONE', #27489, #61832, #35460, .T. ) ;
#54155=B_SPLINE_CURVE_WITH_KNOTS ( 'NONE', 3,
 ( #40299, #60592, #49093, #50636, #60933, #55938, #16364, #51943, #36636, #1408, #26015, #16677, #12337, #12012, #32602, #5749, #16010, #26654 ),
 .UNSPECIFIED., .F., .F.,
 ( 4, 2, 2, 2, 2, 2, 2, 2, 4 ),
 ( 4.168589959160076653E-21, 0.0008349329933307835482, 0.001669865986661567096, 0.002504798979992350644, 0.003339731973323134193, 0.004174664966653918174, 0.005009597959984701289, 0.005844530953315485271, 0.006679463946646270120 ),
 .UNSPECIFIED. ) ;
#54156=CARTESIAN_POINT ( 'NONE',  ( 35.00000000000000000, 0.7214809346830272085, 11.72397916322010936 ) ) ;
#54157=CARTESIAN_POINT ( 'NONE',  ( -17.83419946441818027, -9.720786832536937538, 25.00000000000000000 ) ) ;
#54158=DIRECTION ( 'NONE',  ( 0.000000000000000000, 0.01356324068817998940, -0.9999080150203990547 ) ) ;
#54159=CARTESIAN_POINT ( 'NONE',  ( -47.00000000000000711, 0.000000000000000000, 0.000000000000000000 ) ) ;
#54161=DIRECTION ( 'NONE',  ( -1.000000000000000000, 0.000000000000000000, 0.000000000000000000 ) ) ;
#54162=CARTESIAN_POINT ( 'NONE',  ( -4.984431264850669230, -1.083143072858139710, 11.95218935805936056 ) ) ;
#54165=ORIENTED_EDGE ( 'NONE', *, *, #34680, .T. ) ;
#54166=CARTESIAN_POINT ( 'NONE',  ( -18.35310563997612476, 6.398290920003422144, -10.15549306850661004 ) ) ;
#54167=VERTEX_POINT ( 'NONE', #54811 ) ;
#54168=LINE ( 'NONE', #7979, #13660 ) ;
#54174=DIRECTION ( 'NONE',  ( 1.000000000000000000, 0.000000000000000000, 0.000000000000000000 ) ) ;
#54175=CARTESIAN_POINT ( 'NONE',  ( -35.00000000000000000, 0.000000000000000000, 0.000000000000000000 ) ) ;
#54178=EDGE_CURVE ( 'NONE', #11339, #23831, #14225, .T. ) ;
#54179=EDGE_CURVE ( 'NONE', #60445, #153, #21559, .T. ) ;
#54180=AXIS2_PLACEMENT_3D ( 'NONE', #21574, #46191, #20894 ) ;
#54183=ORIENTED_EDGE ( 'NONE', *, *, #47064, .T. ) ;
#54184=DIRECTION ( 'NONE',  ( 0.000000000000000000, 0.9105187689795969375, -0.4134677391718481476 ) ) ;
#54185=VERTEX_POINT ( 'NONE', #44811 ) ;
#54186=CARTESIAN_POINT ( 'NONE',  ( -37.00000000000000711, 0.000000000000000000, 0.000000000000000000 ) ) ;
#54187=CARTESIAN_POINT ( 'NONE',  ( 3.455388140186510970, 8.284410676190361755, -8.681632586536968788 ) ) ;
#54189=AXIS2_PLACEMENT_3D ( 'NONE', #51775, #47118, #6219 ) ;
#54190=DIRECTION ( 'NONE',  ( 1.000000000000000000, -0.000000000000000000, 0.000000000000000000 ) ) ;
#54192=EDGE_CURVE ( 'NONE', #42378, #7123, #50793, .T. ) ;
#54193=ORIENTED_EDGE ( 'NONE', *, *, #23587, .T. ) ;
#54194=EDGE_LOOP ( 'NONE', ( #24046, #60405, #61687, #44368 ) ) ;
#54195=CARTESIAN_POINT ( 'NONE',  ( -37.00000000000000711, 12.08151691381195825, -4.074242145635881052 ) ) ;
#54196=CIRCLE ( 'NONE', #19319, 12.74999999999999822 ) ;
#54202=VERTEX_POINT ( 'NONE', #55454 ) ;
#54203=EDGE_CURVE ( 'NONE', #27200, #51547, #10218, .T. ) ;
#54204=ORIENTED_EDGE ( 'NONE', *, *, #23895, .T. ) ;
#54205=EDGE_LOOP ( 'NONE', ( #65013, #26564, #60471, #29527 ) ) ;
#54206=DIRECTION ( 'NONE',  ( -1.000000000000000000, -0.000000000000000000, 0.000000000000000000 ) ) ;
#54209=AXIS2_PLACEMENT_3D ( 'NONE', #52380, #43269, #28641 ) ;
#54210=AXIS2_PLACEMENT_3D ( 'NONE', #1079, #62241, #61577 ) ;
#54211=CIRCLE ( 'NONE', #29778, 5.000000000000000888 ) ;
#54212=ORIENTED_EDGE ( 'NONE', *, *, #51401, .F. ) ;
#54213=DIRECTION ( 'NONE',  ( 0.000000000000000000, -0.01356324068817991828, 0.9999080150203990547 ) ) ;
#54215=ORIENTED_EDGE ( 'NONE', *, *, #27654, .T. ) ;
#54217=LINE ( 'NONE', #37610, #60486 ) ;
#54219=DIRECTION ( 'NONE',  ( 0.000000000000000000, 0.04924826701373889726, 0.9987865678893281807 ) ) ;
#54223=EDGE_CURVE ( 'NONE', #42938, #7910, #26981, .T. ) ;
#54225=FILL_AREA_STYLE ('',( #53584 ) ) ;
#54227=VERTEX_POINT ( 'NONE', #46148 ) ;
#54228=ORIENTED_EDGE ( 'NONE', *, *, #48984, .T. ) ;
#54231=CARTESIAN_POINT ( 'NONE',  ( -37.00000000000000711, -9.240395740215685549, 7.251710744571544964 ) ) ;
#54232=DIRECTION ( 'NONE',  ( 1.000000000000000000, 0.000000000000000000, 0.000000000000000000 ) ) ;
#54237=CIRCLE ( 'NONE', #3259, 12.75000000000000178 ) ;
#54239=VECTOR ( 'NONE', #49467, 1000.000000000000000 ) ;
#54240=ORIENTED_EDGE ( 'NONE', *, *, #63899, .T. ) ;
#54241=CARTESIAN_POINT ( 'NONE',  ( 22.36482863261543486, 25.00000000000000000, -0.9234811557364158707 ) ) ;
#54242=CARTESIAN_POINT ( 'NONE',  ( 35.00000000000000000, 4.705694406421931860E-17, -3.469127814946512892E-15 ) ) ;
#54243=CIRCLE ( 'NONE', #24502, 12.18649999999999878 ) ;
#54245=VERTEX_POINT ( 'NONE', #15207 ) ;
#54247=CARTESIAN_POINT ( 'NONE',  ( -15.08738464654653733, 8.458522730116888155, 8.511980925729206504 ) ) ;
#54251=ORIENTED_EDGE ( 'NONE', *, *, #56588, .F. ) ;
#54255=EDGE_LOOP ( 'NONE', ( #9957, #14710, #25834, #58469 ) ) ;
#54256=DIRECTION ( 'NONE',  ( -0.000000000000000000, -1.000000000000000000, -0.000000000000000000 ) ) ;
#54260=AXIS2_PLACEMENT_3D ( 'NONE', #15817, #51445, #50765 ) ;
#54261=CARTESIAN_POINT ( 'NONE',  ( 12.33930588725807631, 11.79251860674097685, -2.229502300750831889 ) ) ;
#54262=ORIENTED_EDGE ( 'NONE', *, *, #43619, .F. ) ;
#54264=CARTESIAN_POINT ( 'NONE',  ( 35.00000000000000000, 4.705694406421931860E-17, -3.469127814946512892E-15 ) ) ;
#54265=CIRCLE ( 'NONE', #59572, 4.999999999999999112 ) ;
#54267=AXIS2_PLACEMENT_3D ( 'NONE', #11546, #25204, #45824 ) ;
#54269=EDGE_CURVE ( 'NONE', #41991, #62732, #30497, .T. ) ;
#54271=CIRCLE ( 'NONE', #58546, 11.99999999999998757 ) ;
#54272=CARTESIAN_POINT ( 'NONE',  ( -17.22530951443547309, -6.628480137379963999, 10.00470364405594204 ) ) ;
#54273=CYLINDRICAL_SURFACE ( 'NONE', #56159, 5.000000000000000888 ) ;
#54275=CARTESIAN_POINT ( 'NONE',  ( 37.00000000000000711, -7.745827850123079727, -10.12742074351894317 ) ) ;
#54276=CARTESIAN_POINT ( 'NONE',  ( 36.00000000000000711, 0.6593684648220483613, -12.73293890771483738 ) ) ;
#54277=EDGE_CURVE ( 'NONE', #46044, #10053, #47132, .T. ) ;
#54278=AXIS2_PLACEMENT_3D ( 'NONE', #54793, #30161, #9209 ) ;
#54279=AXIS2_PLACEMENT_3D ( 'NONE', #60520, #39254, #65494 ) ;
#54280=ORIENTED_EDGE ( 'NONE', *, *, #4909, .F. ) ;
#54281=DIRECTION ( 'NONE',  ( -1.000000000000000000, 0.000000000000000000, 0.000000000000000000 ) ) ;
#54282=CIRCLE ( 'NONE', #34034, 12.75000000000000178 ) ;
#54287=CIRCLE ( 'NONE', #56401, 4.999999999999999112 ) ;
#54290=ORIENTED_EDGE ( 'NONE', *, *, #65188, .T. ) ;
#54291=EDGE_CURVE ( 'NONE', #60108, #39829, #36806, .T. ) ;
#54292=CIRCLE ( 'NONE', #24561, 5.000000000000000000 ) ;
#54294=ORIENTED_EDGE ( 'NONE', *, *, #42607, .T. ) ;
#54299=DIRECTION ( 'NONE',  ( -1.000000000000000000, -0.000000000000000000, -0.000000000000000000 ) ) ;
#54301=AXIS2_PLACEMENT_3D ( 'NONE', #49261, #60185, #8672 ) ;
#54303=ORIENTED_EDGE ( 'NONE', *, *, #16731, .F. ) ;
#54305=DIRECTION ( 'NONE',  ( 1.000000000000000000, -0.000000000000000000, -0.000000000000000000 ) ) ;
#54306=CYLINDRICAL_SURFACE ( 'NONE', #37700, 4.999999999999999112 ) ;
#54311=ORIENTED_EDGE ( 'NONE', *, *, #12080, .F. ) ;
#54313=ORIENTED_EDGE ( 'NONE', *, *, #10788, .T. ) ;
#54316=EDGE_CURVE ( 'NONE', #30274, #136, #51789, .T. ) ;
#54317=CARTESIAN_POINT ( 'NONE',  ( -35.00000000000000000, 9.700295462048664774, 7.376655759824919834 ) ) ;
#54318=CARTESIAN_POINT ( 'NONE',  ( -35.00000000000000000, 0.000000000000000000, 0.000000000000000000 ) ) ;
#54320=VECTOR ( 'NONE', #25375, 1000.000000000000000 ) ;
#54322=CARTESIAN_POINT ( 'NONE',  ( -9.169765030952540030, -3.248313620670495006, -13.10426324017876887 ) ) ;
#54323=CARTESIAN_POINT ( 'NONE',  ( 10.74559270775345432, 13.46648889917082847, -0.9568044215894803139 ) ) ;
#54324=EDGE_CURVE ( 'NONE', #35667, #60506, #46455, .T. ) ;
#54325=ORIENTED_EDGE ( 'NONE', *, *, #60242, .F. ) ;
#54326=DIRECTION ( 'NONE',  ( 1.000000000000000000, 0.000000000000000000, 0.000000000000000000 ) ) ;
#54327=VERTEX_POINT ( 'NONE', #6889 ) ;
#54330=ORIENTED_EDGE ( 'NONE', *, *, #30602, .F. ) ;
#54331=CARTESIAN_POINT ( 'NONE',  ( 22.88594695219327235, -4.822122601967141264, -12.60940655271284427 ) ) ;
#54335=CARTESIAN_POINT ( 'NONE',  ( 35.00000000000000000, -10.14433819232439049, -6.753013023069681431 ) ) ;
#54336=CIRCLE ( 'NONE', #10778, 5.000000000000000000 ) ;
#54337=AXIS2_PLACEMENT_3D ( 'NONE', #20071, #60628, #5451 ) ;
#54340=AXIS2_PLACEMENT_3D ( 'NONE', #29861, #19585, #50171 ) ;
#54341=ORIENTED_EDGE ( 'NONE', *, *, #30829, .T. ) ;
#54342=DIRECTION ( 'NONE',  ( 0.000000000000000000, -0.01356324068817998940, 0.9999080150203990547 ) ) ;
#54344=DIRECTION ( 'NONE',  ( -1.000000000000000000, 0.000000000000000000, 0.000000000000000000 ) ) ;
#54345=DIRECTION ( 'NONE',  ( 0.000000000000000000, -0.8515178078024813191, 0.5243256840888652626 ) ) ;
#54347=AXIS2_PLACEMENT_3D ( 'NONE', #11144, #25438, #42036 ) ;
#54348=ADVANCED_FACE ( 'NONE', ( #6232 ), #21857, .T. ) ;
#54349=CARTESIAN_POINT ( 'NONE',  ( -11.40165637463000259, -7.324853138339117109, 11.34220541683159489 ) ) ;
#54351=AXIS2_PLACEMENT_3D ( 'NONE', #24037, #23719, #53965 ) ;
#54352=CIRCLE ( 'NONE', #38379, 12.18649999999999878 ) ;
#54354=DIRECTION ( 'NONE',  ( 0.000000000000000000, -0.01356324068818001369, 0.9999080150203990547 ) ) ;
#54357=AXIS2_PLACEMENT_3D ( 'NONE', #31124, #61063, #45758 ) ;
#54359=AXIS2_PLACEMENT_3D ( 'NONE', #16055, #32333, #37323 ) ;
#54360=CARTESIAN_POINT ( 'NONE',  ( -25.54435311314727386, 5.747082554913779617, 10.54001105275434291 ) ) ;
#54361=DIRECTION ( 'NONE',  ( 0.000000000000000000, -0.9346839223284579834, 0.3554799084908866202 ) ) ;
#54363=CARTESIAN_POINT ( 'NONE',  ( 19.28625800530496903, 1.699513388191793428, 11.87904264843580471 ) ) ;
#54364=CARTESIAN_POINT ( 'NONE',  ( -9.838098675710270413, -10.18811004032726686, -6.355130291591023273 ) ) ;
#54365=LINE ( 'NONE', #44672, #45627 ) ;
#54366=VERTEX_POINT ( 'NONE', #26182 ) ;
#54367=CARTESIAN_POINT ( 'NONE',  ( 21.44353899438906907, 13.23503942470536643, -2.693104912682990015 ) ) ;
#54368=DIRECTION ( 'NONE',  ( 1.000000000000000000, 0.000000000000000000, 0.000000000000000000 ) ) ;
#54369=ORIENTED_EDGE ( 'NONE', *, *, #20482, .F. ) ;
#54370=EDGE_CURVE ( 'NONE', #37836, #64097, #6822, .T. ) ;
#54371=ORIENTED_EDGE ( 'NONE', *, *, #55728, .T. ) ;
#54372=DIRECTION ( 'NONE',  ( -1.000000000000000000, 0.000000000000000000, 0.000000000000000000 ) ) ;
#54373=AXIS2_PLACEMENT_3D ( 'NONE', #8964, #14267, #54530 ) ;
#54375=VECTOR ( 'NONE', #19267, 1000.000000000000000 ) ;
#54377=AXIS2_PLACEMENT_3D ( 'NONE', #22024, #56286, #42278 ) ;
#54378=DIRECTION ( 'NONE',  ( 0.000000000000000000, -0.01356324068817998940, 0.9999080150203990547 ) ) ;
#54381=CYLINDRICAL_SURFACE ( 'NONE', #4693, 12.75000000000000178 ) ;
#54384=DIRECTION ( 'NONE',  ( -1.000000000000000000, 0.000000000000000000, 0.000000000000000000 ) ) ;
#54385=ORIENTED_EDGE ( 'NONE', *, *, #57172, .T. ) ;
#54386=CARTESIAN_POINT ( 'NONE',  ( -35.00000000000000000, 8.699265615722982403, 8.534258022646129760 ) ) ;
#54387=ORIENTED_EDGE ( 'NONE', *, *, #29435, .F. ) ;
#54388=DIRECTION ( 'NONE',  ( 1.000000000000000000, 0.000000000000000000, -0.000000000000000000 ) ) ;
#54392=CARTESIAN_POINT ( 'NONE',  ( -15.91316379733282282, 8.402199048040264628, 10.56663549368182942 ) ) ;
#54394=ADVANCED_FACE ( 'NONE', ( #57421 ), #21525, .T. ) ;
#54397=FACE_OUTER_BOUND ( 'NONE', #51454, .T. ) ;
#54400=AXIS2_PLACEMENT_3D ( 'NONE', #4851, #61334, #39750 ) ;
#54404=CARTESIAN_POINT ( 'NONE',  ( 35.00000000000000000, 0.9416912585476243658, 12.71517666308946204 ) ) ;
#54405=CARTESIAN_POINT ( 'NONE',  ( -35.00000000000000000, -11.02904044024211849, 4.041347439435823752 ) ) ;
#54407=CYLINDRICAL_SURFACE ( 'NONE', #11473, 4.999999999999999112 ) ;
#54408=CIRCLE ( 'NONE', #59709, 4.999999999999999112 ) ;
#54413=AXIS2_PLACEMENT_3D ( 'NONE', #12789, #33078, #28112 ) ;
#54414=CARTESIAN_POINT ( 'NONE',  ( -37.00000000000000711, 0.000000000000000000, 0.000000000000000000 ) ) ;
#54415=CIRCLE ( 'NONE', #63976, 4.999999999999999112 ) ;
#54417=ORIENTED_EDGE ( 'NONE', *, *, #42991, .T. ) ;
#54418=VERTEX_POINT ( 'NONE', #27160 ) ;
#54422=VECTOR ( 'NONE', #46123, 1000.000000000000000 ) ;
#54423=AXIS2_PLACEMENT_3D ( 'NONE', #18560, #38812, #59111 ) ;
#54424=CYLINDRICAL_SURFACE ( 'NONE', #44041, 5.000000000000000888 ) ;
#54425=CARTESIAN_POINT ( 'NONE',  ( 35.00000000000000000, 4.705694406421931860E-17, -3.469127814946512892E-15 ) ) ;
#54426=EDGE_CURVE ( 'NONE', #50839, #21538, #57758, .T. ) ;
#54427=DIRECTION ( 'NONE',  ( -1.000000000000000000, 0.000000000000000000, -0.000000000000000000 ) ) ;
#54430=DIRECTION ( 'NONE',  ( 0.000000000000000000, -0.5767582926624851281, -0.8169148498130359703 ) ) ;
#54431=EDGE_CURVE ( 'NONE', #8244, #31482, #8893, .T. ) ;
#54432=CARTESIAN_POINT ( 'NONE',  ( 3.291290029914074378, 8.250315036047103590, 25.00000000000000000 ) ) ;
#54433=ORIENTED_EDGE ( 'NONE', *, *, #52579, .F. ) ;
#54434=DIRECTION ( 'NONE',  ( 1.000000000000000000, 0.000000000000000000, 0.000000000000000000 ) ) ;
#54435=CARTESIAN_POINT ( 'NONE',  ( 35.00000000000000000, 12.74068829017553739, 0.4871980014161889083 ) ) ;
#54436=EDGE_CURVE ( 'NONE', #34943, #2113, #36889, .T. ) ;
#54438=CIRCLE ( 'NONE', #25765, 12.18650000000000055 ) ;
#54439=CARTESIAN_POINT ( 'NONE',  ( 3.618261583105314649, 8.318251859915346103, 10.63289868894575463 ) ) ;
#54444=VERTEX_POINT ( 'NONE', #18827 ) ;
#54447=DIRECTION ( 'NONE',  ( -1.000000000000000000, 0.000000000000000000, -0.000000000000000000 ) ) ;
#54448=EDGE_CURVE ( 'NONE', #3635, #63404, #58865, .T. ) ;
#54450=AXIS2_PLACEMENT_3D ( 'NONE', #13947, #34239, #19627 ) ;
#54453=AXIS2_PLACEMENT_3D ( 'NONE', #65119, #11879, #41147 ) ;
#54454=CIRCLE ( 'NONE', #1387, 12.74999999999999822 ) ;
#54458=DIRECTION ( 'NONE',  ( 0.000000000000000000, 0.9847383929261623869, -0.1740410799127578845 ) ) ;
#54461=DIRECTION ( 'NONE',  ( 1.000000000000000000, 0.000000000000000000, 0.000000000000000000 ) ) ;
#54462=DIRECTION ( 'NONE',  ( -1.000000000000000000, 0.000000000000000000, 0.000000000000000000 ) ) ;
#54464=DIRECTION ( 'NONE',  ( 0.000000000000000000, -0.8989688749565110104, -0.4380125133594070519 ) ) ;
#54466=ORIENTED_EDGE ( 'NONE', *, *, #39087, .T. ) ;
#54468=AXIS2_PLACEMENT_3D ( 'NONE', #53875, #65773, #4311 ) ;
#54469=DIRECTION ( 'NONE',  ( 0.000000000000000000, -0.01356324068817992175, 0.9999080150203990547 ) ) ;
#54472=DIRECTION ( 'NONE',  ( -1.000000000000000000, 0.000000000000000000, 0.000000000000000000 ) ) ;
#54473=CARTESIAN_POINT ( 'NONE',  ( -37.00000000000000711, -12.16632754454237464, 0.7008968033238341944 ) ) ;
#54474=CARTESIAN_POINT ( 'NONE',  ( 24.85771399857551600, 0.06729695006813952995, 13.50545047877942650 ) ) ;
#54479=FACE_OUTER_BOUND ( 'NONE', #35337, .T. ) ;
#54480=EDGE_CURVE ( 'NONE', #46064, #55188, #38781, .T. ) ;
#54483=CARTESIAN_POINT ( 'NONE',  ( -37.00000000000000711, 0.000000000000000000, 0.000000000000000000 ) ) ;
#54484=EDGE_CURVE ( 'NONE', #28605, #50714, #767, .T. ) ;
#54487=DIRECTION ( 'NONE',  ( 0.000000000000000000, -0.01356324068817998940, 0.9999080150203990547 ) ) ;
#54488=FACE_OUTER_BOUND ( 'NONE', #50111, .T. ) ;
#54491=DIRECTION ( 'NONE',  ( -1.000000000000000000, 0.000000000000000000, 0.000000000000000000 ) ) ;
#54494=CARTESIAN_POINT ( 'NONE',  ( 29.40624810938076905, 9.599151068884586024, 7.217545767187523609 ) ) ;
#54497=DIRECTION ( 'NONE',  ( 1.000000000000000000, 0.000000000000000000, 0.000000000000000000 ) ) ;
#54499=CIRCLE ( 'NONE', #9909, 12.74999999999999822 ) ;
#54502=CARTESIAN_POINT ( 'NONE',  ( -16.08965205424928868, 8.362593759199420163, -8.606399676289541389 ) ) ;
#54503=EDGE_CURVE ( 'NONE', #63220, #36458, #54074, .T. ) ;
#54505=EDGE_CURVE ( 'NONE', #51431, #21573, #37570, .T. ) ;
#54509=CIRCLE ( 'NONE', #26865, 12.18650000000000055 ) ;
#54511=ADVANCED_FACE ( 'NONE', ( #8506 ), #33466, .T. ) ;
#54513=ORIENTED_EDGE ( 'NONE', *, *, #56223, .F. ) ;
#54514=CIRCLE ( 'NONE', #18453, 12.18650000000000233 ) ;
#54517=DIRECTION ( 'NONE',  ( 0.000000000000000000, 0.01356324068817992175, -0.9999080150203990547 ) ) ;
#54518=DIRECTION ( 'NONE',  ( -1.000000000000000000, 0.000000000000000000, 0.000000000000000000 ) ) ;
#54520=EDGE_CURVE ( 'NONE', #39152, #50397, #3215, .T. ) ;
#54523=ORIENTED_EDGE ( 'NONE', *, *, #8657, .T. ) ;
#54524=EDGE_CURVE ( 'NONE', #35057, #58885, #53755, .T. ) ;
#54526=DIRECTION ( 'NONE',  ( 0.000000000000000000, -0.01356324068817999114, 0.9999080150203989437 ) ) ;
#54527=EDGE_LOOP ( 'NONE', ( #21603, #18294, #41179, #26630 ) ) ;
#54529=DIRECTION ( 'NONE',  ( 1.000000000000000000, -0.000000000000000000, 0.000000000000000000 ) ) ;
#54530=DIRECTION ( 'NONE',  ( 0.000000000000000000, 0.01356324068817998940, -0.9999080150203990547 ) ) ;
#54532=VECTOR ( 'NONE', #32277, 1000.000000000000000 ) ;
#54538=DIRECTION ( 'NONE',  ( 1.000000000000000000, 0.000000000000000000, 0.000000000000000000 ) ) ;
#54539=CARTESIAN_POINT ( 'NONE',  ( -37.00000000000000711, -9.700295462048607931, -7.376655759824990000 ) ) ;
#54543=ORIENTED_EDGE ( 'NONE', *, *, #18987, .T. ) ;
#54544=AXIS2_PLACEMENT_3D ( 'NONE', #28842, #43811, #24500 ) ;
#54545=AXIS2_PLACEMENT_3D ( 'NONE', #57994, #1143, #26403 ) ;
#54546=ORIENTED_EDGE ( 'NONE', *, *, #41598, .F. ) ;
#54550=CARTESIAN_POINT ( 'NONE',  ( -37.00000000000000711, 11.29812557209476864, 3.213188559034282132 ) ) ;
#54551=AXIS2_PLACEMENT_3D ( 'NONE', #4899, #65059, #5559 ) ;
#54552=ORIENTED_EDGE ( 'NONE', *, *, #26494, .T. ) ;
#54553=CARTESIAN_POINT ( 'NONE',  ( -37.00000000000000711, -11.96656215839366055, -4.400442035671074947 ) ) ;
#54554=FACE_BOUND ( 'NONE', #64305, .T. ) ;
#54555=ORIENTED_EDGE ( 'NONE', *, *, #41634, .F. ) ;
#54559=ORIENTED_EDGE ( 'NONE', *, *, #46297, .T. ) ;
#54560=AXIS2_PLACEMENT_3D ( 'NONE', #51150, #30197, #10230 ) ;
#54561=ORIENTED_EDGE ( 'NONE', *, *, #11869, .F. ) ;
#54562=CARTESIAN_POINT ( 'NONE',  ( -37.00000000000000711, 5.130401251914730842, 11.05394794832831629 ) ) ;
#54563=ORIENTED_EDGE ( 'NONE', *, *, #64112, .F. ) ;
#54564=DIRECTION ( 'NONE',  ( -0.000000000000000000, -0.000000000000000000, -1.000000000000000000 ) ) ;
#54565=ORIENTED_EDGE ( 'NONE', *, *, #58899, .F. ) ;
#54566=VECTOR ( 'NONE', #31109, 1000.000000000000000 ) ;
#54567=ORIENTED_EDGE ( 'NONE', *, *, #52565, .F. ) ;
#54568=VERTEX_POINT ( 'NONE', #12499 ) ;
#54569=DIRECTION ( 'NONE',  ( -0.000000000000000000, -1.000000000000000000, -0.000000000000000000 ) ) ;
#54570=AXIS2_PLACEMENT_3D ( 'NONE', #7838, #12153, #27774 ) ;
#54571=DIRECTION ( 'NONE',  ( 0.000000000000000000, 0.8169148498130297531, -0.5767582926624940098 ) ) ;
#54572=EDGE_CURVE ( 'NONE', #58025, #29486, #53084, .T. ) ;
#54573=FACE_OUTER_BOUND ( 'NONE', #20670, .T. ) ;
#54574=DIRECTION ( 'NONE',  ( 0.000000000000000000, 0.01356324068817998940, -0.9999080150203990547 ) ) ;
#54575=DIRECTION ( 'NONE',  ( -1.000000000000000000, -1.836970198721029688E-16, 0.000000000000000000 ) ) ;
#54578=CIRCLE ( 'NONE', #37566, 5.000000000000000888 ) ;
#54579=EDGE_LOOP ( 'NONE', ( #60926, #13152, #573, #65589 ) ) ;
#54580=DIRECTION ( 'NONE',  ( 0.000000000000000000, -1.000000000000000000, 0.000000000000000000 ) ) ;
#54582=FACE_OUTER_BOUND ( 'NONE', #36963, .T. ) ;
#54583=VERTEX_POINT ( 'NONE', #48117 ) ;
#54584=EDGE_CURVE ( 'NONE', #12670, #10959, #2573, .T. ) ;
#54585=CARTESIAN_POINT ( 'NONE',  ( -15.23449087116190093, 8.463651061413711929, 8.506858964723610583 ) ) ;
#54587=DIRECTION ( 'NONE',  ( 0.000000000000000000, -0.01356324068817998940, 0.9999080150203990547 ) ) ;
#54588=ORIENTED_EDGE ( 'NONE', *, *, #35425, .T. ) ;
#54589=CIRCLE ( 'NONE', #25900, 5.000000000000000888 ) ;
#54590=ADVANCED_FACE ( 'NONE', ( #35409 ), #5174, .T. ) ;
#54591=ORIENTED_EDGE ( 'NONE', *, *, #29620, .T. ) ;
#54597=CARTESIAN_POINT ( 'NONE',  ( 35.00000000000000000, -8.624332853795991127, 9.390600770288079602 ) ) ;
#54599=ADVANCED_FACE ( 'NONE', ( #14782 ), #49436, .T. ) ;
#54600=CARTESIAN_POINT ( 'NONE',  ( -19.62351202312758502, -4.052328796303131142, -12.87840960595547557 ) ) ;
#54601=VERTEX_POINT ( 'NONE', #59717 ) ;
#54602=CIRCLE ( 'NONE', #9956, 12.18650000000000055 ) ;
#54605=CARTESIAN_POINT ( 'NONE',  ( -37.00000000000000711, 1.738225594539996477, 12.63095688309029718 ) ) ;
#54610=VECTOR ( 'NONE', #64370, 1000.000000000000000 ) ;
#54612=PRODUCT ( 'tweezer drum assembly', 'tweezer drum assembly', '', ( #57746 ) ) ;
#54613=ADVANCED_FACE ( 'NONE', ( #65345 ), #55373, .T. ) ;
#54614=CARTESIAN_POINT ( 'NONE',  ( 37.00000000000000711, 4.705694406421931860E-17, -3.469127814946512892E-15 ) ) ;
#54615=DIRECTION ( 'NONE',  ( 0.000000000000000000, 0.2355298848897446895, 0.9718671068226476528 ) ) ;
#54616=DIRECTION ( 'NONE',  ( -0.000000000000000000, -1.000000000000000000, -0.000000000000000000 ) ) ;
#54617=CIRCLE ( 'NONE', #25935, 5.000000000000000000 ) ;
#54618=EDGE_CURVE ( 'NONE', #40555, #34975, #42873, .T. ) ;
#54619=AXIS2_PLACEMENT_3D ( 'NONE', #27362, #47347, #52969 ) ;
#54620=ORIENTED_EDGE ( 'NONE', *, *, #38646, .T. ) ;
#54623=ORIENTED_EDGE ( 'NONE', *, *, #24742, .T. ) ;
#54624=CARTESIAN_POINT ( 'NONE',  ( -35.00000000000000000, 0.000000000000000000, 0.000000000000000000 ) ) ;
#54626=CARTESIAN_POINT ( 'NONE',  ( -37.00000000000000711, 11.95840593935201390, 2.346765782874478123 ) ) ;
#54627=AXIS2_PLACEMENT_3D ( 'NONE', #24781, #30412, #5155 ) ;
#54628=EDGE_CURVE ( 'NONE', #38600, #27683, #39693, .T. ) ;
#54631=ORIENTED_EDGE ( 'NONE', *, *, #44726, .T. ) ;
#54634=CIRCLE ( 'NONE', #5788, 12.75000000000000178 ) ;
#54635=VERTEX_POINT ( 'NONE', #15129 ) ;
#54637=CARTESIAN_POINT ( 'NONE',  ( 35.00000000000000000, 2.544412758415841580, -11.91791701451267471 ) ) ;
#54639=CARTESIAN_POINT ( 'NONE',  ( 35.00000000000000000, 4.705694406421931860E-17, -3.469127814946512892E-15 ) ) ;
#54640=VERTEX_POINT ( 'NONE', #45078 ) ;
#54643=CARTESIAN_POINT ( 'NONE',  ( 35.00000000000000000, 11.91791701451269780, 2.544412758415707909 ) ) ;
#54644=DIRECTION ( 'NONE',  ( 1.000000000000000000, -0.000000000000000000, 0.000000000000000000 ) ) ;
#54646=FACE_OUTER_BOUND ( 'NONE', #36281, .T. ) ;
#54647=ORIENTED_EDGE ( 'NONE', *, *, #28978, .T. ) ;
#54648=VECTOR ( 'NONE', #55337, 1000.000000000000000 ) ;
#54649=CARTESIAN_POINT ( 'NONE',  ( -29.76537318338597871, -3.714251817591057492, -11.41077529405955637 ) ) ;
#54651=CARTESIAN_POINT ( 'NONE',  ( -29.57682744818767162, 0.08430219135412277132, -12.00160382718744323 ) ) ;
#54653=DIRECTION ( 'NONE',  ( 0.000000000000000000, 0.7196168960969817618, 0.6943713148249616163 ) ) ;
#54655=EDGE_CURVE ( 'NONE', #23486, #31809, #34739, .T. ) ;
#54657=CARTESIAN_POINT ( 'NONE',  ( -6.584448747071861341, -1.675181234638447814, -13.39582994125472482 ) ) ;
#54659=CARTESIAN_POINT ( 'NONE',  ( 11.84688083938066150, 13.39238687512208870, -1.708653298068749438 ) ) ;
#54661=ORIENTED_EDGE ( 'NONE', *, *, #22214, .T. ) ;
#54662=CARTESIAN_POINT ( 'NONE',  ( 37.00000000000000711, 2.772148766916279872, 11.86701198550352920 ) ) ;
#54667=CARTESIAN_POINT ( 'NONE',  ( 35.00000000000000000, 4.705694406421931860E-17, -3.469127814946512892E-15 ) ) ;
#54671=CIRCLE ( 'NONE', #61008, 5.000000000000001776 ) ;
#54673=LINE ( 'NONE', #4108, #40672 ) ;
#54676=CARTESIAN_POINT ( 'NONE',  ( 37.00000000000000711, -10.63508530065518443, 4.986700593229810963 ) ) ;
#54677=CARTESIAN_POINT ( 'NONE',  ( -17.55783715699735836, -5.649761354908354960, 12.26190536833593292 ) ) ;
#54678=EDGE_CURVE ( 'NONE', #61909, #57845, #11543, .T. ) ;
#54679=VERTEX_POINT ( 'NONE', #8395 ) ;
#54681=DIRECTION ( 'NONE',  ( 0.000000000000000000, 0.01356324068817992175, -0.9999080150203990547 ) ) ;
#54685=PLANE ( 'NONE',  #38582 ) ;
#54687=ADVANCED_FACE ( 'NONE', ( #13060 ), #13379, .T. ) ;
#54688=FACE_OUTER_BOUND ( 'NONE', #22735, .T. ) ;
#54691=VERTEX_POINT ( 'NONE', #9050 ) ;
#54692=CARTESIAN_POINT ( 'NONE',  ( 37.00000000000000711, 4.705694406421931860E-17, -3.469127814946512892E-15 ) ) ;
#54694=CARTESIAN_POINT ( 'NONE',  ( -35.00000000000000000, -6.307491713049102167, 9.908974237959624176 ) ) ;
#54696=EDGE_CURVE ( 'NONE', #52407, #53488, #49626, .T. ) ;
#54697=CARTESIAN_POINT ( 'NONE',  ( 21.48046541981384649, 13.30940734634045519, -2.295139786869221599 ) ) ;
#54698=DIRECTION ( 'NONE',  ( 0.000000000000000000, 0.8169148498130255343, -0.5767582926624998940 ) ) ;
#54699=ORIENTED_EDGE ( 'NONE', *, *, #7413, .F. ) ;
#54702=DIRECTION ( 'NONE',  ( 0.000000000000000000, -0.01356324068817998940, 0.9999080150203990547 ) ) ;
#54703=VECTOR ( 'NONE', #10683, 1000.000000000000000 ) ;
#54704=ORIENTED_EDGE ( 'NONE', *, *, #14272, .T. ) ;
#54705=CARTESIAN_POINT ( 'NONE',  ( 35.00000000000000000, -11.44858830469738109, 2.627174906297032209 ) ) ;
#54708=CYLINDRICAL_SURFACE ( 'NONE', #53480, 5.594511299047803199 ) ;
#54713=ORIENTED_EDGE ( 'NONE', *, *, #43330, .T. ) ;
#54714=DIRECTION ( 'NONE',  ( 1.000000000000000000, 0.000000000000000000, 0.000000000000000000 ) ) ;
#54715=ORIENTED_EDGE ( 'NONE', *, *, #396, .T. ) ;
#54716=ORIENTED_EDGE ( 'NONE', *, *, #29617, .T. ) ;
#54717=DIRECTION ( 'NONE',  ( -0.1699641022377680333, 0.000000000000000000, 0.9854502544271371844 ) ) ;
#54719=CARTESIAN_POINT ( 'NONE',  ( -3.674131796199469946, 7.080541174871527232, 9.698525384827776818 ) ) ;
#54720=CIRCLE ( 'NONE', #29222, 5.000000000000000888 ) ;
#54721=EDGE_CURVE ( 'NONE', #22718, #42768, #38315, .T. ) ;
#54724=DIRECTION ( 'NONE',  ( 1.000000000000000000, 0.000000000000000000, 0.000000000000000000 ) ) ;
#54726=EDGE_CURVE ( 'NONE', #27953, #48271, #61018, .T. ) ;
#54730=ORIENTED_EDGE ( 'NONE', *, *, #62667, .T. ) ;
#54731=EDGE_CURVE ( 'NONE', #41856, #60581, #29330, .T. ) ;
#54732=CARTESIAN_POINT ( 'NONE',  ( -37.00000000000000711, -10.42955799785324444, 6.303578524886909840 ) ) ;
#54734=CARTESIAN_POINT ( 'NONE',  ( 35.00000000000000000, -0.7536123767497623360, 11.72195762423410237 ) ) ;
#54737=DIRECTION ( 'NONE',  ( 0.000000000000000000, -0.01356324068817991828, 0.9999080150203990547 ) ) ;
#54738=VERTEX_POINT ( 'NONE', #17730 ) ;
#54743=EDGE_CURVE ( 'NONE', #40981, #35757, #45576, .T. ) ;
#54744=DIRECTION ( 'NONE',  ( 0.000000000000000000, 0.01356324068817998940, -0.9999080150203989437 ) ) ;
#54745=CARTESIAN_POINT ( 'NONE',  ( 35.00000000000000000, 2.527899948230813987, 12.49688848680881037 ) ) ;
#54748=DIRECTION ( 'NONE',  ( -1.000000000000000000, 0.000000000000000000, 0.000000000000000000 ) ) ;
#54749=CYLINDRICAL_SURFACE ( 'NONE', #29104, 12.18649999999999878 ) ;
#54750=FACE_OUTER_BOUND ( 'NONE', #14930, .T. ) ;
#54752=DIRECTION ( 'NONE',  ( 0.000000000000000000, -0.01356324068817992175, 0.9999080150203990547 ) ) ;
#54753=DIRECTION ( 'NONE',  ( 1.000000000000000000, -0.000000000000000000, 0.000000000000000000 ) ) ;
#54757=CARTESIAN_POINT ( 'NONE',  ( 22.05617246934746589, 13.47655295422366173, -0.7978008018308921923 ) ) ;
#54760=EDGE_CURVE ( 'NONE', #57580, #56864, #40271, .T. ) ;
#54762=CARTESIAN_POINT ( 'NONE',  ( -28.21046445815681381, -10.37508796587660598, -6.038083143907718053 ) ) ;
#54766=DIRECTION ( 'NONE',  ( 0.000000000000000000, -0.01356324068817992175, 0.9999080150203990547 ) ) ;
#54771=CARTESIAN_POINT ( 'NONE',  ( 47.00000000000000711, 4.705694406421931860E-17, -3.469127814946512892E-15 ) ) ;
#54772=DIRECTION ( 'NONE',  ( 1.000000000000000000, 0.000000000000000000, -0.000000000000000000 ) ) ;
#54774=FACE_OUTER_BOUND ( 'NONE', #21925, .T. ) ;
#54776=VERTEX_POINT ( 'NONE', #4747 ) ;
#54777=CARTESIAN_POINT ( 'NONE',  ( -36.00000000000000711, -12.68495603654570836, -1.286231064351445630 ) ) ;
#54779=CARTESIAN_POINT ( 'NONE',  ( -18.34821779656727969, 6.410806818984529087, -11.88355244879351247 ) ) ;
#54780=AXIS2_PLACEMENT_3D ( 'NONE', #23850, #44108, #29454 ) ;
#54785=CARTESIAN_POINT ( 'NONE',  ( 37.00000000000000711, 4.705694406421931860E-17, -3.469127814946512892E-15 ) ) ;
#54787=ORIENTED_EDGE ( 'NONE', *, *, #43907, .T. ) ;
#54790=ORIENTED_EDGE ( 'NONE', *, *, #7328, .F. ) ;
#54791=AXIS2_PLACEMENT_3D ( 'NONE', #52359, #2472, #1494 ) ;
#54792=DIRECTION ( 'NONE',  ( -1.000000000000000000, 0.000000000000000000, 0.000000000000000000 ) ) ;
#54793=CARTESIAN_POINT ( 'NONE',  ( -16.98800322446194855, 2.922502605998049674, 25.00000000000000000 ) ) ;
#54794=ORIENTED_EDGE ( 'NONE', *, *, #31540, .T. ) ;
#54795=DIRECTION ( 'NONE',  ( 0.000000000000000000, -0.01356324068817998940, 0.9999080150203990547 ) ) ;
#54797=CARTESIAN_POINT ( 'NONE',  ( 35.00000000000000000, -11.50504120060945645, -4.018060380616356397 ) ) ;
#54798=CARTESIAN_POINT ( 'NONE',  ( -35.00000000000000000, -10.54834585426215732, -6.102719229070786788 ) ) ;
#54799=ORIENTED_EDGE ( 'NONE', *, *, #34524, .T. ) ;
#54800=EDGE_LOOP ( 'NONE', ( #40291, #10772, #24603, #18083 ) ) ;
#54802=DIRECTION ( 'NONE',  ( 0.000000000000000000, -0.5987040770935736500, 0.8009703041134121904 ) ) ;
#54803=ORIENTED_EDGE ( 'NONE', *, *, #47823, .T. ) ;
#54804=DIRECTION ( 'NONE',  ( 0.000000000000000000, 0.01356324068817998940, -0.9999080150203990547 ) ) ;
#54805=ORIENTED_EDGE ( 'NONE', *, *, #15145, .T. ) ;
#54806=CARTESIAN_POINT ( 'NONE',  ( -19.62362846926598436, -4.052573403833369170, -11.29610975316521859 ) ) ;
#54807=DIRECTION ( 'NONE',  ( -0.000000000000000000, -0.000000000000000000, -1.000000000000000000 ) ) ;
#54810=CARTESIAN_POINT ( 'NONE',  ( -27.01437459610461644, 25.00000000000000000, -2.220455681983952267 ) ) ;
#54811=CARTESIAN_POINT ( 'NONE',  ( 35.00000000000000000, -12.17626345777663310, 0.4993900848168664752 ) ) ;
#54813=CARTESIAN_POINT ( 'NONE',  ( 37.00000000000000711, -9.076753354953932984, 8.954052073409695112 ) ) ;
#54814=DIRECTION ( 'NONE',  ( 1.000000000000000000, 0.000000000000000000, 0.000000000000000000 ) ) ;
#54816=LINE ( 'NONE', #54157, #8339 ) ;
#54817=CARTESIAN_POINT ( 'NONE',  ( 11.50502875988115115, 13.34043489419269335, -2.074406423247350695 ) ) ;
#54819=DIRECTION ( 'NONE',  ( -0.000000000000000000, -0.000000000000000000, -1.000000000000000000 ) ) ;
#54821=DIRECTION ( 'NONE',  ( 0.000000000000000000, 0.01356324068817998940, -0.9999080150203989437 ) ) ;
#54823=CARTESIAN_POINT ( 'NONE',  ( -15.95149727525144101, 8.394611330425535201, -8.575054620236299385 ) ) ;
#54824=AXIS2_PLACEMENT_3D ( 'NONE', #48704, #33717, #39358 ) ;
#54825=ORIENTED_EDGE ( 'NONE', *, *, #63479, .F. ) ;
#54826=DIRECTION ( 'NONE',  ( 1.000000000000000000, 0.000000000000000000, 0.000000000000000000 ) ) ;
#54828=CARTESIAN_POINT ( 'NONE',  ( 35.00000000000000000, -4.018060380616318206, 11.50504120060946533 ) ) ;
#54831=VERTEX_POINT ( 'NONE', #60240 ) ;
#54832=FACE_OUTER_BOUND ( 'NONE', #34989, .T. ) ;
#54833=CARTESIAN_POINT ( 'NONE',  ( 37.00000000000000711, -6.711949091238068377, 10.84030624090613237 ) ) ;
#54834=CARTESIAN_POINT ( 'NONE',  ( 35.00000000000000000, -8.258652103341374229, 8.352657516904754331 ) ) ;
#54836=EDGE_CURVE ( 'NONE', #31870, #45916, #64190, .T. ) ;
#54837=DIRECTION ( 'NONE',  ( 0.000000000000000000, 0.9346839223284527653, -0.3554799084909000539 ) ) ;
#54839=CARTESIAN_POINT ( 'NONE',  ( 37.00000000000000711, -2.185196060783960892, -11.54110654723648466 ) ) ;
#54842=FACE_OUTER_BOUND ( 'NONE', #46730, .T. ) ;
#54844=CARTESIAN_POINT ( 'NONE',  ( 6.806520558696398382, -6.060494548531525361, 12.06920317132890830 ) ) ;
#54846=ORIENTED_EDGE ( 'NONE', *, *, #52411, .T. ) ;
#54847=EDGE_LOOP ( 'NONE', ( #55352, #63830 ) ) ;
#54849=CARTESIAN_POINT ( 'NONE',  ( -35.00000000000000000, -3.033604067594665388, 12.38385022362080790 ) ) ;
#54851=DIRECTION ( 'NONE',  ( -1.000000000000000000, 0.000000000000000000, 0.000000000000000000 ) ) ;
#54853=CARTESIAN_POINT ( 'NONE',  ( 37.00000000000000711, -6.917234959366766134, 9.493370459201765144 ) ) ;
#54856=PLANE ( 'NONE',  #42416 ) ;
#54857=ORIENTED_EDGE ( 'NONE', *, *, #19337, .F. ) ;
#54858=EDGE_LOOP ( 'NONE', ( #45548, #17722, #13334, #24179 ) ) ;
#54860=FACE_OUTER_BOUND ( 'NONE', #40025, .T. ) ;
#54861=CARTESIAN_POINT ( 'NONE',  ( 35.00000000000000000, 10.93004082984027825, 6.564808257521645096 ) ) ;
#54862=ORIENTED_EDGE ( 'NONE', *, *, #12712, .F. ) ;
#54863=FACE_BOUND ( 'NONE', #26987, .T. ) ;
#54865=FACE_OUTER_BOUND ( 'NONE', #47296, .T. ) ;
#54866=EDGE_CURVE ( 'NONE', #19699, #7095, #34509, .T. ) ;
#54868=CARTESIAN_POINT ( 'NONE',  ( 6.849147238560869155, -8.368406977534899482, 8.611611683099951620 ) ) ;
#54869=ORIENTED_EDGE ( 'NONE', *, *, #52496, .F. ) ;
#54870=ORIENTED_EDGE ( 'NONE', *, *, #5740, .F. ) ;
#54871=CYLINDRICAL_SURFACE ( 'NONE', #39549, 12.75000000000000178 ) ;
#54873=ORIENTED_EDGE ( 'NONE', *, *, #31465, .F. ) ;
#54874=CARTESIAN_POINT ( 'NONE',  ( 35.00000000000000000, 11.81949347079746637, -2.968224442958448783 ) ) ;
#54876=ORIENTED_EDGE ( 'NONE', *, *, #45855, .F. ) ;
#54878=CARTESIAN_POINT ( 'NONE',  ( 35.00000000000000000, -4.041347439435937439, -11.02904044024207764 ) ) ;
#54879=CARTESIAN_POINT ( 'NONE',  ( -37.00000000000000711, -5.246972444134096136, 10.99909370905155548 ) ) ;
#54880=CARTESIAN_POINT ( 'NONE',  ( 35.00000000000000000, -12.66641127287626567, -1.457575200925504966 ) ) ;
#54882=DIRECTION ( 'NONE',  ( -1.000000000000000000, 0.000000000000000000, 0.000000000000000000 ) ) ;
#54883=ORIENTED_EDGE ( 'NONE', *, *, #701, .F. ) ;
#54885=EDGE_LOOP ( 'NONE', ( #63778, #34660, #14970, #46697 ) ) ;
#54886=CARTESIAN_POINT ( 'NONE',  ( -35.00000000000000000, -0.4353888892047496628, -11.73808581813438501 ) ) ;
#54887=CARTESIAN_POINT ( 'NONE',  ( -35.00000000000000000, 10.30098186818257666, -5.644643009978957515 ) ) ;
#54888=ORIENTED_EDGE ( 'NONE', *, *, #55843, .F. ) ;
#54890=CYLINDRICAL_SURFACE ( 'NONE', #19076, 12.75000000000000178 ) ;
#54895=EDGE_CURVE ( 'NONE', #5144, #1474, #31259, .T. ) ;
#54897=CARTESIAN_POINT ( 'NONE',  ( -26.99479954988168018, -12.46966287028880593, 5.172898835462513389 ) ) ;
#54901=DIRECTION ( 'NONE',  ( -1.000000000000000000, 0.000000000000000000, -0.000000000000000000 ) ) ;
#54902=ORIENTED_EDGE ( 'NONE', *, *, #30160, .T. ) ;
#54906=AXIS2_PLACEMENT_3D ( 'NONE', #22976, #63194, #43229 ) ;
#54907=DIRECTION ( 'NONE',  ( -1.000000000000000000, 0.000000000000000000, 0.000000000000000000 ) ) ;
#54908=CARTESIAN_POINT ( 'NONE',  ( -36.00000000000000711, -6.711949091238219367, 10.84030624090604356 ) ) ;
#54909=DIRECTION ( 'NONE',  ( 0.000000000000000000, 0.01356324068817998940, -0.9999080150203990547 ) ) ;
#54911=CARTESIAN_POINT ( 'NONE',  ( -35.00000000000000000, -9.240395740215685549, 7.251710744571544964 ) ) ;
#54912=EDGE_CURVE ( 'NONE', #1959, #31052, #11659, .T. ) ;
#54914=ORIENTED_EDGE ( 'NONE', *, *, #34410, .T. ) ;
#54917=CARTESIAN_POINT ( 'NONE',  ( -47.00000000000000711, 0.000000000000000000, 0.000000000000000000 ) ) ;
#54918=CARTESIAN_POINT ( 'NONE',  ( 35.00000000000000000, 4.705694406421931860E-17, -3.469127814946512892E-15 ) ) ;
#54920=LINE ( 'NONE', #25647, #6343 ) ;
#54921=ORIENTED_EDGE ( 'NONE', *, *, #9009, .T. ) ;
#54923=ORIENTED_EDGE ( 'NONE', *, *, #15601, .T. ) ;
#54925=CARTESIAN_POINT ( 'NONE',  ( -27.28563326141737733, 11.69479555401723836, -2.740829448094128207 ) ) ;
#54929=CARTESIAN_POINT ( 'NONE',  ( 35.00000000000000000, 0.4353888892050056802, 11.73808581813437080 ) ) ;
#54931=FACE_OUTER_BOUND ( 'NONE', #14450, .T. ) ;
#54933=DIRECTION ( 'NONE',  ( -1.000000000000000000, -0.000000000000000000, 0.000000000000000000 ) ) ;
#54934=EDGE_CURVE ( 'NONE', #19566, #62364, #53577, .T. ) ;
#54936=FACE_OUTER_BOUND ( 'NONE', #5739, .T. ) ;
#54940=ADVANCED_FACE ( 'NONE', ( #1708 ), #42225, .T. ) ;
#54943=EDGE_LOOP ( 'NONE', ( #45537, #17493, #48264, #40533 ) ) ;
#54944=DIRECTION ( 'NONE',  ( 0.000000000000000000, -0.01356324068817998940, 0.9999080150203990547 ) ) ;
#54945=CARTESIAN_POINT ( 'NONE',  ( 12.19958943313458022, -11.82211122194439312, -2.065116011828826093 ) ) ;
#54947=CARTESIAN_POINT ( 'NONE',  ( 37.00000000000000711, 4.705694406421931860E-17, -3.469127814946512892E-15 ) ) ;
#54948=DIRECTION ( 'NONE',  ( 1.000000000000000000, 0.000000000000000000, -0.000000000000000000 ) ) ;
#54949=AXIS2_PLACEMENT_3D ( 'NONE', #46366, #16748, #21074 ) ;
#54950=EDGE_CURVE ( 'NONE', #52686, #32582, #51604, .T. ) ;
#54952=DIRECTION ( 'NONE',  ( 1.000000000000000000, 0.000000000000000000, 0.000000000000000000 ) ) ;
#54953=LINE ( 'NONE', #9381, #59678 ) ;
#54954=VERTEX_POINT ( 'NONE', #7012 ) ;
#54955=( BOUNDED_CURVE ( )  B_SPLINE_CURVE ( 3, ( #37228, #22267, #22618, #36911 ),
 .UNSPECIFIED., .F., .F. ) 
 B_SPLINE_CURVE_WITH_KNOTS ( ( 4, 4 ),
 ( 1.253538260309761343, 1.290660968744300696 ),
 .UNSPECIFIED. ) 
 CURVE ( )  GEOMETRIC_REPRESENTATION_ITEM ( )  RATIONAL_B_SPLINE_CURVE ( ( 1.000000000000000000, 0.9998851620069661994, 0.9998851620069661994, 1.000000000000000000 ) ) 
 REPRESENTATION_ITEM ( '' )  );
#54956=EDGE_LOOP ( 'NONE', ( #12698, #3832, #62307, #50387 ) ) ;
#54957=CARTESIAN_POINT ( 'NONE',  ( 12.56483561494067658, -13.26188203154483247, -2.530721474258640580 ) ) ;
#54960=VERTEX_POINT ( 'NONE', #720 ) ;
#54961=CARTESIAN_POINT ( 'NONE',  ( 22.57855258442565116, 3.026812727784649493, 13.15630665159948975 ) ) ;
#54963=CARTESIAN_POINT ( 'NONE',  ( 22.78424990826529850, -4.691658877507586034, 11.04575192261954442 ) ) ;
#54965=EDGE_CURVE ( 'NONE', #26733, #13869, #49369, .T. ) ;
#54968=CARTESIAN_POINT ( 'NONE',  ( -35.00000000000000000, -10.25474254703948418, -6.584150480049660636 ) ) ;
#54969=EDGE_CURVE ( 'NONE', #18633, #42493, #36275, .T. ) ;
#54970=ORIENTED_EDGE ( 'NONE', *, *, #9414, .F. ) ;
#54972=EDGE_CURVE ( 'NONE', #3010, #8331, #24892, .T. ) ;
#54977=AXIS2_PLACEMENT_3D ( 'NONE', #31045, #52658, #11103 ) ;
#54981=ORIENTED_EDGE ( 'NONE', *, *, #9816, .T. ) ;
#54984=CARTESIAN_POINT ( 'NONE',  ( 2.745955655249697980, 2.199760390095205409, 11.80339285908471147 ) ) ;
#54985=CIRCLE ( 'NONE', #45395, 12.75000000000000178 ) ;
#54986=ADVANCED_FACE ( 'NONE', ( #29741 ), #10446, .T. ) ;
#54987=EDGE_CURVE ( 'NONE', #48877, #11231, #28082, .T. ) ;
#54989=DIRECTION ( 'NONE',  ( 1.000000000000000000, 0.000000000000000000, 0.000000000000000000 ) ) ;
#54990=DIRECTION ( 'NONE',  ( -1.000000000000000000, 0.000000000000000000, 0.000000000000000000 ) ) ;
#54992=CARTESIAN_POINT ( 'NONE',  ( -37.00000000000000711, 0.000000000000000000, 0.000000000000000000 ) ) ;
#54995=VERTEX_POINT ( 'NONE', #20769 ) ;
#54996=CARTESIAN_POINT ( 'NONE',  ( 22.02397509040500623, 12.24077527228601170, -5.706323397743170212 ) ) ;
#54998=VERTEX_POINT ( 'NONE', #15445 ) ;
#55000=EDGE_LOOP ( 'NONE', ( #35240, #17261, #10105, #27871 ) ) ;
#55001=EDGE_LOOP ( 'NONE', ( #14767, #10034, #43086, #35319 ) ) ;
#55004=ORIENTED_EDGE ( 'NONE', *, *, #48722, .T. ) ;
#55007=CARTESIAN_POINT ( 'NONE',  ( -35.00000000000000000, 7.499679039484183463, -9.040300684349618976 ) ) ;
#55008=CARTESIAN_POINT ( 'NONE',  ( -37.00000000000000711, 2.250029553613937416, -12.54989509947648685 ) ) ;
#55010=DIRECTION ( 'NONE',  ( 0.000000000000000000, -0.9346839223284501008, 0.3554799084909072149 ) ) ;
#55012=VERTEX_POINT ( 'NONE', #25761 ) ;
#55013=DIRECTION ( 'NONE',  ( 1.000000000000000000, -0.000000000000000000, 0.000000000000000000 ) ) ;
#55014=ADVANCED_FACE ( 'NONE', ( #36037 ), #56336, .T. ) ;
#55015=VERTEX_POINT ( 'NONE', #4840 ) ;
#55016=DIRECTION ( 'NONE',  ( 0.000000000000000000, 0.9847383929261610547, -0.1740410799127649344 ) ) ;
#55017=ORIENTED_EDGE ( 'NONE', *, *, #15821, .T. ) ;
#55018=EDGE_LOOP ( 'NONE', ( #39621, #13212, #56166, #26529 ) ) ;
#55021=CIRCLE ( 'NONE', #64596, 12.18649999999999878 ) ;
#55024=CARTESIAN_POINT ( 'NONE',  ( 35.00000000000000000, -12.70128625845191728, 1.113475361586618195 ) ) ;
#55025=CARTESIAN_POINT ( 'NONE',  ( -17.83419946441818027, -9.720786832536937538, -9.367833439828872955 ) ) ;
#55027=AXIS2_PLACEMENT_3D ( 'NONE', #2251, #6913, #21553 ) ;
#55028=ORIENTED_EDGE ( 'NONE', *, *, #58022, .T. ) ;
#55029=LINE ( 'NONE', #39744, #41150 ) ;
#55032=CIRCLE ( 'NONE', #52899, 12.75000000000000178 ) ;
#55036=CIRCLE ( 'NONE', #60304, 5.000000000000000888 ) ;
#55038=CARTESIAN_POINT ( 'NONE',  ( 37.00000000000000711, 6.307491713049029336, -9.908974237959670361 ) ) ;
#55041=CARTESIAN_POINT ( 'NONE',  ( 22.88594695219327235, -4.822122601967141264, 25.00000000000000000 ) ) ;
#55045=ORIENTED_EDGE ( 'NONE', *, *, #35678, .T. ) ;
#55046=EDGE_CURVE ( 'NONE', #37865, #27549, #10135, .T. ) ;
#55050=CARTESIAN_POINT ( 'NONE',  ( -17.96927786591849241, -9.630624776632362938, -7.160636282608098924 ) ) ;
#55051=CIRCLE ( 'NONE', #22161, 5.000000000000000888 ) ;
#55052=DIRECTION ( 'NONE',  ( 0.000000000000000000, -0.01356324068817999114, 0.9999080150203989437 ) ) ;
#55053=AXIS2_PLACEMENT_3D ( 'NONE', #36117, #26487, #31163 ) ;
#55055=LINE ( 'NONE', #35426, #31170 ) ;
#55056=DIRECTION ( 'NONE',  ( 0.000000000000000000, 0.01356324068817991828, -0.9999080150203990547 ) ) ;
#55058=ORIENTED_EDGE ( 'NONE', *, *, #5528, .T. ) ;
#55061=DIRECTION ( 'NONE',  ( 0.000000000000000000, -0.2355298848897586228, -0.9718671068226442111 ) ) ;
#55062=ADVANCED_FACE ( 'NONE', ( #9455 ), #504, .T. ) ;
#55063=DIRECTION ( 'NONE',  ( 0.5702167306099040767, -0.8214942970785323872, 0.000000000000000000 ) ) ;
#55064=ADVANCED_FACE ( 'NONE', ( #31070 ), #25423, .T. ) ;
#55067=AXIS2_PLACEMENT_3D ( 'NONE', #38415, #8482, #58733 ) ;
#55068=VERTEX_POINT ( 'NONE', #27707 ) ;
#55072=ORIENTED_EDGE ( 'NONE', *, *, #24094, .T. ) ;
#55075=CARTESIAN_POINT ( 'NONE',  ( -35.00000000000000000, 12.08151691381195825, -4.074242145635880163 ) ) ;
#55076=LINE ( 'NONE', #20817, #56701 ) ;
#55078=AXIS2_PLACEMENT_3D ( 'NONE', #11532, #6894, #6569 ) ;
#55083=DIRECTION ( 'NONE',  ( 0.000000000000000000, 0.01356324068817998940, -0.9999080150203990547 ) ) ;
#55086=DIRECTION ( 'NONE',  ( 1.000000000000000000, 0.000000000000000000, 0.000000000000000000 ) ) ;
#55087=CARTESIAN_POINT ( 'NONE',  ( -35.00000000000000000, 11.78745411414839594, 3.093009498343968211 ) ) ;
#55089=CYLINDRICAL_SURFACE ( 'NONE', #2145, 12.74999999999999822 ) ;
#55091=ADVANCED_FACE ( 'NONE', ( #51702, #1806 ), #48014, .F. ) ;
#55093=CARTESIAN_POINT ( 'NONE',  ( 35.00000000000000000, 4.705694406421931860E-17, -3.469127814946512892E-15 ) ) ;
#55094=VERTEX_POINT ( 'NONE', #11752 ) ;
#55095=EDGE_CURVE ( 'NONE', #56356, #63372, #29125, .T. ) ;
#55099=EDGE_LOOP ( 'NONE', ( #23923, #6460, #65500, #22604 ) ) ;
#55100=LINE ( 'NONE', #14516, #17061 ) ;
#55101=CARTESIAN_POINT ( 'NONE',  ( -27.19357181888462094, -12.48377454417556542, 5.138615876886901468 ) ) ;
#55102=AXIS2_PLACEMENT_3D ( 'NONE', #7431, #62972, #17437 ) ;
#55103=CARTESIAN_POINT ( 'NONE',  ( 23.20064169955008282, 3.175852713112300663, 13.12357665716721478 ) ) ;
#55105=VERTEX_POINT ( 'NONE', #47034 ) ;
#55106=CARTESIAN_POINT ( 'NONE',  ( 35.00000000000000000, -7.094637218249427058, -10.59380114696467601 ) ) ;
#55109=ORIENTED_EDGE ( 'NONE', *, *, #18767, .T. ) ;
#55111=EDGE_CURVE ( 'NONE', #44528, #27612, #11127, .T. ) ;
#55112=CARTESIAN_POINT ( 'NONE',  ( -4.989057617119011745, -0.9162120371760335003, 25.00000000000000000 ) ) ;
#55113=AXIS2_PLACEMENT_3D ( 'NONE', #23193, #57469, #43454 ) ;
#55115=DIRECTION ( 'NONE',  ( 0.8867529933577789070, 0.000000000000000000, -0.4622435816439414147 ) ) ;
#55118=CIRCLE ( 'NONE', #43429, 12.75000000000000178 ) ;
#55119=ORIENTED_EDGE ( 'NONE', *, *, #22003, .F. ) ;
#55121=CARTESIAN_POINT ( 'NONE',  ( -35.00000000000000000, 11.70009620280411688, 1.039216533672945753 ) ) ;
#55122=ADVANCED_FACE ( 'NONE', ( #36387 ), #56696, .T. ) ;
#55123=CARTESIAN_POINT ( 'NONE',  ( -35.00000000000000000, -12.02534193257723949, 4.237174932027182095 ) ) ;
#55128=CARTESIAN_POINT ( 'NONE',  ( 12.10998784662220729, 8.443435280036798218, -8.526922110106905706 ) ) ;
#55129=AXIS2_PLACEMENT_3D ( 'NONE', #53689, #64298, #9096 ) ;
#55130=FACE_OUTER_BOUND ( 'NONE', #35825, .T. ) ;
#55133=EDGE_CURVE ( 'NONE', #22402, #3402, #55869, .T. ) ;
#55136=CARTESIAN_POINT ( 'NONE',  ( -3.224836612564374594, -7.386197834073436219, 9.465828205825033592 ) ) ;
#55137=DIRECTION ( 'NONE',  ( 0.000000000000000000, 0.01356324068817992175, -0.9999080150203990547 ) ) ;
#55141=ORIENTED_EDGE ( 'NONE', *, *, #18415, .T. ) ;
#55142=CARTESIAN_POINT ( 'NONE',  ( -11.31756720043940767, -8.578238994477491275, -10.42748751657815198 ) ) ;
#55146=CIRCLE ( 'NONE', #38195, 12.18649999999999878 ) ;
#55147=EDGE_CURVE ( 'NONE', #3036, #51673, #17082, .T. ) ;
#55148=DIRECTION ( 'NONE',  ( 1.000000000000000000, 0.000000000000000000, 0.000000000000000000 ) ) ;
#55150=ORIENTED_EDGE ( 'NONE', *, *, #17689, .F. ) ;
#55152=DIRECTION ( 'NONE',  ( 0.000000000000000000, 0.01356324068817998940, -0.9999080150203990547 ) ) ;
#55156=FACE_OUTER_BOUND ( 'NONE', #26240, .T. ) ;
#55157=CARTESIAN_POINT ( 'NONE',  ( -29.68541646480311869, -1.416020129149132334, -13.42553116244736877 ) ) ;
#55158=CIRCLE ( 'NONE', #29703, 1.750000000000000000 ) ;
#55159=ORIENTED_EDGE ( 'NONE', *, *, #7105, .T. ) ;
#55160=ORIENTED_EDGE ( 'NONE', *, *, #21092, .F. ) ;
#55162=EDGE_LOOP ( 'NONE', ( #43378, #54647, #24975, #42030 ) ) ;
#55163=CIRCLE ( 'NONE', #14793, 5.000000000000000888 ) ;
#55165=DIRECTION ( 'NONE',  ( 1.000000000000000000, -0.000000000000000000, 0.000000000000000000 ) ) ;
#55169=DIRECTION ( 'NONE',  ( 0.000000000000000000, -0.5767582926625031137, -0.8169148498130233138 ) ) ;
#55172=EDGE_CURVE ( 'NONE', #1814, #37251, #49520, .T. ) ;
#55175=AXIS2_PLACEMENT_3D ( 'NONE', #31943, #52265, #6705 ) ;
#55178=EDGE_CURVE ( 'NONE', #53714, #21888, #27072, .T. ) ;
#55179=CARTESIAN_POINT ( 'NONE',  ( -37.00000000000000711, -7.608228585767650820, -10.23119532541081078 ) ) ;
#55181=FACE_BOUND ( 'NONE', #11379, .T. ) ;
#55182=ORIENTED_EDGE ( 'NONE', *, *, #64279, .F. ) ;
#55183=CARTESIAN_POINT ( 'NONE',  ( 47.00000000000000711, 4.705694406421931860E-17, -3.469127814946512892E-15 ) ) ;
#55184=DIRECTION ( 'NONE',  ( 0.000000000000000000, -0.7381862504172023165, 0.6745969609292585822 ) ) ;
#55187=ORIENTED_EDGE ( 'NONE', *, *, #2080, .F. ) ;
#55188=VERTEX_POINT ( 'NONE', #6798 ) ;
#55190=ORIENTED_EDGE ( 'NONE', *, *, #33567, .F. ) ;
#55191=CARTESIAN_POINT ( 'NONE',  ( 35.00000000000000000, -5.927257550915237871, 10.64792938439761549 ) ) ;
#55192=ORIENTED_EDGE ( 'NONE', *, *, #36342, .F. ) ;
#55193=ORIENTED_EDGE ( 'NONE', *, *, #33043, .T. ) ;
#55194=ORIENTED_EDGE ( 'NONE', *, *, #60871, .F. ) ;
#55196=EDGE_CURVE ( 'NONE', #53449, #6611, #39945, .T. ) ;
#55198=AXIS2_PLACEMENT_3D ( 'NONE', #2594, #41814, #47155 ) ;
#55199=VECTOR ( 'NONE', #11534, 1000.000000000000000 ) ;
#55202=ORIENTED_EDGE ( 'NONE', *, *, #21731, .F. ) ;
#55204=ORIENTED_EDGE ( 'NONE', *, *, #51882, .F. ) ;
#55205=AXIS2_PLACEMENT_3D ( 'NONE', #17366, #11697, #47619 ) ;
#55206=DIRECTION ( 'NONE',  ( 1.000000000000000000, 0.000000000000000000, -0.000000000000000000 ) ) ;
#55207=B_SPLINE_CURVE_WITH_KNOTS ( 'NONE', 3,
 ( #13444, #63009, #28744, #17472, #49059, #3513, #44047, #64318, #54996, #30053, #50366, #4813, #64628, #54367, #54697, #5126, #9118, #34391 ),
 .UNSPECIFIED., .F., .F.,
 ( 4, 2, 2, 2, 2, 2, 2, 2, 4 ),
 ( 1.734723475976807094E-18, 0.001213967396161172267, 0.002427934792322344101, 0.003641902188483516368, 0.004855869584644688201, 0.006069836980805859601, 0.007283804376967032736, 0.008497771773128205003, 0.009711739169289378137 ),
 .UNSPECIFIED. ) ;
#55208=DIRECTION ( 'NONE',  ( -1.000000000000000000, 0.000000000000000000, -0.000000000000000000 ) ) ;
#55209=ORIENTED_EDGE ( 'NONE', *, *, #16385, .F. ) ;
#55210=CARTESIAN_POINT ( 'NONE',  ( -27.69447987491729890, 12.79070223153173202, -4.327645566905162333 ) ) ;
#55214=ADVANCED_FACE ( 'NONE', ( #31402 ), #47676, .T. ) ;
#55215=B_SPLINE_CURVE_WITH_KNOTS ( 'NONE', 3,
 ( #22442, #42707, #32720, #53030, #27113, #1845, #63004, #37740, #7465, #27757, #48060, #2519, #22790, #15161 ),
 .UNSPECIFIED., .F., .F.,
 ( 4, 2, 2, 2, 2, 2, 4 ),
 ( 7.113556129967474992E-17, 0.002809884958117719617, 0.004214827437176541479, 0.005619769916235362907, 0.007024712395294183467, 0.008429654874353006630, 0.01123953983247064949 ),
 .UNSPECIFIED. ) ;
#55216=ORIENTED_EDGE ( 'NONE', *, *, #39016, .T. ) ;
#55218=VECTOR ( 'NONE', #48807, 1000.000000000000000 ) ;
#55221=CARTESIAN_POINT ( 'NONE',  ( -19.88336747883694500, -13.23946304221971282, -2.721115890609613341 ) ) ;
#55224=FACE_OUTER_BOUND ( 'NONE', #42304, .T. ) ;
#55225=ORIENTED_EDGE ( 'NONE', *, *, #3009, .T. ) ;
#55226=DIRECTION ( 'NONE',  ( 0.000000000000000000, -0.01356324068817998940, 0.9999080150203990547 ) ) ;
#55228=CIRCLE ( 'NONE', #11690, 5.000000000000000888 ) ;
#55230=CARTESIAN_POINT ( 'NONE',  ( -30.01205539201145811, -3.373358488642692166, 13.07763805471449992 ) ) ;
#55231=EDGE_CURVE ( 'NONE', #42736, #56824, #57012, .T. ) ;
#55236=CARTESIAN_POINT ( 'NONE',  ( -7.291047549687195151, -5.640864668324916842, -10.59540170654024926 ) ) ;
#55237=FACE_OUTER_BOUND ( 'NONE', #37981, .T. ) ;
#55239=AXIS2_PLACEMENT_3D ( 'NONE', #20131, #16125, #56720 ) ;
#55243=DIRECTION ( 'NONE',  ( 0.000000000000000000, -0.9718671068226435450, 0.2355298848897615926 ) ) ;
#55244=ORIENTED_EDGE ( 'NONE', *, *, #28603, .F. ) ;
#55245=DIRECTION ( 'NONE',  ( 1.000000000000000000, 0.000000000000000000, 0.000000000000000000 ) ) ;
#55247=DIRECTION ( 'NONE',  ( -0.000000000000000000, -1.000000000000000000, -0.000000000000000000 ) ) ;
#55248=LINE ( 'NONE', #49940, #1024 ) ;
#55250=ADVANCED_FACE ( 'NONE', ( #34006 ), #34342, .T. ) ;
#55251=ORIENTED_EDGE ( 'NONE', *, *, #62323, .F. ) ;
#55254=VECTOR ( 'NONE', #32665, 1000.000000000000000 ) ;
#55257=FACE_OUTER_BOUND ( 'NONE', #11954, .T. ) ;
#55259=CIRCLE ( 'NONE', #44605, 5.000000000000000888 ) ;
#55260=CARTESIAN_POINT ( 'NONE',  ( 35.00000000000000000, -6.584150480049477672, 10.25474254703959431 ) ) ;
#55261=ORIENTED_EDGE ( 'NONE', *, *, #21216, .T. ) ;
#55263=DIRECTION ( 'NONE',  ( -0.000000000000000000, -0.000000000000000000, -1.000000000000000000 ) ) ;
#55266=DIRECTION ( 'NONE',  ( -1.000000000000000000, 0.000000000000000000, 0.000000000000000000 ) ) ;
#55267=ORIENTED_EDGE ( 'NONE', *, *, #42042, .F. ) ;
#55268=DIRECTION ( 'NONE',  ( 1.000000000000000000, -0.000000000000000000, 0.000000000000000000 ) ) ;
#55269=ORIENTED_EDGE ( 'NONE', *, *, #43146, .T. ) ;
#55271=CARTESIAN_POINT ( 'NONE',  ( 12.94129669753463041, -11.57272345498358312, -3.180035631305769606 ) ) ;
#55272=CARTESIAN_POINT ( 'NONE',  ( -36.00000000000000711, 8.624332853796195408, -9.390600770287900190 ) ) ;
#55274=CARTESIAN_POINT ( 'NONE',  ( -25.15598030215514314, -10.22730567488070008, 6.279923306559322960 ) ) ;
#55275=LINE ( 'NONE', #19395, #58013 ) ;
#55277=CARTESIAN_POINT ( 'NONE',  ( 35.00000000000000000, -6.753013023069642351, 10.14433819232440825 ) ) ;
#55278=CARTESIAN_POINT ( 'NONE',  ( -35.00000000000000000, -0.4353888892047496628, -11.73808581813438501 ) ) ;
#55279=DIRECTION ( 'NONE',  ( -1.000000000000000000, 0.000000000000000000, -0.000000000000000000 ) ) ;
#55281=AXIS2_PLACEMENT_3D ( 'NONE', #36109, #5572, #19860 ) ;
#55282=ORIENTED_EDGE ( 'NONE', *, *, #50842, .F. ) ;
#55283=DIRECTION ( 'NONE',  ( 0.000000000000000000, -0.6269146997508042718, -0.7790879021242460567 ) ) ;
#55285=ORIENTED_EDGE ( 'NONE', *, *, #43244, .F. ) ;
#55287=DIRECTION ( 'NONE',  ( 0.000000000000000000, -0.01356324068817992001, 0.9999080150203990547 ) ) ;
#55291=VECTOR ( 'NONE', #38471, 1000.000000000000000 ) ;
#55292=AXIS2_PLACEMENT_3D ( 'NONE', #26513, #10553, #50814 ) ;
#55293=AXIS2_PLACEMENT_3D ( 'NONE', #8233, #7575, #3607 ) ;
#55294=CARTESIAN_POINT ( 'NONE',  ( 35.00000000000000000, -9.821084925794620446, -7.215058775251224077 ) ) ;
#55300=B_SPLINE_CURVE_WITH_KNOTS ( 'NONE', 3,
 ( #37268, #11032, #36940, #11998, #47918, #56590, #22296, #61893, #62868, #16352, #36624, #52896, #56930, #11349, #31619, #32280, #51932, #6374, #27292, #47586, #46935, #1396 ),
 .UNSPECIFIED., .F., .F.,
 ( 4, 2, 2, 2, 2, 2, 2, 2, 2, 2, 4 ),
 ( 8.673617379884034509E-19, 0.001199317212602414714, 0.002398634425204828561, 0.003597951637807242625, 0.004797268850409656255, 0.005396927456710863720, 0.005996586063012071185, 0.006596244669313276916, 0.007195903275614484382, 0.008395220488216890639, 0.009594537700819298631 ),
 .UNSPECIFIED. ) ;
#55301=AXIS2_PLACEMENT_3D ( 'NONE', #49076, #59353, #3850 ) ;
#55303=EDGE_CURVE ( 'NONE', #9194, #57308, #36731, .T. ) ;
#55305=CIRCLE ( 'NONE', #27669, 11.99999999999998757 ) ;
#55308=AXIS2_PLACEMENT_3D ( 'NONE', #49514, #44822, #65416 ) ;
#55309=DIRECTION ( 'NONE',  ( -0.000000000000000000, -1.000000000000000000, -0.000000000000000000 ) ) ;
#55310=CARTESIAN_POINT ( 'NONE',  ( -35.00000000000000000, 6.584150480049696164, -10.25474254703945931 ) ) ;
#55312=ORIENTED_EDGE ( 'NONE', *, *, #15454, .T. ) ;
#55314=CARTESIAN_POINT ( 'NONE',  ( -37.00000000000000711, -12.16893194857547655, -3.805206332242601963 ) ) ;
#55315=CARTESIAN_POINT ( 'NONE',  ( 1.959574367826918628, 1.098676416133668399, 11.95516700061986626 ) ) ;
#55316=VECTOR ( 'NONE', #8584, 1000.000000000000000 ) ;
#55317=ADVANCED_FACE ( 'NONE', ( #3127 ), #38342, .T. ) ;
#55318=CARTESIAN_POINT ( 'NONE',  ( 35.00000000000000000, -10.68873102412837639, 6.950793414699901085 ) ) ;
#55320=AXIS2_PLACEMENT_3D ( 'NONE', #60262, #14684, #34967 ) ;
#55321=ORIENTED_EDGE ( 'NONE', *, *, #1109, .T. ) ;
#55326=ORIENTED_EDGE ( 'NONE', *, *, #21027, .T. ) ;
#55327=CARTESIAN_POINT ( 'NONE',  ( 9.220846792691668625, 1.923872522168136090, 13.36437008182772779 ) ) ;
#55328=CIRCLE ( 'NONE', #63814, 12.74999999999999822 ) ;
#55329=DIRECTION ( 'NONE',  ( 0.000000000000000000, -0.2618041379715496664, 0.9651210252299831094 ) ) ;
#55331=ORIENTED_EDGE ( 'NONE', *, *, #4902, .F. ) ;
#55334=AXIS2_PLACEMENT_3D ( 'NONE', #46330, #21032, #1098 ) ;
#55336=EDGE_CURVE ( 'NONE', #59597, #47265, #25058, .T. ) ;
#55337=DIRECTION ( 'NONE',  ( 1.000000000000000000, 0.000000000000000000, 0.000000000000000000 ) ) ;
#55341=( BOUNDED_CURVE ( )  B_SPLINE_CURVE ( 3, ( #4236, #3614, #39465, #8558 ),
 .UNSPECIFIED., .F., .F. ) 
 B_SPLINE_CURVE_WITH_KNOTS ( ( 4, 4 ),
 ( 5.469309591143874272, 5.496147290052819656 ),
 .UNSPECIFIED. ) 
 CURVE ( )  GEOMETRIC_REPRESENTATION_ITEM ( )  RATIONAL_B_SPLINE_CURVE ( ( 1.000000000000000000, 0.9999399790604226457, 0.9999399790604226457, 1.000000000000000000 ) ) 
 REPRESENTATION_ITEM ( '' )  );
#55342=AXIS2_PLACEMENT_3D ( 'NONE', #17439, #46381, #62975 ) ;
#55345=CARTESIAN_POINT ( 'NONE',  ( 24.71169205770840094, -2.101182526020552999, -13.33689344900551887 ) ) ;
#55347=VERTEX_POINT ( 'NONE', #10697 ) ;
#55348=CARTESIAN_POINT ( 'NONE',  ( 35.00000000000000000, -3.033604067594490417, 12.38385022362084520 ) ) ;
#55350=CARTESIAN_POINT ( 'NONE',  ( -20.79170840334646542, 25.00000000000000000, -3.921648409140116698 ) ) ;
#55351=ORIENTED_EDGE ( 'NONE', *, *, #61600, .T. ) ;
#55352=ORIENTED_EDGE ( 'NONE', *, *, #28482, .F. ) ;
#55353=CARTESIAN_POINT ( 'NONE',  ( -37.00000000000000711, -8.927548052240958043, 8.295159312811820840 ) ) ;
#55354=VECTOR ( 'NONE', #60251, 1000.000000000000000 ) ;
#55356=FACE_OUTER_BOUND ( 'NONE', #16991, .T. ) ;
#55362=DIRECTION ( 'NONE',  ( 0.000000000000000000, -0.2618041379715496664, 0.9651210252299831094 ) ) ;
#55363=VERTEX_POINT ( 'NONE', #4429 ) ;
#55365=ORIENTED_EDGE ( 'NONE', *, *, #13241, .F. ) ;
#55366=AXIS2_PLACEMENT_3D ( 'NONE', #30808, #593, #16536 ) ;
#55368=CARTESIAN_POINT ( 'NONE',  ( 35.00000000000000000, 4.705694406421931860E-17, -3.469127814946512892E-15 ) ) ;
#55371=ADVANCED_FACE ( 'NONE', ( #60590 ), #25032, .T. ) ;
#55372=DIRECTION ( 'NONE',  ( -0.000000000000000000, -0.000000000000000000, -1.000000000000000000 ) ) ;
#55373=CYLINDRICAL_SURFACE ( 'NONE', #41827, 5.000000000000000888 ) ;
#55376=ORIENTED_EDGE ( 'NONE', *, *, #50377, .T. ) ;
#55377=AXIS2_PLACEMENT_3D ( 'NONE', #24685, #65243, #19711 ) ;
#55378=CIRCLE ( 'NONE', #13984, 5.000000000000000000 ) ;
#55379=DIRECTION ( 'NONE',  ( -1.000000000000000000, 0.000000000000000000, -0.000000000000000000 ) ) ;
#55384=CARTESIAN_POINT ( 'NONE',  ( 37.00000000000000711, 4.705694406421931860E-17, -3.469127814946512892E-15 ) ) ;
#55385=EDGE_CURVE ( 'NONE', #16289, #63348, #60265, .T. ) ;
#55387=DIRECTION ( 'NONE',  ( 0.000000000000000000, -0.01356324068817999114, 0.9999080150203989437 ) ) ;
#55389=CARTESIAN_POINT ( 'NONE',  ( 11.74548640120467979, 25.00000000000000000, -8.184666801472349817 ) ) ;
#55390=EDGE_CURVE ( 'NONE', #31183, #47524, #5080, .T. ) ;
#55391=VERTEX_POINT ( 'NONE', #15675 ) ;
#55395=AXIS2_PLACEMENT_3D ( 'NONE', #18154, #28135, #7175 ) ;
#55398=FACE_OUTER_BOUND ( 'NONE', #38944, .T. ) ;
#55399=DIRECTION ( 'NONE',  ( 1.000000000000000000, 0.000000000000000000, 0.000000000000000000 ) ) ;
#55400=ORIENTED_EDGE ( 'NONE', *, *, #43608, .T. ) ;
#55401=DIRECTION ( 'NONE',  ( -0.000000000000000000, -1.000000000000000000, -0.000000000000000000 ) ) ;
#55402=EDGE_CURVE ( 'NONE', #26919, #13695, #16564, .T. ) ;
#55403=VECTOR ( 'NONE', #60021, 1000.000000000000000 ) ;
#55405=VERTEX_POINT ( 'NONE', #20357 ) ;
#55406=DIRECTION ( 'NONE',  ( 1.000000000000000000, -0.000000000000000000, 0.000000000000000000 ) ) ;
#55407=DIRECTION ( 'NONE',  ( 1.000000000000000000, -0.000000000000000000, 0.000000000000000000 ) ) ;
#55409=EDGE_CURVE ( 'NONE', #36164, #36570, #55275, .T. ) ;
#55412=ORIENTED_EDGE ( 'NONE', *, *, #21092, .T. ) ;
#55413=CARTESIAN_POINT ( 'NONE',  ( -9.732421658388632935, -11.42231192723528999, -7.206575063207262488 ) ) ;
#55415=DIRECTION ( 'NONE',  ( 1.000000000000000000, 0.000000000000000000, 0.000000000000000000 ) ) ;
#55418=ADVANCED_FACE ( 'NONE', ( #34652 ), #44979, .T. ) ;
#55420=AXIS2_PLACEMENT_3D ( 'NONE', #44995, #20634, #681 ) ;
#55422=CARTESIAN_POINT ( 'NONE',  ( -15.49709305134071791, 8.465732809859909835, -10.51591234632406113 ) ) ;
#55423=DIRECTION ( 'NONE',  ( 0.000000000000000000, -0.1740410799127685426, -0.9847383929261604996 ) ) ;
#55425=EDGE_CURVE ( 'NONE', #46122, #27103, #29317, .T. ) ;
#55426=FACE_OUTER_BOUND ( 'NONE', #31065, .T. ) ;
#55427=CYLINDRICAL_SURFACE ( 'NONE', #23364, 5.683183579532407492 ) ;
#55432=AXIS2_PLACEMENT_3D ( 'NONE', #8545, #44431, #35102 ) ;
#55433=DIRECTION ( 'NONE',  ( -1.000000000000000000, 0.000000000000000000, 0.000000000000000000 ) ) ;
#55435=CIRCLE ( 'NONE', #7647, 5.000000000000000000 ) ;
#55437=ORIENTED_EDGE ( 'NONE', *, *, #31018, .T. ) ;
#55439=CARTESIAN_POINT ( 'NONE',  ( 11.80992030851978747, 11.76240988603115767, -2.380505417832655457 ) ) ;
#55440=CARTESIAN_POINT ( 'NONE',  ( 24.17956874138577916, -3.375310251640146308, 13.07616833750467045 ) ) ;
#55450=AXIS2_PLACEMENT_3D ( 'NONE', #26452, #1198, #51089 ) ;
#55451=ADVANCED_FACE ( 'NONE', ( #6719 ), #32290, .T. ) ;
#55454=CARTESIAN_POINT ( 'NONE',  ( 35.00000000000000000, 12.42372387097886310, 2.865935305911484932 ) ) ;
#55455=ORIENTED_EDGE ( 'NONE', *, *, #1904, .T. ) ;
#55457=CIRCLE ( 'NONE', #34183, 12.75000000000000178 ) ;
#55459=CARTESIAN_POINT ( 'NONE',  ( -36.00000000000000711, 5.865551165831237590, -11.32068061209289134 ) ) ;
#55460=CARTESIAN_POINT ( 'NONE',  ( 12.18790794593922655, 11.12778131062980336, -7.651757715589151410 ) ) ;
#55461=CARTESIAN_POINT ( 'NONE',  ( -37.00000000000000711, 0.000000000000000000, 0.000000000000000000 ) ) ;
#55463=CARTESIAN_POINT ( 'NONE',  ( 37.00000000000000711, 0.6593684648220483613, -12.73293890771483738 ) ) ;
#55465=CARTESIAN_POINT ( 'NONE',  ( 37.00000000000000711, 11.37311665002363270, 2.936739658819908616 ) ) ;
#55466=ORIENTED_EDGE ( 'NONE', *, *, #41882, .T. ) ;
#55467=CARTESIAN_POINT ( 'NONE',  ( -37.00000000000000711, -1.030638227056651424, 12.14284015767849567 ) ) ;
#55468=AXIS2_PLACEMENT_3D ( 'NONE', #5929, #14860, #45808 ) ;
#55470=CARTESIAN_POINT ( 'NONE',  ( -2.960381377298834327, -6.422849866723894685, 10.16751138944930588 ) ) ;
#55471=DIRECTION ( 'NONE',  ( 1.000000000000000000, 0.000000000000000000, 0.000000000000000000 ) ) ;
#55472=CARTESIAN_POINT ( 'NONE',  ( -35.00000000000000000, 4.426194442447240363, 11.35427606708807957 ) ) ;
#55473=CYLINDRICAL_SURFACE ( 'NONE', #54340, 5.000000000000000888 ) ;
#55474=DIRECTION ( 'NONE',  ( 0.000000000000000000, 0.04924826701373889726, 0.9987865678893281807 ) ) ;
#55475=EDGE_CURVE ( 'NONE', #18023, #3400, #22975, .T. ) ;
#55479=AXIS2_PLACEMENT_3D ( 'NONE', #16345, #5057, #30961 ) ;
#55480=FACE_OUTER_BOUND ( 'NONE', #43601, .T. ) ;
#55482=ADVANCED_FACE ( 'NONE', ( #21686 ), #52279, .T. ) ;
#55483=AXIS2_PLACEMENT_3D ( 'NONE', #52630, #17702, #42602 ) ;
#55486=CARTESIAN_POINT ( 'NONE',  ( 35.00000000000000000, -12.74613886779084382, 0.3137578094510532489 ) ) ;
#55489=ORIENTED_EDGE ( 'NONE', *, *, #62097, .T. ) ;
#55491=CYLINDRICAL_SURFACE ( 'NONE', #18254, 12.18649999999999878 ) ;
#55493=ADVANCED_FACE ( 'NONE', ( #20997 ), #46299, .T. ) ;
#55495=EDGE_CURVE ( 'NONE', #2301, #52651, #18712, .T. ) ;
#55496=CIRCLE ( 'NONE', #1360, 5.000000000000001776 ) ;
#55498=ORIENTED_EDGE ( 'NONE', *, *, #32474, .F. ) ;
#55499=FACE_OUTER_BOUND ( 'NONE', #23114, .T. ) ;
#55500=EDGE_CURVE ( 'NONE', #60956, #59860, #6070, .T. ) ;
#55501=VERTEX_POINT ( 'NONE', #61562 ) ;
#55502=DIRECTION ( 'NONE',  ( 0.000000000000000000, 0.2960891610144441022, 0.9551603052523501836 ) ) ;
#55503=DIRECTION ( 'NONE',  ( 1.000000000000000000, 0.000000000000000000, 0.000000000000000000 ) ) ;
#55504=CIRCLE ( 'NONE', #56611, 12.18650000000000055 ) ;
#55508=AXIS2_PLACEMENT_3D ( 'NONE', #36875, #11599, #8256 ) ;
#55512=VERTEX_POINT ( 'NONE', #7031 ) ;
#55514=VERTEX_POINT ( 'NONE', #16009 ) ;
#55517=VERTEX_POINT ( 'NONE', #57252 ) ;
#55519=DIRECTION ( 'NONE',  ( -0.000000000000000000, -0.000000000000000000, -1.000000000000000000 ) ) ;
#55520=ORIENTED_EDGE ( 'NONE', *, *, #59298, .T. ) ;
#55521=DIRECTION ( 'NONE',  ( 0.000000000000000000, -0.01356324068818000328, 0.9999080150203990547 ) ) ;
#55522=DIRECTION ( 'NONE',  ( 0.000000000000000000, 0.01356324068817998940, -0.9999080150203989437 ) ) ;
#55523=CARTESIAN_POINT ( 'NONE',  ( -37.00000000000000711, 0.000000000000000000, 0.000000000000000000 ) ) ;
#55530=ORIENTED_EDGE ( 'NONE', *, *, #9747, .T. ) ;
#55531=CIRCLE ( 'NONE', #15163, 12.18649999999999700 ) ;
#55533=ORIENTED_EDGE ( 'NONE', *, *, #49730, .F. ) ;
#55534=VERTEX_POINT ( 'NONE', #31323 ) ;
#55535=CARTESIAN_POINT ( 'NONE',  ( -35.00000000000000000, 10.23119532541083743, -7.608228585767614405 ) ) ;
#55537=VECTOR ( 'NONE', #18196, 1000.000000000000000 ) ;
#55543=EDGE_LOOP ( 'NONE', ( #37269, #63908, #50949, #59040 ) ) ;
#55546=( BOUNDED_CURVE ( )  B_SPLINE_CURVE ( 3, ( #10273, #44873, #65152, #19624 ),
 .UNSPECIFIED., .F., .F. ) 
 B_SPLINE_CURVE_WITH_KNOTS ( ( 4, 4 ),
 ( 1.570796326794896780, 1.601226737761092922 ),
 .UNSPECIFIED. ) 
 CURVE ( )  GEOMETRIC_REPRESENTATION_ITEM ( )  RATIONAL_B_SPLINE_CURVE ( ( 1.000000000000000000, 0.9999228339960630763, 0.9999228339960630763, 1.000000000000000000 ) ) 
 REPRESENTATION_ITEM ( '' )  );
#55548=CARTESIAN_POINT ( 'NONE',  ( 35.00000000000000000, 4.705694406421931860E-17, -3.469127814946512892E-15 ) ) ;
#55549=VECTOR ( 'NONE', #31008, 1000.000000000000000 ) ;
#55550=CARTESIAN_POINT ( 'NONE',  ( -2.729590200410152434, 12.79012149208910465, 4.331891749362731581 ) ) ;
#55551=ORIENTED_EDGE ( 'NONE', *, *, #10742, .F. ) ;
#55552=CARTESIAN_POINT ( 'NONE',  ( -27.65083951610984059, 12.87947692035696612, -4.055531763492385977 ) ) ;
#55555=CARTESIAN_POINT ( 'NONE',  ( 35.00000000000000000, 10.84030624090615724, 6.711949091238026632 ) ) ;
#55556=EDGE_CURVE ( 'NONE', #37018, #12385, #48427, .T. ) ;
#55557=VECTOR ( 'NONE', #56484, 1000.000000000000000 ) ;
#55560=VERTEX_POINT ( 'NONE', #26653 ) ;
#55567=EDGE_CURVE ( 'NONE', #60864, #45219, #50565, .T. ) ;
#55568=ADVANCED_FACE ( 'NONE', ( #2733 ), #48595, .T. ) ;
#55570=DIRECTION ( 'NONE',  ( 1.000000000000000000, 0.000000000000000000, 0.000000000000000000 ) ) ;
#55571=LINE ( 'NONE', #61515, #13133 ) ;
#55573=DIRECTION ( 'NONE',  ( 0.000000000000000000, 0.01356324068817992175, -0.9999080150203990547 ) ) ;
#55574=EDGE_CURVE ( 'NONE', #57258, #65189, #27979, .T. ) ;
#55579=CARTESIAN_POINT ( 'NONE',  ( -35.00000000000000000, 0.000000000000000000, 0.000000000000000000 ) ) ;
#55582=CIRCLE ( 'NONE', #20548, 5.000000000000000888 ) ;
#55584=CIRCLE ( 'NONE', #35388, 4.999999999999999112 ) ;
#55585=AXIS2_PLACEMENT_3D ( 'NONE', #37594, #26625, #52248 ) ;
#55586=ORIENTED_EDGE ( 'NONE', *, *, #50264, .T. ) ;
#55588=ADVANCED_FACE ( 'NONE', ( #22666 ), #63856, .T. ) ;
#55589=ORIENTED_EDGE ( 'NONE', *, *, #51994, .T. ) ;
#55590=CARTESIAN_POINT ( 'NONE',  ( -29.68541646480307250, -1.416020129149132334, 13.42553116244733680 ) ) ;
#55591=CARTESIAN_POINT ( 'NONE',  ( 35.00000000000000000, 7.817492529713852889, -9.348667969174437431 ) ) ;
#55592=DIRECTION ( 'NONE',  ( 0.000000000000000000, -0.01356324068817999114, 0.9999080150203989437 ) ) ;
#55595=VERTEX_POINT ( 'NONE', #8674 ) ;
#55600=CARTESIAN_POINT ( 'NONE',  ( 36.00000000000000711, -8.496612874013091954, 9.506317355798456603 ) ) ;
#55601=CIRCLE ( 'NONE', #19526, 5.000000000000000888 ) ;
#55602=CARTESIAN_POINT ( 'NONE',  ( -37.00000000000000711, -3.704519465651228138, -11.60979404548638705 ) ) ;
#55603=ORIENTED_EDGE ( 'NONE', *, *, #19483, .F. ) ;
#55604=DIRECTION ( 'NONE',  ( 1.000000000000000000, 0.000000000000000000, -0.000000000000000000 ) ) ;
#55606=VERTEX_POINT ( 'NONE', #33617 ) ;
#55607=AXIS2_PLACEMENT_3D ( 'NONE', #53649, #18405, #37683 ) ;
#55609=CIRCLE ( 'NONE', #5693, 5.000000000000000000 ) ;
#55611=CARTESIAN_POINT ( 'NONE',  ( 35.00000000000000000, -11.74226168163341555, -0.3025107581130825896 ) ) ;
#55613=VERTEX_POINT ( 'NONE', #13331 ) ;
#55614=CARTESIAN_POINT ( 'NONE',  ( -36.00000000000000711, -10.39746860227885428, -7.379373053628983214 ) ) ;
#55615=ORIENTED_EDGE ( 'NONE', *, *, #8900, .T. ) ;
#55616=CARTESIAN_POINT ( 'NONE',  ( 35.00000000000000000, 6.307491713049029336, -9.908974237959670361 ) ) ;
#55617=ORIENTED_EDGE ( 'NONE', *, *, #23767, .F. ) ;
#55621=LINE ( 'NONE', #10057, #47142 ) ;
#55622=CARTESIAN_POINT ( 'NONE',  ( 19.28625800530496903, -1.699513388191772778, 11.87904264843580471 ) ) ;
#55623=AXIS2_PLACEMENT_3D ( 'NONE', #54133, #64106, #43157 ) ;
#55625=CARTESIAN_POINT ( 'NONE',  ( -29.43980975494970309, -3.641506875706034041, -12.99959336572439561 ) ) ;
#55627=PLANE ( 'NONE',  #23734 ) ;
#55628=CARTESIAN_POINT ( 'NONE',  ( 7.228533150787943562, -7.187350446428427020, 11.43552089456373899 ) ) ;
#55629=ORIENTED_EDGE ( 'NONE', *, *, #43589, .T. ) ;
#55630=CARTESIAN_POINT ( 'NONE',  ( -35.00000000000000000, 11.74614673114903951, 0.01609748574465447862 ) ) ;
#55631=EDGE_CURVE ( 'NONE', #48262, #19477, #61409, .T. ) ;
#55632=ORIENTED_EDGE ( 'NONE', *, *, #24711, .T. ) ;
#55634=VERTEX_POINT ( 'NONE', #63211 ) ;
#55635=ORIENTED_EDGE ( 'NONE', *, *, #28283, .F. ) ;
#55636=CARTESIAN_POINT ( 'NONE',  ( -35.00000000000000000, 1.488153103997124971, -11.65150730582933036 ) ) ;
#55639=DIRECTION ( 'NONE',  ( 0.000000000000000000, 0.9246979985058709772, 0.3807014730195252272 ) ) ;
#55640=CIRCLE ( 'NONE', #16328, 12.18649999999999878 ) ;
#55643=CARTESIAN_POINT ( 'NONE',  ( 35.00000000000000000, -6.307491713048959170, 9.908974237959705889 ) ) ;
#55644=VECTOR ( 'NONE', #64702, 1000.000000000000000 ) ;
#55645=ORIENTED_EDGE ( 'NONE', *, *, #33773, .T. ) ;
#55646=CARTESIAN_POINT ( 'NONE',  ( -32.00000000000000000, 15.00000000000000000, 0.000000000000000000 ) ) ;
#55649=CARTESIAN_POINT ( 'NONE',  ( -37.00000000000000711, 9.913596905230114942, 8.017674001891819557 ) ) ;
#55650=EDGE_CURVE ( 'NONE', #1032, #30904, #16793, .T. ) ;
#55652=AXIS2_PLACEMENT_3D ( 'NONE', #37343, #57653, #17406 ) ;
#55653=CARTESIAN_POINT ( 'NONE',  ( -37.00000000000000711, 4.237174932027226504, 12.02534193257722528 ) ) ;
#55656=DIRECTION ( 'NONE',  ( -0.000000000000000000, -1.000000000000000000, -0.000000000000000000 ) ) ;
#55660=CARTESIAN_POINT ( 'NONE',  ( 37.00000000000000711, 0.7214809346830272085, 11.72397916322010936 ) ) ;
#55661=DIRECTION ( 'NONE',  ( 1.000000000000000000, 0.000000000000000000, 0.000000000000000000 ) ) ;
#55662=DIRECTION ( 'NONE',  ( 0.000000000000000000, 0.01356324068817998940, -0.9999080150203990547 ) ) ;
#55664=LINE ( 'NONE', #19765, #33215 ) ;
#55667=ORIENTED_EDGE ( 'NONE', *, *, #38918, .T. ) ;
#55669=DIRECTION ( 'NONE',  ( -1.000000000000000000, 0.000000000000000000, 0.000000000000000000 ) ) ;
#55670=ORIENTED_EDGE ( 'NONE', *, *, #28003, .T. ) ;
#55671=VECTOR ( 'NONE', #47553, 1000.000000000000000 ) ;
#55672=EDGE_CURVE ( 'NONE', #34466, #50843, #53591, .T. ) ;
#55673=CIRCLE ( 'NONE', #60988, 12.74999999999999822 ) ;
#55675=VERTEX_POINT ( 'NONE', #7694 ) ;
#55680=DIRECTION ( 'NONE',  ( 0.1034490876700550344, -0.000000000000000000, 0.9946347501772866417 ) ) ;
#55684=CARTESIAN_POINT ( 'NONE',  ( 24.18120799216340089, -3.372877268056853506, -13.07685726758646538 ) ) ;
#55686=ORIENTED_EDGE ( 'NONE', *, *, #6188, .T. ) ;
#55689=DIRECTION ( 'NONE',  ( -1.000000000000000000, 0.000000000000000000, 0.000000000000000000 ) ) ;
#55690=CIRCLE ( 'NONE', #37597, 12.18650000000000055 ) ;
#55691=EDGE_LOOP ( 'NONE', ( #33339, #14403, #38847, #20416 ) ) ;
#55692=VERTEX_POINT ( 'NONE', #48286 ) ;
#55695=AXIS2_PLACEMENT_3D ( 'NONE', #14828, #10507, #35114 ) ;
#55696=CYLINDRICAL_SURFACE ( 'NONE', #4664, 12.74999999999999822 ) ;
#55699=CARTESIAN_POINT ( 'NONE',  ( 35.00000000000000000, 4.705694406421931860E-17, -3.469127814946512892E-15 ) ) ;
#55701=VERTEX_POINT ( 'NONE', #23980 ) ;
#55702=EDGE_CURVE ( 'NONE', #20343, #6763, #6225, .T. ) ;
#55703=ORIENTED_EDGE ( 'NONE', *, *, #41970, .T. ) ;
#55704=ADVANCED_FACE ( 'NONE', ( #54573 ), #51470, .T. ) ;
#55706=ORIENTED_EDGE ( 'NONE', *, *, #45374, .T. ) ;
#55707=AXIS2_PLACEMENT_3D ( 'NONE', #61011, #21080, #30081 ) ;
#55709=ORIENTED_EDGE ( 'NONE', *, *, #24265, .T. ) ;
#55710=PLANE ( 'NONE',  #18998 ) ;
#55711=CARTESIAN_POINT ( 'NONE',  ( 10.16591523190729163, 8.042301321965682703, -8.910861195510744182 ) ) ;
#55713=CARTESIAN_POINT ( 'NONE',  ( 18.39714084132998195, 4.205996179170882421, 11.25142999110358133 ) ) ;
#55715=DIRECTION ( 'NONE',  ( -1.000000000000000000, 0.000000000000000000, -0.000000000000000000 ) ) ;
#55716=AXIS2_PLACEMENT_3D ( 'NONE', #39509, #59802, #65102 ) ;
#55717=ADVANCED_FACE ( 'NONE', ( #15523 ), #5236, .T. ) ;
#55722=CARTESIAN_POINT ( 'NONE',  ( -37.00000000000000711, 0.000000000000000000, 0.000000000000000000 ) ) ;
#55725=DIRECTION ( 'NONE',  ( -1.000000000000000000, 0.000000000000000000, 0.000000000000000000 ) ) ;
#55726=CARTESIAN_POINT ( 'NONE',  ( 3.708583301347321726, -10.51590576721076964, 5.781912091200419823 ) ) ;
#55727=DIRECTION ( 'NONE',  ( 0.8317381556525372810, -0.5551681190699946367, 0.000000000000000000 ) ) ;
#55728=EDGE_CURVE ( 'NONE', #7867, #9912, #17905, .T. ) ;
#55729=CARTESIAN_POINT ( 'NONE',  ( 23.75192053619575461, -3.113835264533937774, -13.14002899460337304 ) ) ;
#55732=ORIENTED_EDGE ( 'NONE', *, *, #12383, .F. ) ;
#55733=AXIS2_PLACEMENT_3D ( 'NONE', #10619, #39906, #25602 ) ;
#55735=DIRECTION ( 'NONE',  ( 1.000000000000000000, 0.000000000000000000, 0.000000000000000000 ) ) ;
#55736=CIRCLE ( 'NONE', #21807, 12.18649999999999878 ) ;
#55737=DIRECTION ( 'NONE',  ( 0.000000000000000000, 0.01356324068817998940, -0.9999080150203990547 ) ) ;
#55740=VERTEX_POINT ( 'NONE', #896 ) ;
#55741=CARTESIAN_POINT ( 'NONE',  ( -18.17455973634320898, -4.727991781583684272, -12.64561680075576255 ) ) ;
#55742=CARTESIAN_POINT ( 'NONE',  ( 26.73134588528545663, 13.02586532392652785, 3.554799201164403843 ) ) ;
#55746=CARTESIAN_POINT ( 'NONE',  ( -2.532614230583026593, 25.00000000000000000, 10.89930238848911337 ) ) ;
#55747=CARTESIAN_POINT ( 'NONE',  ( 37.00000000000000711, -11.30684963584392477, -4.545979934229371189 ) ) ;
#55748=FACE_OUTER_BOUND ( 'NONE', #52377, .T. ) ;
#55749=EDGE_LOOP ( 'NONE', ( #19445, #65614, #60099, #10774 ) ) ;
#55751=EDGE_CURVE ( 'NONE', #50088, #10101, #1894, .T. ) ;
#55753=EDGE_LOOP ( 'NONE', ( #29136, #31061, #23373, #65624 ) ) ;
#55754=CARTESIAN_POINT ( 'NONE',  ( -35.00000000000000000, -8.551552972817024312, -8.052525312709976291 ) ) ;
#55755=DIRECTION ( 'NONE',  ( 0.000000000000000000, -0.01356324068817992175, 0.9999080150203990547 ) ) ;
#55756=CARTESIAN_POINT ( 'NONE',  ( 22.57855258442564761, -4.427776684447072952, -11.15324139578564910 ) ) ;
#55757=CARTESIAN_POINT ( 'NONE',  ( 8.498256429135825130, 5.239437556988991496, -12.44347423756361160 ) ) ;
#55759=CARTESIAN_POINT ( 'NONE',  ( 35.00000000000000000, 4.705694406421931860E-17, -3.469127814946512892E-15 ) ) ;
#55763=CYLINDRICAL_SURFACE ( 'NONE', #49113, 5.000000000000000888 ) ;
#55765=DIRECTION ( 'NONE',  ( 0.000000000000000000, 0.01356324068817998940, -0.9999080150203990547 ) ) ;
#55767=CARTESIAN_POINT ( 'NONE',  ( -35.00000000000000000, 0.000000000000000000, 0.000000000000000000 ) ) ;
#55768=EDGE_CURVE ( 'NONE', #9488, #64485, #58253, .T. ) ;
#55769=DIRECTION ( 'NONE',  ( 0.000000000000000000, 0.01356324068817992522, -0.9999080150203990547 ) ) ;
#55772=CARTESIAN_POINT ( 'NONE',  ( 35.00000000000000000, 0.8294751490779324055, -12.15823808070322798 ) ) ;
#55773=EDGE_CURVE ( 'NONE', #30777, #11634, #51904, .T. ) ;
#55781=FACE_OUTER_BOUND ( 'NONE', #65147, .T. ) ;
#55782=DIRECTION ( 'NONE',  ( 0.000000000000000000, 0.9937233664769765662, -0.1118654143051581590 ) ) ;
#55784=DIRECTION ( 'NONE',  ( -0.000000000000000000, -0.000000000000000000, -1.000000000000000000 ) ) ;
#55786=CARTESIAN_POINT ( 'NONE',  ( -37.00000000000000711, 10.63508530065528923, -4.986700593229593359 ) ) ;
#55788=DIRECTION ( 'NONE',  ( 1.000000000000000000, 0.000000000000000000, 0.000000000000000000 ) ) ;
#55791=ADVANCED_FACE ( 'NONE', ( #17831 ), #42096, .T. ) ;
#55800=ADVANCED_FACE ( 'NONE', ( #53426 ), #2218, .T. ) ;
#55801=AXIS2_PLACEMENT_3D ( 'NONE', #42953, #63232, #53270 ) ;
#55803=ORIENTED_EDGE ( 'NONE', *, *, #39001, .T. ) ;
#55805=EDGE_CURVE ( 'NONE', #43228, #2417, #5140, .T. ) ;
#55807=CARTESIAN_POINT ( 'NONE',  ( -35.00000000000000000, -12.00000000000000000, 0.000000000000000000 ) ) ;
#55809=CARTESIAN_POINT ( 'NONE',  ( -16.78314026428192207, 7.533399764774538987, -11.20369790611374228 ) ) ;
#55810=ADVANCED_FACE ( 'NONE', ( #6882 ), #63365, .T. ) ;
#55812=CARTESIAN_POINT ( 'NONE',  ( -35.00000000000000000, -8.573591947375380329, 8.029056188533655103 ) ) ;
#55813=VERTEX_POINT ( 'NONE', #38096 ) ;
#55814=CARTESIAN_POINT ( 'NONE',  ( 36.00000000000000711, -4.561791185930328396, 11.90598845858538013 ) ) ;
#55819=CARTESIAN_POINT ( 'NONE',  ( 29.51976981715666781, -4.571419055710073565, 11.09513982864076276 ) ) ;
#55820=DIRECTION ( 'NONE',  ( 1.000000000000000000, 0.000000000000000000, 0.000000000000000000 ) ) ;
#55822=ORIENTED_EDGE ( 'NONE', *, *, #13626, .F. ) ;
#55824=ORIENTED_EDGE ( 'NONE', *, *, #10696, .T. ) ;
#55827=CARTESIAN_POINT ( 'NONE',  ( 28.78308862069595264, -9.765596609978194564, 6.977306409396123676 ) ) ;
#55828=DIRECTION ( 'NONE',  ( 0.000000000000000000, 0.01356324068817992175, -0.9999080150203990547 ) ) ;
#55830=EDGE_CURVE ( 'NONE', #57845, #50922, #27963, .T. ) ;
#55832=ORIENTED_EDGE ( 'NONE', *, *, #23159, .T. ) ;
#55834=ORIENTED_EDGE ( 'NONE', *, *, #10886, .T. ) ;
#55836=DIRECTION ( 'NONE',  ( 0.000000000000000000, -0.7617968321374944951, -0.6478160128811867313 ) ) ;
#55837=CYLINDRICAL_SURFACE ( 'NONE', #56423, 12.74999999999999822 ) ;
#55838=CARTESIAN_POINT ( 'NONE',  ( -27.45775109278351067, 10.51123867646838583, -8.471355351200609007 ) ) ;
#55839=DIRECTION ( 'NONE',  ( 0.000000000000000000, 0.01356324068817992695, -0.9999080150203990547 ) ) ;
#55842=VERTEX_POINT ( 'NONE', #32766 ) ;
#55843=EDGE_CURVE ( 'NONE', #45661, #36765, #63542, .T. ) ;
#55844=CARTESIAN_POINT ( 'NONE',  ( -7.959843492831086387, -7.020518735649992514, -9.756886859334462869 ) ) ;
#55845=VERTEX_POINT ( 'NONE', #43089 ) ;
#55847=EDGE_CURVE ( 'NONE', #27703, #17490, #60366, .T. ) ;
#55848=EDGE_LOOP ( 'NONE', ( #51984, #1715, #38105, #13589 ) ) ;
#55850=ORIENTED_EDGE ( 'NONE', *, *, #11648, .T. ) ;
#55851=CARTESIAN_POINT ( 'NONE',  ( 35.00000000000000000, -10.32377448871663006, 6.475373545682407972 ) ) ;
#55852=CARTESIAN_POINT ( 'NONE',  ( 5.417119996861458731, -9.515710175651925340, -9.580509969479626520 ) ) ;
#55854=ORIENTED_EDGE ( 'NONE', *, *, #7110, .T. ) ;
#55855=VERTEX_POINT ( 'NONE', #43409 ) ;
#55859=DIRECTION ( 'NONE',  ( -1.000000000000000000, -0.000000000000000000, 0.000000000000000000 ) ) ;
#55861=EDGE_LOOP ( 'NONE', ( #53220, #34662, #55028, #33105 ) ) ;
#55862=VERTEX_POINT ( 'NONE', #57761 ) ;
#55866=CARTESIAN_POINT ( 'NONE',  ( -34.00000000000000000, 1.836970198721036590E-16, 0.000000000000000000 ) ) ;
#55867=DIRECTION ( 'NONE',  ( 0.000000000000000000, -0.01356324068817998940, 0.9999080150203990547 ) ) ;
#55868=VERTEX_POINT ( 'NONE', #63688 ) ;
#55869=CIRCLE ( 'NONE', #26146, 12.74999999999999822 ) ;
#55870=DIRECTION ( 'NONE',  ( 0.000000000000000000, 0.01356324068817991828, -0.9999080150203990547 ) ) ;
#55871=AXIS2_PLACEMENT_3D ( 'NONE', #11788, #32070, #2511 ) ;
#55873=LINE ( 'NONE', #40567, #10456 ) ;
#55874=CARTESIAN_POINT ( 'NONE',  ( -3.363016410184096028, 10.07324327587569002, 8.995337225020698213 ) ) ;
#55875=ORIENTED_EDGE ( 'NONE', *, *, #2730, .T. ) ;
#55880=VECTOR ( 'NONE', #9720, 1000.000000000000000 ) ;
#55881=VERTEX_POINT ( 'NONE', #17515 ) ;
#55882=DIRECTION ( 'NONE',  ( 0.000000000000000000, 0.01356324068817998940, -0.9999080150203990547 ) ) ;
#55883=EDGE_CURVE ( 'NONE', #3051, #33198, #6235, .T. ) ;
#55885=CARTESIAN_POINT ( 'NONE',  ( -25.32301808527470044, -7.777392180360524598, 11.03968484280607676 ) ) ;
#55887=EDGE_CURVE ( 'NONE', #65451, #20070, #13612, .T. ) ;
#55888=FACE_OUTER_BOUND ( 'NONE', #49576, .T. ) ;
#55889=CARTESIAN_POINT ( 'NONE',  ( 37.00000000000000711, 4.705694406421931860E-17, -3.469127814946512892E-15 ) ) ;
#55890=ORIENTED_EDGE ( 'NONE', *, *, #55847, .F. ) ;
#55892=DIRECTION ( 'NONE',  ( 1.000000000000000000, -0.000000000000000000, 0.000000000000000000 ) ) ;
#55894=CARTESIAN_POINT ( 'NONE',  ( 22.08055403950514517, -12.79402759897448583, -4.312350172591147057 ) ) ;
#55895=DIRECTION ( 'NONE',  ( 0.000000000000000000, 0.01356324068817998940, -0.9999080150203990547 ) ) ;
#55900=EDGE_CURVE ( 'NONE', #54137, #39298, #27807, .T. ) ;
#55902=ORIENTED_EDGE ( 'NONE', *, *, #53341, .F. ) ;
#55903=ADVANCED_FACE ( 'NONE', ( #38775 ), #54407, .T. ) ;
#55904=CIRCLE ( 'NONE', #50601, 12.18649999999999878 ) ;
#55905=ORIENTED_EDGE ( 'NONE', *, *, #43667, .T. ) ;
#55912=EDGE_LOOP ( 'NONE', ( #22332, #19852, #20004, #47267 ) ) ;
#55913=ORIENTED_EDGE ( 'NONE', *, *, #27839, .F. ) ;
#55914=CARTESIAN_POINT ( 'NONE',  ( 29.70345330596045130, -6.346709636665306853, 10.23243518362844107 ) ) ;
#55919=CARTESIAN_POINT ( 'NONE',  ( -17.71957339262799280, 3.746001421221477834, -11.40215424527250754 ) ) ;
#55921=ORIENTED_EDGE ( 'NONE', *, *, #55390, .F. ) ;
#55922=( BOUNDED_CURVE ( )  B_SPLINE_CURVE ( 3, ( #41874, #37199, #41205, #6004 ),
 .UNSPECIFIED., .F., .F. ) 
 B_SPLINE_CURVE_WITH_KNOTS ( ( 4, 4 ),
 ( 4.761198528795062224, 4.801918529528334645 ),
 .UNSPECIFIED. ) 
 CURVE ( )  GEOMETRIC_REPRESENTATION_ITEM ( )  RATIONAL_B_SPLINE_CURVE ( ( 1.000000000000000000, 0.9998618282348130659, 0.9998618282348130659, 1.000000000000000000 ) ) 
 REPRESENTATION_ITEM ( '' )  );
#55923=CARTESIAN_POINT ( 'NONE',  ( 35.00000000000000000, 11.16627499335655216, 3.645068577060061266 ) ) ;
#55925=CARTESIAN_POINT ( 'NONE',  ( 145.1370849898475797, 3.309064568108273190E-14, 0.000000000000000000 ) ) ;
#55929=ORIENTED_EDGE ( 'NONE', *, *, #30165, .F. ) ;
#55931=ORIENTED_EDGE ( 'NONE', *, *, #25701, .F. ) ;
#55933=EDGE_CURVE ( 'NONE', #9681, #48363, #32719, .T. ) ;
#55934=CYLINDRICAL_SURFACE ( 'NONE', #59604, 5.000000000000000888 ) ;
#55938=CARTESIAN_POINT ( 'NONE',  ( 10.62696271159157568, 0.6044469518327795221, 11.98545746328775863 ) ) ;
#55939=DIRECTION ( 'NONE',  ( 1.000000000000000000, 0.000000000000000000, -0.000000000000000000 ) ) ;
#55941=CARTESIAN_POINT ( 'NONE',  ( -17.29244623348158783, 2.525873743887551814, -13.26159725786978072 ) ) ;
#55942=ORIENTED_EDGE ( 'NONE', *, *, #29547, .T. ) ;
#55944=ORIENTED_EDGE ( 'NONE', *, *, #52349, .F. ) ;
#55945=DIRECTION ( 'NONE',  ( -1.000000000000000000, 0.000000000000000000, 0.000000000000000000 ) ) ;
#55946=EDGE_LOOP ( 'NONE', ( #8606, #19859, #3628, #56345 ) ) ;
#55947=CARTESIAN_POINT ( 'NONE',  ( 37.00000000000000711, 9.512294188640899151, -6.891188680298859559 ) ) ;
#55948=ORIENTED_EDGE ( 'NONE', *, *, #42392, .F. ) ;
#55950=CARTESIAN_POINT ( 'NONE',  ( 35.00000000000000000, 10.49626516989280844, 7.238157050195512809 ) ) ;
#55952=CARTESIAN_POINT ( 'NONE',  ( 37.00000000000000711, -5.391785509271032062, -10.43555801961473861 ) ) ;
#55953=EDGE_CURVE ( 'NONE', #55012, #59346, #65621, .T. ) ;
#55954=CARTESIAN_POINT ( 'NONE',  ( 3.780834652287974773, 8.352030633203074927, -10.60629927458383470 ) ) ;
#55955=ORIENTED_EDGE ( 'NONE', *, *, #62441, .T. ) ;
#55959=ORIENTED_EDGE ( 'NONE', *, *, #36964, .F. ) ;
#55961=DIRECTION ( 'NONE',  ( 1.000000000000000000, 0.000000000000000000, -0.000000000000000000 ) ) ;
#55963=B_SPLINE_CURVE_WITH_KNOTS ( 'NONE', 3,
 ( #12772, #6499, #63000, #17462, #37734, #52391 ),
 .UNSPECIFIED., .F., .F.,
 ( 4, 2, 4 ),
 ( 0.004590869839051449006, 0.006605404212303630021, 0.008619938585555811036 ),
 .UNSPECIFIED. ) ;
#55966=CARTESIAN_POINT ( 'NONE',  ( 35.00000000000000000, -11.67026961469347768, -4.564151185897032725 ) ) ;
#55970=DIRECTION ( 'NONE',  ( 1.000000000000000000, 0.000000000000000000, -0.000000000000000000 ) ) ;
#55971=LINE ( 'NONE', #9755, #61185 ) ;
#55974=CARTESIAN_POINT ( 'NONE',  ( 18.31241578173652940, -9.284453232853790539, 9.826491150957114229 ) ) ;
#55976=VERTEX_POINT ( 'NONE', #14458 ) ;
#55977=AXIS2_PLACEMENT_3D ( 'NONE', #3478, #62974, #53344 ) ;
#55979=CARTESIAN_POINT ( 'NONE',  ( -1.734723475976807094E-15, -3.469446951953614189E-15, 12.00000000000000178 ) ) ;
#55980=CARTESIAN_POINT ( 'NONE',  ( -35.00000000000000000, 0.000000000000000000, 0.000000000000000000 ) ) ;
#55981=ORIENTED_EDGE ( 'NONE', *, *, #18836, .T. ) ;
#55982=CARTESIAN_POINT ( 'NONE',  ( -18.56118279717487951, 4.671099544038118445, 11.05659470145910639 ) ) ;
#55983=DIRECTION ( 'NONE',  ( 0.000000000000000000, 0.01356324068817998940, -0.9999080150203989437 ) ) ;
#55987=ORIENTED_EDGE ( 'NONE', *, *, #61191, .F. ) ;
#55988=EDGE_CURVE ( 'NONE', #39732, #18175, #24130, .T. ) ;
#55989=VERTEX_POINT ( 'NONE', #54732 ) ;
#55990=CARTESIAN_POINT ( 'NONE',  ( 35.00000000000000000, 4.705694406421931860E-17, -3.469127814946512892E-15 ) ) ;
#55992=CARTESIAN_POINT ( 'NONE',  ( -35.00000000000000000, -12.12087942037210553, 1.262958560998716617 ) ) ;
#55994=CARTESIAN_POINT ( 'NONE',  ( -21.24030193723618609, 25.00000000000000000, -5.230344621181295395 ) ) ;
#55996=DIRECTION ( 'NONE',  ( 0.000000000000000000, 0.1387779952735747890, -0.9903235168508558450 ) ) ;
#55997=CYLINDRICAL_SURFACE ( 'NONE', #30843, 12.18649999999999878 ) ;
#55998=ORIENTED_EDGE ( 'NONE', *, *, #47388, .F. ) ;
#56000=EDGE_CURVE ( 'NONE', #58250, #29408, #29129, .T. ) ;
#56001=EDGE_LOOP ( 'NONE', ( #20789, #4257, #33337, #25268 ) ) ;
#56003=ORIENTED_EDGE ( 'NONE', *, *, #10043, .T. ) ;
#56004=ORIENTED_EDGE ( 'NONE', *, *, #8715, .T. ) ;
#56007=EDGE_CURVE ( 'NONE', #63926, #42135, #22111, .T. ) ;
#56010=CARTESIAN_POINT ( 'NONE',  ( -35.00000000000000000, 2.080187960898735255, -12.57916205664478859 ) ) ;
#56012=ORIENTED_EDGE ( 'NONE', *, *, #30380, .F. ) ;
#56013=ORIENTED_EDGE ( 'NONE', *, *, #14598, .T. ) ;
#56016=EDGE_LOOP ( 'NONE', ( #10630, #62107, #8967, #26073 ) ) ;
#56017=CARTESIAN_POINT ( 'NONE',  ( 26.08439714455133185, 25.00000000000000000, 3.743551691817327942 ) ) ;
#56023=CARTESIAN_POINT ( 'NONE',  ( -9.097493606629301510, -2.480532761269033770, -11.74397547306413259 ) ) ;
#56026=ORIENTED_EDGE ( 'NONE', *, *, #64842, .T. ) ;
#56028=PLANE ( 'NONE',  #41409 ) ;
#56029=CIRCLE ( 'NONE', #20992, 12.18650000000000411 ) ;
#56030=CYLINDRICAL_SURFACE ( 'NONE', #46873, 5.000000000000000888 ) ;
#56033=CARTESIAN_POINT ( 'NONE',  ( -37.00000000000000711, 7.717887834988368390, -8.854740511458771834 ) ) ;
#56034=AXIS2_PLACEMENT_3D ( 'NONE', #49345, #58310, #58658 ) ;
#56036=CARTESIAN_POINT ( 'NONE',  ( 37.00000000000000711, 10.99909370905164430, 5.246972444133898072 ) ) ;
#56040=DIRECTION ( 'NONE',  ( 0.000000000000000000, -0.01356324068817998940, 0.9999080150203990547 ) ) ;
#56041=DIRECTION ( 'NONE',  ( 1.000000000000000000, -0.000000000000000000, 0.000000000000000000 ) ) ;
#56042=FACE_OUTER_BOUND ( 'NONE', #12461, .T. ) ;
#56044=EDGE_CURVE ( 'NONE', #38122, #58003, #35058, .T. ) ;
#56049=VERTEX_POINT ( 'NONE', #15456 ) ;
#56054=FACE_OUTER_BOUND ( 'NONE', #32124, .T. ) ;
#56056=LINE ( 'NONE', #36087, #33119 ) ;
#56057=CIRCLE ( 'NONE', #32692, 12.18650000000000055 ) ;
#56058=EDGE_CURVE ( 'NONE', #42804, #21758, #10458, .T. ) ;
#56059=CARTESIAN_POINT ( 'NONE',  ( 11.74548640120467979, -8.775604215601116920, -8.184666801472349817 ) ) ;
#56060=B_SPLINE_CURVE_WITH_KNOTS ( 'NONE', 3,
 ( #41112, #62375, #16836, #56086, #15836, #1233, #41437, #31481, #36114, #36796, #31159, #51778, #25849, #52442, #51121, #26484, #46138, #61728, #57091, #6880 ),
 .UNSPECIFIED., .F., .F.,
 ( 4, 2, 2, 2, 2, 2, 2, 2, 2, 4 ),
 ( 0.000000000000000000, 0.001253695096289122709, 0.001880542644433685039, 0.002507390192578247152, 0.003761085288867371812, 0.005014780385156495171, 0.006268475481445620265, 0.007522170577734745359, 0.008775865674023870452, 0.01002956077031299555 ),
 .UNSPECIFIED. ) ;
#56061=VERTEX_POINT ( 'NONE', #19804 ) ;
#56064=AXIS2_PLACEMENT_3D ( 'NONE', #52768, #7194, #23487 ) ;
#56067=CARTESIAN_POINT ( 'NONE',  ( 8.437200413559441614, 4.476360154859202467, -12.73625532737110966 ) ) ;
#56068=CARTESIAN_POINT ( 'NONE',  ( -17.50119111604729483, 2.686101418262018647, 13.23107945010674413 ) ) ;
#56070=VECTOR ( 'NONE', #61327, 1000.000000000000000 ) ;
#56071=ORIENTED_EDGE ( 'NONE', *, *, #39569, .T. ) ;
#56072=DIRECTION ( 'NONE',  ( -1.000000000000000000, 0.000000000000000000, 0.000000000000000000 ) ) ;
#56080=VERTEX_POINT ( 'NONE', #15767 ) ;
#56082=CARTESIAN_POINT ( 'NONE',  ( 11.37704067788454942, 11.83906243856773344, -1.962618476695794589 ) ) ;
#56083=DIRECTION ( 'NONE',  ( 1.000000000000000000, 0.000000000000000000, 0.000000000000000000 ) ) ;
#56084=ORIENTED_EDGE ( 'NONE', *, *, #52671, .F. ) ;
#56085=ORIENTED_EDGE ( 'NONE', *, *, #53772, .F. ) ;
#56086=CARTESIAN_POINT ( 'NONE',  ( 27.22053583440688840, -12.68463422843485056, 4.622893925193950260 ) ) ;
#56087=ORIENTED_EDGE ( 'NONE', *, *, #13054, .F. ) ;
#56088=CARTESIAN_POINT ( 'NONE',  ( 24.73855084333399290, -8.970947471680776886, -7.973041315719463284 ) ) ;
#56089=CARTESIAN_POINT ( 'NONE',  ( 35.00000000000000000, 4.705694406421931860E-17, -3.469127814946512892E-15 ) ) ;
#56092=CARTESIAN_POINT ( 'NONE',  ( 9.650011408859196393, 13.48023745212357838, -0.7481333718491257612 ) ) ;
#56097=VECTOR ( 'NONE', #8840, 1000.000000000000000 ) ;
#56098=DIRECTION ( 'NONE',  ( 1.000000000000000000, 0.000000000000000000, 0.000000000000000000 ) ) ;
#56101=CARTESIAN_POINT ( 'NONE',  ( -37.00000000000000711, 0.000000000000000000, 0.000000000000000000 ) ) ;
#56105=CIRCLE ( 'NONE', #14647, 5.000000000000001776 ) ;
#56106=EDGE_CURVE ( 'NONE', #4994, #46189, #10475, .T. ) ;
#56108=CARTESIAN_POINT ( 'NONE',  ( 11.74548640120467979, 10.73597826697114677, -8.184666801472349817 ) ) ;
#56110=CIRCLE ( 'NONE', #64601, 5.000000000000000888 ) ;
#56111=( BOUNDED_CURVE ( )  B_SPLINE_CURVE ( 3, ( #32287, #52605, #47596, #2039 ),
 .UNSPECIFIED., .F., .F. ) 
 B_SPLINE_CURVE_WITH_KNOTS ( ( 4, 4 ),
 ( 1.213047816902216081, 1.252925267387245523 ),
 .UNSPECIFIED. ) 
 CURVE ( )  GEOMETRIC_REPRESENTATION_ITEM ( )  RATIONAL_B_SPLINE_CURVE ( ( 1.000000000000000000, 0.9998674868020707152, 0.9998674868020707152, 1.000000000000000000 ) ) 
 REPRESENTATION_ITEM ( '' )  );
#56112=VERTEX_POINT ( 'NONE', #40060 ) ;
#56114=DIRECTION ( 'NONE',  ( 1.000000000000000000, 0.000000000000000000, -0.000000000000000000 ) ) ;
#56117=EDGE_LOOP ( 'NONE', ( #34865, #12720, #40325, #17745 ) ) ;
#56121=CIRCLE ( 'NONE', #43392, 12.18650000000000055 ) ;
#56122=DIRECTION ( 'NONE',  ( -0.4531421102008652557, 0.000000000000000000, -0.8914382917301156839 ) ) ;
#56123=EDGE_CURVE ( 'NONE', #2304, #35366, #13663, .T. ) ;
#56124=CARTESIAN_POINT ( 'NONE',  ( -17.13751750617693403, -7.344255242515008497, 9.496604519765444508 ) ) ;
#56125=FACE_OUTER_BOUND ( 'NONE', #11350, .T. ) ;
#56128=DIRECTION ( 'NONE',  ( 0.000000000000000000, -0.01356324068817998940, 0.9999080150203990547 ) ) ;
#56130=ADVANCED_FACE ( 'NONE', ( #174 ), #55710, .T. ) ;
#56131=DIRECTION ( 'NONE',  ( -1.000000000000000000, 0.000000000000000000, 0.000000000000000000 ) ) ;
#56133=CARTESIAN_POINT ( 'NONE',  ( 28.96537032880950591, -9.359309874800233686, 7.513625803917611812 ) ) ;
#56134=CARTESIAN_POINT ( 'NONE',  ( -10.76005699428653806, -6.156792290948529534, 10.30836155159126299 ) ) ;
#56135=VECTOR ( 'NONE', #33949, 1000.000000000000000 ) ;
#56136=EDGE_LOOP ( 'NONE', ( #56172, #42081, #40195, #13559 ) ) ;
#56137=EDGE_CURVE ( 'NONE', #52670, #1326, #26418, .T. ) ;
#56138=ORIENTED_EDGE ( 'NONE', *, *, #17173, .T. ) ;
#56139=CARTESIAN_POINT ( 'NONE',  ( 10.75853767213705225, 7.830989516993144051, -10.99661780661415733 ) ) ;
#56140=ORIENTED_EDGE ( 'NONE', *, *, #38746, .T. ) ;
#56143=DIRECTION ( 'NONE',  ( 0.000000000000000000, 0.01356324068817998940, -0.9999080150203990547 ) ) ;
#56144=CYLINDRICAL_SURFACE ( 'NONE', #1433, 12.18649999999999878 ) ;
#56146=EDGE_CURVE ( 'NONE', #42786, #42779, #30734, .T. ) ;
#56149=ORIENTED_EDGE ( 'NONE', *, *, #37821, .T. ) ;
#56150=CARTESIAN_POINT ( 'NONE',  ( -7.594202851097166196, -6.461772726810069756, -10.13291195006097745 ) ) ;
#56151=ORIENTED_EDGE ( 'NONE', *, *, #29958, .T. ) ;
#56156=ORIENTED_EDGE ( 'NONE', *, *, #16756, .F. ) ;
#56159=AXIS2_PLACEMENT_3D ( 'NONE', #24009, #18706, #19682 ) ;
#56161=DIRECTION ( 'NONE',  ( 0.000000000000000000, 0.6943713148249588407, -0.7196168960969844264 ) ) ;
#56162=DIRECTION ( 'NONE',  ( -0.000000000000000000, -0.000000000000000000, -1.000000000000000000 ) ) ;
#56165=ORIENTED_EDGE ( 'NONE', *, *, #64731, .T. ) ;
#56166=ORIENTED_EDGE ( 'NONE', *, *, #23182, .F. ) ;
#56167=EDGE_CURVE ( 'NONE', #41839, #7978, #51950, .T. ) ;
#56169=DIRECTION ( 'NONE',  ( 0.000000000000000000, -0.01356324068818000328, 0.9999080150203990547 ) ) ;
#56170=VERTEX_POINT ( 'NONE', #30422 ) ;
#56171=CARTESIAN_POINT ( 'NONE',  ( -28.41827485489077532, 3.509237424706437292, -11.47541949982828413 ) ) ;
#56172=ORIENTED_EDGE ( 'NONE', *, *, #59985, .F. ) ;
#56173=ORIENTED_EDGE ( 'NONE', *, *, #51761, .F. ) ;
#56174=AXIS2_PLACEMENT_3D ( 'NONE', #47701, #53011, #2144 ) ;
#56176=CYLINDRICAL_SURFACE ( 'NONE', #46887, 3.594603870727467676 ) ;
#56178=DIRECTION ( 'NONE',  ( 1.000000000000000000, 0.000000000000000000, 0.000000000000000000 ) ) ;
#56179=DIRECTION ( 'NONE',  ( -0.000000000000000000, -1.000000000000000000, -0.000000000000000000 ) ) ;
#56182=CARTESIAN_POINT ( 'NONE',  ( -25.86628395826706850, -5.139808748864358456, 10.84354029019568522 ) ) ;
#56184=DIRECTION ( 'NONE',  ( -1.000000000000000000, 0.000000000000000000, 0.000000000000000000 ) ) ;
#56185=DIRECTION ( 'NONE',  ( 0.000000000000000000, -1.000000000000000000, 0.000000000000000000 ) ) ;
#56186=DIRECTION ( 'NONE',  ( 1.000000000000000000, -0.000000000000000000, 0.000000000000000000 ) ) ;
#56190=ADVANCED_FACE ( 'NONE', ( #50403 ), #40731, .T. ) ;
#56191=ADVANCED_FACE ( 'NONE', ( #36399 ), #45382, .T. ) ;
#56193=ORIENTED_EDGE ( 'NONE', *, *, #16948, .F. ) ;
#56194=CARTESIAN_POINT ( 'NONE',  ( 35.00000000000000000, 9.493370459201798894, 6.917234959366719060 ) ) ;
#56195=ORIENTED_EDGE ( 'NONE', *, *, #21624, .F. ) ;
#56198=CARTESIAN_POINT ( 'NONE',  ( 10.33711885797364083, -13.43829105577338190, -1.303661106969844274 ) ) ;
#56200=CARTESIAN_POINT ( 'NONE',  ( 37.00000000000000711, 4.705694406421931860E-17, -3.469127814946512892E-15 ) ) ;
#56201=ORIENTED_EDGE ( 'NONE', *, *, #20418, .F. ) ;
#56202=ADVANCED_FACE ( 'NONE', ( #62625 ), #42669, .F. ) ;
#56203=LINE ( 'NONE', #1356, #6935 ) ;
#56205=CARTESIAN_POINT ( 'NONE',  ( 22.04496710003973803, 10.54007463054590232, -5.749627913936380175 ) ) ;
#56206=CARTESIAN_POINT ( 'NONE',  ( 22.36482863261543486, -13.46837713145126791, -0.9234811557364140944 ) ) ;
#56207=CIRCLE ( 'NONE', #49855, 12.75000000000000178 ) ;
#56208=EDGE_CURVE ( 'NONE', #31482, #4661, #40188, .T. ) ;
#56209=CIRCLE ( 'NONE', #10583, 5.000000000000000000 ) ;
#56211=DIRECTION ( 'NONE',  ( 1.000000000000000000, -0.000000000000000000, 0.000000000000000000 ) ) ;
#56212=EDGE_CURVE ( 'NONE', #59369, #34055, #23265, .T. ) ;
#56215=DIRECTION ( 'NONE',  ( -1.000000000000000000, -0.000000000000000000, 0.000000000000000000 ) ) ;
#56216=AXIS2_PLACEMENT_3D ( 'NONE', #9968, #50545, #30250 ) ;
#56223=EDGE_CURVE ( 'NONE', #52684, #31963, #4134, .T. ) ;
#56224=CARTESIAN_POINT ( 'NONE',  ( -36.00000000000000711, 12.73293890771483383, 0.6593684648220944355 ) ) ;
#56225=EDGE_LOOP ( 'NONE', ( #11352, #46632, #4643, #59785 ) ) ;
#56227=ORIENTED_EDGE ( 'NONE', *, *, #42655, .T. ) ;
#56228=VERTEX_POINT ( 'NONE', #12416 ) ;
#56230=ADVANCED_FACE ( 'NONE', ( #12746 ), #52688, .T. ) ;
#56231=CIRCLE ( 'NONE', #62577, 5.000000000000000000 ) ;
#56232=CARTESIAN_POINT ( 'NONE',  ( -35.00000000000000000, -0.3025107581132014389, 11.74226168163341200 ) ) ;
#56234=EDGE_CURVE ( 'NONE', #31673, #62587, #47688, .T. ) ;
#56236=DIRECTION ( 'NONE',  ( 0.000000000000000000, 0.8169148498130255343, -0.5767582926624997830 ) ) ;
#56239=CIRCLE ( 'NONE', #54114, 12.75000000000000178 ) ;
#56241=DIRECTION ( 'NONE',  ( 0.000000000000000000, -0.01356324068817992175, 0.9999080150203990547 ) ) ;
#56242=ORIENTED_EDGE ( 'NONE', *, *, #51060, .F. ) ;
#56243=EDGE_CURVE ( 'NONE', #48365, #16579, #45510, .T. ) ;
#56246=CARTESIAN_POINT ( 'NONE',  ( -37.00000000000000711, 9.196955404009424129, -8.830544224262844466 ) ) ;
#56247=VERTEX_POINT ( 'NONE', #22759 ) ;
#56248=CARTESIAN_POINT ( 'NONE',  ( 13.40667394824980896, -10.89379735224136603, -5.037499513965738807 ) ) ;
#56249=AXIS2_PLACEMENT_3D ( 'NONE', #4660, #65778, #60825 ) ;
#56254=CARTESIAN_POINT ( 'NONE',  ( 37.00000000000000711, 4.705694406421931860E-17, -3.469127814946512892E-15 ) ) ;
#56255=CARTESIAN_POINT ( 'NONE',  ( -35.00000000000000000, -7.251710744571512102, -9.240395740215712195 ) ) ;
#56256=CYLINDRICAL_SURFACE ( 'NONE', #26716, 12.74999999999999822 ) ;
#56258=ORIENTED_EDGE ( 'NONE', *, *, #49628, .T. ) ;
#56261=EDGE_LOOP ( 'NONE', ( #50025, #12257, #24078, #63075 ) ) ;
#56262=DIRECTION ( 'NONE',  ( 0.000000000000000000, -0.01356324068817999114, 0.9999080150203989437 ) ) ;
#56264=VERTEX_POINT ( 'NONE', #27080 ) ;
#56265=CARTESIAN_POINT ( 'NONE',  ( 24.97568612634365692, 8.683198485571637093, -8.285225425757136719 ) ) ;
#56266=DIRECTION ( 'NONE',  ( 0.000000000000000000, -0.01356324068817999114, 0.9999080150203989437 ) ) ;
#56267=CIRCLE ( 'NONE', #10593, 5.000000000000000000 ) ;
#56269=DIRECTION ( 'NONE',  ( -1.000000000000000000, 0.000000000000000000, 0.000000000000000000 ) ) ;
#56271=EDGE_CURVE ( 'NONE', #32582, #37450, #33833, .T. ) ;
#56272=ORIENTED_EDGE ( 'NONE', *, *, #39656, .T. ) ;
#56273=CARTESIAN_POINT ( 'NONE',  ( -17.50773065187699018, -5.755997118861490236, -10.53071770204327251 ) ) ;
#56274=ORIENTED_EDGE ( 'NONE', *, *, #42596, .F. ) ;
#56276=DIRECTION ( 'NONE',  ( 1.000000000000000000, 0.000000000000000000, 0.000000000000000000 ) ) ;
#56277=CARTESIAN_POINT ( 'NONE',  ( -27.01437459610461644, 25.00000000000000000, -2.220455681983952267 ) ) ;
#56280=EDGE_CURVE ( 'NONE', #51182, #19771, #21140, .T. ) ;
#56282=AXIS2_PLACEMENT_3D ( 'NONE', #6345, #42533, #2692 ) ;
#56283=AXIS2_PLACEMENT_3D ( 'NONE', #34097, #3566, #39094 ) ;
#56286=DIRECTION ( 'NONE',  ( -1.000000000000000000, 0.000000000000000000, 0.000000000000000000 ) ) ;
#56289=ORIENTED_EDGE ( 'NONE', *, *, #54987, .F. ) ;
#56293=EDGE_CURVE ( 'NONE', #48492, #35533, #41288, .T. ) ;
#56294=CARTESIAN_POINT ( 'NONE',  ( -15.21621911491949319, 7.970342840283608510, 10.89608346908821446 ) ) ;
#56295=CARTESIAN_POINT ( 'NONE',  ( 19.28625800530497258, -6.413918128308385036, 11.87904264843581537 ) ) ;
#56297=ORIENTED_EDGE ( 'NONE', *, *, #19231, .T. ) ;
#56298=LINE ( 'NONE', #11091, #31080 ) ;
#56299=FACE_OUTER_BOUND ( 'NONE', #23971, .T. ) ;
#56301=ORIENTED_EDGE ( 'NONE', *, *, #41595, .T. ) ;
#56303=DIRECTION ( 'NONE',  ( 0.000000000000000000, 0.01356324068817992175, -0.9999080150203990547 ) ) ;
#56306=ORIENTED_EDGE ( 'NONE', *, *, #30204, .F. ) ;
#56308=EDGE_CURVE ( 'NONE', #13765, #34180, #38107, .T. ) ;
#56311=EDGE_CURVE ( 'NONE', #30052, #82, #43420, .T. ) ;
#56315=CIRCLE ( 'NONE', #36176, 12.75000000000000178 ) ;
#56320=CARTESIAN_POINT ( 'NONE',  ( -35.00000000000000000, 12.16893194857549965, 3.805206332242515366 ) ) ;
#56323=EDGE_CURVE ( 'NONE', #24519, #52930, #41709, .T. ) ;
#56324=AXIS2_PLACEMENT_3D ( 'NONE', #63023, #32097, #31458 ) ;
#56325=ORIENTED_EDGE ( 'NONE', *, *, #8180, .T. ) ;
#56329=DIRECTION ( 'NONE',  ( 0.000000000000000000, -0.01356324068817991828, 0.9999080150203990547 ) ) ;
#56331=DIRECTION ( 'NONE',  ( 0.000000000000000000, -0.01356324068817998940, 0.9999080150203990547 ) ) ;
#56333=EDGE_LOOP ( 'NONE', ( #47563, #44970, #3090, #34804 ) ) ;
#56334=AXIS2_PLACEMENT_3D ( 'NONE', #23998, #34283, #64853 ) ;
#56335=AXIS2_PLACEMENT_3D ( 'NONE', #27007, #21700, #31642 ) ;
#56336=CYLINDRICAL_SURFACE ( 'NONE', #17446, 12.75000000000000178 ) ;
#56339=CARTESIAN_POINT ( 'NONE',  ( 19.67311005600952711, -0.7004819783312107306, 25.00000000000000000 ) ) ;
#56341=ORIENTED_EDGE ( 'NONE', *, *, #7833, .F. ) ;
#56342=ORIENTED_EDGE ( 'NONE', *, *, #15732, .F. ) ;
#56345=ORIENTED_EDGE ( 'NONE', *, *, #19391, .F. ) ;
#56346=DIRECTION ( 'NONE',  ( 1.000000000000000000, -0.000000000000000000, -0.000000000000000000 ) ) ;
#56349=CARTESIAN_POINT ( 'NONE',  ( 16.84448096326508804, -10.22195168550365985, 6.309017530714546851 ) ) ;
#56350=DIRECTION ( 'NONE',  ( 1.000000000000000000, 0.000000000000000000, 0.000000000000000000 ) ) ;
#56351=CARTESIAN_POINT ( 'NONE',  ( -37.00000000000000711, -3.827046518385164742, 11.56998259273176188 ) ) ;
#56352=DIRECTION ( 'NONE',  ( 1.000000000000000000, 0.000000000000000000, 0.000000000000000000 ) ) ;
#56354=VECTOR ( 'NONE', #53791, 1000.000000000000000 ) ;
#56355=EDGE_CURVE ( 'NONE', #13695, #6530, #1817, .T. ) ;
#56356=VERTEX_POINT ( 'NONE', #27391 ) ;
#56357=VECTOR ( 'NONE', #41633, 1000.000000000000000 ) ;
#56358=DIRECTION ( 'NONE',  ( 0.000000000000000000, -0.01356324068817998940, 0.9999080150203990547 ) ) ;
#56359=DIRECTION ( 'NONE',  ( 0.000000000000000000, 0.01356324068817991828, -0.9999080150203990547 ) ) ;
#56360=AXIS2_PLACEMENT_3D ( 'NONE', #29283, #45229, #24286 ) ;
#56362=LINE ( 'NONE', #60362, #23889 ) ;
#56363=DIRECTION ( 'NONE',  ( 0.000000000000000000, -0.01356324068817991828, 0.9999080150203990547 ) ) ;
#56364=AXIS2_PLACEMENT_3D ( 'NONE', #65176, #18674, #38934 ) ;
#56365=CARTESIAN_POINT ( 'NONE',  ( 35.00000000000000000, 10.32377448871667625, -6.475373545682339582 ) ) ;
#56366=CARTESIAN_POINT ( 'NONE',  ( 3.780834652287974773, 8.352030633203074927, -8.616471685210672860 ) ) ;
#56367=CARTESIAN_POINT ( 'NONE',  ( 8.437200413559441614, 4.476360154859203355, -11.13383131558893346 ) ) ;
#56371=LINE ( 'NONE', #10817, #53693 ) ;
#56375=AXIS2_PLACEMENT_3D ( 'NONE', #30379, #30688, #25073 ) ;
#56376=CIRCLE ( 'NONE', #47892, 12.18650000000000055 ) ;
#56377=CIRCLE ( 'NONE', #39377, 12.18649999999999878 ) ;
#56378=CARTESIAN_POINT ( 'NONE',  ( -27.09220147993978145, 10.57952257801956009, 5.663481862083665774 ) ) ;
#56379=DIRECTION ( 'NONE',  ( 1.000000000000000000, 0.000000000000000000, 0.000000000000000000 ) ) ;
#56383=CARTESIAN_POINT ( 'NONE',  ( -27.23354391799197316, -11.01738125875938046, -7.819786289819207425 ) ) ;
#56386=DIRECTION ( 'NONE',  ( -1.000000000000000000, -1.836970198721029688E-16, 0.000000000000000000 ) ) ;
#56387=CARTESIAN_POINT ( 'NONE',  ( -16.18648497833802224, 7.819859351283344751, -9.103005354533555860 ) ) ;
#56388=CARTESIAN_POINT ( 'NONE',  ( -35.00000000000000000, -2.544412758415929066, 11.91791701451265340 ) ) ;
#56390=ORIENTED_EDGE ( 'NONE', *, *, #48956, .T. ) ;
#56392=ADVANCED_FACE ( 'NONE', ( #19067 ), #34663, .T. ) ;
#56393=CIRCLE ( 'NONE', #3308, 12.75000000000000178 ) ;
#56395=ORIENTED_EDGE ( 'NONE', *, *, #15773, .T. ) ;
#56397=LINE ( 'NONE', #17147, #52125 ) ;
#56398=CARTESIAN_POINT ( 'NONE',  ( 22.86339282875463752, 2.804778511300523913, -11.66987002196172796 ) ) ;
#56399=DIRECTION ( 'NONE',  ( 0.000000000000000000, 0.01356324068817998940, -0.9999080150203990547 ) ) ;
#56400=CARTESIAN_POINT ( 'NONE',  ( 26.17141335727526652, 13.01134923558398704, 3.602278675730977930 ) ) ;
#56401=AXIS2_PLACEMENT_3D ( 'NONE', #3113, #23375, #43644 ) ;
#56402=CARTESIAN_POINT ( 'NONE',  ( -10.95212338237647920, -9.902220863987562183, 25.00000000000000000 ) ) ;
#56406=ORIENTED_EDGE ( 'NONE', *, *, #49029, .F. ) ;
#56407=DIRECTION ( 'NONE',  ( 0.000000000000000000, -0.4935949184179322380, 0.8696919319575150409 ) ) ;
#56411=CYLINDRICAL_SURFACE ( 'NONE', #34749, 12.75000000000000178 ) ;
#56415=EDGE_LOOP ( 'NONE', ( #16329, #65253, #15667, #39471 ) ) ;
#56416=CIRCLE ( 'NONE', #22484, 12.74999999999999822 ) ;
#56420=VERTEX_POINT ( 'NONE', #3477 ) ;
#56421=EDGE_LOOP ( 'NONE', ( #62474, #9446, #64259, #22553 ) ) ;
#56422=PLANE ( 'NONE',  #47020 ) ;
#56423=AXIS2_PLACEMENT_3D ( 'NONE', #61147, #45858, #56143 ) ;
#56426=FACE_OUTER_BOUND ( 'NONE', #62024, .T. ) ;
#56428=CARTESIAN_POINT ( 'NONE',  ( -35.00000000000000000, -9.557269938331609538, 7.561043153947932360 ) ) ;
#56429=CIRCLE ( 'NONE', #15028, 5.000000000000000000 ) ;
#56430=AXIS2_PLACEMENT_3D ( 'NONE', #22342, #37654, #52943 ) ;
#56431=CARTESIAN_POINT ( 'NONE',  ( -35.00000000000000000, 9.908974237959645492, 6.307491713049065751 ) ) ;
#56433=AXIS2_PLACEMENT_3D ( 'NONE', #26861, #31829, #16877 ) ;
#56434=CARTESIAN_POINT ( 'NONE',  ( -36.00000000000000711, 11.10408318471068689, -6.265926637539373623 ) ) ;
#56435=EDGE_CURVE ( 'NONE', #21573, #7430, #43668, .T. ) ;
#56436=ORIENTED_EDGE ( 'NONE', *, *, #41562, .T. ) ;
#56439=DIRECTION ( 'NONE',  ( -1.000000000000000000, 0.000000000000000000, 0.000000000000000000 ) ) ;
#56440=DIRECTION ( 'NONE',  ( -1.000000000000000000, 0.000000000000000000, 0.000000000000000000 ) ) ;
#56441=CARTESIAN_POINT ( 'NONE',  ( -9.329544065157421073, 10.53307963029291372, -5.752532211403271312 ) ) ;
#56442=CARTESIAN_POINT ( 'NONE',  ( -36.00000000000000711, 10.12742074351907817, -7.745827850122903868 ) ) ;
#56445=DIRECTION ( 'NONE',  ( -1.000000000000000000, 0.000000000000000000, 0.000000000000000000 ) ) ;
#56446=CIRCLE ( 'NONE', #46911, 12.18649999999999878 ) ;
#56448=VECTOR ( 'NONE', #18939, 1000.000000000000000 ) ;
#56451=CARTESIAN_POINT ( 'NONE',  ( 37.00000000000000711, 4.705694406421931860E-17, -3.469127814946512892E-15 ) ) ;
#56452=CIRCLE ( 'NONE', #27771, 12.18650000000000055 ) ;
#56457=CARTESIAN_POINT ( 'NONE',  ( 37.00000000000000711, -12.12087942037208776, 1.262958560998883595 ) ) ;
#56458=ADVANCED_FACE ( 'NONE', ( #13730 ), #14065, .T. ) ;
#56459=ORIENTED_EDGE ( 'NONE', *, *, #4045, .T. ) ;
#56460=CARTESIAN_POINT ( 'NONE',  ( 35.00000000000000000, -7.608228585767794705, -10.23119532541070420 ) ) ;
#56461=CARTESIAN_POINT ( 'NONE',  ( 35.00000000000000000, 4.705694406421931860E-17, -3.469127814946512892E-15 ) ) ;
#56462=VECTOR ( 'NONE', #30101, 1000.000000000000000 ) ;
#56465=DIRECTION ( 'NONE',  ( 0.000000000000000000, -0.01356324068817991828, 0.9999080150203990547 ) ) ;
#56468=EDGE_LOOP ( 'NONE', ( #36612, #27818, #19307, #35848 ) ) ;
#56469=CARTESIAN_POINT ( 'NONE',  ( 21.90174657591892071, 25.00000000000000000, -0.7349207973210698519 ) ) ;
#56472=DIRECTION ( 'NONE',  ( 0.000000000000000000, 0.01356324068817991828, -0.9999080150203990547 ) ) ;
#56474=DIRECTION ( 'NONE',  ( 0.000000000000000000, 0.01356324068817992175, -0.9999080150203990547 ) ) ;
#56475=CARTESIAN_POINT ( 'NONE',  ( -10.87564620705865082, -6.846636899367037010, 9.863669315241368807 ) ) ;
#56480=VERTEX_POINT ( 'NONE', #54331 ) ;
#56482=ORIENTED_EDGE ( 'NONE', *, *, #11490, .T. ) ;
#56484=DIRECTION ( 'NONE',  ( -1.000000000000000000, 0.000000000000000000, 0.000000000000000000 ) ) ;
#56487=CARTESIAN_POINT ( 'NONE',  ( 22.57855258442565116, 3.026812727784649493, 11.61199400236328749 ) ) ;
#56488=CARTESIAN_POINT ( 'NONE',  ( -11.20102014733715201, -9.173601788332002016, 9.918148130496701853 ) ) ;
#56489=CARTESIAN_POINT ( 'NONE',  ( -7.990345058477248408, -1.715916948163764166, 11.87819946997459120 ) ) ;
#56490=ORIENTED_EDGE ( 'NONE', *, *, #41634, .T. ) ;
#56493=VERTEX_POINT ( 'NONE', #44635 ) ;
#56494=DIRECTION ( 'NONE',  ( 0.000000000000000000, 0.9246979985058709772, 0.3807014730195252827 ) ) ;
#56496=DIRECTION ( 'NONE',  ( 0.000000000000000000, 0.01356324068817998940, -0.9999080150203989437 ) ) ;
#56497=EDGE_CURVE ( 'NONE', #4780, #52024, #16504, .T. ) ;
#56498=AXIS2_PLACEMENT_3D ( 'NONE', #7564, #63095, #38478 ) ;
#56499=CARTESIAN_POINT ( 'NONE',  ( 18.46659823902355768, 7.261787737648400132, 11.40465664842433924 ) ) ;
#56500=ORIENTED_EDGE ( 'NONE', *, *, #24116, .F. ) ;
#56501=CIRCLE ( 'NONE', #207, 4.999999999999998224 ) ;
#56504=CYLINDRICAL_SURFACE ( 'NONE', #32248, 12.74999999999999822 ) ;
#56508=EDGE_LOOP ( 'NONE', ( #32186, #37914, #5603, #13377 ) ) ;
#56509=AXIS2_PLACEMENT_3D ( 'NONE', #49571, #3371, #48278 ) ;
#56510=VERTEX_POINT ( 'NONE', #54961 ) ;
#56512=ORIENTED_EDGE ( 'NONE', *, *, #20567, .T. ) ;
#56514=ORIENTED_EDGE ( 'NONE', *, *, #21176, .T. ) ;
#56524=CARTESIAN_POINT ( 'NONE',  ( -37.00000000000000711, 9.752226076388895493, 6.547236723514054724 ) ) ;
#56526=CARTESIAN_POINT ( 'NONE',  ( 37.00000000000000711, -11.54110654723647400, 2.185196060784003524 ) ) ;
#56527=CIRCLE ( 'NONE', #4513, 4.999999999999999112 ) ;
#56528=EDGE_CURVE ( 'NONE', #13407, #49728, #9728, .T. ) ;
#56529=ORIENTED_EDGE ( 'NONE', *, *, #32611, .F. ) ;
#56532=EDGE_CURVE ( 'NONE', #11586, #41673, #7302, .T. ) ;
#56533=CARTESIAN_POINT ( 'NONE',  ( -3.288880356639787728, 9.825749110095811645, 9.264667814138983104 ) ) ;
#56534=EDGE_CURVE ( 'NONE', #38662, #35317, #29674, .T. ) ;
#56537=DIRECTION ( 'NONE',  ( 1.000000000000000000, -0.000000000000000000, 0.000000000000000000 ) ) ;
#56539=CIRCLE ( 'NONE', #17376, 12.18650000000000055 ) ;
#56540=AXIS2_PLACEMENT_3D ( 'NONE', #2686, #17947, #49213 ) ;
#56542=EDGE_LOOP ( 'NONE', ( #51968, #24108, #17761, #59675 ) ) ;
#56543=EDGE_CURVE ( 'NONE', #10925, #61800, #61453, .T. ) ;
#56544=DIRECTION ( 'NONE',  ( 0.000000000000000000, 0.6745969609292609137, 0.7381862504172000961 ) ) ;
#56545=ORIENTED_EDGE ( 'NONE', *, *, #56137, .T. ) ;
#56546=ADVANCED_FACE ( 'NONE', ( #10073 ), #10710, .T. ) ;
#56547=CARTESIAN_POINT ( 'NONE',  ( -10.79971841461723336, -9.842872838453388340, -6.865048668419079014 ) ) ;
#56548=DIRECTION ( 'NONE',  ( -1.000000000000000000, -0.000000000000000000, 0.000000000000000000 ) ) ;
#56551=CARTESIAN_POINT ( 'NONE',  ( -37.00000000000000711, 0.000000000000000000, 0.000000000000000000 ) ) ;
#56552=ORIENTED_EDGE ( 'NONE', *, *, #49874, .T. ) ;
#56553=DIRECTION ( 'NONE',  ( 1.000000000000000000, 0.000000000000000000, 0.000000000000000000 ) ) ;
#56555=CARTESIAN_POINT ( 'NONE',  ( 22.61260652651741054, 9.961396833084766200, -6.701065456133467713 ) ) ;
#56557=CIRCLE ( 'NONE', #61858, 12.18649999999999878 ) ;
#56559=DIRECTION ( 'NONE',  ( -1.000000000000000000, 0.000000000000000000, -0.000000000000000000 ) ) ;
#56560=AXIS2_PLACEMENT_3D ( 'NONE', #30169, #50138, #45451 ) ;
#56563=CARTESIAN_POINT ( 'NONE',  ( -20.79170840334646542, -11.34110549087206898, -3.921648409140116698 ) ) ;
#56565=ORIENTED_EDGE ( 'NONE', *, *, #28909, .T. ) ;
#56566=CIRCLE ( 'NONE', #45932, 5.000000000000000888 ) ;
#56567=VERTEX_POINT ( 'NONE', #21011 ) ;
#56570=CARTESIAN_POINT ( 'NONE',  ( -35.00000000000000000, 0.000000000000000000, 0.000000000000000000 ) ) ;
#56571=LINE ( 'NONE', #56224, #65766 ) ;
#56572=ORIENTED_EDGE ( 'NONE', *, *, #6470, .F. ) ;
#56573=VECTOR ( 'NONE', #7388, 1000.000000000000000 ) ;
#56574=AXIS2_PLACEMENT_3D ( 'NONE', #61541, #15986, #51605 ) ;
#56576=ORIENTED_EDGE ( 'NONE', *, *, #11090, .F. ) ;
#56578=AXIS2_PLACEMENT_3D ( 'NONE', #25798, #27106, #56040 ) ;
#56579=EDGE_CURVE ( 'NONE', #6611, #59647, #20047, .T. ) ;
#56581=AXIS2_PLACEMENT_3D ( 'NONE', #24089, #60310, #19438 ) ;
#56582=B_SPLINE_CURVE_WITH_KNOTS ( 'NONE', 3,
 ( #64537, #23682, #29956, #19008, #55230, #34610 ),
 .UNSPECIFIED., .F., .F.,
 ( 4, 2, 4 ),
 ( 0.005421911171979544933, 0.006610292730091626295, 0.007798674288203707658 ),
 .UNSPECIFIED. ) ;
#56583=ORIENTED_EDGE ( 'NONE', *, *, #45086, .F. ) ;
#56584=CARTESIAN_POINT ( 'NONE',  ( 47.00000000000000711, 4.705694406421931860E-17, -3.469127814946512892E-15 ) ) ;
#56585=DIRECTION ( 'NONE',  ( -1.000000000000000000, 0.000000000000000000, 0.000000000000000000 ) ) ;
#56588=EDGE_CURVE ( 'NONE', #27860, #10268, #64673, .T. ) ;
#56590=CARTESIAN_POINT ( 'NONE',  ( 24.54437410765793004, 1.233057148241763823, 11.94190642173460759 ) ) ;
#56591=ORIENTED_EDGE ( 'NONE', *, *, #11385, .F. ) ;
#56593=VERTEX_POINT ( 'NONE', #40982 ) ;
#56595=AXIS2_PLACEMENT_3D ( 'NONE', #42352, #62642, #58021 ) ;
#56596=ORIENTED_EDGE ( 'NONE', *, *, #52708, .T. ) ;
#56597=DIRECTION ( 'NONE',  ( 1.000000000000000000, 0.000000000000000000, 0.000000000000000000 ) ) ;
#56599=CARTESIAN_POINT ( 'NONE',  ( 145.1370849898475797, 3.309064568108273190E-14, 0.000000000000000000 ) ) ;
#56600=CIRCLE ( 'NONE', #6675, 12.18649999999999878 ) ;
#56601=CARTESIAN_POINT ( 'NONE',  ( 35.00000000000000000, 12.08151691381189785, -4.074242145636050694 ) ) ;
#56605=CARTESIAN_POINT ( 'NONE',  ( -37.00000000000000711, -7.238157050195700215, 10.49626516989268588 ) ) ;
#56607=DIRECTION ( 'NONE',  ( 1.000000000000000000, 0.000000000000000000, 0.000000000000000000 ) ) ;
#56608=VERTEX_POINT ( 'NONE', #51636 ) ;
#56610=DIRECTION ( 'NONE',  ( -1.000000000000000000, 0.000000000000000000, 0.000000000000000000 ) ) ;
#56611=AXIS2_PLACEMENT_3D ( 'NONE', #26401, #31398, #6793 ) ;
#56614=EDGE_CURVE ( 'NONE', #48464, #47999, #63629, .T. ) ;
#56615=AXIS2_PLACEMENT_3D ( 'NONE', #33112, #32764, #43407 ) ;
#56616=DIRECTION ( 'NONE',  ( 0.000000000000000000, -0.01356324068817992175, 0.9999080150203990547 ) ) ;
#56619=CARTESIAN_POINT ( 'NONE',  ( 37.00000000000000711, -1.039216533672818299, 11.70009620280412399 ) ) ;
#56620=DIRECTION ( 'NONE',  ( -1.000000000000000000, -0.000000000000000000, 0.000000000000000000 ) ) ;
#56623=CARTESIAN_POINT ( 'NONE',  ( 12.10998784662220729, 8.443435280036798218, -8.526922110106905706 ) ) ;
#56625=CARTESIAN_POINT ( 'NONE',  ( -17.38983135432702909, -6.044891695814540000, -10.36758421901369331 ) ) ;
#56626=VERTEX_POINT ( 'NONE', #46960 ) ;
#56627=ADVANCED_FACE ( 'NONE', ( #1078 ), #21698, .T. ) ;
#56629=DIRECTION ( 'NONE',  ( 0.000000000000000000, 0.01356324068817998940, -0.9999080150203990547 ) ) ;
#56630=CARTESIAN_POINT ( 'NONE',  ( -35.00000000000000000, 8.352657516904674395, 8.258652103341463047 ) ) ;
#56632=ORIENTED_EDGE ( 'NONE', *, *, #19716, .F. ) ;
#56633=CIRCLE ( 'NONE', #65098, 5.000000000000000000 ) ;
#56634=VECTOR ( 'NONE', #38085, 1000.000000000000000 ) ;
#56636=ADVANCED_FACE ( 'NONE', ( #7042 ), #31336, .T. ) ;
#56637=VECTOR ( 'NONE', #16050, 1000.000000000000000 ) ;
#56638=CIRCLE ( 'NONE', #5671, 5.000000000000000888 ) ;
#56639=EDGE_CURVE ( 'NONE', #8976, #55634, #49845, .T. ) ;
#56640=CARTESIAN_POINT ( 'NONE',  ( 29.03457606387295087, 7.862146963512124387, 10.97436308512422265 ) ) ;
#56642=CIRCLE ( 'NONE', #30091, 12.18649999999999878 ) ;
#56644=DIRECTION ( 'NONE',  ( 1.000000000000000000, 0.000000000000000000, 0.000000000000000000 ) ) ;
#56645=CARTESIAN_POINT ( 'NONE',  ( 8.485946503340201730, 5.237987331432492510, 12.44894516775456239 ) ) ;
#56646=PLANE ( 'NONE',  #29851 ) ;
#56647=CARTESIAN_POINT ( 'NONE',  ( -35.00000000000000000, 8.389074212634412220, -8.839356091079954680 ) ) ;
#56648=CARTESIAN_POINT ( 'NONE',  ( -35.00000000000000000, -3.287724142101498437, 11.73463472867575064 ) ) ;
#56649=AXIS2_PLACEMENT_3D ( 'NONE', #22186, #43115, #37146 ) ;
#56651=AXIS2_PLACEMENT_3D ( 'NONE', #44773, #65056, #35457 ) ;
#56652=ORIENTED_EDGE ( 'NONE', *, *, #15882, .T. ) ;
#56653=CARTESIAN_POINT ( 'NONE',  ( -17.88705001012359830, 6.214010860753471199, 11.98683707068579452 ) ) ;
#56654=LINE ( 'NONE', #59188, #1241 ) ;
#56655=AXIS2_PLACEMENT_3D ( 'NONE', #26723, #1473, #52000 ) ;
#56660=DIRECTION ( 'NONE',  ( 1.000000000000000000, 0.000000000000000000, 0.000000000000000000 ) ) ;
#56661=VERTEX_POINT ( 'NONE', #56950 ) ;
#56662=CARTESIAN_POINT ( 'NONE',  ( 26.08439714455133185, -12.97057518889163674, 3.743551691817328386 ) ) ;
#56663=FACE_OUTER_BOUND ( 'NONE', #28436, .T. ) ;
#56665=DIRECTION ( 'NONE',  ( 0.000000000000000000, -0.01356324068817992175, 0.9999080150203990547 ) ) ;
#56666=VERTEX_POINT ( 'NONE', #17010 ) ;
#56667=ORIENTED_EDGE ( 'NONE', *, *, #25177, .F. ) ;
#56669=EDGE_CURVE ( 'NONE', #49156, #51803, #14784, .T. ) ;
#56670=VECTOR ( 'NONE', #52183, 1000.000000000000000 ) ;
#56672=CARTESIAN_POINT ( 'NONE',  ( 35.00000000000000000, -3.093009498343839869, 11.78745411414842437 ) ) ;
#56674=CARTESIAN_POINT ( 'NONE',  ( 35.00000000000000000, -4.400442035670861785, 11.96656215839372805 ) ) ;
#56675=CARTESIAN_POINT ( 'NONE',  ( 37.00000000000000711, 4.705694406421931860E-17, -3.469127814946512892E-15 ) ) ;
#56682=ORIENTED_EDGE ( 'NONE', *, *, #65601, .T. ) ;
#56683=CARTESIAN_POINT ( 'NONE',  ( 35.00000000000000000, 12.68495603654573323, 1.286231064351170739 ) ) ;
#56684=EDGE_LOOP ( 'NONE', ( #62795, #62136, #46952, #46488 ) ) ;
#56685=AXIS2_PLACEMENT_3D ( 'NONE', #33392, #42350, #32392 ) ;
#56687=ORIENTED_EDGE ( 'NONE', *, *, #33257, .F. ) ;
#56688=EDGE_CURVE ( 'NONE', #14898, #62196, #46992, .T. ) ;
#56689=VECTOR ( 'NONE', #58661, 1000.000000000000000 ) ;
#56690=ORIENTED_EDGE ( 'NONE', *, *, #23268, .F. ) ;
#56692=LINE ( 'NONE', #11123, #2255 ) ;
#56693=AXIS2_PLACEMENT_3D ( 'NONE', #5364, #51907, #382 ) ;
#56694=CYLINDRICAL_SURFACE ( 'NONE', #50331, 5.000000000000002665 ) ;
#56695=VERTEX_POINT ( 'NONE', #28631 ) ;
#56696=CYLINDRICAL_SURFACE ( 'NONE', #674, 12.75000000000000178 ) ;
#56697=EDGE_CURVE ( 'NONE', #64338, #21860, #49588, .T. ) ;
#56698=DIRECTION ( 'NONE',  ( -1.000000000000000000, 0.000000000000000000, 0.000000000000000000 ) ) ;
#56699=CARTESIAN_POINT ( 'NONE',  ( -36.00000000000000711, -7.379373053628941470, 10.39746860227888270 ) ) ;
#56700=VERTEX_POINT ( 'NONE', #39257 ) ;
#56701=VECTOR ( 'NONE', #9190, 1000.000000000000000 ) ;
#56702=ORIENTED_EDGE ( 'NONE', *, *, #39716, .T. ) ;
#56703=DIRECTION ( 'NONE',  ( 0.000000000000000000, -0.4935949184179136418, 0.8696919319575254770 ) ) ;
#56704=ORIENTED_EDGE ( 'NONE', *, *, #52846, .F. ) ;
#56705=VECTOR ( 'NONE', #26196, 1000.000000000000000 ) ;
#56708=AXIS2_PLACEMENT_3D ( 'NONE', #29157, #44750, #65032 ) ;
#56710=CARTESIAN_POINT ( 'NONE',  ( -37.00000000000000711, 8.830544224262947495, 9.196955404009329982 ) ) ;
#56711=CARTESIAN_POINT ( 'NONE',  ( 36.00000000000000711, 5.710938531231875004, 11.39945968423464784 ) ) ;
#56713=CARTESIAN_POINT ( 'NONE',  ( 36.00000000000000711, -12.73293890771483561, -0.6593684648220077271 ) ) ;
#56715=DIRECTION ( 'NONE',  ( 1.000000000000000000, -0.000000000000000000, -0.000000000000000000 ) ) ;
#56716=CARTESIAN_POINT ( 'NONE',  ( -37.00000000000000711, 7.499679039484183463, -9.040300684349618976 ) ) ;
#56717=VERTEX_POINT ( 'NONE', #8045 ) ;
#56720=DIRECTION ( 'NONE',  ( 0.000000000000000000, -0.6478160128811839558, 0.7617968321374970486 ) ) ;
#56721=EDGE_CURVE ( 'NONE', #62845, #36702, #37053, .T. ) ;
#56722=DIRECTION ( 'NONE',  ( 1.000000000000000000, 0.000000000000000000, -0.000000000000000000 ) ) ;
#56723=VECTOR ( 'NONE', #42260, 1000.000000000000000 ) ;
#56724=CARTESIAN_POINT ( 'NONE',  ( -35.00000000000000000, -12.05416472667164207, -1.791059740004549372 ) ) ;
#56727=DIRECTION ( 'NONE',  ( -1.000000000000000000, -0.000000000000000000, -0.000000000000000000 ) ) ;
#56729=ADVANCED_FACE ( 'NONE', ( #58593 ), #2746, .T. ) ;
#56730=CARTESIAN_POINT ( 'NONE',  ( 12.47628546223243617, 0.000000000000000000, -11.99999999999998224 ) ) ;
#56732=DIRECTION ( 'NONE',  ( -1.000000000000000000, -1.836970198721029688E-16, -0.000000000000000000 ) ) ;
#56733=AXIS2_PLACEMENT_3D ( 'NONE', #24838, #38820, #65379 ) ;
#56734=CARTESIAN_POINT ( 'NONE',  ( 36.00000000000000711, 8.954052073409734192, 9.076753354953895681 ) ) ;
#56735=CARTESIAN_POINT ( 'NONE',  ( -25.64121911577780821, 4.545061814456081706, 11.11074877336984379 ) ) ;
#56736=AXIS2_PLACEMENT_3D ( 'NONE', #50516, #65762, #39864 ) ;
#56739=DIRECTION ( 'NONE',  ( 1.000000000000000000, 0.000000000000000000, 0.000000000000000000 ) ) ;
#56741=ORIENTED_EDGE ( 'NONE', *, *, #57455, .F. ) ;
#56742=DIRECTION ( 'NONE',  ( 1.000000000000000000, -0.000000000000000000, -0.000000000000000000 ) ) ;
#56743=CARTESIAN_POINT ( 'NONE',  ( -27.01437459610461644, -13.31613970204372421, -2.220455681983950935 ) ) ;
#56747=CARTESIAN_POINT ( 'NONE',  ( -17.96206987120463694, 6.006607899627029568, -10.39122312062567133 ) ) ;
#56749=AXIS2_PLACEMENT_3D ( 'NONE', #48376, #12753, #63299 ) ;
#56750=DIRECTION ( 'NONE',  ( 1.000000000000000000, -0.000000000000000000, -0.000000000000000000 ) ) ;
#56751=ORIENTED_EDGE ( 'NONE', *, *, #11536, .T. ) ;
#56753=AXIS2_PLACEMENT_3D ( 'NONE', #43983, #10596, #25919 ) ;
#56759=CARTESIAN_POINT ( 'NONE',  ( 36.00000000000000711, -9.621072037176935154, 8.366449238204463512 ) ) ;
#56760=CARTESIAN_POINT ( 'NONE',  ( 37.00000000000000711, -12.66641127287626745, -1.457575200925504300 ) ) ;
#56762=CARTESIAN_POINT ( 'NONE',  ( 37.00000000000000711, 5.130401251914885385, 11.05394794832823813 ) ) ;
#56763=AXIS2_PLACEMENT_3D ( 'NONE', #30724, #46371, #35712 ) ;
#56764=DIRECTION ( 'NONE',  ( 0.000000000000000000, 0.7381862504171974315, -0.6745969609292639113 ) ) ;
#56766=EDGE_LOOP ( 'NONE', ( #28402, #54923, #5419, #919 ) ) ;
#56767=ORIENTED_EDGE ( 'NONE', *, *, #22697, .T. ) ;
#56769=VERTEX_POINT ( 'NONE', #49277 ) ;
#56771=EDGE_CURVE ( 'NONE', #62930, #21730, #51282, .T. ) ;
#56772=CARTESIAN_POINT ( 'NONE',  ( -47.00000000000000711, 0.000000000000000000, 0.000000000000000000 ) ) ;
#56773=CIRCLE ( 'NONE', #60974, 5.000000000000000888 ) ;
#56774=CARTESIAN_POINT ( 'NONE',  ( -35.00000000000000000, 11.13736569743281457, -4.946702696913053643 ) ) ;
#56776=CARTESIAN_POINT ( 'NONE',  ( -35.00000000000000000, 0.000000000000000000, 0.000000000000000000 ) ) ;
#56778=FACE_BOUND ( 'NONE', #20452, .T. ) ;
#56779=EDGE_LOOP ( 'NONE', ( #61963, #52745, #6651, #35101 ) ) ;
#56780=ORIENTED_EDGE ( 'NONE', *, *, #56721, .T. ) ;
#56781=DIRECTION ( 'NONE',  ( -1.000000000000000000, 0.000000000000000000, -0.000000000000000000 ) ) ;
#56783=EDGE_CURVE ( 'NONE', #41081, #38995, #65713, .T. ) ;
#56784=AXIS2_PLACEMENT_3D ( 'NONE', #40354, #50373, #46351 ) ;
#56785=ORIENTED_EDGE ( 'NONE', *, *, #61209, .F. ) ;
#56788=CARTESIAN_POINT ( 'NONE',  ( 10.88606639118328445, 1.033256646594155947, 13.46088457202628241 ) ) ;
#56792=DIRECTION ( 'NONE',  ( 1.000000000000000000, 0.000000000000000000, 0.000000000000000000 ) ) ;
#56796=EDGE_CURVE ( 'NONE', #56264, #35347, #46257, .T. ) ;
#56797=CYLINDRICAL_SURFACE ( 'NONE', #31074, 4.999999999999999112 ) ;
#56798=DIRECTION ( 'NONE',  ( 1.000000000000000000, 0.000000000000000000, 0.000000000000000000 ) ) ;
#56799=DIRECTION ( 'NONE',  ( 0.000000000000000000, 0.01356324068817991828, -0.9999080150203990547 ) ) ;
#56800=DIRECTION ( 'NONE',  ( 1.000000000000000000, -0.000000000000000000, -0.000000000000000000 ) ) ;
#56801=CARTESIAN_POINT ( 'NONE',  ( -17.54726996257253191, 11.36053454945672847, 3.865003848717349033 ) ) ;
#56802=DIRECTION ( 'NONE',  ( 0.000000000000000000, -0.01356324068817999114, 0.9999080150203989437 ) ) ;
#56803=EDGE_CURVE ( 'NONE', #48103, #37848, #30583, .T. ) ;
#56804=AXIS2_PLACEMENT_3D ( 'NONE', #53050, #53393, #48412 ) ;
#56805=ORIENTED_EDGE ( 'NONE', *, *, #32105, .F. ) ;
#56806=VERTEX_POINT ( 'NONE', #5338 ) ;
#56807=LINE ( 'NONE', #31500, #17380 ) ;
#56811=DIRECTION ( 'NONE',  ( 0.000000000000000000, -0.01356324068817991828, 0.9999080150203990547 ) ) ;
#56813=DIRECTION ( 'NONE',  ( -1.000000000000000000, 0.000000000000000000, 0.000000000000000000 ) ) ;
#56814=ORIENTED_EDGE ( 'NONE', *, *, #52702, .T. ) ;
#56816=DIRECTION ( 'NONE',  ( 1.000000000000000000, 0.000000000000000000, 0.000000000000000000 ) ) ;
#56817=CYLINDRICAL_SURFACE ( 'NONE', #44949, 4.999999999999999112 ) ;
#56819=CIRCLE ( 'NONE', #28131, 12.18650000000000055 ) ;
#56820=DIRECTION ( 'NONE',  ( 0.000000000000000000, -0.01356324068817998940, 0.9999080150203990547 ) ) ;
#56822=ORIENTED_EDGE ( 'NONE', *, *, #19878, .T. ) ;
#56824=VERTEX_POINT ( 'NONE', #40911 ) ;
#56826=DIRECTION ( 'NONE',  ( 1.000000000000000000, -0.000000000000000000, 0.000000000000000000 ) ) ;
#56827=CARTESIAN_POINT ( 'NONE',  ( -37.00000000000000711, 0.000000000000000000, 0.000000000000000000 ) ) ;
#56828=CIRCLE ( 'NONE', #15406, 5.000000000000000888 ) ;
#56829=CARTESIAN_POINT ( 'NONE',  ( -30.18541646480307250, -0.9656489334300984995, -13.47303279728103931 ) ) ;
#56830=CARTESIAN_POINT ( 'NONE',  ( -10.90165637463012516, -7.508992741355087652, 9.360289953322833867 ) ) ;
#56832=ORIENTED_EDGE ( 'NONE', *, *, #50012, .T. ) ;
#56834=ORIENTED_EDGE ( 'NONE', *, *, #46263, .T. ) ;
#56835=ADVANCED_FACE ( 'NONE', ( #4705 ), #30275, .T. ) ;
#56838=AXIS2_PLACEMENT_3D ( 'NONE', #4538, #35734, #51410 ) ;
#56840=DIRECTION ( 'NONE',  ( 1.000000000000000000, 0.000000000000000000, -0.000000000000000000 ) ) ;
#56841=CARTESIAN_POINT ( 'NONE',  ( -17.29244623348158783, 2.525873743887551814, -13.26159725786978072 ) ) ;
#56842=CYLINDRICAL_SURFACE ( 'NONE', #25400, 3.477897737712717152 ) ;
#56843=CARTESIAN_POINT ( 'NONE',  ( -10.37062606838457768, -3.961740123981947193, 11.32887242500305724 ) ) ;
#56844=VERTEX_POINT ( 'NONE', #50575 ) ;
#56845=CARTESIAN_POINT ( 'NONE',  ( -9.316560581850643175, -10.03332002416863133, -6.593889625719990377 ) ) ;
#56847=CIRCLE ( 'NONE', #28160, 12.74999999999999822 ) ;
#56848=CARTESIAN_POINT ( 'NONE',  ( 21.81308386904231256, -12.46974327601525623, -5.176071965619618354 ) ) ;
#56851=ORIENTED_EDGE ( 'NONE', *, *, #14318, .F. ) ;
#56854=ORIENTED_EDGE ( 'NONE', *, *, #28806, .F. ) ;
#56856=CARTESIAN_POINT ( 'NONE',  ( -37.00000000000000711, 0.1414404973752139416, 12.74921544981111232 ) ) ;
#56857=CARTESIAN_POINT ( 'NONE',  ( 36.00000000000000711, -1.286231064351218478, 12.68495603654572612 ) ) ;
#56863=VERTEX_POINT ( 'NONE', #20939 ) ;
#56864=VERTEX_POINT ( 'NONE', #26926 ) ;
#56865=ORIENTED_EDGE ( 'NONE', *, *, #11396, .F. ) ;
#56867=EDGE_CURVE ( 'NONE', #57124, #2445, #47226, .T. ) ;
#56869=VECTOR ( 'NONE', #55961, 1000.000000000000000 ) ;
#56870=CARTESIAN_POINT ( 'NONE',  ( 47.00000000000000711, 4.705694406421931860E-17, -3.469127814946512892E-15 ) ) ;
#56872=CARTESIAN_POINT ( 'NONE',  ( -37.00000000000000711, -2.772148766916031182, -11.86701198550359315 ) ) ;
#56873=ORIENTED_EDGE ( 'NONE', *, *, #31577, .T. ) ;
#56874=ORIENTED_EDGE ( 'NONE', *, *, #13962, .T. ) ;
#56875=CARTESIAN_POINT ( 'NONE',  ( 37.00000000000000711, -6.946017217730009463, -10.01317267707884362 ) ) ;
#56876=CARTESIAN_POINT ( 'NONE',  ( -3.278282182819570956, 12.28207346570795266, 5.615173697092686211 ) ) ;
#56877=CARTESIAN_POINT ( 'NONE',  ( 35.00000000000000000, -11.38112321385048631, 2.905556151562744382 ) ) ;
#56881=DIRECTION ( 'NONE',  ( 0.000000000000000000, 0.01356324068817998940, -0.9999080150203989437 ) ) ;
#56883=VERTEX_POINT ( 'NONE', #31890 ) ;
#56885=AXIS2_PLACEMENT_3D ( 'NONE', #11317, #31904, #51896 ) ;
#56886=ORIENTED_EDGE ( 'NONE', *, *, #56614, .F. ) ;
#56892=VERTEX_POINT ( 'NONE', #31571 ) ;
#56893=DIRECTION ( 'NONE',  ( 0.000000000000000000, -0.01356324068817991828, 0.9999080150203990547 ) ) ;
#56897=AXIS2_PLACEMENT_3D ( 'NONE', #42565, #51613, #46599 ) ;
#56901=FACE_OUTER_BOUND ( 'NONE', #4240, .T. ) ;
#56903=CARTESIAN_POINT ( 'NONE',  ( 35.00000000000000000, -12.63095688309027587, 1.738225594540123042 ) ) ;
#56905=CIRCLE ( 'NONE', #607, 12.74999999999999822 ) ;
#56906=ORIENTED_EDGE ( 'NONE', *, *, #45559, .F. ) ;
#56911=CARTESIAN_POINT ( 'NONE',  ( 9.575800908719084958, 25.00000000000000000, -1.072919909436247154 ) ) ;
#56914=ADVANCED_FACE ( 'NONE', ( #36894 ), #52210, .T. ) ;
#56915=ORIENTED_EDGE ( 'NONE', *, *, #34994, .T. ) ;
#56916=VERTEX_POINT ( 'NONE', #682 ) ;
#56917=ORIENTED_EDGE ( 'NONE', *, *, #31480, .T. ) ;
#56921=ORIENTED_EDGE ( 'NONE', *, *, #17102, .T. ) ;
#56922=AXIS2_PLACEMENT_3D ( 'NONE', #30343, #40968, #30644 ) ;
#56924=CARTESIAN_POINT ( 'NONE',  ( 37.00000000000000711, 2.936739658819871313, -11.37311665002364869 ) ) ;
#56925=ORIENTED_EDGE ( 'NONE', *, *, #2915, .F. ) ;
#56926=CIRCLE ( 'NONE', #35628, 5.000000000000000000 ) ;
#56930=CARTESIAN_POINT ( 'NONE',  ( 24.80106626973253370, -1.726837946067656171, 11.87669879134540096 ) ) ;
#56932=CARTESIAN_POINT ( 'NONE',  ( -35.00000000000000000, 0.000000000000000000, 0.000000000000000000 ) ) ;
#56933=ORIENTED_EDGE ( 'NONE', *, *, #2098, .T. ) ;
#56934=EDGE_CURVE ( 'NONE', #45445, #429, #16900, .T. ) ;
#56936=LINE ( 'NONE', #62875, #10678 ) ;
#56939=CARTESIAN_POINT ( 'NONE',  ( -35.00000000000000000, 8.146229107149400406, 9.063649021438985542 ) ) ;
#56940=CARTESIAN_POINT ( 'NONE',  ( 24.82652845881425208, -10.42385221765392700, -8.578654028722157321 ) ) ;
#56941=CARTESIAN_POINT ( 'NONE',  ( -37.00000000000000711, 7.745827850123013114, 10.12742074351899468 ) ) ;
#56942=LINE ( 'NONE', #57255, #27811 ) ;
#56944=EDGE_CURVE ( 'NONE', #12123, #52081, #45397, .T. ) ;
#56945=DIRECTION ( 'NONE',  ( 1.000000000000000000, 0.000000000000000000, -0.000000000000000000 ) ) ;
#56946=ORIENTED_EDGE ( 'NONE', *, *, #26365, .F. ) ;
#56947=CYLINDRICAL_SURFACE ( 'NONE', #9401, 12.18650000000000055 ) ;
#56948=CARTESIAN_POINT ( 'NONE',  ( -25.64121911577780466, -4.545061814456073712, 11.11074877336984912 ) ) ;
#56949=ORIENTED_EDGE ( 'NONE', *, *, #14727, .F. ) ;
#56950=CARTESIAN_POINT ( 'NONE',  ( 35.00000000000000000, -4.074242145636090662, -12.08151691381188364 ) ) ;
#56951=CARTESIAN_POINT ( 'NONE',  ( -29.68541646480307250, -1.416020129149132334, 25.00000000000000000 ) ) ;
#56952=CARTESIAN_POINT ( 'NONE',  ( -37.00000000000000711, 11.44858830469740241, -2.627174906296955381 ) ) ;
#56953=CARTESIAN_POINT ( 'NONE',  ( -36.00000000000000711, -4.400442035671033203, 11.96656215839367654 ) ) ;
#56954=DIRECTION ( 'NONE',  ( 1.000000000000000000, 0.000000000000000000, 0.000000000000000000 ) ) ;
#56955=VERTEX_POINT ( 'NONE', #7625 ) ;
#56957=ORIENTED_EDGE ( 'NONE', *, *, #24358, .F. ) ;
#56958=DIRECTION ( 'NONE',  ( 0.000000000000000000, -0.7381862504172023165, 0.6745969609292584712 ) ) ;
#56959=CARTESIAN_POINT ( 'NONE',  ( -35.00000000000000000, 0.000000000000000000, 0.000000000000000000 ) ) ;
#56960=DIRECTION ( 'NONE',  ( 0.000000000000000000, 0.9346839223284554299, -0.3554799084908935036 ) ) ;
#56961=VERTEX_POINT ( 'NONE', #27908 ) ;
#56963=EDGE_CURVE ( 'NONE', #43998, #53899, #45561, .T. ) ;
#56964=CARTESIAN_POINT ( 'NONE',  ( 28.67799586904336806, 11.72473780571475466, 6.702742294911029575 ) ) ;
#56965=DIRECTION ( 'NONE',  ( -1.000000000000000000, 0.000000000000000000, 0.000000000000000000 ) ) ;
#56966=CARTESIAN_POINT ( 'NONE',  ( 12.10998784662220551, 10.46621227226785322, -8.526922110106907482 ) ) ;
#56967=FACE_OUTER_BOUND ( 'NONE', #3546, .T. ) ;
#56968=DIRECTION ( 'NONE',  ( -1.000000000000000000, 0.000000000000000000, 0.000000000000000000 ) ) ;
#56971=ADVANCED_FACE ( 'NONE', ( #49192 ), #38866, .T. ) ;
#56972=VERTEX_POINT ( 'NONE', #58504 ) ;
#56975=ORIENTED_EDGE ( 'NONE', *, *, #56, .T. ) ;
#56977=DIRECTION ( 'NONE',  ( -1.000000000000000000, 0.000000000000000000, 0.000000000000000000 ) ) ;
#56979=CARTESIAN_POINT ( 'NONE',  ( 9.150617453175268423, 5.808824337495268608, -10.50676510956234289 ) ) ;
#56981=DIRECTION ( 'NONE',  ( 1.000000000000000000, 0.000000000000000000, -0.000000000000000000 ) ) ;
#56982=EDGE_CURVE ( 'NONE', #54227, #64858, #48766, .T. ) ;
#56986=EDGE_LOOP ( 'NONE', ( #6151, #21508, #53969, #56565 ) ) ;
#56990=CARTESIAN_POINT ( 'NONE',  ( -25.04938166283714196, -9.464668315551032052, 7.379181612682862657 ) ) ;
#56992=CARTESIAN_POINT ( 'NONE',  ( 37.00000000000000711, 4.705694406421931860E-17, -3.469127814946512892E-15 ) ) ;
#56993=CYLINDRICAL_SURFACE ( 'NONE', #26933, 12.75000000000000178 ) ;
#56998=DIRECTION ( 'NONE',  ( -1.000000000000000000, 0.000000000000000000, 0.000000000000000000 ) ) ;
#57001=CARTESIAN_POINT ( 'NONE',  ( -28.25052396502597674, 10.95476879881297272, -4.908481086492510137 ) ) ;
#57005=VERTEX_POINT ( 'NONE', #12934 ) ;
#57006=AXIS2_PLACEMENT_3D ( 'NONE', #43246, #21684, #22305 ) ;
#57007=DIRECTION ( 'NONE',  ( 1.000000000000000000, 0.000000000000000000, 0.000000000000000000 ) ) ;
#57011=ORIENTED_EDGE ( 'NONE', *, *, #41357, .T. ) ;
#57012=LINE ( 'NONE', #49011, #53736 ) ;
#57013=AXIS2_PLACEMENT_3D ( 'NONE', #58215, #11993, #12317 ) ;
#57015=LINE ( 'NONE', #35714, #20316 ) ;
#57016=EDGE_CURVE ( 'NONE', #26553, #55701, #1023, .T. ) ;
#57017=ORIENTED_EDGE ( 'NONE', *, *, #43181, .F. ) ;
#57018=VERTEX_POINT ( 'NONE', #14862 ) ;
#57019=FACE_OUTER_BOUND ( 'NONE', #22971, .T. ) ;
#57020=VERTEX_POINT ( 'NONE', #9902 ) ;
#57021=EDGE_CURVE ( 'NONE', #60276, #32830, #50489, .T. ) ;
#57023=DIRECTION ( 'NONE',  ( 0.000000000000000000, -0.01356324068818697166, 0.9999080150203988326 ) ) ;
#57025=CARTESIAN_POINT ( 'NONE',  ( 35.00000000000000000, -0.2661492558802491248, 12.18359334611896116 ) ) ;
#57027=DIRECTION ( 'NONE',  ( 1.000000000000000000, 0.000000000000000000, 0.000000000000000000 ) ) ;
#57028=CARTESIAN_POINT ( 'NONE',  ( 35.00000000000000000, 4.705694406421931860E-17, -3.469127814946512892E-15 ) ) ;
#57029=DIRECTION ( 'NONE',  ( -1.000000000000000000, 0.000000000000000000, -0.000000000000000000 ) ) ;
#57030=ORIENTED_EDGE ( 'NONE', *, *, #28999, .F. ) ;
#57031=CYLINDRICAL_SURFACE ( 'NONE', #17973, 2.977897737712716708 ) ;
#57032=CARTESIAN_POINT ( 'NONE',  ( -4.020473488733464329, -8.896967761833661115, 8.055697172489294289 ) ) ;
#57036=CYLINDRICAL_SURFACE ( 'NONE', #30043, 12.18650000000000055 ) ;
#57038=CARTESIAN_POINT ( 'NONE',  ( 1.656291714771122692, 0.7705446217105330620, -11.97644560228689414 ) ) ;
#57039=CARTESIAN_POINT ( 'NONE',  ( 8.623231295854225209, 3.167640682658209528, -11.57732002835950880 ) ) ;
#57043=CYLINDRICAL_SURFACE ( 'NONE', #61935, 10.70557198542813815 ) ;
#57044=EDGE_CURVE ( 'NONE', #16664, #26657, #42207, .T. ) ;
#57047=EDGE_CURVE ( 'NONE', #32997, #27860, #272, .T. ) ;
#57048=AXIS2_PLACEMENT_3D ( 'NONE', #62209, #35624, #61231 ) ;
#57049=CARTESIAN_POINT ( 'NONE',  ( 11.32985899526506834, 0.8050469939657922680, -13.47645748469515681 ) ) ;
#57052=CARTESIAN_POINT ( 'NONE',  ( -18.90004703488476423, -4.071512182036163274, -12.87324253533143903 ) ) ;
#57053=CARTESIAN_POINT ( 'NONE',  ( -27.27771710733888710, -13.23190005995061647, -2.725643356596643585 ) ) ;
#57055=ORIENTED_EDGE ( 'NONE', *, *, #2602, .F. ) ;
#57060=ORIENTED_EDGE ( 'NONE', *, *, #28053, .T. ) ;
#57063=EDGE_LOOP ( 'NONE', ( #24113, #47466, #14746, #19936 ) ) ;
#57064=DIRECTION ( 'NONE',  ( 0.000000000000000000, -0.3807014730195283359, 0.9246979985058697560 ) ) ;
#57065=LINE ( 'NONE', #56759, #20258 ) ;
#57066=CARTESIAN_POINT ( 'NONE',  ( 24.36224182249226899, -0.009850770392023379049, -12.00517586461388575 ) ) ;
#57067=LINE ( 'NONE', #46426, #58483 ) ;
#57071=DIRECTION ( 'NONE',  ( -1.000000000000000000, 0.000000000000000000, 0.000000000000000000 ) ) ;
#57072=ORIENTED_EDGE ( 'NONE', *, *, #48586, .T. ) ;
#57073=EDGE_CURVE ( 'NONE', #43919, #38911, #29693, .T. ) ;
#57074=VERTEX_POINT ( 'NONE', #51794 ) ;
#57075=CARTESIAN_POINT ( 'NONE',  ( 24.68219558003250924, 0.8422048916808957397, -11.97679777458489347 ) ) ;
#57082=EDGE_CURVE ( 'NONE', #1623, #14535, #8450, .T. ) ;
#57084=ORIENTED_EDGE ( 'NONE', *, *, #6794, .T. ) ;
#57085=DIRECTION ( 'NONE',  ( -1.000000000000000000, 0.000000000000000000, 0.000000000000000000 ) ) ;
#57086=DIRECTION ( 'NONE',  ( -1.000000000000000000, 0.000000000000000000, 0.000000000000000000 ) ) ;
#57088=VERTEX_POINT ( 'NONE', #1252 ) ;
#57089=VERTEX_POINT ( 'NONE', #23086 ) ;
#57091=CARTESIAN_POINT ( 'NONE',  ( 29.09509651717319301, -8.201516007081412596, 10.73123560021122636 ) ) ;
#57092=ORIENTED_EDGE ( 'NONE', *, *, #6342, .F. ) ;
#57093=B_SPLINE_CURVE_WITH_KNOTS ( 'NONE', 3,
 ( #31025, #31354, #51333, #41313, #36668, #16046, #36336, #56645, #11081, #51658 ),
 .UNSPECIFIED., .F., .F.,
 ( 4, 2, 2, 2, 4 ),
 ( 0.000000000000000000, 0.001226751953743790424, 0.002453503907487580848, 0.003680255861231371273, 0.004907007814975161697 ),
 .UNSPECIFIED. ) ;
#57098=CARTESIAN_POINT ( 'NONE',  ( 47.00000000000000711, 4.705694406421931860E-17, -3.469127814946512892E-15 ) ) ;
#57103=ORIENTED_EDGE ( 'NONE', *, *, #40071, .F. ) ;
#57105=CARTESIAN_POINT ( 'NONE',  ( 37.00000000000000711, 8.854740511458958352, 7.717887834988148121 ) ) ;
#57106=ORIENTED_EDGE ( 'NONE', *, *, #33029, .T. ) ;
#57109=CARTESIAN_POINT ( 'NONE',  ( -8.891032880924177206, 11.36194426013951997, -3.860857758255646921 ) ) ;
#57111=DIRECTION ( 'NONE',  ( 1.000000000000000000, -0.000000000000000000, -0.000000000000000000 ) ) ;
#57113=DIRECTION ( 'NONE',  ( -1.000000000000000000, 0.000000000000000000, 0.000000000000000000 ) ) ;
#57114=ORIENTED_EDGE ( 'NONE', *, *, #376, .F. ) ;
#57115=ADVANCED_FACE ( 'NONE', ( #21533 ), #38365, .T. ) ;
#57116=ORIENTED_EDGE ( 'NONE', *, *, #39861, .T. ) ;
#57117=DIRECTION ( 'NONE',  ( 0.000000000000000000, -0.4380125133593848474, 0.8989688749565218906 ) ) ;
#57118=EDGE_CURVE ( 'NONE', #59596, #54960, #32139, .T. ) ;
#57121=CARTESIAN_POINT ( 'NONE',  ( 37.00000000000000711, -11.02904044024205987, 4.041347439435972966 ) ) ;
#57124=VERTEX_POINT ( 'NONE', #41799 ) ;
#57125=CARTESIAN_POINT ( 'NONE',  ( 3.459614771489464946, -11.09853614738469396, 25.00000000000000000 ) ) ;
#57132=CARTESIAN_POINT ( 'NONE',  ( -36.00000000000000711, -12.08151691381193160, 4.074242145635959211 ) ) ;
#57133=AXIS2_PLACEMENT_3D ( 'NONE', #2418, #62565, #37309 ) ;
#57134=VERTEX_POINT ( 'NONE', #63622 ) ;
#57136=ORIENTED_EDGE ( 'NONE', *, *, #53370, .F. ) ;
#57137=VECTOR ( 'NONE', #65335, 1000.000000000000000 ) ;
#57138=CARTESIAN_POINT ( 'NONE',  ( 35.00000000000000000, -11.42599468261425955, 4.237620530777920003 ) ) ;
#57140=DIRECTION ( 'NONE',  ( 0.000000000000000000, -0.01356324068817992175, 0.9999080150203990547 ) ) ;
#57141=ADVANCED_FACE ( 'NONE', ( #11860 ), #37127, .T. ) ;
#57142=AXIS2_PLACEMENT_3D ( 'NONE', #40316, #59974, #65274 ) ;
#57143=CARTESIAN_POINT ( 'NONE',  ( -35.00000000000000000, -9.506317355798309165, -8.496612874013260708 ) ) ;
#57144=EDGE_CURVE ( 'NONE', #34377, #35021, #62093, .T. ) ;
#57145=CARTESIAN_POINT ( 'NONE',  ( 35.00000000000000000, -9.040300684349746874, -7.499679039484027143 ) ) ;
#57147=ORIENTED_EDGE ( 'NONE', *, *, #34289, .F. ) ;
#57148=ORIENTED_EDGE ( 'NONE', *, *, #49184, .T. ) ;
#57149=CARTESIAN_POINT ( 'NONE',  ( -37.00000000000000711, 11.73808581813437968, -0.4353888892048790038 ) ) ;
#57151=DIRECTION ( 'NONE',  ( 1.000000000000000000, 0.000000000000000000, -0.000000000000000000 ) ) ;
#57152=CARTESIAN_POINT ( 'NONE',  ( 35.00000000000000000, 4.705694406421931860E-17, -3.469127814946512892E-15 ) ) ;
#57153=CARTESIAN_POINT ( 'NONE',  ( 37.00000000000000711, -10.07641281632173325, 6.036400161834665212 ) ) ;
#57154=CARTESIAN_POINT ( 'NONE',  ( -10.95212338237647920, -9.902220863987562183, 9.175839033069923545 ) ) ;
#57156=ORIENTED_EDGE ( 'NONE', *, *, #6828, .F. ) ;
#57158=EDGE_LOOP ( 'NONE', ( #47518, #56957, #30309, #3217 ) ) ;
#57159=CYLINDRICAL_SURFACE ( 'NONE', #65291, 5.000000000000001776 ) ;
#57161=CARTESIAN_POINT ( 'NONE',  ( -37.00000000000000711, -2.905556151562544986, -11.38112321385053960 ) ) ;
#57162=DIRECTION ( 'NONE',  ( 0.000000000000000000, -0.01356324068817992175, 0.9999080150203990547 ) ) ;
#57163=EDGE_CURVE ( 'NONE', #38173, #34288, #39039, .T. ) ;
#57164=DIRECTION ( 'NONE',  ( 0.000000000000000000, -0.01356324068817998940, 0.9999080150203990547 ) ) ;
#57165=ORIENTED_EDGE ( 'NONE', *, *, #53900, .F. ) ;
#57166=LINE ( 'NONE', #31548, #21641 ) ;
#57167=DIRECTION ( 'NONE',  ( 0.000000000000000000, 0.01356324068817998940, -0.9999080150203990547 ) ) ;
#57170=VERTEX_POINT ( 'NONE', #21864 ) ;
#57171=VERTEX_POINT ( 'NONE', #42108 ) ;
#57172=EDGE_CURVE ( 'NONE', #10928, #44959, #21055, .T. ) ;
#57173=CARTESIAN_POINT ( 'NONE',  ( 0.3463514696222815270, 0.2404099497127392404, 13.50000000000000533 ) ) ;
#57175=ORIENTED_EDGE ( 'NONE', *, *, #39496, .T. ) ;
#57176=ORIENTED_EDGE ( 'NONE', *, *, #52964, .T. ) ;
#57177=ORIENTED_EDGE ( 'NONE', *, *, #45645, .T. ) ;
#57180=CIRCLE ( 'NONE', #15755, 12.74999999999999822 ) ;
#57181=DIRECTION ( 'NONE',  ( 0.000000000000000000, 0.7790879021242529401, -0.6269146997507959451 ) ) ;
#57182=CARTESIAN_POINT ( 'NONE',  ( 35.00000000000000000, -9.196955404009232282, 8.830544224263039865 ) ) ;
#57183=DIRECTION ( 'NONE',  ( 0.000000000000000000, 0.8515178078024887576, -0.5243256840888532722 ) ) ;
#57184=ORIENTED_EDGE ( 'NONE', *, *, #29438, .T. ) ;
#57185=EDGE_CURVE ( 'NONE', #32930, #44305, #63682, .T. ) ;
#57187=CIRCLE ( 'NONE', #49761, 12.18650000000000055 ) ;
#57188=CIRCLE ( 'NONE', #39115, 5.000000000000001776 ) ;
#57190=DIRECTION ( 'NONE',  ( 0.000000000000000000, 0.01356324068817998940, -0.9999080150203990547 ) ) ;
#57191=FACE_OUTER_BOUND ( 'NONE', #4142, .T. ) ;
#57192=CIRCLE ( 'NONE', #7279, 5.000000000000000000 ) ;
#57196=CARTESIAN_POINT ( 'NONE',  ( -35.00000000000000000, 11.59605747147786836, 5.300372733891681953 ) ) ;
#57197=CIRCLE ( 'NONE', #65651, 12.74999999999999822 ) ;
#57199=DIRECTION ( 'NONE',  ( 0.000000000000000000, 0.01356324068817992175, -0.9999080150203990547 ) ) ;
#57200=ADVANCED_FACE ( 'NONE', ( #4453 ), #3486, .T. ) ;
#57201=ORIENTED_EDGE ( 'NONE', *, *, #11639, .F. ) ;
#57202=CARTESIAN_POINT ( 'NONE',  ( -35.00000000000000000, -11.65554240571058031, 1.456211999474302798 ) ) ;
#57204=DIRECTION ( 'NONE',  ( 0.000000000000000000, -0.01356324068817998940, 0.9999080150203990547 ) ) ;
#57206=DIRECTION ( 'NONE',  ( -1.000000000000000000, 0.000000000000000000, 0.000000000000000000 ) ) ;
#57208=FACE_OUTER_BOUND ( 'NONE', #42812, .T. ) ;
#57209=CARTESIAN_POINT ( 'NONE',  ( -10.48620311856347875, -9.720786832536937538, -9.367833439828894271 ) ) ;
#57212=CIRCLE ( 'NONE', #17900, 4.999999999999999112 ) ;
#57220=ORIENTED_EDGE ( 'NONE', *, *, #62272, .F. ) ;
#57221=CIRCLE ( 'NONE', #31710, 4.999999999999999112 ) ;
#57223=VERTEX_POINT ( 'NONE', #9094 ) ;
#57226=DIRECTION ( 'NONE',  ( -1.000000000000000000, 0.000000000000000000, 0.000000000000000000 ) ) ;
#57228=CARTESIAN_POINT ( 'NONE',  ( -47.00000000000000711, 0.000000000000000000, 0.000000000000000000 ) ) ;
#57229=VERTEX_POINT ( 'NONE', #59981 ) ;
#57230=ORIENTED_EDGE ( 'NONE', *, *, #15126, .T. ) ;
#57232=VERTEX_POINT ( 'NONE', #39022 ) ;
#57234=EDGE_CURVE ( 'NONE', #10479, #39914, #13740, .T. ) ;
#57235=FACE_OUTER_BOUND ( 'NONE', #24755, .T. ) ;
#57236=ORIENTED_EDGE ( 'NONE', *, *, #12914, .T. ) ;
#57237=CARTESIAN_POINT ( 'NONE',  ( 6.812204945636112896, -4.138731716409435712, 12.84993773446340803 ) ) ;
#57239=ORIENTED_EDGE ( 'NONE', *, *, #21483, .T. ) ;
#57240=CYLINDRICAL_SURFACE ( 'NONE', #38564, 12.74999999999999822 ) ;
#57241=FACE_OUTER_BOUND ( 'NONE', #44235, .T. ) ;
#57242=CYLINDRICAL_SURFACE ( 'NONE', #36688, 12.75000000000000178 ) ;
#57245=EDGE_LOOP ( 'NONE', ( #6445, #36029, #9650, #38566 ) ) ;
#57248=CYLINDRICAL_SURFACE ( 'NONE', #35126, 5.000000000000000888 ) ;
#57250=DIRECTION ( 'NONE',  ( 1.000000000000000000, 0.000000000000000000, 0.000000000000000000 ) ) ;
#57252=CARTESIAN_POINT ( 'NONE',  ( 37.00000000000000711, 8.496612874013157679, -9.506317355798403312 ) ) ;
#57253=CARTESIAN_POINT ( 'NONE',  ( -36.00000000000000711, 7.379373053629018742, -10.39746860227882763 ) ) ;
#57254=DIRECTION ( 'NONE',  ( -1.000000000000000000, -0.000000000000000000, 0.000000000000000000 ) ) ;
#57255=CARTESIAN_POINT ( 'NONE',  ( 12.47628546223243617, 0.000000000000000000, 25.00000000000000000 ) ) ;
#57257=DIRECTION ( 'NONE',  ( 0.000000000000000000, -0.01356324068817999114, 0.9999080150203989437 ) ) ;
#57258=VERTEX_POINT ( 'NONE', #34028 ) ;
#57259=AXIS2_PLACEMENT_3D ( 'NONE', #58167, #32867, #38532 ) ;
#57260=DIRECTION ( 'NONE',  ( -1.000000000000000000, 0.000000000000000000, 0.000000000000000000 ) ) ;
#57261=FACE_OUTER_BOUND ( 'NONE', #20698, .T. ) ;
#57263=CARTESIAN_POINT ( 'NONE',  ( -18.58686583997225839, 5.151216734910813777, 10.83812558286603789 ) ) ;
#57265=DIRECTION ( 'NONE',  ( -1.000000000000000000, 0.000000000000000000, 0.000000000000000000 ) ) ;
#57267=CIRCLE ( 'NONE', #9431, 5.000000000000000000 ) ;
#57268=AXIS2_PLACEMENT_3D ( 'NONE', #58122, #17227, #63097 ) ;
#57269=ORIENTED_EDGE ( 'NONE', *, *, #5872, .F. ) ;
#57271=LINE ( 'NONE', #46633, #25827 ) ;
#57272=CIRCLE ( 'NONE', #21178, 5.000000000000000000 ) ;
#57276=DIRECTION ( 'NONE',  ( 1.000000000000000000, 0.000000000000000000, 0.000000000000000000 ) ) ;
#57277=EDGE_CURVE ( 'NONE', #48941, #44984, #28626, .T. ) ;
#57278=CYLINDRICAL_SURFACE ( 'NONE', #16927, 4.999999999999999112 ) ;
#57282=EDGE_CURVE ( 'NONE', #3877, #21253, #65759, .T. ) ;
#57283=( BOUNDED_CURVE ( )  B_SPLINE_CURVE ( 3, ( #62568, #4546, #26357, #36978 ),
 .UNSPECIFIED., .F., .F. ) 
 B_SPLINE_CURVE_WITH_KNOTS ( ( 4, 4 ),
 ( 2.328873244820985011, 2.340611521109171811 ),
 .UNSPECIFIED. ) 
 CURVE ( )  GEOMETRIC_REPRESENTATION_ITEM ( )  RATIONAL_B_SPLINE_CURVE ( ( 1.000000000000000000, 0.9999885177721090646, 0.9999885177721090646, 1.000000000000000000 ) ) 
 REPRESENTATION_ITEM ( '' )  );
#57284=CARTESIAN_POINT ( 'NONE',  ( 29.03190650753573010, 11.07607182691292280, 7.728831390951418356 ) ) ;
#57285=DIRECTION ( 'NONE',  ( 0.000000000000000000, -0.01356324068817999114, 0.9999080150203989437 ) ) ;
#57286=CARTESIAN_POINT ( 'NONE',  ( 35.00000000000000000, 3.704519465651471499, 11.60979404548630178 ) ) ;
#57287=CARTESIAN_POINT ( 'NONE',  ( -37.00000000000000711, 4.824807283154123994, 11.80185301892982608 ) ) ;
#57289=EDGE_CURVE ( 'NONE', #48293, #52670, #56239, .T. ) ;
#57291=FACE_OUTER_BOUND ( 'NONE', #53202, .T. ) ;
#57292=CIRCLE ( 'NONE', #64712, 12.18650000000000233 ) ;
#57296=ORIENTED_EDGE ( 'NONE', *, *, #15074, .F. ) ;
#57299=DIRECTION ( 'NONE',  ( 0.000000000000000000, 0.9651210252299803338, 0.2618041379715599914 ) ) ;
#57300=FACE_OUTER_BOUND ( 'NONE', #25690, .T. ) ;
#57301=ORIENTED_EDGE ( 'NONE', *, *, #4260, .T. ) ;
#57303=ORIENTED_EDGE ( 'NONE', *, *, #30080, .F. ) ;
#57308=VERTEX_POINT ( 'NONE', #54001 ) ;
#57309=CARTESIAN_POINT ( 'NONE',  ( -26.09207032238876423, -10.32898249965824355, 6.109300428488008805 ) ) ;
#57312=DIRECTION ( 'NONE',  ( -1.000000000000000000, 0.000000000000000000, 0.000000000000000000 ) ) ;
#57314=VERTEX_POINT ( 'NONE', #9399 ) ;
#57318=DIRECTION ( 'NONE',  ( 1.000000000000000000, -0.000000000000000000, 0.000000000000000000 ) ) ;
#57319=ORIENTED_EDGE ( 'NONE', *, *, #47801, .T. ) ;
#57320=DIRECTION ( 'NONE',  ( 0.000000000000000000, -0.01356324068817991828, 0.9999080150203990547 ) ) ;
#57322=CARTESIAN_POINT ( 'NONE',  ( 37.00000000000000711, 12.31350058095522826, -3.307597835713291801 ) ) ;
#57323=VECTOR ( 'NONE', #6300, 1000.000000000000000 ) ;
#57324=VERTEX_POINT ( 'NONE', #24380 ) ;
#57325=CARTESIAN_POINT ( 'NONE',  ( 23.59784752820392839, -9.149736952257297773, -7.769756470210803734 ) ) ;
#57326=CYLINDRICAL_SURFACE ( 'NONE', #31053, 12.74999999999999822 ) ;
#57329=ORIENTED_EDGE ( 'NONE', *, *, #35696, .T. ) ;
#57334=VERTEX_POINT ( 'NONE', #18448 ) ;
#57335=DIRECTION ( 'NONE',  ( -0.000000000000000000, -0.000000000000000000, -1.000000000000000000 ) ) ;
#57337=VERTEX_POINT ( 'NONE', #8779 ) ;
#57338=CARTESIAN_POINT ( 'NONE',  ( -37.00000000000000711, -8.052525312709946093, 8.551552972817052733 ) ) ;
#57339=DIRECTION ( 'NONE',  ( 0.000000000000000000, -0.01356324068817991828, 0.9999080150203990547 ) ) ;
#57341=CARTESIAN_POINT ( 'NONE',  ( -37.00000000000000711, 0.000000000000000000, 0.000000000000000000 ) ) ;
#57343=DIRECTION ( 'NONE',  ( -1.000000000000000000, 0.000000000000000000, 0.000000000000000000 ) ) ;
#57344=CARTESIAN_POINT ( 'NONE',  ( -37.00000000000000711, 0.000000000000000000, 0.000000000000000000 ) ) ;
#57346=EDGE_CURVE ( 'NONE', #13346, #12647, #38708, .T. ) ;
#57347=AXIS2_PLACEMENT_3D ( 'NONE', #57861, #62813, #52545 ) ;
#57348=DIRECTION ( 'NONE',  ( 1.000000000000000000, -0.000000000000000000, 0.000000000000000000 ) ) ;
#57349=EDGE_CURVE ( 'NONE', #31372, #34842, #21207, .T. ) ;
#57351=ADVANCED_FACE ( 'NONE', ( #64604, #448 ), #5432, .F. ) ;
#57353=CARTESIAN_POINT ( 'NONE',  ( -3.908087423533649130, -8.112892239103171477, 8.853223187161773922 ) ) ;
#57354=VECTOR ( 'NONE', #1216, 1000.000000000000000 ) ;
#57356=CARTESIAN_POINT ( 'NONE',  ( 35.00000000000000000, 4.705694406421931860E-17, -3.469127814946512892E-15 ) ) ;
#57357=EDGE_CURVE ( 'NONE', #64161, #46955, #41539, .T. ) ;
#57358=CIRCLE ( 'NONE', #39301, 5.000000000000000000 ) ;
#57360=EDGE_CURVE ( 'NONE', #4651, #14286, #62583, .T. ) ;
#57364=FACE_OUTER_BOUND ( 'NONE', #50122, .T. ) ;
#57366=FACE_OUTER_BOUND ( 'NONE', #6267, .T. ) ;
#57368=CARTESIAN_POINT ( 'NONE',  ( 8.937200413559439838, 4.243156749116337778, -12.81821838531965518 ) ) ;
#57369=CARTESIAN_POINT ( 'NONE',  ( -26.05227667049377160, -12.02424670906742321, 6.138434551438939124 ) ) ;
#57376=VERTEX_POINT ( 'NONE', #41304 ) ;
#57378=DIRECTION ( 'NONE',  ( -1.000000000000000000, 0.000000000000000000, 0.000000000000000000 ) ) ;
#57379=CARTESIAN_POINT ( 'NONE',  ( 37.00000000000000711, 7.474872387601131152, 9.060822531525964507 ) ) ;
#57380=ORIENTED_EDGE ( 'NONE', *, *, #14467, .T. ) ;
#57381=CARTESIAN_POINT ( 'NONE',  ( 36.00000000000000711, -10.23119532541067045, 7.608228585767832897 ) ) ;
#57384=AXIS2_PLACEMENT_3D ( 'NONE', #14737, #29090, #34697 ) ;
#57386=ORIENTED_EDGE ( 'NONE', *, *, #13658, .F. ) ;
#57387=CARTESIAN_POINT ( 'NONE',  ( -7.489022030332961322, 25.00000000000000000, -10.84914964302385521 ) ) ;
#57388=FACE_OUTER_BOUND ( 'NONE', #19462, .T. ) ;
#57389=DIRECTION ( 'NONE',  ( -1.000000000000000000, 0.000000000000000000, 0.000000000000000000 ) ) ;
#57390=CARTESIAN_POINT ( 'NONE',  ( -3.854685187122629308, -9.944885401855350082, 9.163283342679498844 ) ) ;
#57392=CYLINDRICAL_SURFACE ( 'NONE', #29159, 4.999999999999999112 ) ;
#57393=CARTESIAN_POINT ( 'NONE',  ( -35.00000000000000000, 4.983891302653582933, 11.73555825188278234 ) ) ;
#57395=ORIENTED_EDGE ( 'NONE', *, *, #3136, .T. ) ;
#57396=DIRECTION ( 'NONE',  ( 1.000000000000000000, -0.000000000000000000, 0.000000000000000000 ) ) ;
#57397=ORIENTED_EDGE ( 'NONE', *, *, #56867, .T. ) ;
#57399=FACE_OUTER_BOUND ( 'NONE', #39566, .T. ) ;
#57400=CIRCLE ( 'NONE', #51052, 5.000000000000000000 ) ;
#57401=CARTESIAN_POINT ( 'NONE',  ( 9.575800908719084958, 11.95193887484099093, -1.072919909436247154 ) ) ;
#57405=ORIENTED_EDGE ( 'NONE', *, *, #54895, .T. ) ;
#57407=CARTESIAN_POINT ( 'NONE',  ( -35.00000000000000000, 4.946702696913171771, 11.13736569743276306 ) ) ;
#57408=ORIENTED_EDGE ( 'NONE', *, *, #63777, .F. ) ;
#57411=EDGE_CURVE ( 'NONE', #36759, #35917, #39252, .T. ) ;
#57413=CIRCLE ( 'NONE', #17111, 5.000000000000000888 ) ;
#57416=CARTESIAN_POINT ( 'NONE',  ( 9.380725061917582153, 2.629308567162621735, 13.24320193369290877 ) ) ;
#57419=DIRECTION ( 'NONE',  ( 1.000000000000000000, 0.000000000000000000, 0.000000000000000000 ) ) ;
#57421=FACE_OUTER_BOUND ( 'NONE', #34713, .T. ) ;
#57425=AXIS2_PLACEMENT_3D ( 'NONE', #30469, #45432, #60739 ) ;
#57426=CARTESIAN_POINT ( 'NONE',  ( 37.00000000000000711, 4.946702696913328090, 11.13736569743268845 ) ) ;
#57429=CARTESIAN_POINT ( 'NONE',  ( -8.602359018442378158, 8.118472317678492089, -8.864987646168081881 ) ) ;
#57432=DIRECTION ( 'NONE',  ( -1.000000000000000000, 0.000000000000000000, 0.000000000000000000 ) ) ;
#57433=ORIENTED_EDGE ( 'NONE', *, *, #10741, .F. ) ;
#57434=CIRCLE ( 'NONE', #26672, 12.74999999999999822 ) ;
#57435=CIRCLE ( 'NONE', #93, 12.74999999999999822 ) ;
#57436=ORIENTED_EDGE ( 'NONE', *, *, #38182, .T. ) ;
#57437=CIRCLE ( 'NONE', #28754, 12.18650000000000055 ) ;
#57443=CARTESIAN_POINT ( 'NONE',  ( 35.00000000000000000, 4.705694406421931860E-17, -3.469127814946512892E-15 ) ) ;
#57444=CARTESIAN_POINT ( 'NONE',  ( 35.00000000000000000, -7.817610399097575602, -8.766823244861962294 ) ) ;
#57446=ADVANCED_FACE ( 'NONE', ( #21362 ), #7051, .T. ) ;
#57451=DIRECTION ( 'NONE',  ( -1.000000000000000000, 0.000000000000000000, 0.000000000000000000 ) ) ;
#57452=EDGE_CURVE ( 'NONE', #38595, #33373, #23353, .T. ) ;
#57453=AXIS2_PLACEMENT_3D ( 'NONE', #38162, #53496, #48827 ) ;
#57454=AXIS2_PLACEMENT_3D ( 'NONE', #30682, #39696, #19428 ) ;
#57455=EDGE_CURVE ( 'NONE', #8028, #34466, #13746, .T. ) ;
#57457=ADVANCED_FACE ( 'NONE', ( #62901 ), #37644, .T. ) ;
#57458=CARTESIAN_POINT ( 'NONE',  ( 24.82652845881425208, 25.00000000000000000, -8.578654028722157321 ) ) ;
#57459=AXIS2_PLACEMENT_3D ( 'NONE', #61780, #41832, #47487 ) ;
#57460=CARTESIAN_POINT ( 'NONE',  ( 9.650000913499871658, -11.97776111335497795, -0.7481793053950416272 ) ) ;
#57461=VERTEX_POINT ( 'NONE', #61927 ) ;
#57463=EDGE_CURVE ( 'NONE', #9113, #29799, #47758, .T. ) ;
#57467=LINE ( 'NONE', #1928, #23468 ) ;
#57468=AXIS2_PLACEMENT_3D ( 'NONE', #18256, #43840, #47854 ) ;
#57469=DIRECTION ( 'NONE',  ( 1.000000000000000000, -0.000000000000000000, 0.000000000000000000 ) ) ;
#57470=FACE_OUTER_BOUND ( 'NONE', #12345, .T. ) ;
#57471=VERTEX_POINT ( 'NONE', #31979 ) ;
#57474=EDGE_LOOP ( 'NONE', ( #23706, #34787, #33533, #46838 ) ) ;
#57477=CARTESIAN_POINT ( 'NONE',  ( 35.00000000000000000, 4.705694406421931860E-17, -3.469127814946512892E-15 ) ) ;
#57478=CARTESIAN_POINT ( 'NONE',  ( -35.00000000000000000, 0.000000000000000000, 0.000000000000000000 ) ) ;
#57480=FACE_OUTER_BOUND ( 'NONE', #19170, .T. ) ;
#57484=CIRCLE ( 'NONE', #131, 12.75000000000000178 ) ;
#57485=CYLINDRICAL_SURFACE ( 'NONE', #16193, 5.000000000000000888 ) ;
#57486=VERTEX_POINT ( 'NONE', #41963 ) ;
#57487=FACE_OUTER_BOUND ( 'NONE', #51946, .T. ) ;
#57489=DIRECTION ( 'NONE',  ( -1.000000000000000000, 0.000000000000000000, 0.000000000000000000 ) ) ;
#57490=EDGE_CURVE ( 'NONE', #51040, #3036, #55051, .T. ) ;
#57491=AXIS2_PLACEMENT_3D ( 'NONE', #36979, #56965, #57285 ) ;
#57492=AXIS2_PLACEMENT_3D ( 'NONE', #1277, #27502, #47800 ) ;
#57493=CARTESIAN_POINT ( 'NONE',  ( 35.00000000000000000, 4.705694406421931860E-17, -3.469127814946512892E-15 ) ) ;
#57494=ORIENTED_EDGE ( 'NONE', *, *, #40611, .T. ) ;
#57496=( BOUNDED_CURVE ( )  B_SPLINE_CURVE ( 3, ( #39211, #34550, #38903, #44207 ),
 .UNSPECIFIED., .F., .F. ) 
 B_SPLINE_CURVE_WITH_KNOTS ( ( 4, 4 ),
 ( 1.082322874641048704, 1.128276431546378022 ),
 .UNSPECIFIED. ) 
 CURVE ( )  GEOMETRIC_REPRESENTATION_ITEM ( )  RATIONAL_B_SPLINE_CURVE ( ( 1.000000000000000000, 0.9998240302925252010, 0.9998240302925252010, 1.000000000000000000 ) ) 
 REPRESENTATION_ITEM ( '' )  );
#57498=DIRECTION ( 'NONE',  ( 0.000000000000000000, -0.9796553971857721033, -0.2006870767258996657 ) ) ;
#57501=EDGE_LOOP ( 'NONE', ( #18693, #36172, #52443, #823 ) ) ;
#57502=LINE ( 'NONE', #5995, #18365 ) ;
#57503=ORIENTED_EDGE ( 'NONE', *, *, #37502, .F. ) ;
#57507=ORIENTED_EDGE ( 'NONE', *, *, #51653, .T. ) ;
#57508=VERTEX_POINT ( 'NONE', #27647 ) ;
#57512=CIRCLE ( 'NONE', #37358, 1.750000000000000000 ) ;
#57513=DIRECTION ( 'NONE',  ( 0.000000000000000000, 0.01356324068817999114, -0.9999080150203990547 ) ) ;
#57515=DIRECTION ( 'NONE',  ( 1.000000000000000000, -0.000000000000000000, 0.000000000000000000 ) ) ;
#57517=AXIS2_PLACEMENT_3D ( 'NONE', #64148, #38882, #59172 ) ;
#57518=CYLINDRICAL_SURFACE ( 'NONE', #31157, 12.75000000000000178 ) ;
#57519=ORIENTED_EDGE ( 'NONE', *, *, #49382, .F. ) ;
#57520=CARTESIAN_POINT ( 'NONE',  ( -29.76531599071173062, -3.714239038275569449, -12.97905452356682865 ) ) ;
#57521=CARTESIAN_POINT ( 'NONE',  ( 35.00000000000000000, 8.699265615723106748, 8.534258022645994757 ) ) ;
#57522=DIRECTION ( 'NONE',  ( 1.000000000000000000, 0.000000000000000000, 0.000000000000000000 ) ) ;
#57525=CARTESIAN_POINT ( 'NONE',  ( -37.00000000000000711, -12.01765980939843281, 2.021542716731355771 ) ) ;
#57527=CYLINDRICAL_SURFACE ( 'NONE', #50409, 12.18649999999999878 ) ;
#57529=DIRECTION ( 'NONE',  ( -1.000000000000000000, 0.000000000000000000, 0.000000000000000000 ) ) ;
#57530=AXIS2_PLACEMENT_3D ( 'NONE', #30176, #51126, #30806 ) ;
#57531=EDGE_LOOP ( 'NONE', ( #48993, #36375, #2459, #33913 ) ) ;
#57534=CARTESIAN_POINT ( 'NONE',  ( -35.00000000000000000, -5.428340790341781741, 10.91072401419408777 ) ) ;
#57535=DIRECTION ( 'NONE',  ( 0.000000000000000000, -0.8696919319575131535, -0.4935949184179356797 ) ) ;
#57538=ORIENTED_EDGE ( 'NONE', *, *, #28898, .T. ) ;
#57539=DIRECTION ( 'NONE',  ( 0.000000000000000000, 0.01356324068817992175, -0.9999080150203990547 ) ) ;
#57544=ADVANCED_FACE ( 'NONE', ( #48305 ), #12032, .T. ) ;
#57545=CIRCLE ( 'NONE', #28853, 12.74999999999999822 ) ;
#57546=CIRCLE ( 'NONE', #59664, 12.18650000000000411 ) ;
#57547=ADVANCED_FACE ( 'NONE', ( #21710 ), #41639, .T. ) ;
#57549=ORIENTED_EDGE ( 'NONE', *, *, #47111, .F. ) ;
#57552=CARTESIAN_POINT ( 'NONE',  ( -35.00000000000000000, -11.86701198550358427, 2.772148766916072926 ) ) ;
#57554=AXIS2_PLACEMENT_3D ( 'NONE', #19603, #39865, #14569 ) ;
#57555=VERTEX_POINT ( 'NONE', #43594 ) ;
#57557=VERTEX_POINT ( 'NONE', #64852 ) ;
#57560=DIRECTION ( 'NONE',  ( 0.000000000000000000, -1.000000000000000000, 0.000000000000000000 ) ) ;
#57562=CARTESIAN_POINT ( 'NONE',  ( 36.00000000000000711, 7.238157050195626496, -10.49626516989273561 ) ) ;
#57563=ORIENTED_EDGE ( 'NONE', *, *, #42145, .T. ) ;
#57566=ORIENTED_EDGE ( 'NONE', *, *, #22959, .T. ) ;
#57568=PRODUCT_DEFINITION ( 'UNKNOWN', '', #41979, #17306 ) ;
#57569=CARTESIAN_POINT ( 'NONE',  ( -37.00000000000000711, -11.91791701451264629, -2.544412758415973030 ) ) ;
#57570=EDGE_CURVE ( 'NONE', #45531, #28625, #18995, .T. ) ;
#57571=ORIENTED_EDGE ( 'NONE', *, *, #35554, .F. ) ;
#57572=FACE_OUTER_BOUND ( 'NONE', #56421, .T. ) ;
#57573=CIRCLE ( 'NONE', #48032, 4.999999999999999112 ) ;
#57574=FACE_OUTER_BOUND ( 'NONE', #12472, .T. ) ;
#57575=EDGE_CURVE ( 'NONE', #62291, #47988, #28319, .T. ) ;
#57576=ORIENTED_EDGE ( 'NONE', *, *, #18300, .F. ) ;
#57578=CARTESIAN_POINT ( 'NONE',  ( 35.00000000000000000, -6.657191900728386180, -9.677500615117878624 ) ) ;
#57579=FACE_OUTER_BOUND ( 'NONE', #27329, .T. ) ;
#57580=VERTEX_POINT ( 'NONE', #23997 ) ;
#57582=ORIENTED_EDGE ( 'NONE', *, *, #58754, .T. ) ;
#57584=EDGE_CURVE ( 'NONE', #19021, #37431, #28339, .T. ) ;
#57591=CIRCLE ( 'NONE', #246, 5.000000000000000000 ) ;
#57592=CARTESIAN_POINT ( 'NONE',  ( 36.00000000000000711, 12.66641127287627810, 1.457575200925408820 ) ) ;
#57593=FACE_OUTER_BOUND ( 'NONE', #61677, .T. ) ;
#57596=CARTESIAN_POINT ( 'NONE',  ( 35.00000000000000000, 2.865935305911623487, -12.42372387097883468 ) ) ;
#57597=EDGE_LOOP ( 'NONE', ( #62789, #25426, #52060, #35810 ) ) ;
#57599=CARTESIAN_POINT ( 'NONE',  ( 37.00000000000000711, 11.29812557209481483, 3.213188559034117819 ) ) ;
#57602=VERTEX_POINT ( 'NONE', #3403 ) ;
#57603=CARTESIAN_POINT ( 'NONE',  ( -17.99474996755618861, 7.056835936932178477, 9.708762815230446819 ) ) ;
#57604=CARTESIAN_POINT ( 'NONE',  ( -37.00000000000000711, 0.000000000000000000, 0.000000000000000000 ) ) ;
#57605=DIRECTION ( 'NONE',  ( 0.000000000000000000, 0.5472293298355214164, -0.8369827122275381726 ) ) ;
#57606=CIRCLE ( 'NONE', #53368, 5.000000000000000000 ) ;
#57607=EDGE_CURVE ( 'NONE', #53292, #45368, #58294, .T. ) ;
#57610=VERTEX_POINT ( 'NONE', #29607 ) ;
#57611=CARTESIAN_POINT ( 'NONE',  ( 36.00000000000000711, 9.390600770288115129, 8.624332853795948495 ) ) ;
#57612=CIRCLE ( 'NONE', #24706, 12.75000000000000178 ) ;
#57613=ORIENTED_EDGE ( 'NONE', *, *, #23596, .F. ) ;
#57614=CARTESIAN_POINT ( 'NONE',  ( -35.00000000000000000, -11.72397916322012890, 0.7214809346828189307 ) ) ;
#57617=CYLINDRICAL_SURFACE ( 'NONE', #14947, 5.000000000000000888 ) ;
#57619=DIRECTION ( 'NONE',  ( 0.000000000000000000, -0.01356324068817999114, 0.9999080150203989437 ) ) ;
#57620=ORIENTED_EDGE ( 'NONE', *, *, #31349, .T. ) ;
#57621=CARTESIAN_POINT ( 'NONE',  ( -35.00000000000000000, 7.215058775251398160, -9.821084925794490772 ) ) ;
#57622=EDGE_CURVE ( 'NONE', #49993, #64161, #43268, .T. ) ;
#57627=CARTESIAN_POINT ( 'NONE',  ( 23.18891912316549053, 11.76268964777006509, -6.631469957982857544 ) ) ;
#57628=DIRECTION ( 'NONE',  ( 0.000000000000000000, -0.8989688749565202253, -0.4380125133593882336 ) ) ;
#57629=FACE_OUTER_BOUND ( 'NONE', #43695, .T. ) ;
#57632=CIRCLE ( 'NONE', #28950, 5.000000000000000000 ) ;
#57633=CIRCLE ( 'NONE', #45946, 12.75000000000000178 ) ;
#57634=AXIS2_PLACEMENT_3D ( 'NONE', #3093, #48638, #64882 ) ;
#57635=ORIENTED_EDGE ( 'NONE', *, *, #36603, .F. ) ;
#57636=CARTESIAN_POINT ( 'NONE',  ( 37.00000000000000711, 5.865551165831078606, -11.32068061209297483 ) ) ;
#57637=CARTESIAN_POINT ( 'NONE',  ( 35.00000000000000000, 4.705694406421931860E-17, -3.469127814946512892E-15 ) ) ;
#57639=CARTESIAN_POINT ( 'NONE',  ( -21.23983773598477498, -7.447593303288433830, 25.00000000000000000 ) ) ;
#57641=ORIENTED_EDGE ( 'NONE', *, *, #10807, .T. ) ;
#57642=DIRECTION ( 'NONE',  ( -1.000000000000000000, -1.836970198721029688E-16, -0.000000000000000000 ) ) ;
#57643=ORIENTED_EDGE ( 'NONE', *, *, #9168, .F. ) ;
#57644=AXIS2_PLACEMENT_3D ( 'NONE', #46082, #1175, #55727 ) ;
#57645=DIRECTION ( 'NONE',  ( -1.000000000000000000, 0.000000000000000000, 0.000000000000000000 ) ) ;
#57646=EDGE_LOOP ( 'NONE', ( #63685, #11126, #18536, #25199 ) ) ;
#57647=ORIENTED_EDGE ( 'NONE', *, *, #34019, .T. ) ;
#57648=AXIS2_PLACEMENT_3D ( 'NONE', #31847, #21578, #20897 ) ;
#57653=DIRECTION ( 'NONE',  ( 1.000000000000000000, 0.000000000000000000, -0.000000000000000000 ) ) ;
#57654=CARTESIAN_POINT ( 'NONE',  ( 9.777179481675013051, 6.950299379875443329, 9.786861771856294467 ) ) ;
#57656=ORIENTED_EDGE ( 'NONE', *, *, #54950, .F. ) ;
#57658=CIRCLE ( 'NONE', #35360, 5.000000000000000000 ) ;
#57661=CARTESIAN_POINT ( 'NONE',  ( 12.49336221634852429, 0.1658369216508866484, -13.50000000000000355 ) ) ;
#57663=DIRECTION ( 'NONE',  ( 0.000000000000000000, -0.01356324068817991828, 0.9999080150203990547 ) ) ;
#57664=EDGE_LOOP ( 'NONE', ( #18999, #4791, #45931, #32734 ) ) ;
#57666=CARTESIAN_POINT ( 'NONE',  ( 21.44782229496123094, -11.52858179529749094, -3.336984548882474311 ) ) ;
#57667=DIRECTION ( 'NONE',  ( 0.000000000000000000, 0.07632122047556491595, -0.9970832820307039546 ) ) ;
#57670=EDGE_CURVE ( 'NONE', #20925, #56892, #53926, .T. ) ;
#57675=ORIENTED_EDGE ( 'NONE', *, *, #43153, .F. ) ;
#57677=ORIENTED_EDGE ( 'NONE', *, *, #54203, .T. ) ;
#57682=DIRECTION ( 'NONE',  ( 0.000000000000000000, 0.01356324068817992175, -0.9999080150203990547 ) ) ;
#57685=DIRECTION ( 'NONE',  ( -1.000000000000000000, -0.000000000000000000, -0.000000000000000000 ) ) ;
#57686=DIRECTION ( 'NONE',  ( 0.000000000000000000, 0.01356324068817992175, -0.9999080150203990547 ) ) ;
#57687=CIRCLE ( 'NONE', #31127, 5.000000000000000888 ) ;
#57688=CARTESIAN_POINT ( 'NONE',  ( -35.00000000000000000, 10.75351884295727700, -4.725891942574793170 ) ) ;
#57689=( BOUNDED_CURVE ( )  B_SPLINE_CURVE ( 3, ( #21597, #42169, #11925, #7259 ),
 .UNSPECIFIED., .F., .F. ) 
 B_SPLINE_CURVE_WITH_KNOTS ( ( 4, 4 ),
 ( 1.782871955780958029, 1.816812352449447499 ),
 .UNSPECIFIED. ) 
 CURVE ( )  GEOMETRIC_REPRESENTATION_ITEM ( )  RATIONAL_B_SPLINE_CURVE ( ( 1.000000000000000000, 0.9999040064266120353, 0.9999040064266120353, 1.000000000000000000 ) ) 
 REPRESENTATION_ITEM ( '' )  );
#57690=EDGE_LOOP ( 'NONE', ( #42924, #779, #48403, #48660 ) ) ;
#57694=AXIS2_PLACEMENT_3D ( 'NONE', #27263, #6991, #23258 ) ;
#57695=ADVANCED_FACE ( 'NONE', ( #49287 ), #14323, .F. ) ;
#57697=CARTESIAN_POINT ( 'NONE',  ( -35.00000000000000000, 0.000000000000000000, 0.000000000000000000 ) ) ;
#57698=DIRECTION ( 'NONE',  ( 1.000000000000000000, -0.000000000000000000, -0.000000000000000000 ) ) ;
#57699=DIRECTION ( 'NONE',  ( 0.000000000000000000, -0.01356324068817999114, 0.9999080150203989437 ) ) ;
#57701=AXIS2_PLACEMENT_3D ( 'NONE', #9635, #29931, #55870 ) ;
#57702=DIRECTION ( 'NONE',  ( 0.000000000000000000, -0.5987040770935562195, 0.8009703041134254020 ) ) ;
#57703=ORIENTED_EDGE ( 'NONE', *, *, #58103, .T. ) ;
#57705=CARTESIAN_POINT ( 'NONE',  ( -35.00000000000000000, 0.000000000000000000, 0.000000000000000000 ) ) ;
#57708=EDGE_CURVE ( 'NONE', #33918, #5651, #10409, .T. ) ;
#57709=AXIS2_PLACEMENT_3D ( 'NONE', #9721, #24053, #29356 ) ;
#57711=CARTESIAN_POINT ( 'NONE',  ( -25.66889450307327891, -8.265805117747651920, 10.67728274434794500 ) ) ;
#57712=ORIENTED_EDGE ( 'NONE', *, *, #41357, .F. ) ;
#57713=LINE ( 'NONE', #37404, #446 ) ;
#57715=CARTESIAN_POINT ( 'NONE',  ( 35.00000000000000000, 10.91072401419418014, 5.428340790341585453 ) ) ;
#57717=VERTEX_POINT ( 'NONE', #364 ) ;
#57718=DIRECTION ( 'NONE',  ( 0.000000000000000000, -0.01356324068817999114, 0.9999080150203989437 ) ) ;
#57720=CIRCLE ( 'NONE', #31176, 5.000000000000000000 ) ;
#57721=AXIS2_PLACEMENT_3D ( 'NONE', #25421, #10445, #20441 ) ;
#57722=DIRECTION ( 'NONE',  ( 0.000000000000000000, -0.4380125133593849029, 0.8989688749565220016 ) ) ;
#57724=DIRECTION ( 'NONE',  ( -0.000000000000000000, -0.000000000000000000, -1.000000000000000000 ) ) ;
#57725=AXIS2_PLACEMENT_3D ( 'NONE', #58620, #43611, #13040 ) ;
#57726=AXIS2_PLACEMENT_3D ( 'NONE', #64402, #33172, #17890 ) ;
#57727=EDGE_CURVE ( 'NONE', #8982, #40981, #41928, .T. ) ;
#57728=CARTESIAN_POINT ( 'NONE',  ( -35.00000000000000000, 3.640372113593719927, -12.21925492305358318 ) ) ;
#57729=ORIENTED_EDGE ( 'NONE', *, *, #13889, .F. ) ;
#57732=DIRECTION ( 'NONE',  ( 1.000000000000000000, -0.000000000000000000, 0.000000000000000000 ) ) ;
#57734=EDGE_CURVE ( 'NONE', #33841, #1348, #14964, .T. ) ;
#57735=CARTESIAN_POINT ( 'NONE',  ( -37.00000000000000711, -4.603882218679629545, 10.80631716521665453 ) ) ;
#57741=EDGE_CURVE ( 'NONE', #39147, #50042, #62496, .T. ) ;
#57742=CARTESIAN_POINT ( 'NONE',  ( -36.00000000000000711, 3.805206332242643263, -12.16893194857546412 ) ) ;
#57743=ORIENTED_EDGE ( 'NONE', *, *, #172, .F. ) ;
#57746=PRODUCT_CONTEXT ( 'NONE', #9387, 'mechanical' ) ;
#57748=CARTESIAN_POINT ( 'NONE',  ( -3.978895040306493769, 10.13474746098345491, 6.440914979617118341 ) ) ;
#57751=CARTESIAN_POINT ( 'NONE',  ( 35.00000000000000000, 12.09831040184923978, -1.463443770872822736 ) ) ;
#57753=AXIS2_PLACEMENT_3D ( 'NONE', #45686, #14434, #145 ) ;
#57756=ADVANCED_FACE ( 'NONE', ( #689 ), #20643, .T. ) ;
#57758=CIRCLE ( 'NONE', #65186, 5.000000000000000000 ) ;
#57760=ORIENTED_EDGE ( 'NONE', *, *, #62906, .F. ) ;
#57761=CARTESIAN_POINT ( 'NONE',  ( 11.74548640120467979, -10.73597826697111124, -8.184666801472349817 ) ) ;
#57762=DIRECTION ( 'NONE',  ( -1.000000000000000000, 0.000000000000000000, 0.000000000000000000 ) ) ;
#57763=CARTESIAN_POINT ( 'NONE',  ( 36.00000000000000711, 11.80185301892980654, -4.824807283154167514 ) ) ;
#57765=CARTESIAN_POINT ( 'NONE',  ( 35.00000000000000000, -3.473736367725341001, -12.26766708251990323 ) ) ;
#57766=CARTESIAN_POINT ( 'NONE',  ( -27.19357181888462094, -10.84410562793472543, 5.138615876886901468 ) ) ;
#57767=AXIS2_PLACEMENT_3D ( 'NONE', #50544, #15594, #9967 ) ;
#57769=DIRECTION ( 'NONE',  ( 1.000000000000000000, 0.000000000000000000, 0.000000000000000000 ) ) ;
#57771=CARTESIAN_POINT ( 'NONE',  ( 35.00000000000000000, 4.705694406421931860E-17, -3.469127814946512892E-15 ) ) ;
#57772=ORIENTED_EDGE ( 'NONE', *, *, #33348, .T. ) ;
#57773=CARTESIAN_POINT ( 'NONE',  ( 36.00000000000000711, 6.018036132182164266, -11.24036214326523009 ) ) ;
#57774=CARTESIAN_POINT ( 'NONE',  ( -9.343255928485906026, -12.02898473248699496, -6.138655790224737174 ) ) ;
#57775=VECTOR ( 'NONE', #21285, 1000.000000000000000 ) ;
#57777=AXIS2_PLACEMENT_3D ( 'NONE', #53159, #1965, #17262 ) ;
#57778=FACE_OUTER_BOUND ( 'NONE', #12657, .T. ) ;
#57780=ORIENTED_EDGE ( 'NONE', *, *, #4708, .F. ) ;
#57782=CIRCLE ( 'NONE', #37592, 12.18649999999999700 ) ;
#57784=FACE_OUTER_BOUND ( 'NONE', #52089, .T. ) ;
#57785=DIRECTION ( 'NONE',  ( 1.000000000000000000, -0.000000000000000000, 0.000000000000000000 ) ) ;
#57787=DIRECTION ( 'NONE',  ( 0.000000000000000000, 0.01356324068817998940, -0.9999080150203990547 ) ) ;
#57791=DIRECTION ( 'NONE',  ( -1.000000000000000000, -0.000000000000000000, -0.000000000000000000 ) ) ;
#57792=CYLINDRICAL_SURFACE ( 'NONE', #1448, 12.18649999999999878 ) ;
#57793=CARTESIAN_POINT ( 'NONE',  ( 35.00000000000000000, 6.475373545682446164, 10.32377448871660519 ) ) ;
#57794=AXIS2_PLACEMENT_3D ( 'NONE', #17457, #56732, #16479 ) ;
#57795=EDGE_CURVE ( 'NONE', #41918, #64690, #26383, .T. ) ;
#57796=FACE_OUTER_BOUND ( 'NONE', #42633, .T. ) ;
#57799=LINE ( 'NONE', #7561, #40254 ) ;
#57800=EDGE_LOOP ( 'NONE', ( #13943, #36972, #37549, #35618 ) ) ;
#57801=CARTESIAN_POINT ( 'NONE',  ( -6.514004847085159255, -1.134796399304650372, -13.45231326553087747 ) ) ;
#57803=DIRECTION ( 'NONE',  ( 1.000000000000000000, -0.000000000000000000, 0.000000000000000000 ) ) ;
#57804=DIRECTION ( 'NONE',  ( 0.3509218304786018705, 0.9364047569793457759, 0.000000000000000000 ) ) ;
#57806=DIRECTION ( 'NONE',  ( 0.000000000000000000, 0.01356324068817998940, -0.9999080150203990547 ) ) ;
#57807=AXIS2_PLACEMENT_3D ( 'NONE', #31002, #11371, #57605 ) ;
#57810=ORIENTED_EDGE ( 'NONE', *, *, #39569, .F. ) ;
#57812=ORIENTED_EDGE ( 'NONE', *, *, #29268, .T. ) ;
#57813=CARTESIAN_POINT ( 'NONE',  ( 2.706962116719304312, 3.188935572973642607, 11.57463990576596302 ) ) ;
#57814=DIRECTION ( 'NONE',  ( 1.000000000000000000, -0.000000000000000000, 0.000000000000000000 ) ) ;
#57815=CYLINDRICAL_SURFACE ( 'NONE', #44781, 4.999999999999999112 ) ;
#57816=DIRECTION ( 'NONE',  ( -1.000000000000000000, 0.000000000000000000, 0.000000000000000000 ) ) ;
#57817=DIRECTION ( 'NONE',  ( 0.000000000000000000, 0.01356324068817991828, -0.9999080150203990547 ) ) ;
#57818=EDGE_CURVE ( 'NONE', #25796, #17080, #20032, .T. ) ;
#57820=CYLINDRICAL_SURFACE ( 'NONE', #36103, 13.50000000000000178 ) ;
#57822=ADVANCED_FACE ( 'NONE', ( #1349 ), #22258, .T. ) ;
#57825=CARTESIAN_POINT ( 'NONE',  ( -35.00000000000000000, -12.09831040184925044, 1.463443770872731919 ) ) ;
#57830=DIRECTION ( 'NONE',  ( 0.000000000000000000, -0.01356324068817999114, 0.9999080150203989437 ) ) ;
#57831=EDGE_LOOP ( 'NONE', ( #43936, #26378, #64546, #53709 ) ) ;
#57832=CARTESIAN_POINT ( 'NONE',  ( -37.00000000000000711, -11.66953048682402283, 3.511814412392074480 ) ) ;
#57835=EDGE_CURVE ( 'NONE', #19802, #14030, #12609, .T. ) ;
#57837=VERTEX_POINT ( 'NONE', #17625 ) ;
#57839=VERTEX_POINT ( 'NONE', #11628 ) ;
#57845=VERTEX_POINT ( 'NONE', #31898 ) ;
#57848=AXIS2_PLACEMENT_3D ( 'NONE', #58377, #16816, #37093 ) ;
#57850=DIRECTION ( 'NONE',  ( 1.000000000000000000, 0.000000000000000000, 0.000000000000000000 ) ) ;
#57851=FACE_OUTER_BOUND ( 'NONE', #8221, .T. ) ;
#57852=CYLINDRICAL_SURFACE ( 'NONE', #1590, 4.999999999999999112 ) ;
#57853=ADVANCED_FACE ( 'NONE', ( #47235 ), #52858, .T. ) ;
#57854=CARTESIAN_POINT ( 'NONE',  ( 17.27839441901508977, 12.20388373500084711, 5.771933972472493402 ) ) ;
#57856=CARTESIAN_POINT ( 'NONE',  ( -35.00000000000000000, -10.80478261802186246, 5.636262487437281976 ) ) ;
#57858=EDGE_CURVE ( 'NONE', #50610, #25109, #21106, .T. ) ;
#57861=CARTESIAN_POINT ( 'NONE',  ( -35.00000000000000000, 0.000000000000000000, 0.000000000000000000 ) ) ;
#57862=CARTESIAN_POINT ( 'NONE',  ( 35.00000000000000000, -5.814360711498364864, -10.70999494708490829 ) ) ;
#57864=CARTESIAN_POINT ( 'NONE',  ( -14.65220012252043880, 8.414276895534435141, -8.555797441148357052 ) ) ;
#57865=ORIENTED_EDGE ( 'NONE', *, *, #14678, .F. ) ;
#57869=CYLINDRICAL_SURFACE ( 'NONE', #16040, 12.18650000000000055 ) ;
#57873=CARTESIAN_POINT ( 'NONE',  ( 37.00000000000000711, -7.499679039483992504, 9.040300684349768190 ) ) ;
#57874=CARTESIAN_POINT ( 'NONE',  ( -35.00000000000000000, 9.752226076388895493, 6.547236723514054724 ) ) ;
#57875=CARTESIAN_POINT ( 'NONE',  ( 35.00000000000000000, -5.015831474386232891, 10.62137734850272786 ) ) ;
#57876=CARTESIAN_POINT ( 'NONE',  ( -3.964071950788559562, 10.45352654835910045, 8.551872867741371564 ) ) ;
#57879=CARTESIAN_POINT ( 'NONE',  ( 37.00000000000000711, 9.733281772932162568, -8.235637554476683775 ) ) ;
#57880=CIRCLE ( 'NONE', #37685, 12.74999999999999822 ) ;
#57884=DIRECTION ( 'NONE',  ( 1.000000000000000000, 0.000000000000000000, 0.000000000000000000 ) ) ;
#57886=AXIS2_PLACEMENT_3D ( 'NONE', #64512, #44552, #64832 ) ;
#57888=AXIS2_PLACEMENT_3D ( 'NONE', #50697, #41346, #41026 ) ;
#57892=CARTESIAN_POINT ( 'NONE',  ( 12.47628546223243617, 0.000000000000000000, 13.50000000000000178 ) ) ;
#57893=( BOUNDED_CURVE ( )  B_SPLINE_CURVE ( 3, ( #6850, #3095, #53952, #58963 ),
 .UNSPECIFIED., .F., .F. ) 
 B_SPLINE_CURVE_WITH_KNOTS ( ( 4, 4 ),
 ( 1.796926956229685013, 1.827009492773266297 ),
 .UNSPECIFIED. ) 
 CURVE ( )  GEOMETRIC_REPRESENTATION_ITEM ( )  RATIONAL_B_SPLINE_CURVE ( ( 1.000000000000000000, 0.9999245881713708650, 0.9999245881713708650, 1.000000000000000000 ) ) 
 REPRESENTATION_ITEM ( '' )  );
#57899=EDGE_CURVE ( 'NONE', #18117, #13538, #54168, .T. ) ;
#57900=VERTEX_POINT ( 'NONE', #18280 ) ;
#57903=VECTOR ( 'NONE', #20718, 1000.000000000000000 ) ;
#57904=DIRECTION ( 'NONE',  ( -0.000000000000000000, -0.000000000000000000, -1.000000000000000000 ) ) ;
#57906=DIRECTION ( 'NONE',  ( 0.000000000000000000, -0.01356324068817999114, 0.9999080150203989437 ) ) ;
#57907=DIRECTION ( 'NONE',  ( 0.000000000000000000, -1.000000000000000000, 0.000000000000000000 ) ) ;
#57908=ORIENTED_EDGE ( 'NONE', *, *, #29370, .F. ) ;
#57912=ORIENTED_EDGE ( 'NONE', *, *, #36858, .F. ) ;
#57915=VERTEX_POINT ( 'NONE', #13583 ) ;
#57917=EDGE_CURVE ( 'NONE', #36458, #38941, #38047, .T. ) ;
#57918=CARTESIAN_POINT ( 'NONE',  ( 37.00000000000000711, 4.705694406421931860E-17, -3.469127814946512892E-15 ) ) ;
#57919=DIRECTION ( 'NONE',  ( 1.000000000000000000, 0.000000000000000000, -0.000000000000000000 ) ) ;
#57921=DIRECTION ( 'NONE',  ( 1.000000000000000000, -0.000000000000000000, 0.000000000000000000 ) ) ;
#57922=DIRECTION ( 'NONE',  ( 1.000000000000000000, 0.000000000000000000, 0.000000000000000000 ) ) ;
#57923=DIRECTION ( 'NONE',  ( 0.000000000000000000, 0.8827602140260297769, -0.4698238015817396418 ) ) ;
#57924=VERTEX_POINT ( 'NONE', #59479 ) ;
#57925=ADVANCED_FACE ( 'NONE', ( #39185 ), #3660, .T. ) ;
#57926=CYLINDRICAL_SURFACE ( 'NONE', #18460, 12.00000000000000000 ) ;
#57927=CIRCLE ( 'NONE', #56885, 12.18649999999999878 ) ;
#57928=ORIENTED_EDGE ( 'NONE', *, *, #19881, .F. ) ;
#57929=CYLINDRICAL_SURFACE ( 'NONE', #46583, 4.999999999999999112 ) ;
#57931=EDGE_CURVE ( 'NONE', #41192, #44052, #13595, .T. ) ;
#57936=CIRCLE ( 'NONE', #590, 12.74999999999999822 ) ;
#57937=ORIENTED_EDGE ( 'NONE', *, *, #15696, .T. ) ;
#57939=CARTESIAN_POINT ( 'NONE',  ( -35.00000000000000000, 8.927548052241016663, -8.295159312811756891 ) ) ;
#57940=EDGE_LOOP ( 'NONE', ( #32591, #32204, #41491, #2012 ) ) ;
#57941=CARTESIAN_POINT ( 'NONE',  ( -35.00000000000000000, 10.63508530065528923, -4.986700593229593359 ) ) ;
#57942=CARTESIAN_POINT ( 'NONE',  ( -47.00000000000000711, 0.000000000000000000, 0.000000000000000000 ) ) ;
#57943=DIRECTION ( 'NONE',  ( 0.000000000000000000, 0.3807014730195152907, -0.9246979985058750851 ) ) ;
#57945=ORIENTED_EDGE ( 'NONE', *, *, #61213, .T. ) ;
#57947=VECTOR ( 'NONE', #59171, 1000.000000000000000 ) ;
#57948=EDGE_CURVE ( 'NONE', #57258, #49577, #46566, .T. ) ;
#57952=LINE ( 'NONE', #17381, #22437 ) ;
#57958=EDGE_CURVE ( 'NONE', #51664, #63220, #57212, .T. ) ;
#57959=ORIENTED_EDGE ( 'NONE', *, *, #28234, .F. ) ;
#57963=ORIENTED_EDGE ( 'NONE', *, *, #21774, .T. ) ;
#57965=CARTESIAN_POINT ( 'NONE',  ( 36.00000000000000711, 12.57916205664484188, 2.080187960898426169 ) ) ;
#57968=ORIENTED_EDGE ( 'NONE', *, *, #42884, .T. ) ;
#57970=PLANE ( 'NONE',  #13675 ) ;
#57971=VERTEX_POINT ( 'NONE', #34197 ) ;
#57973=EDGE_CURVE ( 'NONE', #60414, #19006, #17939, .T. ) ;
#57974=AXIS2_PLACEMENT_3D ( 'NONE', #46054, #40722, #26096 ) ;
#57976=VERTEX_POINT ( 'NONE', #23250 ) ;
#57977=CARTESIAN_POINT ( 'NONE',  ( -47.00000000000000711, 0.000000000000000000, 0.000000000000000000 ) ) ;
#57978=CARTESIAN_POINT ( 'NONE',  ( 3.864517994186338790, 5.325084099531887993, 12.40733688370094256 ) ) ;
#57979=CARTESIAN_POINT ( 'NONE',  ( 35.00000000000000000, -10.12742074351890764, 7.745827850123116143 ) ) ;
#57982=DIRECTION ( 'NONE',  ( -1.000000000000000000, 0.000000000000000000, 0.000000000000000000 ) ) ;
#57984=DIRECTION ( 'NONE',  ( 0.000000000000000000, -0.4134677391718385997, -0.9105187689796011563 ) ) ;
#57985=CARTESIAN_POINT ( 'NONE',  ( -24.54625327245882360, 6.852894237372495034, 9.860103603378655990 ) ) ;
#57986=ORIENTED_EDGE ( 'NONE', *, *, #24742, .F. ) ;
#57988=ORIENTED_EDGE ( 'NONE', *, *, #28770, .T. ) ;
#57989=CYLINDRICAL_SURFACE ( 'NONE', #62473, 5.000000000000000888 ) ;
#57991=FACE_OUTER_BOUND ( 'NONE', #444, .T. ) ;
#57994=CARTESIAN_POINT ( 'NONE',  ( 35.00000000000000000, 4.705694406421931860E-17, -3.469127814946512892E-15 ) ) ;
#57996=DIRECTION ( 'NONE',  ( -1.000000000000000000, 0.000000000000000000, -0.000000000000000000 ) ) ;
#58000=EDGE_CURVE ( 'NONE', #52203, #57900, #34849, .T. ) ;
#58001=ORIENTED_EDGE ( 'NONE', *, *, #25207, .F. ) ;
#58003=VERTEX_POINT ( 'NONE', #8288 ) ;
#58004=EDGE_CURVE ( 'NONE', #11187, #21416, #42302, .T. ) ;
#58007=CARTESIAN_POINT ( 'NONE',  ( -18.04845295627699286, -11.93556515273317942, 1.283449352624662199 ) ) ;
#58008=DIRECTION ( 'NONE',  ( -1.000000000000000000, 0.000000000000000000, -0.000000000000000000 ) ) ;
#58010=CARTESIAN_POINT ( 'NONE',  ( -37.00000000000000711, 7.971186206369601734, -9.217970097227642157 ) ) ;
#58011=DIRECTION ( 'NONE',  ( 0.000000000000000000, -0.01356324068817998940, 0.9999080150203990547 ) ) ;
#58012=EDGE_CURVE ( 'NONE', #35021, #58885, #5225, .T. ) ;
#58013=VECTOR ( 'NONE', #15030, 1000.000000000000000 ) ;
#58014=DIRECTION ( 'NONE',  ( 1.000000000000000000, 0.000000000000000000, 0.000000000000000000 ) ) ;
#58017=CARTESIAN_POINT ( 'NONE',  ( 47.00000000000000711, 4.705694406421931860E-17, -3.469127814946512892E-15 ) ) ;
#58020=CARTESIAN_POINT ( 'NONE',  ( 35.00000000000000000, 11.78977382767499549, -4.245927698352105928 ) ) ;
#58021=DIRECTION ( 'NONE',  ( 0.000000000000000000, -0.01356324068817998940, 0.9999080150203990547 ) ) ;
#58022=EDGE_CURVE ( 'NONE', #57602, #52645, #45823, .T. ) ;
#58025=VERTEX_POINT ( 'NONE', #50813 ) ;
#58028=FACE_OUTER_BOUND ( 'NONE', #8876, .T. ) ;
#58030=EDGE_CURVE ( 'NONE', #15725, #40578, #15225, .T. ) ;
#58032=CARTESIAN_POINT ( 'NONE',  ( -26.18760594837597822, -12.07028982502884418, 6.047005920582382288 ) ) ;
#58033=VERTEX_POINT ( 'NONE', #60449 ) ;
#58035=DIRECTION ( 'NONE',  ( -1.000000000000000000, 0.000000000000000000, 0.000000000000000000 ) ) ;
#58037=ORIENTED_EDGE ( 'NONE', *, *, #58971, .T. ) ;
#58039=CARTESIAN_POINT ( 'NONE',  ( 35.00000000000000000, 4.705694406421931860E-17, -3.469127814946512892E-15 ) ) ;
#58040=ORIENTED_EDGE ( 'NONE', *, *, #38198, .F. ) ;
#58041=EDGE_CURVE ( 'NONE', #6845, #39606, #54072, .T. ) ;
#58042=ORIENTED_EDGE ( 'NONE', *, *, #30996, .T. ) ;
#58044=EDGE_CURVE ( 'NONE', #29266, #58976, #4906, .T. ) ;
#58045=AXIS2_PLACEMENT_3D ( 'NONE', #39300, #29020, #29334 ) ;
#58047=ORIENTED_EDGE ( 'NONE', *, *, #18199, .F. ) ;
#58051=CARTESIAN_POINT ( 'NONE',  ( -3.167554099594523720, -12.87069030742389764, 4.088466244554556539 ) ) ;
#58055=ORIENTED_EDGE ( 'NONE', *, *, #33599, .F. ) ;
#58056=CARTESIAN_POINT ( 'NONE',  ( 8.979959331610965378, 5.149046574253878461, 12.48452308162177538 ) ) ;
#58057=VERTEX_POINT ( 'NONE', #59812 ) ;
#58061=ORIENTED_EDGE ( 'NONE', *, *, #3584, .F. ) ;
#58063=CARTESIAN_POINT ( 'NONE',  ( 37.00000000000000711, 11.80185301892980654, -4.824807283154168402 ) ) ;
#58065=ADVANCED_FACE ( 'NONE', ( #24890 ), #65744, .T. ) ;
#58066=CARTESIAN_POINT ( 'NONE',  ( -4.046008612244236247, 9.338948392566903678, 7.538928574057408127 ) ) ;
#58067=CARTESIAN_POINT ( 'NONE',  ( -37.00000000000000711, -12.15823808070322265, -0.8294751490780611913 ) ) ;
#58068=LINE ( 'NONE', #47439, #26737 ) ;
#58069=ORIENTED_EDGE ( 'NONE', *, *, #57463, .T. ) ;
#58074=ORIENTED_EDGE ( 'NONE', *, *, #4374, .F. ) ;
#58077=ORIENTED_EDGE ( 'NONE', *, *, #35653, .F. ) ;
#58079=LINE ( 'NONE', #16192, #31924 ) ;
#58080=LINE ( 'NONE', #57763, #51166 ) ;
#58081=CARTESIAN_POINT ( 'NONE',  ( -37.00000000000000711, 0.000000000000000000, 0.000000000000000000 ) ) ;
#58084=CARTESIAN_POINT ( 'NONE',  ( -29.68541646480307250, -0.9867458123558492389, 13.47080766332845592 ) ) ;
#58090=CARTESIAN_POINT ( 'NONE',  ( -8.019454758349086276, -9.419150639783058665, -9.692301608309891847 ) ) ;
#58091=CARTESIAN_POINT ( 'NONE',  ( -37.00000000000000711, -11.95840593935199792, -2.346765782874564277 ) ) ;
#58092=VECTOR ( 'NONE', #57250, 1000.000000000000000 ) ;
#58094=ORIENTED_EDGE ( 'NONE', *, *, #29193, .T. ) ;
#58097=VECTOR ( 'NONE', #20012, 1000.000000000000000 ) ;
#58098=ADVANCED_FACE ( 'NONE', ( #60789 ), #50499, .T. ) ;
#58099=ORIENTED_EDGE ( 'NONE', *, *, #59433, .T. ) ;
#58100=CARTESIAN_POINT ( 'NONE',  ( 35.00000000000000000, -11.30684963584392477, -4.545979934229371189 ) ) ;
#58102=DIRECTION ( 'NONE',  ( 0.000000000000000000, 0.01356324068818000328, -0.9999080150203990547 ) ) ;
#58103=EDGE_CURVE ( 'NONE', #29107, #49616, #19034, .T. ) ;
#58105=EDGE_LOOP ( 'NONE', ( #28850, #7605, #43877, #33741 ) ) ;
#58111=DIRECTION ( 'NONE',  ( -1.000000000000000000, 0.000000000000000000, 0.000000000000000000 ) ) ;
#58112=CARTESIAN_POINT ( 'NONE',  ( -35.00000000000000000, 9.430788938294162094, -7.718225330433707398 ) ) ;
#58114=CARTESIAN_POINT ( 'NONE',  ( 145.1370849898475797, -13.49999999999996803, 0.000000000000000000 ) ) ;
#58117=VERTEX_POINT ( 'NONE', #3198 ) ;
#58118=CARTESIAN_POINT ( 'NONE',  ( -16.98800322446194855, 2.922502605998049674, -13.17987020110343543 ) ) ;
#58122=CARTESIAN_POINT ( 'NONE',  ( 35.00000000000000000, 2.216820770815085773, -11.53507381115584529 ) ) ;
#58123=CARTESIAN_POINT ( 'NONE',  ( 3.423896178748678576, -10.94279856996580413, 7.910751437345123982 ) ) ;
#58124=ORIENTED_EDGE ( 'NONE', *, *, #7201, .F. ) ;
#58125=ORIENTED_EDGE ( 'NONE', *, *, #10018, .F. ) ;
#58126=FACE_OUTER_BOUND ( 'NONE', #21919, .T. ) ;
#58127=ORIENTED_EDGE ( 'NONE', *, *, #15156, .F. ) ;
#58128=CARTESIAN_POINT ( 'NONE',  ( 2.316650205446322719, 2.457467282897404459, 11.75170002979209194 ) ) ;
#58135=ORIENTED_EDGE ( 'NONE', *, *, #60221, .F. ) ;
#58136=ORIENTED_EDGE ( 'NONE', *, *, #20957, .F. ) ;
#58137=CARTESIAN_POINT ( 'NONE',  ( -35.00000000000000000, 0.000000000000000000, 0.000000000000000000 ) ) ;
#58140=DIRECTION ( 'NONE',  ( 0.000000000000000000, 0.01356324068817998940, -0.9999080150203990547 ) ) ;
#58142=AXIS2_PLACEMENT_3D ( 'NONE', #47029, #16093, #51698 ) ;
#58147=DIRECTION ( 'NONE',  ( 0.000000000000000000, -0.9999080150203989437, -0.01356324068819032662 ) ) ;
#58148=EDGE_CURVE ( 'NONE', #57924, #48534, #62537, .T. ) ;
#58149=ORIENTED_EDGE ( 'NONE', *, *, #18034, .T. ) ;
#58150=EDGE_LOOP ( 'NONE', ( #8210, #27545, #29824, #60755 ) ) ;
#58152=ORIENTED_EDGE ( 'NONE', *, *, #32975, .T. ) ;
#58153=ORIENTED_EDGE ( 'NONE', *, *, #60954, .T. ) ;
#58154=CYLINDRICAL_SURFACE ( 'NONE', #38632, 5.000000000000000888 ) ;
#58155=ORIENTED_EDGE ( 'NONE', *, *, #11229, .F. ) ;
#58156=ORIENTED_EDGE ( 'NONE', *, *, #39840, .T. ) ;
#58160=CARTESIAN_POINT ( 'NONE',  ( -20.95894390668759044, -11.53024028107489585, -3.336574098666279742 ) ) ;
#58161=LINE ( 'NONE', #12266, #55316 ) ;
#58162=CARTESIAN_POINT ( 'NONE',  ( 37.00000000000000711, 12.66641127287627810, 1.457575200925408820 ) ) ;
#58164=LINE ( 'NONE', #57856, #22180 ) ;
#58167=CARTESIAN_POINT ( 'NONE',  ( -37.00000000000000711, 0.000000000000000000, 0.000000000000000000 ) ) ;
#58168=CYLINDRICAL_SURFACE ( 'NONE', #32873, 4.999999999999999112 ) ;
#58169=FACE_OUTER_BOUND ( 'NONE', #59931, .T. ) ;
#58171=DIRECTION ( 'NONE',  ( 1.000000000000000000, 0.000000000000000000, 0.000000000000000000 ) ) ;
#58172=CIRCLE ( 'NONE', #29472, 5.000000000000000888 ) ;
#58174=ORIENTED_EDGE ( 'NONE', *, *, #1871, .T. ) ;
#58175=CARTESIAN_POINT ( 'NONE',  ( -35.00000000000000000, -9.677500615117949678, 6.657191900728284928 ) ) ;
#58176=CIRCLE ( 'NONE', #49726, 5.000000000000000888 ) ;
#58178=EDGE_CURVE ( 'NONE', #45342, #51818, #11252, .T. ) ;
#58181=CARTESIAN_POINT ( 'NONE',  ( 12.44547025303417698, -13.08988633905116039, -3.306802340674645180 ) ) ;
#58182=DIRECTION ( 'NONE',  ( 1.000000000000000000, 0.000000000000000000, 0.000000000000000000 ) ) ;
#58185=ORIENTED_EDGE ( 'NONE', *, *, #16120, .F. ) ;
#58186=DIRECTION ( 'NONE',  ( -1.000000000000000000, -0.000000000000000000, 0.000000000000000000 ) ) ;
#58187=DIRECTION ( 'NONE',  ( 0.000000000000000000, -0.01356324068817998940, 0.9999080150203990547 ) ) ;
#58188=CARTESIAN_POINT ( 'NONE',  ( 35.00000000000000000, -8.017674001891711200, 9.913596905230193101 ) ) ;
#58191=AXIS2_PLACEMENT_3D ( 'NONE', #38007, #13081, #22742 ) ;
#58192=EDGE_CURVE ( 'NONE', #43264, #6288, #23261, .T. ) ;
#58195=EDGE_CURVE ( 'NONE', #54568, #52675, #18152, .T. ) ;
#58197=CARTESIAN_POINT ( 'NONE',  ( 3.780834652287974773, 8.352030633203074927, -8.616471685210672860 ) ) ;
#58198=ORIENTED_EDGE ( 'NONE', *, *, #16648, .F. ) ;
#58199=DIRECTION ( 'NONE',  ( -1.000000000000000000, 0.000000000000000000, 0.000000000000000000 ) ) ;
#58200=EDGE_CURVE ( 'NONE', #54327, #16429, #11569, .T. ) ;
#58201=EDGE_LOOP ( 'NONE', ( #867, #33840, #62658, #29185 ) ) ;
#58203=DIRECTION ( 'NONE',  ( 1.000000000000000000, 0.000000000000000000, 0.000000000000000000 ) ) ;
#58204=FACE_OUTER_BOUND ( 'NONE', #1790, .T. ) ;
#58205=CARTESIAN_POINT ( 'NONE',  ( 12.93723047338301058, 4.476360154859203355, 25.00000000000000000 ) ) ;
#58206=EDGE_CURVE ( 'NONE', #6535, #24257, #58741, .T. ) ;
#58208=ORIENTED_EDGE ( 'NONE', *, *, #4514, .F. ) ;
#58209=ORIENTED_EDGE ( 'NONE', *, *, #6181, .F. ) ;
#58210=ORIENTED_EDGE ( 'NONE', *, *, #17109, .F. ) ;
#58211=CARTESIAN_POINT ( 'NONE',  ( -37.00000000000000711, 5.428340790341860789, -10.91072401419405402 ) ) ;
#58212=AXIS2_PLACEMENT_3D ( 'NONE', #46536, #2312, #31254 ) ;
#58215=CARTESIAN_POINT ( 'NONE',  ( -35.00000000000000000, -5.672855678558757830, 10.28547182238005853 ) ) ;
#58216=DIRECTION ( 'NONE',  ( 1.000000000000000000, 0.000000000000000000, 0.000000000000000000 ) ) ;
#58217=EDGE_LOOP ( 'NONE', ( #5043, #29603, #2887, #50782 ) ) ;
#58218=LINE ( 'NONE', #32918, #34341 ) ;
#58221=ORIENTED_EDGE ( 'NONE', *, *, #57016, .T. ) ;
#58222=VERTEX_POINT ( 'NONE', #59059 ) ;
#58226=ORIENTED_EDGE ( 'NONE', *, *, #12443, .F. ) ;
#58227=VECTOR ( 'NONE', #49364, 1000.000000000000000 ) ;
#58230=DIRECTION ( 'NONE',  ( 0.000000000000000000, -0.01356324068817991828, 0.9999080150203990547 ) ) ;
#58233=LINE ( 'NONE', #12654, #11779 ) ;
#58234=FACE_OUTER_BOUND ( 'NONE', #22125, .T. ) ;
#58235=DIRECTION ( 'NONE',  ( 1.000000000000000000, 0.000000000000000000, 0.000000000000000000 ) ) ;
#58236=ORIENTED_EDGE ( 'NONE', *, *, #65090, .F. ) ;
#58237=DIRECTION ( 'NONE',  ( 1.000000000000000000, 0.000000000000000000, -0.000000000000000000 ) ) ;
#58238=ORIENTED_EDGE ( 'NONE', *, *, #59047, .F. ) ;
#58240=DIRECTION ( 'NONE',  ( 0.000000000000000000, -0.01356324068817999114, 0.9999080150203989437 ) ) ;
#58245=DIRECTION ( 'NONE',  ( -0.000000000000000000, -1.000000000000000000, -0.000000000000000000 ) ) ;
#58246=ORIENTED_EDGE ( 'NONE', *, *, #41255, .F. ) ;
#58248=AXIS2_PLACEMENT_3D ( 'NONE', #23755, #29377, #24724 ) ;
#58249=ADVANCED_FACE ( 'NONE', ( #55224 ), #33954, .T. ) ;
#58250=VERTEX_POINT ( 'NONE', #34287 ) ;
#58253=CIRCLE ( 'NONE', #39100, 12.74999999999999822 ) ;
#58254=ORIENTED_EDGE ( 'NONE', *, *, #57727, .T. ) ;
#58257=CARTESIAN_POINT ( 'NONE',  ( -3.547682422092472976, -11.41132889151838725, 7.222740821714795700 ) ) ;
#58258=EDGE_CURVE ( 'NONE', #62820, #47648, #23296, .T. ) ;
#58259=DIRECTION ( 'NONE',  ( -1.000000000000000000, -0.000000000000000000, 0.000000000000000000 ) ) ;
#58261=DIRECTION ( 'NONE',  ( -1.000000000000000000, -0.000000000000000000, 0.000000000000000000 ) ) ;
#58262=CIRCLE ( 'NONE', #46575, 5.000000000000000888 ) ;
#58264=CIRCLE ( 'NONE', #45387, 12.18650000000000411 ) ;
#58266=( BOUNDED_CURVE ( )  B_SPLINE_CURVE ( 3, ( #58197, #18637, #54187, #17640 ),
 .UNSPECIFIED., .F., .F. ) 
 B_SPLINE_CURVE_WITH_KNOTS ( ( 4, 4 ),
 ( 3.942573786070413977, 3.954312062358601221 ),
 .UNSPECIFIED. ) 
 CURVE ( )  GEOMETRIC_REPRESENTATION_ITEM ( )  RATIONAL_B_SPLINE_CURVE ( ( 1.000000000000000000, 0.9999885177721090646, 0.9999885177721090646, 1.000000000000000000 ) ) 
 REPRESENTATION_ITEM ( '' )  );
#58267=EDGE_CURVE ( 'NONE', #41839, #9878, #48762, .T. ) ;
#58268=CARTESIAN_POINT ( 'NONE',  ( 21.98157680265827452, 12.95962480054460819, -3.798644489114345824 ) ) ;
#58270=VECTOR ( 'NONE', #1337, 1000.000000000000000 ) ;
#58271=EDGE_CURVE ( 'NONE', #22647, #48416, #46650, .T. ) ;
#58272=FACE_OUTER_BOUND ( 'NONE', #34701, .T. ) ;
#58275=AXIS2_PLACEMENT_3D ( 'NONE', #43501, #64132, #65097 ) ;
#58276=EDGE_CURVE ( 'NONE', #18784, #10110, #37254, .T. ) ;
#58277=ORIENTED_EDGE ( 'NONE', *, *, #59384, .F. ) ;
#58279=CARTESIAN_POINT ( 'NONE',  ( 12.17435499564740908, -9.235710332726100091, -7.670499671992002888 ) ) ;
#58280=ORIENTED_EDGE ( 'NONE', *, *, #30358, .T. ) ;
#58281=CARTESIAN_POINT ( 'NONE',  ( 35.00000000000000000, 11.47561260193577048, -5.556331110570448040 ) ) ;
#58283=DIRECTION ( 'NONE',  ( 0.000000000000000000, -0.01356324068817999114, 0.9999080150203989437 ) ) ;
#58284=VERTEX_POINT ( 'NONE', #49599 ) ;
#58285=EDGE_CURVE ( 'NONE', #53955, #5474, #42351, .T. ) ;
#58287=DIRECTION ( 'NONE',  ( 0.000000000000000000, 0.1118654143051546479, 0.9937233664769768993 ) ) ;
#58288=ORIENTED_EDGE ( 'NONE', *, *, #38401, .T. ) ;
#58289=LINE ( 'NONE', #12706, #12618 ) ;
#58290=VERTEX_POINT ( 'NONE', #34914 ) ;
#58291=ORIENTED_EDGE ( 'NONE', *, *, #65228, .F. ) ;
#58292=CARTESIAN_POINT ( 'NONE',  ( -10.48620311856347875, -9.720786832536937538, -7.036071585506805448 ) ) ;
#58294=CIRCLE ( 'NONE', #27472, 12.74999999999999822 ) ;
#58295=ORIENTED_EDGE ( 'NONE', *, *, #64345, .F. ) ;
#58297=FACE_OUTER_BOUND ( 'NONE', #41032, .T. ) ;
#58298=DIRECTION ( 'NONE',  ( 1.000000000000000000, -0.000000000000000000, 0.000000000000000000 ) ) ;
#58299=CARTESIAN_POINT ( 'NONE',  ( -47.00000000000000711, 0.000000000000000000, 0.000000000000000000 ) ) ;
#58300=VERTEX_POINT ( 'NONE', #50903 ) ;
#58301=CARTESIAN_POINT ( 'NONE',  ( -37.00000000000000711, 0.000000000000000000, 0.000000000000000000 ) ) ;
#58304=CARTESIAN_POINT ( 'NONE',  ( 47.00000000000000711, 4.705694406421931860E-17, -3.469127814946512892E-15 ) ) ;
#58305=ORIENTED_EDGE ( 'NONE', *, *, #61374, .T. ) ;
#58306=CARTESIAN_POINT ( 'NONE',  ( -27.45775109278351067, 11.83395752356219077, -1.989333891161980894 ) ) ;
#58308=CARTESIAN_POINT ( 'NONE',  ( -35.00000000000000000, -8.052525312709946093, 8.551552972817052733 ) ) ;
#58310=DIRECTION ( 'NONE',  ( -1.000000000000000000, 0.000000000000000000, 0.000000000000000000 ) ) ;
#58311=CARTESIAN_POINT ( 'NONE',  ( 35.00000000000000000, 1.285879139104720949E-14, 0.000000000000000000 ) ) ;
#58312=AXIS2_PLACEMENT_3D ( 'NONE', #32814, #2266, #57804 ) ;
#58317=DIRECTION ( 'NONE',  ( 0.000000000000000000, -0.9903235168508535136, -0.1387779952735920808 ) ) ;
#58318=CARTESIAN_POINT ( 'NONE',  ( 13.15812208069034384, 12.98105700980179833, -3.712867825188221449 ) ) ;
#58319=VERTEX_POINT ( 'NONE', #41229 ) ;
#58322=FACE_OUTER_BOUND ( 'NONE', #16539, .T. ) ;
#58323=ORIENTED_EDGE ( 'NONE', *, *, #21566, .F. ) ;
#58325=ORIENTED_EDGE ( 'NONE', *, *, #54179, .F. ) ;
#58329=AXIS2_PLACEMENT_3D ( 'NONE', #2497, #63304, #18099 ) ;
#58335=ORIENTED_EDGE ( 'NONE', *, *, #45056, .F. ) ;
#58339=EDGE_CURVE ( 'NONE', #53221, #17893, #6276, .T. ) ;
#58340=DIRECTION ( 'NONE',  ( -1.000000000000000000, 0.000000000000000000, 0.000000000000000000 ) ) ;
#58341=DIRECTION ( 'NONE',  ( 1.000000000000000000, 0.000000000000000000, 0.000000000000000000 ) ) ;
#58346=VERTEX_POINT ( 'NONE', #51891 ) ;
#58347=FACE_OUTER_BOUND ( 'NONE', #29307, .T. ) ;
#58351=CIRCLE ( 'NONE', #63601, 11.99999999999999822 ) ;
#58352=EDGE_CURVE ( 'NONE', #743, #18633, #60412, .T. ) ;
#58357=CARTESIAN_POINT ( 'NONE',  ( 47.00000000000000711, 4.705694406421931860E-17, -3.469127814946512892E-15 ) ) ;
#58358=DIRECTION ( 'NONE',  ( -1.000000000000000000, 0.000000000000000000, -0.000000000000000000 ) ) ;
#58359=CARTESIAN_POINT ( 'NONE',  ( 35.00000000000000000, -11.02904044024205987, 4.041347439435972966 ) ) ;
#58366=VERTEX_POINT ( 'NONE', #1353 ) ;
#58367=CARTESIAN_POINT ( 'NONE',  ( -37.00000000000000711, 3.704519465651306742, 11.60979404548636218 ) ) ;
#58370=ORIENTED_EDGE ( 'NONE', *, *, #19413, .T. ) ;
#58371=CIRCLE ( 'NONE', #30728, 4.999999999999999112 ) ;
#58374=CARTESIAN_POINT ( 'NONE',  ( 35.00000000000000000, 12.15823808070323508, 0.8294751490777961811 ) ) ;
#58377=CARTESIAN_POINT ( 'NONE',  ( -37.00000000000000711, -11.26103545359858060, 3.340853584269496412 ) ) ;
#58381=ORIENTED_EDGE ( 'NONE', *, *, #26876, .F. ) ;
#58386=CARTESIAN_POINT ( 'NONE',  ( -27.27855387000350262, 25.00000000000000000, 5.631341004100471892 ) ) ;
#58388=CARTESIAN_POINT ( 'NONE',  ( -3.908294913248263835, 8.114081195363114674, 8.852078639661073112 ) ) ;
#58389=AXIS2_PLACEMENT_3D ( 'NONE', #23169, #64374, #13819 ) ;
#58390=AXIS2_PLACEMENT_3D ( 'NONE', #10889, #602, #30189 ) ;
#58391=CARTESIAN_POINT ( 'NONE',  ( 35.00000000000000000, -8.854740511458901508, -7.717887834988215623 ) ) ;
#58393=VERTEX_POINT ( 'NONE', #51246 ) ;
#58394=EDGE_CURVE ( 'NONE', #35661, #45163, #44502, .T. ) ;
#58395=CARTESIAN_POINT ( 'NONE',  ( -25.29745827051326756, -10.31977495403786627, 6.126035789533863074 ) ) ;
#58396=VECTOR ( 'NONE', #36487, 1000.000000000000000 ) ;
#58397=CARTESIAN_POINT ( 'NONE',  ( -35.00000000000000000, -11.65554240571058031, 1.456211999474302798 ) ) ;
#58401=ORIENTED_EDGE ( 'NONE', *, *, #25043, .F. ) ;
#58402=CARTESIAN_POINT ( 'NONE',  ( -37.00000000000000711, 10.23119532541083743, -7.608228585767615293 ) ) ;
#58403=ORIENTED_EDGE ( 'NONE', *, *, #17114, .F. ) ;
#58404=CARTESIAN_POINT ( 'NONE',  ( 35.00000000000000000, 3.916263239775349625, -11.07407352312214144 ) ) ;
#58407=CARTESIAN_POINT ( 'NONE',  ( -37.00000000000000711, 6.265926637539497079, 11.10408318471061584 ) ) ;
#58408=AXIS2_PLACEMENT_3D ( 'NONE', #21819, #62348, #1852 ) ;
#58409=CARTESIAN_POINT ( 'NONE',  ( 35.00000000000000000, -3.511814412392203266, -11.66953048682398730 ) ) ;
#58410=CARTESIAN_POINT ( 'NONE',  ( -29.57728396573499552, 0.08119487476310269236, 13.50144130734792292 ) ) ;
#58411=DIRECTION ( 'NONE',  ( 0.000000000000000000, 0.000000000000000000, -1.000000000000000000 ) ) ;
#58412=VECTOR ( 'NONE', #27592, 1000.000000000000000 ) ;
#58415=ORIENTED_EDGE ( 'NONE', *, *, #32438, .T. ) ;
#58417=B_SPLINE_CURVE_WITH_KNOTS ( 'NONE', 3,
 ( #22331, #12357, #62905, #28005, #17369, #32625, #7369, #38284, #33639, #37648, #42955, #53615, #3072, #47314, #63235, #48309, #2760, #23017 ),
 .UNSPECIFIED., .F., .F.,
 ( 4, 2, 2, 2, 2, 2, 2, 2, 4 ),
 ( 0.000000000000000000, 0.0009233824328804393286, 0.001385073649320658342, 0.001846764865760876922, 0.002770147298641318419, 0.003693529731521760350, 0.004616912164402201847, 0.005540294597282643778, 0.007387059463043525905 ),
 .UNSPECIFIED. ) ;
#58418=EDGE_CURVE ( 'NONE', #63537, #17242, #50891, .T. ) ;
#58422=CIRCLE ( 'NONE', #1080, 5.000000000000000888 ) ;
#58423=DIRECTION ( 'NONE',  ( 1.000000000000000000, 0.000000000000000000, -0.000000000000000000 ) ) ;
#58424=ADVANCED_FACE ( 'NONE', ( #16312 ), #36588, .F. ) ;
#58427=ORIENTED_EDGE ( 'NONE', *, *, #26123, .T. ) ;
#58438=AXIS2_PLACEMENT_3D ( 'NONE', #43595, #63885, #18364 ) ;
#58440=DIRECTION ( 'NONE',  ( -1.000000000000000000, 0.000000000000000000, -0.000000000000000000 ) ) ;
#58442=DIRECTION ( 'NONE',  ( -1.000000000000000000, -0.000000000000000000, -0.000000000000000000 ) ) ;
#58443=DIRECTION ( 'NONE',  ( 0.000000000000000000, 0.01356324068817998940, -0.9999080150203989437 ) ) ;
#58446=CARTESIAN_POINT ( 'NONE',  ( -18.08686583997275221, 5.151216734910927464, -12.47858029384662970 ) ) ;
#58447=CARTESIAN_POINT ( 'NONE',  ( 37.00000000000000711, -7.882940143791699050, 10.02106554660717030 ) ) ;
#58452=EDGE_CURVE ( 'NONE', #9460, #56593, #31730, .T. ) ;
#58454=DIRECTION ( 'NONE',  ( 0.000000000000000000, -0.01356324068817999114, 0.9999080150203990547 ) ) ;
#58456=AXIS2_PLACEMENT_3D ( 'NONE', #29473, #6196, #4892 ) ;
#58458=( BOUNDED_CURVE ( )  B_SPLINE_CURVE ( 3, ( #7496, #882, #21154, #3192 ),
 .UNSPECIFIED., .F., .F. ) 
 B_SPLINE_CURVE_WITH_KNOTS ( ( 4, 4 ),
 ( 1.852694126892728388, 1.873650368502720598 ),
 .UNSPECIFIED. ) 
 CURVE ( )  GEOMETRIC_REPRESENTATION_ITEM ( )  RATIONAL_B_SPLINE_CURVE ( ( 1.000000000000000000, 0.9999634033296326274, 0.9999634033296326274, 1.000000000000000000 ) ) 
 REPRESENTATION_ITEM ( '' )  );
#58462=DIRECTION ( 'NONE',  ( -1.000000000000000000, 0.000000000000000000, 0.000000000000000000 ) ) ;
#58464=CYLINDRICAL_SURFACE ( 'NONE', #27624, 12.74999999999999822 ) ;
#58466=ORIENTED_EDGE ( 'NONE', *, *, #22517, .F. ) ;
#58468=CIRCLE ( 'NONE', #1117, 12.74999999999999822 ) ;
#58469=ORIENTED_EDGE ( 'NONE', *, *, #31472, .T. ) ;
#58470=( LENGTH_UNIT ( ) NAMED_UNIT ( * ) SI_UNIT ( .MILLI., .METRE. ) );
#58474=VERTEX_POINT ( 'NONE', #11960 ) ;
#58475=CARTESIAN_POINT ( 'NONE',  ( -37.00000000000000711, 12.12087942037211263, -1.262958560998631796 ) ) ;
#58476=EDGE_CURVE ( 'NONE', #64903, #15913, #53192, .T. ) ;
#58481=DIRECTION ( 'NONE',  ( 1.000000000000000000, 0.000000000000000000, 0.000000000000000000 ) ) ;
#58483=VECTOR ( 'NONE', #36775, 1000.000000000000000 ) ;
#58485=DIRECTION ( 'NONE',  ( 0.000000000000000000, -0.9903235168508535136, -0.1387779952735920808 ) ) ;
#58486=ORIENTED_EDGE ( 'NONE', *, *, #42431, .F. ) ;
#58490=AXIS2_PLACEMENT_3D ( 'NONE', #44846, #34211, #18934 ) ;
#58492=VECTOR ( 'NONE', #55471, 1000.000000000000000 ) ;
#58493=LINE ( 'NONE', #17269, #64 ) ;
#58495=DIRECTION ( 'NONE',  ( -1.000000000000000000, 0.000000000000000000, 0.000000000000000000 ) ) ;
#58497=ORIENTED_EDGE ( 'NONE', *, *, #56106, .F. ) ;
#58498=CARTESIAN_POINT ( 'NONE',  ( -35.00000000000000000, 0.000000000000000000, 0.000000000000000000 ) ) ;
#58504=CARTESIAN_POINT ( 'NONE',  ( 35.00000000000000000, 11.32068061209303167, 5.865551165830956926 ) ) ;
#58505=DIRECTION ( 'NONE',  ( 0.000000000000000000, 0.01356324068817998940, -0.9999080150203990547 ) ) ;
#58507=DIRECTION ( 'NONE',  ( 1.000000000000000000, -0.000000000000000000, 0.000000000000000000 ) ) ;
#58508=CARTESIAN_POINT ( 'NONE',  ( -27.01437459610461644, -10.69338818478079922, -8.240233560378637634 ) ) ;
#58509=CIRCLE ( 'NONE', #29795, 5.000000000000000000 ) ;
#58510=AXIS2_PLACEMENT_3D ( 'NONE', #9310, #29596, #28965 ) ;
#58511=EDGE_LOOP ( 'NONE', ( #1898, #25594, #4812, #1568 ) ) ;
#58512=CARTESIAN_POINT ( 'NONE',  ( -35.00000000000000000, -2.936739658819952581, 11.37311665002362560 ) ) ;
#58515=ORIENTED_EDGE ( 'NONE', *, *, #12809, .T. ) ;
#58516=DIRECTION ( 'NONE',  ( -1.000000000000000000, 0.000000000000000000, 0.000000000000000000 ) ) ;
#58518=CARTESIAN_POINT ( 'NONE',  ( 11.34652066572562568, -13.36077880898726811, -1.937500768320442157 ) ) ;
#58521=ORIENTED_EDGE ( 'NONE', *, *, #23439, .T. ) ;
#58523=DIRECTION ( 'NONE',  ( -1.000000000000000000, 0.000000000000000000, 0.000000000000000000 ) ) ;
#58524=CIRCLE ( 'NONE', #9644, 5.000000000000000888 ) ;
#58532=AXIS2_PLACEMENT_3D ( 'NONE', #11803, #32086, #36082 ) ;
#58537=AXIS2_PLACEMENT_3D ( 'NONE', #27754, #2161, #44040 ) ;
#58540=CIRCLE ( 'NONE', #60612, 12.75000000000000178 ) ;
#58542=CARTESIAN_POINT ( 'NONE',  ( -9.843269086711673665, 12.00503757583305742, -6.187402193203074496 ) ) ;
#58543=ORIENTED_EDGE ( 'NONE', *, *, #46880, .T. ) ;
#58545=DIRECTION ( 'NONE',  ( 0.000000000000000000, 0.9467777615094582488, 0.3218879778915939571 ) ) ;
#58546=AXIS2_PLACEMENT_3D ( 'NONE', #14067, #53003, #27721 ) ;
#58547=CARTESIAN_POINT ( 'NONE',  ( 47.00000000000000711, 4.705694406421931860E-17, -3.469127814946512892E-15 ) ) ;
#58548=CARTESIAN_POINT ( 'NONE',  ( 35.00000000000000000, 11.38112321385050585, -2.905556151562669331 ) ) ;
#58549=LINE ( 'NONE', #33255, #47769 ) ;
#58550=ORIENTED_EDGE ( 'NONE', *, *, #19716, .T. ) ;
#58552=VERTEX_POINT ( 'NONE', #50172 ) ;
#58555=AXIS2_PLACEMENT_3D ( 'NONE', #46006, #464, #20730 ) ;
#58556=CYLINDRICAL_SURFACE ( 'NONE', #29977, 10.70557198542813815 ) ;
#58557=EDGE_CURVE ( 'NONE', #3064, #11516, #46705, .T. ) ;
#58558=ORIENTED_EDGE ( 'NONE', *, *, #61031, .F. ) ;
#58562=ORIENTED_EDGE ( 'NONE', *, *, #63059, .T. ) ;
#58563=FACE_OUTER_BOUND ( 'NONE', #7952, .T. ) ;
#58564=EDGE_CURVE ( 'NONE', #58552, #56112, #56231, .T. ) ;
#58567=VERTEX_POINT ( 'NONE', #23595 ) ;
#58568=EDGE_LOOP ( 'NONE', ( #15404, #62595, #38948, #21966 ) ) ;
#58569=CARTESIAN_POINT ( 'NONE',  ( 10.75853767213705225, 7.830989516993144051, 9.092612561015865680 ) ) ;
#58570=EDGE_CURVE ( 'NONE', #26022, #26770, #37102, .T. ) ;
#58571=VERTEX_POINT ( 'NONE', #33877 ) ;
#58572=CARTESIAN_POINT ( 'NONE',  ( -19.12691312516887265, 11.92229376959483211, -1.407263896924768387 ) ) ;
#58577=DIRECTION ( 'NONE',  ( 1.000000000000000000, 0.000000000000000000, -0.000000000000000000 ) ) ;
#58578=DIRECTION ( 'NONE',  ( 0.000000000000000000, 0.1387779952735818667, -0.9903235168508549569 ) ) ;
#58580=EDGE_CURVE ( 'NONE', #55881, #9403, #4222, .T. ) ;
#58581=DIRECTION ( 'NONE',  ( 0.000000000000000000, -0.01356324068817991828, 0.9999080150203990547 ) ) ;
#58582=CARTESIAN_POINT ( 'NONE',  ( -27.73981011261383856, -10.56186010129852093, -5.703782696336726410 ) ) ;
#58583=ORIENTED_EDGE ( 'NONE', *, *, #51164, .T. ) ;
#58585=CIRCLE ( 'NONE', #24566, 5.000000000000000000 ) ;
#58586=VERTEX_POINT ( 'NONE', #8948 ) ;
#58590=CIRCLE ( 'NONE', #25665, 12.18650000000000055 ) ;
#58592=ORIENTED_EDGE ( 'NONE', *, *, #6546, .F. ) ;
#58593=FACE_OUTER_BOUND ( 'NONE', #14660, .T. ) ;
#58596=VERTEX_POINT ( 'NONE', #33566 ) ;
#58598=AXIS2_PLACEMENT_3D ( 'NONE', #48044, #22778, #43034 ) ;
#58601=DIRECTION ( 'NONE',  ( 0.000000000000000000, -0.5987040770935561085, 0.8009703041134255130 ) ) ;
#58602=EDGE_CURVE ( 'NONE', #55347, #62855, #34945, .T. ) ;
#58603=EDGE_LOOP ( 'NONE', ( #27210, #23656, #25166, #23590 ) ) ;
#58604=CARTESIAN_POINT ( 'NONE',  ( -26.25036423639542349, -12.35650188709325015, 5.438569221978448276 ) ) ;
#58608=ORIENTED_EDGE ( 'NONE', *, *, #49724, .T. ) ;
#58609=DIRECTION ( 'NONE',  ( 0.000000000000000000, -0.1387779952735677669, 0.9903235168508569553 ) ) ;
#58610=VECTOR ( 'NONE', #45061, 1000.000000000000000 ) ;
#58611=AXIS2_PLACEMENT_3D ( 'NONE', #43451, #8223, #48801 ) ;
#58612=AXIS2_PLACEMENT_3D ( 'NONE', #10815, #26122, #32066 ) ;
#58614=B_SPLINE_CURVE_WITH_KNOTS ( 'NONE', 3,
 ( #17284, #37564, #57864, #60128, #40152, #54823, #54502, #34194, #29853, #3658, #50164, #60446, #23922, #44180, #65422, #54166, #39842, #59167, #3311, #14550 ),
 .UNSPECIFIED., .F., .F.,
 ( 4, 2, 2, 2, 2, 2, 2, 2, 2, 4 ),
 ( 0.000000000000000000, 0.0008692636490269044875, 0.001738527298053808975, 0.002173159122567255852, 0.002607790947080702512, 0.003477054596107587159, 0.004346318245134472673, 0.005215581894161356452, 0.006084845543188241099, 0.006954109192215124878 ),
 .UNSPECIFIED. ) ;
#58615=VECTOR ( 'NONE', #47025, 1000.000000000000000 ) ;
#58616=CARTESIAN_POINT ( 'NONE',  ( -28.56473390530001311, 3.589939350442137300, 11.45074047018220753 ) ) ;
#58618=PLANE ( 'NONE',  #59642 ) ;
#58619=CARTESIAN_POINT ( 'NONE',  ( 3.849043803728001922, -10.99600197132397206, -4.807418468138718204 ) ) ;
#58620=CARTESIAN_POINT ( 'NONE',  ( -37.00000000000000711, 11.53507381115580444, 2.216820770815288721 ) ) ;
#58621=CIRCLE ( 'NONE', #221, 12.75000000000000178 ) ;
#58622=EDGE_CURVE ( 'NONE', #2448, #42463, #44549, .T. ) ;
#58626=ORIENTED_EDGE ( 'NONE', *, *, #62097, .F. ) ;
#58627=CYLINDRICAL_SURFACE ( 'NONE', #50146, 5.000000000000000888 ) ;
#58630=ORIENTED_EDGE ( 'NONE', *, *, #61312, .T. ) ;
#58634=ORIENTED_EDGE ( 'NONE', *, *, #40071, .T. ) ;
#58635=ORIENTED_EDGE ( 'NONE', *, *, #25393, .F. ) ;
#58636=CARTESIAN_POINT ( 'NONE',  ( -10.89043372599972059, -7.929194153844475679, -9.011149282957994444 ) ) ;
#58639=VECTOR ( 'NONE', #24398, 1000.000000000000000 ) ;
#58644=DIRECTION ( 'NONE',  ( -1.000000000000000000, 0.000000000000000000, 0.000000000000000000 ) ) ;
#58650=CARTESIAN_POINT ( 'NONE',  ( -29.68541646480313645, -1.416020129149148543, -11.91616074890925780 ) ) ;
#58651=CARTESIAN_POINT ( 'NONE',  ( -25.15730131298249006, 10.22820549693168246, 6.278442145667771257 ) ) ;
#58652=ORIENTED_EDGE ( 'NONE', *, *, #33838, .F. ) ;
#58656=CARTESIAN_POINT ( 'NONE',  ( -19.74705739643458102, 13.27343858888937334, -2.482339776708336387 ) ) ;
#58657=ORIENTED_EDGE ( 'NONE', *, *, #36555, .F. ) ;
#58658=DIRECTION ( 'NONE',  ( 0.000000000000000000, -0.9346839223284580944, 0.3554799084908867868 ) ) ;
#58659=CARTESIAN_POINT ( 'NONE',  ( -37.00000000000000711, -1.591260454995328866, 12.08216339958900321 ) ) ;
#58661=DIRECTION ( 'NONE',  ( -1.000000000000000000, 0.000000000000000000, 0.000000000000000000 ) ) ;
#58662=AXIS2_PLACEMENT_3D ( 'NONE', #54624, #9042, #40606 ) ;
#58666=CIRCLE ( 'NONE', #14977, 12.18650000000000055 ) ;
#58672=EDGE_CURVE ( 'NONE', #59719, #55105, #54106, .T. ) ;
#58675=CARTESIAN_POINT ( 'NONE',  ( -18.36675263200364228, -11.99999999999999289, 0.3149281170547481579 ) ) ;
#58676=CYLINDRICAL_SURFACE ( 'NONE', #59936, 4.999999999999999112 ) ;
#58679=DIRECTION ( 'NONE',  ( 0.000000000000000000, -1.000000000000000000, 0.000000000000000000 ) ) ;
#58682=EDGE_CURVE ( 'NONE', #44984, #2788, #47753, .T. ) ;
#58683=VECTOR ( 'NONE', #56439, 1000.000000000000000 ) ;
#58685=ORIENTED_EDGE ( 'NONE', *, *, #387, .T. ) ;
#58687=ADVANCED_FACE ( 'NONE', ( #10238 ), #5266, .T. ) ;
#58689=AXIS2_PLACEMENT_3D ( 'NONE', #22973, #47575, #2024 ) ;
#58690=VECTOR ( 'NONE', #39715, 1000.000000000000000 ) ;
#58691=CARTESIAN_POINT ( 'NONE',  ( -18.04458733766117362, -11.34280559204704097, 3.916728392552376370 ) ) ;
#58693=AXIS2_PLACEMENT_3D ( 'NONE', #18616, #38870, #43855 ) ;
#58694=DIRECTION ( 'NONE',  ( -1.000000000000000000, 0.000000000000000000, 0.000000000000000000 ) ) ;
#58696=ORIENTED_EDGE ( 'NONE', *, *, #54836, .F. ) ;
#58697=CARTESIAN_POINT ( 'NONE',  ( -37.00000000000000711, -10.14408668126209001, -5.921969905510467314 ) ) ;
#58699=DIRECTION ( 'NONE',  ( -1.000000000000000000, 0.000000000000000000, 0.000000000000000000 ) ) ;
#58700=AXIS2_PLACEMENT_3D ( 'NONE', #20833, #35464, #40448 ) ;
#58701=CIRCLE ( 'NONE', #2446, 12.18650000000000055 ) ;
#58703=CYLINDRICAL_SURFACE ( 'NONE', #15031, 12.00000000000000000 ) ;
#58705=AXIS2_PLACEMENT_3D ( 'NONE', #65156, #19630, #39889 ) ;
#58706=EDGE_LOOP ( 'NONE', ( #33602, #43563, #26979, #46027 ) ) ;
#58707=DIRECTION ( 'NONE',  ( -1.000000000000000000, 0.000000000000000000, 0.000000000000000000 ) ) ;
#58709=CIRCLE ( 'NONE', #32082, 12.74999999999999822 ) ;
#58710=DIRECTION ( 'NONE',  ( 0.000000000000000000, -0.01356324068817991828, 0.9999080150203990547 ) ) ;
#58711=VERTEX_POINT ( 'NONE', #56457 ) ;
#58712=DIRECTION ( 'NONE',  ( -1.000000000000000000, 0.000000000000000000, 0.000000000000000000 ) ) ;
#58715=EDGE_CURVE ( 'NONE', #13694, #3037, #57292, .T. ) ;
#58717=FACE_OUTER_BOUND ( 'NONE', #14121, .T. ) ;
#58718=ADVANCED_FACE ( 'NONE', ( #10902 ), #40842, .T. ) ;
#58723=CARTESIAN_POINT ( 'NONE',  ( -47.00000000000000711, 0.000000000000000000, 0.000000000000000000 ) ) ;
#58724=DIRECTION ( 'NONE',  ( -1.000000000000000000, 0.000000000000000000, 0.000000000000000000 ) ) ;
#58725=CARTESIAN_POINT ( 'NONE',  ( -27.71501699605894231, 10.41584495806773880, -5.966219686924770116 ) ) ;
#58726=CARTESIAN_POINT ( 'NONE',  ( 37.00000000000000711, 4.705694406421931860E-17, -3.469127814946512892E-15 ) ) ;
#58728=ORIENTED_EDGE ( 'NONE', *, *, #3034, .F. ) ;
#58729=CARTESIAN_POINT ( 'NONE',  ( 35.00000000000000000, 9.512294188640899151, -6.891188680298859559 ) ) ;
#58731=ORIENTED_EDGE ( 'NONE', *, *, #50598, .F. ) ;
#58733=DIRECTION ( 'NONE',  ( 0.000000000000000000, -0.5987040770935737610, 0.8009703041134123014 ) ) ;
#58734=ORIENTED_EDGE ( 'NONE', *, *, #11541, .T. ) ;
#58735=ORIENTED_EDGE ( 'NONE', *, *, #46809, .F. ) ;
#58736=CARTESIAN_POINT ( 'NONE',  ( -25.50214104994386233, 8.498208897971778697, 10.49406410904484765 ) ) ;
#58738=AXIS2_PLACEMENT_3D ( 'NONE', #56461, #26520, #46805 ) ;
#58739=CARTESIAN_POINT ( 'NONE',  ( 47.00000000000000711, 4.705694406421931860E-17, -3.469127814946512892E-15 ) ) ;
#58740=VECTOR ( 'NONE', #17393, 1000.000000000000000 ) ;
#58741=LINE ( 'NONE', #13161, #16890 ) ;
#58742=DIRECTION ( 'NONE',  ( 0.000000000000000000, 0.9346839223284527653, -0.3554799084909000539 ) ) ;
#58744=EDGE_LOOP ( 'NONE', ( #20395, #24751, #26819, #56004 ) ) ;
#58747=DIRECTION ( 'NONE',  ( 0.000000000000000000, -0.01356324068817999114, 0.9999080150203989437 ) ) ;
#58748=ORIENTED_EDGE ( 'NONE', *, *, #24185, .F. ) ;
#58750=ORIENTED_EDGE ( 'NONE', *, *, #58934, .T. ) ;
#58751=AXIS2_PLACEMENT_3D ( 'NONE', #20308, #15325, #50590 ) ;
#58752=DIRECTION ( 'NONE',  ( -0.000000000000000000, -0.000000000000000000, -1.000000000000000000 ) ) ;
#58754=EDGE_CURVE ( 'NONE', #50843, #19597, #15872, .T. ) ;
#58755=DIRECTION ( 'NONE',  ( 1.000000000000000000, 0.000000000000000000, -0.000000000000000000 ) ) ;
#58758=DIRECTION ( 'NONE',  ( 0.000000000000000000, 0.9246979985058736418, 0.3807014730195186214 ) ) ;
#58759=EDGE_CURVE ( 'NONE', #38324, #52526, #45483, .T. ) ;
#58760=CARTESIAN_POINT ( 'NONE',  ( -9.197602943758386829, 12.97439165539572592, -3.730917860933687269 ) ) ;
#58762=CARTESIAN_POINT ( 'NONE',  ( -19.69476066079020171, -4.201994156881551312, 25.00000000000000000 ) ) ;
#58763=ORIENTED_EDGE ( 'NONE', *, *, #24522, .F. ) ;
#58766=DIRECTION ( 'NONE',  ( -1.000000000000000000, -0.000000000000000000, 0.000000000000000000 ) ) ;
#58770=AXIS2_PLACEMENT_3D ( 'NONE', #3886, #44743, #49120 ) ;
#58772=ORIENTED_EDGE ( 'NONE', *, *, #14940, .F. ) ;
#58774=CARTESIAN_POINT ( 'NONE',  ( 8.909527563550417639, 6.491711137615684635, 10.09430667957289174 ) ) ;
#58776=FACE_OUTER_BOUND ( 'NONE', #1616, .T. ) ;
#58777=VERTEX_POINT ( 'NONE', #7542 ) ;
#58779=DIRECTION ( 'NONE',  ( 0.000000000000000000, 0.8696919319575167062, 0.4935949184179292404 ) ) ;
#58780=DIRECTION ( 'NONE',  ( -1.000000000000000000, 0.000000000000000000, 0.000000000000000000 ) ) ;
#58781=AXIS2_PLACEMENT_3D ( 'NONE', #23069, #49008, #44309 ) ;
#58784=AXIS2_PLACEMENT_3D ( 'NONE', #44037, #38044, #54014 ) ;
#58785=EDGE_CURVE ( 'NONE', #25246, #45531, #22525, .T. ) ;
#58787=EDGE_CURVE ( 'NONE', #21888, #44528, #33928, .T. ) ;
#58788=DIRECTION ( 'NONE',  ( -1.000000000000000000, 0.000000000000000000, -0.000000000000000000 ) ) ;
#58789=ORIENTED_EDGE ( 'NONE', *, *, #25184, .F. ) ;
#58791=DIRECTION ( 'NONE',  ( -0.000000000000000000, -1.000000000000000000, -0.000000000000000000 ) ) ;
#58792=AXIS2_PLACEMENT_3D ( 'NONE', #41889, #15312, #41221 ) ;
#58794=ORIENTED_EDGE ( 'NONE', *, *, #6617, .T. ) ;
#58795=CARTESIAN_POINT ( 'NONE',  ( -17.71459495912815996, 3.737299794473689651, -12.97394593183730116 ) ) ;
#58797=DIRECTION ( 'NONE',  ( -1.000000000000000000, -0.000000000000000000, 0.000000000000000000 ) ) ;
#58798=CIRCLE ( 'NONE', #35400, 4.999999999999999112 ) ;
#58800=DIRECTION ( 'NONE',  ( 0.000000000000000000, -0.01356324068817999114, 0.9999080150203989437 ) ) ;
#58802=ORIENTED_EDGE ( 'NONE', *, *, #36752, .T. ) ;
#58804=ORIENTED_EDGE ( 'NONE', *, *, #34120, .F. ) ;
#58806=CARTESIAN_POINT ( 'NONE',  ( 36.00000000000000711, 12.21925492305367200, 3.640372113593418835 ) ) ;
#58809=DIRECTION ( 'NONE',  ( 1.000000000000000000, 0.000000000000000000, 0.000000000000000000 ) ) ;
#58810=CARTESIAN_POINT ( 'NONE',  ( -35.00000000000000000, -11.73555825188280011, 4.983891302653540301 ) ) ;
#58815=ADVANCED_FACE ( 'NONE', ( #28169 ), #27834, .T. ) ;
#58817=ORIENTED_EDGE ( 'NONE', *, *, #30449, .T. ) ;
#58818=CARTESIAN_POINT ( 'NONE',  ( 35.00000000000000000, 8.146229107149526527, 9.063649021438864750 ) ) ;
#58819=ORIENTED_EDGE ( 'NONE', *, *, #29435, .T. ) ;
#58820=EDGE_CURVE ( 'NONE', #62620, #33705, #52134, .T. ) ;
#58823=AXIS2_PLACEMENT_3D ( 'NONE', #19937, #25249, #5309 ) ;
#58824=CARTESIAN_POINT ( 'NONE',  ( 35.00000000000000000, -3.093009498343839869, 11.78745411414842437 ) ) ;
#58825=VERTEX_POINT ( 'NONE', #37808 ) ;
#58826=DIRECTION ( 'NONE',  ( -1.000000000000000000, 0.000000000000000000, 0.000000000000000000 ) ) ;
#58829=ORIENTED_EDGE ( 'NONE', *, *, #41723, .F. ) ;
#58830=ORIENTED_EDGE ( 'NONE', *, *, #39399, .F. ) ;
#58833=AXIS2_PLACEMENT_3D ( 'NONE', #28723, #40249, #60216 ) ;
#58836=ORIENTED_EDGE ( 'NONE', *, *, #51801, .T. ) ;
#58837=DIRECTION ( 'NONE',  ( 1.000000000000000000, 0.000000000000000000, -0.000000000000000000 ) ) ;
#58840=AXIS2_PLACEMENT_3D ( 'NONE', #24320, #34929, #34616 ) ;
#58843=DIRECTION ( 'NONE',  ( 0.000000000000000000, 0.7617968321374855023, 0.6478160128811972784 ) ) ;
#58847=AXIS2_PLACEMENT_3D ( 'NONE', #51740, #46731, #1192 ) ;
#58849=AXIS2_PLACEMENT_3D ( 'NONE', #20868, #16551, #46468 ) ;
#58850=CARTESIAN_POINT ( 'NONE',  ( -17.15625955527509916, 7.251550614233345016, 9.562613488379174242 ) ) ;
#58857=CARTESIAN_POINT ( 'NONE',  ( -28.56462394502010937, 3.589878760083829334, -13.01421318288084095 ) ) ;
#58860=VERTEX_POINT ( 'NONE', #27179 ) ;
#58862=ORIENTED_EDGE ( 'NONE', *, *, #22220, .F. ) ;
#58865=CIRCLE ( 'NONE', #25893, 1.750000000000000000 ) ;
#58866=CARTESIAN_POINT ( 'NONE',  ( 12.19141456596091011, -11.13119688865502255, -7.646933030662562025 ) ) ;
#58867=CARTESIAN_POINT ( 'NONE',  ( -37.00000000000000711, -1.113475361586400814, -12.70128625845194215 ) ) ;
#58868=DIRECTION ( 'NONE',  ( 0.000000000000000000, -0.8169148498130339719, 0.5767582926624881257 ) ) ;
#58869=ORIENTED_EDGE ( 'NONE', *, *, #19856, .F. ) ;
#58871=DIRECTION ( 'NONE',  ( 1.000000000000000000, 0.000000000000000000, 0.000000000000000000 ) ) ;
#58872=CARTESIAN_POINT ( 'NONE',  ( -37.00000000000000711, 0.000000000000000000, 0.000000000000000000 ) ) ;
#58873=CARTESIAN_POINT ( 'NONE',  ( -35.00000000000000000, -11.59095880812009582, 1.903127969211145132 ) ) ;
#58874=EDGE_CURVE ( 'NONE', #26482, #8029, #14780, .T. ) ;
#58875=CARTESIAN_POINT ( 'NONE',  ( 35.00000000000000000, 7.608228585767871976, 10.23119532541064203 ) ) ;
#58880=CARTESIAN_POINT ( 'NONE',  ( 37.00000000000000711, 0.000000000000000000, 0.000000000000000000 ) ) ;
#58881=VECTOR ( 'NONE', #6990, 1000.000000000000000 ) ;
#58882=AXIS2_PLACEMENT_3D ( 'NONE', #61245, #2962, #11041 ) ;
#58884=ORIENTED_EDGE ( 'NONE', *, *, #36334, .T. ) ;
#58885=VERTEX_POINT ( 'NONE', #8859 ) ;
#58886=CARTESIAN_POINT ( 'NONE',  ( -7.489022030332961322, 8.034049540753141372, -10.84914964302385521 ) ) ;
#58888=DIRECTION ( 'NONE',  ( 1.000000000000000000, 0.000000000000000000, 0.000000000000000000 ) ) ;
#58890=CARTESIAN_POINT ( 'NONE',  ( -36.00000000000000711, -9.076753354954062658, 8.954052073409570767 ) ) ;
#58891=DIRECTION ( 'NONE',  ( 0.000000000000000000, -0.9796553971857763221, -0.2006870767258792099 ) ) ;
#58893=VERTEX_POINT ( 'NONE', #49452 ) ;
#58894=EDGE_CURVE ( 'NONE', #10423, #15438, #24385, .T. ) ;
#58895=CIRCLE ( 'NONE', #7896, 5.000000000000000888 ) ;
#58896=VERTEX_POINT ( 'NONE', #24466 ) ;
#58897=ORIENTED_EDGE ( 'NONE', *, *, #61080, .F. ) ;
#58899=EDGE_CURVE ( 'NONE', #2111, #6900, #22254, .T. ) ;
#58900=VECTOR ( 'NONE', #36189, 1000.000000000000000 ) ;
#58901=DIRECTION ( 'NONE',  ( 0.000000000000000000, 0.6478160128811947249, -0.7617968321374878338 ) ) ;
#58902=EDGE_LOOP ( 'NONE', ( #47665, #43346, #36998, #46913 ) ) ;
#58903=FACE_OUTER_BOUND ( 'NONE', #5196, .T. ) ;
#58905=ORIENTED_EDGE ( 'NONE', *, *, #37883, .F. ) ;
#58907=CARTESIAN_POINT ( 'NONE',  ( -37.00000000000000711, 5.300372733891804522, -11.59605747147781152 ) ) ;
#58908=DIRECTION ( 'NONE',  ( -0.000000000000000000, -0.000000000000000000, -1.000000000000000000 ) ) ;
#58909=ORIENTED_EDGE ( 'NONE', *, *, #56323, .F. ) ;
#58911=DIRECTION ( 'NONE',  ( 0.000000000000000000, -0.6943713148249535116, 0.7196168960969895334 ) ) ;
#58912=ORIENTED_EDGE ( 'NONE', *, *, #34242, .F. ) ;
#58913=DIRECTION ( 'NONE',  ( 1.000000000000000000, 0.000000000000000000, 0.000000000000000000 ) ) ;
#58914=VERTEX_POINT ( 'NONE', #19499 ) ;
#58916=CYLINDRICAL_SURFACE ( 'NONE', #47883, 5.000000000000000888 ) ;
#58917=ADVANCED_FACE ( 'NONE', ( #2909 ), #59398, .T. ) ;
#58919=CIRCLE ( 'NONE', #16406, 5.000000000000001776 ) ;
#58925=EDGE_LOOP ( 'NONE', ( #14670, #19116, #43707, #44129 ) ) ;
#58929=VERTEX_POINT ( 'NONE', #19159 ) ;
#58930=CARTESIAN_POINT ( 'NONE',  ( 47.00000000000000711, 4.705694406421931860E-17, -3.469127814946512892E-15 ) ) ;
#58933=VERTEX_POINT ( 'NONE', #44746 ) ;
#58934=EDGE_CURVE ( 'NONE', #61089, #9977, #30740, .T. ) ;
#58935=ORIENTED_EDGE ( 'NONE', *, *, #23576, .F. ) ;
#58937=ORIENTED_EDGE ( 'NONE', *, *, #54120, .F. ) ;
#58938=CARTESIAN_POINT ( 'NONE',  ( -24.95335564517041149, -11.81240985965305512, 6.538156315917978745 ) ) ;
#58939=CARTESIAN_POINT ( 'NONE',  ( -4.045980568306387859, -9.337516854300243807, 7.540689691057082200 ) ) ;
#58941=CARTESIAN_POINT ( 'NONE',  ( 37.00000000000000711, 5.636262487437473823, 10.80478261802175233 ) ) ;
#58942=CARTESIAN_POINT ( 'NONE',  ( -35.00000000000000000, 11.60979404548639948, -3.704519465651187282 ) ) ;
#58943=AXIS2_PLACEMENT_3D ( 'NONE', #5674, #35573, #55867 ) ;
#58944=ORIENTED_EDGE ( 'NONE', *, *, #44600, .F. ) ;
#58945=CYLINDRICAL_SURFACE ( 'NONE', #14651, 4.999999999999999112 ) ;
#58946=CIRCLE ( 'NONE', #44020, 4.999999999999999112 ) ;
#58947=EDGE_CURVE ( 'NONE', #64141, #34055, #11623, .T. ) ;
#58951=ADVANCED_FACE ( 'NONE', ( #53771 ), #59733, .T. ) ;
#58954=CARTESIAN_POINT ( 'NONE',  ( -36.00000000000000711, -0.4871980014162358152, 12.74068829017553739 ) ) ;
#58955=ADVANCED_FACE ( 'NONE', ( #18193 ), #64057, .T. ) ;
#58958=ORIENTED_EDGE ( 'NONE', *, *, #62800, .F. ) ;
#58961=CARTESIAN_POINT ( 'NONE',  ( 8.937200413559443390, 4.476360154859203355, -12.73625532737111143 ) ) ;
#58963=CARTESIAN_POINT ( 'NONE',  ( 22.88594695219327235, 3.421158645304719137, -13.05931366970166962 ) ) ;
#58968=CARTESIAN_POINT ( 'NONE',  ( 29.73149305502989392, -9.424759817252279959, 9.675963828540520950 ) ) ;
#58970=ORIENTED_EDGE ( 'NONE', *, *, #4211, .T. ) ;
#58971=EDGE_CURVE ( 'NONE', #63621, #31648, #55146, .T. ) ;
#58972=DIRECTION ( 'NONE',  ( -1.000000000000000000, -0.000000000000000000, 0.000000000000000000 ) ) ;
#58974=CARTESIAN_POINT ( 'NONE',  ( -35.00000000000000000, 4.946702696913171771, 11.13736569743276306 ) ) ;
#58975=CARTESIAN_POINT ( 'NONE',  ( 17.38697840126492622, 10.06593862365382464, 6.600811317301616299 ) ) ;
#58976=VERTEX_POINT ( 'NONE', #14160 ) ;
#58977=CIRCLE ( 'NONE', #23936, 12.18649999999999700 ) ;
#58978=CYLINDRICAL_SURFACE ( 'NONE', #21391, 5.000000000000000888 ) ;
#58979=CARTESIAN_POINT ( 'NONE',  ( 35.00000000000000000, 4.705694406421931860E-17, -3.469127814946512892E-15 ) ) ;
#58980=DIRECTION ( 'NONE',  ( -1.000000000000000000, 0.000000000000000000, 0.000000000000000000 ) ) ;
#58983=CARTESIAN_POINT ( 'NONE',  ( -35.00000000000000000, 8.295159312811854591, 8.927548052240926069 ) ) ;
#58987=CARTESIAN_POINT ( 'NONE',  ( 37.00000000000000711, -7.094637218249427946, -10.59380114696467778 ) ) ;
#58989=AXIS2_PLACEMENT_3D ( 'NONE', #55611, #60921, #14674 ) ;
#58991=DIRECTION ( 'NONE',  ( -1.000000000000000000, -0.000000000000000000, 0.000000000000000000 ) ) ;
#58993=CARTESIAN_POINT ( 'NONE',  ( -10.39032328888078105, -5.036169502593281777, -12.53141698666758685 ) ) ;
#58996=DIRECTION ( 'NONE',  ( 0.000000000000000000, 0.01356324068817998940, -0.9999080150203989437 ) ) ;
#58997=ORIENTED_EDGE ( 'NONE', *, *, #44146, .F. ) ;
#58998=VERTEX_POINT ( 'NONE', #44106 ) ;
#58999=CARTESIAN_POINT ( 'NONE',  ( -35.00000000000000000, -6.303578524886872536, -10.42955799785326576 ) ) ;
#59000=CARTESIAN_POINT ( 'NONE',  ( -17.54726996257253191, -11.36053454945672136, 3.865003848717349033 ) ) ;
#59003=EDGE_CURVE ( 'NONE', #65768, #11428, #26474, .T. ) ;
#59004=CYLINDRICAL_SURFACE ( 'NONE', #10685, 5.000000000000000888 ) ;
#59005=AXIS2_PLACEMENT_3D ( 'NONE', #11071, #12033, #56629 ) ;
#59006=B_SPLINE_CURVE_WITH_KNOTS ( 'NONE', 3,
 ( #48654, #58975, #23717, #13068, #8740, #8089, #43641, #29022, #42990, #28356, #28042, #63266, #13386, #33671 ),
 .UNSPECIFIED., .F., .F.,
 ( 4, 2, 2, 2, 2, 2, 4 ),
 ( 1.701886623846052835E-17, 0.002810228430025432916, 0.004215342645038138748, 0.005620456860050845882, 0.007025571075063551281, 0.008430685290076256680, 0.01124091372010166921 ),
 .UNSPECIFIED. ) ;
#59009=CARTESIAN_POINT ( 'NONE',  ( 35.00000000000000000, -5.246972444133939817, 10.99909370905162298 ) ) ;
#59011=DIRECTION ( 'NONE',  ( 0.000000000000000000, -0.01356324068817998940, 0.9999080150203990547 ) ) ;
#59014=ADVANCED_FACE ( 'NONE', ( #58776 ), #28475, .T. ) ;
#59015=AXIS2_PLACEMENT_3D ( 'NONE', #50425, #60713, #9831 ) ;
#59016=CARTESIAN_POINT ( 'NONE',  ( -9.053705415859559125, -2.444157173645027381, 13.27951883727767246 ) ) ;
#59018=CARTESIAN_POINT ( 'NONE',  ( -9.443643884643755371, -3.548096057925545388, 13.02630244985499353 ) ) ;
#59023=DIRECTION ( 'NONE',  ( 1.000000000000000000, -0.000000000000000000, 0.000000000000000000 ) ) ;
#59024=EDGE_CURVE ( 'NONE', #56049, #51886, #57283, .T. ) ;
#59025=CARTESIAN_POINT ( 'NONE',  ( -36.00000000000000711, -10.84030624090602046, -6.711949091238257559 ) ) ;
#59026=CARTESIAN_POINT ( 'NONE',  ( -37.00000000000000711, 11.65150730582932503, 1.488153103997165605 ) ) ;
#59029=EDGE_CURVE ( 'NONE', #50088, #32109, #39405, .T. ) ;
#59030=CARTESIAN_POINT ( 'NONE',  ( -9.603270190229855174, -9.180294942608449915, -7.739257472663321202 ) ) ;
#59033=CARTESIAN_POINT ( 'NONE',  ( -10.48620311856347875, -9.720786832536937538, 9.367833439828908482 ) ) ;
#59037=CARTESIAN_POINT ( 'NONE',  ( -37.00000000000000711, -11.24036214326516436, -6.018036132182280618 ) ) ;
#59038=EDGE_CURVE ( 'NONE', #15001, #11288, #49872, .T. ) ;
#59039=AXIS2_PLACEMENT_3D ( 'NONE', #38793, #43778, #53446 ) ;
#59040=ORIENTED_EDGE ( 'NONE', *, *, #22270, .F. ) ;
#59042=CARTESIAN_POINT ( 'NONE',  ( -37.00000000000000711, 0.000000000000000000, 0.000000000000000000 ) ) ;
#59044=( BOUNDED_CURVE ( )  B_SPLINE_CURVE ( 3, ( #7720, #12680, #47956, #62562 ),
 .UNSPECIFIED., .F., .F. ) 
 B_SPLINE_CURVE_WITH_KNOTS ( ( 4, 4 ),
 ( 0.4415372860933093335, 0.5130637748270454601 ),
 .UNSPECIFIED. ) 
 CURVE ( )  GEOMETRIC_REPRESENTATION_ITEM ( )  RATIONAL_B_SPLINE_CURVE ( ( 1.000000000000000000, 0.9995737088895612077, 0.9995737088895612077, 1.000000000000000000 ) ) 
 REPRESENTATION_ITEM ( '' )  );
#59045=FACE_OUTER_BOUND ( 'NONE', #22487, .T. ) ;
#59046=DIRECTION ( 'NONE',  ( 1.000000000000000000, 0.000000000000000000, -0.000000000000000000 ) ) ;
#59047=EDGE_CURVE ( 'NONE', #30510, #23409, #51972, .T. ) ;
#59049=DIRECTION ( 'NONE',  ( 0.4826047536471247956, 0.8758382566188793739, -0.000000000000000000 ) ) ;
#59050=ORIENTED_EDGE ( 'NONE', *, *, #20872, .F. ) ;
#59052=ORIENTED_EDGE ( 'NONE', *, *, #23266, .F. ) ;
#59054=VERTEX_POINT ( 'NONE', #21372 ) ;
#59055=ORIENTED_EDGE ( 'NONE', *, *, #60548, .F. ) ;
#59056=CARTESIAN_POINT ( 'NONE',  ( -18.58686583997218378, 5.410928820688530649, 12.37136992127100932 ) ) ;
#59058=CARTESIAN_POINT ( 'NONE',  ( -24.38047113150638268, 9.758145127762370308, 9.337300561328881088 ) ) ;
#59059=CARTESIAN_POINT ( 'NONE',  ( -37.00000000000000711, 12.54989509947650994, 2.250029553613800637 ) ) ;
#59060=AXIS2_PLACEMENT_3D ( 'NONE', #46610, #1407, #37623 ) ;
#59062=DIRECTION ( 'NONE',  ( -1.000000000000000000, -0.000000000000000000, 0.000000000000000000 ) ) ;
#59066=CARTESIAN_POINT ( 'NONE',  ( 35.00000000000000000, -11.65150730582935523, -1.488153103996925797 ) ) ;
#59067=CARTESIAN_POINT ( 'NONE',  ( -35.00000000000000000, -12.15823808070322087, -0.8294751490780611913 ) ) ;
#59068=ORIENTED_EDGE ( 'NONE', *, *, #10484, .F. ) ;
#59069=DIRECTION ( 'NONE',  ( -1.000000000000000000, 0.000000000000000000, 0.000000000000000000 ) ) ;
#59070=VERTEX_POINT ( 'NONE', #35985 ) ;
#59073=CARTESIAN_POINT ( 'NONE',  ( 35.00000000000000000, 7.971186206369472060, -9.217970097227754067 ) ) ;
#59074=AXIS2_PLACEMENT_3D ( 'NONE', #16754, #37027, #58317 ) ;
#59076=EDGE_CURVE ( 'NONE', #36481, #34717, #20725, .T. ) ;
#59078=DIRECTION ( 'NONE',  ( 0.000000000000000000, -0.8169148498130338609, 0.5767582926624880146 ) ) ;
#59079=CARTESIAN_POINT ( 'NONE',  ( -7.489022030332961322, -8.034049540753116503, -10.84914964302385521 ) ) ;
#59083=CYLINDRICAL_SURFACE ( 'NONE', #24432, 5.000000000000000888 ) ;
#59086=CARTESIAN_POINT ( 'NONE',  ( -18.10791796330941850, -9.538085361946238905, -7.283445145555471179 ) ) ;
#59088=CARTESIAN_POINT ( 'NONE',  ( -37.00000000000000711, 12.74613886779085448, -0.3137578094507852411 ) ) ;
#59090=CARTESIAN_POINT ( 'NONE',  ( -47.00000000000000711, 0.000000000000000000, 0.000000000000000000 ) ) ;
#59093=CARTESIAN_POINT ( 'NONE',  ( -37.00000000000000711, 0.000000000000000000, 0.000000000000000000 ) ) ;
#59094=EDGE_CURVE ( 'NONE', #15359, #61567, #38233, .T. ) ;
#59095=ORIENTED_EDGE ( 'NONE', *, *, #6692, .T. ) ;
#59097=CARTESIAN_POINT ( 'NONE',  ( 19.09841239469957941, 7.043214802939539609, 11.53926296509304450 ) ) ;
#59098=CARTESIAN_POINT ( 'NONE',  ( 37.00000000000000711, 0.3025107581131208367, -11.74226168163341555 ) ) ;
#59099=LINE ( 'NONE', #15065, #29571 ) ;
#59102=CARTESIAN_POINT ( 'NONE',  ( -27.67949680227653175, -8.923181436745910133, -8.045965622785404392 ) ) ;
#59103=CIRCLE ( 'NONE', #44225, 5.000000000000000888 ) ;
#59104=ORIENTED_EDGE ( 'NONE', *, *, #42947, .F. ) ;
#59109=ORIENTED_EDGE ( 'NONE', *, *, #40335, .F. ) ;
#59111=DIRECTION ( 'NONE',  ( 0.000000000000000000, -0.01356324068817998940, 0.9999080150203990547 ) ) ;
#59112=LINE ( 'NONE', #23524, #56354 ) ;
#59115=CARTESIAN_POINT ( 'NONE',  ( -9.351388602708162523, -12.99278190472486827, -3.665735721005250358 ) ) ;
#59116=EDGE_CURVE ( 'NONE', #45883, #12635, #5444, .T. ) ;
#59120=DIRECTION ( 'NONE',  ( -1.000000000000000000, 0.000000000000000000, 0.000000000000000000 ) ) ;
#59121=LINE ( 'NONE', #44131, #31920 ) ;
#59126=EDGE_CURVE ( 'NONE', #16453, #33841, #5323, .T. ) ;
#59130=ORIENTED_EDGE ( 'NONE', *, *, #43211, .F. ) ;
#59135=CARTESIAN_POINT ( 'NONE',  ( -35.00000000000000000, -4.237174932027140350, -12.02534193257725548 ) ) ;
#59137=DIRECTION ( 'NONE',  ( -1.000000000000000000, 0.000000000000000000, -0.000000000000000000 ) ) ;
#59141=VERTEX_POINT ( 'NONE', #32967 ) ;
#59143=CARTESIAN_POINT ( 'NONE',  ( -35.00000000000000000, 10.64792938439755332, 5.927257550915355999 ) ) ;
#59144=EDGE_LOOP ( 'NONE', ( #7097, #46316, #39653, #23883, #24069, #63649, #13860, #60327, #64967, #32358, #52109, #9026 ) ) ;
#59145=VECTOR ( 'NONE', #31954, 1000.000000000000000 ) ;
#59151=DIRECTION ( 'NONE',  ( 0.000000000000000000, 0.4698238015817303159, 0.8827602140260348840 ) ) ;
#59152=FACE_OUTER_BOUND ( 'NONE', #18107, .T. ) ;
#59153=DIRECTION ( 'NONE',  ( -1.000000000000000000, -0.000000000000000000, -0.000000000000000000 ) ) ;
#59155=EDGE_LOOP ( 'NONE', ( #33313, #49538, #55921, #19096 ) ) ;
#59157=CARTESIAN_POINT ( 'NONE',  ( -37.00000000000000711, 9.821084925794570708, 7.215058775251291578 ) ) ;
#59159=CARTESIAN_POINT ( 'NONE',  ( 37.00000000000000711, -11.44858830469738109, 2.627174906297032209 ) ) ;
#59165=DIRECTION ( 'NONE',  ( -0.5244426074294280538, 0.000000000000000000, 0.8514458006899926490 ) ) ;
#59166=ORIENTED_EDGE ( 'NONE', *, *, #1748, .T. ) ;
#59167=CARTESIAN_POINT ( 'NONE',  ( -18.55539683905438864, 5.671985714705006565, -10.57868011600847602 ) ) ;
#59170=CARTESIAN_POINT ( 'NONE',  ( -35.00000000000000000, 0.000000000000000000, 0.000000000000000000 ) ) ;
#59171=DIRECTION ( 'NONE',  ( 1.000000000000000000, -0.000000000000000000, -0.000000000000000000 ) ) ;
#59172=DIRECTION ( 'NONE',  ( 0.000000000000000000, 0.01356324068817998940, -0.9999080150203990547 ) ) ;
#59174=EDGE_CURVE ( 'NONE', #25143, #10126, #44586, .T. ) ;
#59175=ORIENTED_EDGE ( 'NONE', *, *, #48045, .T. ) ;
#59176=CARTESIAN_POINT ( 'NONE',  ( -37.00000000000000711, 3.033604067594749765, -12.38385022362078836 ) ) ;
#59177=DIRECTION ( 'NONE',  ( -1.000000000000000000, -1.836970198721029688E-16, 0.000000000000000000 ) ) ;
#59178=FACE_OUTER_BOUND ( 'NONE', #38559, .T. ) ;
#59180=ADVANCED_FACE ( 'NONE', ( #4046 ), #25297, .T. ) ;
#59183=DIRECTION ( 'NONE',  ( 1.000000000000000000, -0.000000000000000000, 0.000000000000000000 ) ) ;
#59187=CIRCLE ( 'NONE', #7139, 12.74999999999999822 ) ;
#59188=CARTESIAN_POINT ( 'NONE',  ( 36.00000000000000711, 3.307597835713413481, 12.31350058095519273 ) ) ;
#59190=ORIENTED_EDGE ( 'NONE', *, *, #47562, .F. ) ;
#59191=VERTEX_POINT ( 'NONE', #49299 ) ;
#59192=CARTESIAN_POINT ( 'NONE',  ( 35.00000000000000000, -8.551552972817137999, -8.052525312709853722 ) ) ;
#59193=EDGE_CURVE ( 'NONE', #26426, #55701, #19424, .T. ) ;
#59198=ADVANCED_FACE ( 'NONE', ( #46905 ), #62190, .T. ) ;
#59200=ORIENTED_EDGE ( 'NONE', *, *, #44290, .T. ) ;
#59204=CARTESIAN_POINT ( 'NONE',  ( -35.00000000000000000, 0.000000000000000000, 0.000000000000000000 ) ) ;
#59212=LINE ( 'NONE', #48275, #31376 ) ;
#59213=ORIENTED_EDGE ( 'NONE', *, *, #32021, .T. ) ;
#59214=ORIENTED_EDGE ( 'NONE', *, *, #15811, .F. ) ;
#59216=ORIENTED_EDGE ( 'NONE', *, *, #17851, .T. ) ;
#59217=CARTESIAN_POINT ( 'NONE',  ( 8.437200413559441614, 4.476360154859202467, -12.73625532737110966 ) ) ;
#59218=ORIENTED_EDGE ( 'NONE', *, *, #35408, .F. ) ;
#59219=ORIENTED_EDGE ( 'NONE', *, *, #19577, .F. ) ;
#59225=DIRECTION ( 'NONE',  ( -1.000000000000000000, 0.000000000000000000, 0.000000000000000000 ) ) ;
#59226=ORIENTED_EDGE ( 'NONE', *, *, #57349, .F. ) ;
#59227=DIRECTION ( 'NONE',  ( 1.000000000000000000, 0.000000000000000000, 0.000000000000000000 ) ) ;
#59228=ADVANCED_FACE ( 'NONE', ( #25975 ), #41236, .T. ) ;
#59229=ORIENTED_EDGE ( 'NONE', *, *, #64253, .F. ) ;
#59230=CARTESIAN_POINT ( 'NONE',  ( 35.00000000000000000, 4.705694406421931860E-17, -3.469127814946512892E-15 ) ) ;
#59232=ORIENTED_EDGE ( 'NONE', *, *, #60369, .F. ) ;
#59233=CARTESIAN_POINT ( 'NONE',  ( -15.66545752291940019, 8.441064718611558604, 8.529329405872159597 ) ) ;
#59234=DIRECTION ( 'NONE',  ( 0.000000000000000000, 0.000000000000000000, 1.000000000000000000 ) ) ;
#59235=LINE ( 'NONE', #7707, #40802 ) ;
#59239=VERTEX_POINT ( 'NONE', #1362 ) ;
#59240=VECTOR ( 'NONE', #25336, 1000.000000000000000 ) ;
#59242=( BOUNDED_CURVE ( )  B_SPLINE_CURVE ( 3, ( #352, #50571, #15616, #20631 ),
 .UNSPECIFIED., .F., .F. ) 
 B_SPLINE_CURVE_WITH_KNOTS ( ( 4, 4 ),
 ( 1.759007296960887645, 1.789005565290672672 ),
 .UNSPECIFIED. ) 
 CURVE ( )  GEOMETRIC_REPRESENTATION_ITEM ( )  RATIONAL_B_SPLINE_CURVE ( ( 1.000000000000000000, 0.9999250100640160177, 0.9999250100640160177, 1.000000000000000000 ) ) 
 REPRESENTATION_ITEM ( '' )  );
#59245=CARTESIAN_POINT ( 'NONE',  ( -3.979081881654057629, -10.13347235061305796, 6.442799153484752850 ) ) ;
#59247=DIRECTION ( 'NONE',  ( -1.000000000000000000, -0.000000000000000000, 0.000000000000000000 ) ) ;
#59250=ORIENTED_EDGE ( 'NONE', *, *, #59862, .T. ) ;
#59252=CARTESIAN_POINT ( 'NONE',  ( 37.00000000000000711, -4.725891942574827809, -10.75351884295726101 ) ) ;
#59253=EDGE_CURVE ( 'NONE', #15087, #27683, #40326, .T. ) ;
#59254=CARTESIAN_POINT ( 'NONE',  ( -35.00000000000000000, 11.74226168163341555, 0.3025107581131598611 ) ) ;
#59255=CARTESIAN_POINT ( 'NONE',  ( -18.12051508114042164, -4.789732380985432414, 11.00348193257416973 ) ) ;
#59258=CYLINDRICAL_SURFACE ( 'NONE', #2827, 5.000000000000000888 ) ;
#59259=DIRECTION ( 'NONE',  ( 0.000000000000000000, 0.01356324068817998940, -0.9999080150203990547 ) ) ;
#59260=EDGE_CURVE ( 'NONE', #19597, #33743, #61521, .T. ) ;
#59263=CARTESIAN_POINT ( 'NONE',  ( 12.42313808479329218, -9.574587216605449314, -7.236090607063219160 ) ) ;
#59266=ORIENTED_EDGE ( 'NONE', *, *, #36005, .T. ) ;
#59270=CARTESIAN_POINT ( 'NONE',  ( -35.00000000000000000, 5.300372733891805410, -11.59605747147781152 ) ) ;
#59272=ORIENTED_EDGE ( 'NONE', *, *, #1389, .F. ) ;
#59276=ORIENTED_EDGE ( 'NONE', *, *, #12744, .F. ) ;
#59280=CARTESIAN_POINT ( 'NONE',  ( -15.27729454824424948, 5.151216734910788908, 25.00000000000000000 ) ) ;
#59281=ORIENTED_EDGE ( 'NONE', *, *, #27319, .F. ) ;
#59282=CARTESIAN_POINT ( 'NONE',  ( 35.00000000000000000, -6.753013023069642351, 10.14433819232440825 ) ) ;
#59286=ORIENTED_EDGE ( 'NONE', *, *, #65327, .F. ) ;
#59288=ORIENTED_EDGE ( 'NONE', *, *, #65767, .F. ) ;
#59289=CARTESIAN_POINT ( 'NONE',  ( 35.00000000000000000, -10.59380114696464581, 7.094637218249467026 ) ) ;
#59293=DIRECTION ( 'NONE',  ( 0.000000000000000000, 0.01356324068817998940, -0.9999080150203990547 ) ) ;
#59296=CARTESIAN_POINT ( 'NONE',  ( -10.22413763068411541, -4.688135402597775503, -12.66488886014959725 ) ) ;
#59297=CARTESIAN_POINT ( 'NONE',  ( 37.00000000000000711, -3.645068577059948911, 11.16627499335658413 ) ) ;
#59298=EDGE_CURVE ( 'NONE', #43145, #26931, #36596, .T. ) ;
#59299=EDGE_LOOP ( 'NONE', ( #39074, #30075, #36345, #4026 ) ) ;
#59301=DIRECTION ( 'NONE',  ( 0.000000000000000000, -0.01356324068817998940, 0.9999080150203990547 ) ) ;
#59304=ORIENTED_EDGE ( 'NONE', *, *, #1109, .F. ) ;
#59306=DIRECTION ( 'NONE',  ( 0.000000000000000000, -0.9987865678893272925, 0.04924826701375684818 ) ) ;
#59309=CIRCLE ( 'NONE', #17863, 12.75000000000000178 ) ;
#59310=CARTESIAN_POINT ( 'NONE',  ( -37.00000000000000711, 1.171570255487447643, 11.68758509253248867 ) ) ;
#59311=EDGE_CURVE ( 'NONE', #8578, #8085, #21257, .T. ) ;
#59314=AXIS2_PLACEMENT_3D ( 'NONE', #59358, #54388, #53400 ) ;
#59315=ORIENTED_EDGE ( 'NONE', *, *, #17715, .T. ) ;
#59316=CARTESIAN_POINT ( 'NONE',  ( 35.00000000000000000, 11.65150730582934635, 1.488153103997001514 ) ) ;
#59317=DIRECTION ( 'NONE',  ( 0.000000000000000000, -0.7617968321374946061, -0.6478160128811869534 ) ) ;
#59318=AXIS2_PLACEMENT_3D ( 'NONE', #14619, #40907, #44904 ) ;
#59320=EDGE_CURVE ( 'NONE', #57170, #63179, #39284, .T. ) ;
#59322=AXIS2_PLACEMENT_3D ( 'NONE', #25517, #45809, #271 ) ;
#59323=CARTESIAN_POINT ( 'NONE',  ( -8.519593703685796271, -2.053853521695917728, 13.34350279803584449 ) ) ;
#59324=LINE ( 'NONE', #63311, #34178 ) ;
#59325=ORIENTED_EDGE ( 'NONE', *, *, #11134, .T. ) ;
#59328=CARTESIAN_POINT ( 'NONE',  ( 2.506442445385721474, 1.822928711644228761, 11.86634058133937053 ) ) ;
#59330=CYLINDRICAL_SURFACE ( 'NONE', #63925, 12.75000000000000178 ) ;
#59332=ORIENTED_EDGE ( 'NONE', *, *, #49272, .F. ) ;
#59333=AXIS2_PLACEMENT_3D ( 'NONE', #2817, #49019, #34352 ) ;
#59337=CARTESIAN_POINT ( 'NONE',  ( -18.48144388550085182, 4.313438978693093340, -11.19870530402159226 ) ) ;
#59338=ORIENTED_EDGE ( 'NONE', *, *, #3399, .T. ) ;
#59341=ORIENTED_EDGE ( 'NONE', *, *, #24377, .T. ) ;
#59342=VERTEX_POINT ( 'NONE', #58875 ) ;
#59344=AXIS2_PLACEMENT_3D ( 'NONE', #65461, #7748, #39550 ) ;
#59345=EDGE_CURVE ( 'NONE', #30591, #44042, #22954, .T. ) ;
#59346=VERTEX_POINT ( 'NONE', #57879 ) ;
#59347=FACE_OUTER_BOUND ( 'NONE', #49017, .T. ) ;
#59348=FACE_OUTER_BOUND ( 'NONE', #26009, .T. ) ;
#59353=DIRECTION ( 'NONE',  ( -1.000000000000000000, -0.000000000000000000, 0.000000000000000000 ) ) ;
#59356=DIRECTION ( 'NONE',  ( -1.000000000000000000, -0.000000000000000000, 0.000000000000000000 ) ) ;
#59357=ORIENTED_EDGE ( 'NONE', *, *, #42829, .F. ) ;
#59358=CARTESIAN_POINT ( 'NONE',  ( 35.00000000000000000, 4.705694406421931860E-17, -3.469127814946512892E-15 ) ) ;
#59361=ORIENTED_EDGE ( 'NONE', *, *, #58004, .F. ) ;
#59362=CARTESIAN_POINT ( 'NONE',  ( -35.00000000000000000, 0.06441628369853458214, -12.18632975068353019 ) ) ;
#59364=CARTESIAN_POINT ( 'NONE',  ( -24.38798772506720169, 11.02001175613503925, 7.800463590741535391 ) ) ;
#59365=ADVANCED_FACE ( 'NONE', ( #8301 ), #21958, .T. ) ;
#59366=CARTESIAN_POINT ( 'NONE',  ( 24.17751860031820144, -2.141477541963367592, 11.80861164620684711 ) ) ;
#59369=VERTEX_POINT ( 'NONE', #2002 ) ;
#59370=ORIENTED_EDGE ( 'NONE', *, *, #6994, .F. ) ;
#59371=EDGE_CURVE ( 'NONE', #35410, #25804, #36088, .T. ) ;
#59372=DIRECTION ( 'NONE',  ( 0.000000000000000000, 0.01356324068817998940, -0.9999080150203990547 ) ) ;
#59373=LINE ( 'NONE', #26333, #65079 ) ;
#59378=CARTESIAN_POINT ( 'NONE',  ( 37.00000000000000711, -5.921969905510278132, 10.14408668126219304 ) ) ;
#59380=DIRECTION ( 'NONE',  ( 0.000000000000000000, -0.01356324068817998940, 0.9999080150203990547 ) ) ;
#59381=EDGE_CURVE ( 'NONE', #60329, #53266, #24431, .T. ) ;
#59382=ORIENTED_EDGE ( 'NONE', *, *, #50996, .T. ) ;
#59383=AXIS2_PLACEMENT_3D ( 'NONE', #63221, #11057, #17691 ) ;
#59384=EDGE_CURVE ( 'NONE', #40797, #24451, #4275, .T. ) ;
#59385=EDGE_LOOP ( 'NONE', ( #59618, #60047, #27893, #49248 ) ) ;
#59386=DIRECTION ( 'NONE',  ( -1.000000000000000000, 0.000000000000000000, 0.000000000000000000 ) ) ;
#59389=AXIS2_PLACEMENT_3D ( 'NONE', #48802, #44124, #38139 ) ;
#59390=AXIS2_PLACEMENT_3D ( 'NONE', #3908, #39127, #60077 ) ;
#59391=CARTESIAN_POINT ( 'NONE',  ( -17.83419946441818027, -9.720786832536937538, -7.036071585506806336 ) ) ;
#59394=AXIS2_PLACEMENT_3D ( 'NONE', #17554, #26866, #47169 ) ;
#59395=CARTESIAN_POINT ( 'NONE',  ( -7.200201640635544464, -1.899635279488593120, -11.84901858051199142 ) ) ;
#59398=PLANE ( 'NONE',  #51980 ) ;
#59399=ORIENTED_EDGE ( 'NONE', *, *, #57835, .T. ) ;
#59407=ORIENTED_EDGE ( 'NONE', *, *, #24598, .F. ) ;
#59408=FACE_OUTER_BOUND ( 'NONE', #57158, .T. ) ;
#59411=ORIENTED_EDGE ( 'NONE', *, *, #16070, .T. ) ;
#59412=CARTESIAN_POINT ( 'NONE',  ( -9.367105207800477729, -2.739720568162369307, -13.21991852363683506 ) ) ;
#59413=DIRECTION ( 'NONE',  ( 0.000000000000000000, -0.01356324068817992175, 0.9999080150203990547 ) ) ;
#59414=CARTESIAN_POINT ( 'NONE',  ( 17.00162812139343416, -11.45156432714296635, 7.188684627388551185 ) ) ;
#59415=DIRECTION ( 'NONE',  ( -1.000000000000000000, 0.000000000000000000, 0.000000000000000000 ) ) ;
#59416=CARTESIAN_POINT ( 'NONE',  ( -9.502270498702225510, -12.89234730350994340, -4.021714702740394110 ) ) ;
#59418=AXIS2_PLACEMENT_3D ( 'NONE', #48866, #9249, #58868 ) ;
#59420=ORIENTED_EDGE ( 'NONE', *, *, #16120, .T. ) ;
#59421=DIRECTION ( 'NONE',  ( 0.000000000000000000, -0.01356324068817991828, 0.9999080150203990547 ) ) ;
#59423=DIRECTION ( 'NONE',  ( -1.000000000000000000, 0.000000000000000000, 0.000000000000000000 ) ) ;
#59424=CARTESIAN_POINT ( 'NONE',  ( 37.00000000000000711, 7.817610399097634222, 8.766823244861901898 ) ) ;
#59426=DIRECTION ( 'NONE',  ( -1.000000000000000000, 0.000000000000000000, -0.000000000000000000 ) ) ;
#59427=AXIS2_PLACEMENT_3D ( 'NONE', #32621, #16698, #42952 ) ;
#59429=CARTESIAN_POINT ( 'NONE',  ( -30.04249239712260788, 0.3851321492415041847, -12.00220082160331891 ) ) ;
#59431=ORIENTED_EDGE ( 'NONE', *, *, #60715, .F. ) ;
#59432=VERTEX_POINT ( 'NONE', #12957 ) ;
#59433=EDGE_CURVE ( 'NONE', #57314, #38680, #60192, .T. ) ;
#59434=CARTESIAN_POINT ( 'NONE',  ( -17.74424199868676766, -6.571554700141313710, -10.04532163134672551 ) ) ;
#59435=ORIENTED_EDGE ( 'NONE', *, *, #3512, .T. ) ;
#59437=AXIS2_PLACEMENT_3D ( 'NONE', #10668, #61534, #716 ) ;
#59438=CARTESIAN_POINT ( 'NONE',  ( -35.00000000000000000, -5.636262487437237567, -10.80478261802188023 ) ) ;
#59440=CARTESIAN_POINT ( 'NONE',  ( 35.00000000000000000, -11.56998259273180274, -3.827046518385039064 ) ) ;
#59441=CIRCLE ( 'NONE', #2102, 4.999999999999999112 ) ;
#59443=LINE ( 'NONE', #38504, #63058 ) ;
#59447=ORIENTED_EDGE ( 'NONE', *, *, #31166, .T. ) ;
#59448=ORIENTED_EDGE ( 'NONE', *, *, #63752, .F. ) ;
#59454=DIRECTION ( 'NONE',  ( 1.000000000000000000, 0.000000000000000000, 0.000000000000000000 ) ) ;
#59455=DIRECTION ( 'NONE',  ( -1.000000000000000000, -0.000000000000000000, 0.000000000000000000 ) ) ;
#59457=CARTESIAN_POINT ( 'NONE',  ( -7.489022030332961322, 8.034049540753141372, -10.84914964302385521 ) ) ;
#59463=CARTESIAN_POINT ( 'NONE',  ( -16.80243436552160574, 7.513500008141047459, 9.356964553287092201 ) ) ;
#59465=EDGE_CURVE ( 'NONE', #51290, #27983, #1095, .T. ) ;
#59477=EDGE_CURVE ( 'NONE', #44848, #3064, #3196, .T. ) ;
#59478=ORIENTED_EDGE ( 'NONE', *, *, #24598, .T. ) ;
#59479=CARTESIAN_POINT ( 'NONE',  ( 37.00000000000000711, -12.74068829017554094, -0.4871980014161064743 ) ) ;
#59480=CARTESIAN_POINT ( 'NONE',  ( 35.00000000000000000, 4.705694406421931860E-17, -3.469127814946512892E-15 ) ) ;
#59482=EDGE_CURVE ( 'NONE', #29583, #57508, #24903, .T. ) ;
#59484=CARTESIAN_POINT ( 'NONE',  ( -35.00000000000000000, -6.036400161834495570, -10.07641281632183983 ) ) ;
#59487=DIRECTION ( 'NONE',  ( 0.000000000000000000, -1.000000000000000000, 0.000000000000000000 ) ) ;
#59488=CARTESIAN_POINT ( 'NONE',  ( 12.52750123246316072, 0.4973700281276248192, 11.98968819674307618 ) ) ;
#59490=AXIS2_PLACEMENT_3D ( 'NONE', #29811, #4576, #60404 ) ;
#59491=AXIS2_PLACEMENT_3D ( 'NONE', #44128, #18566, #35104 ) ;
#59493=EDGE_LOOP ( 'NONE', ( #8521, #22548, #12622, #49570 ) ) ;
#59495=VERTEX_POINT ( 'NONE', #9256 ) ;
#59497=CARTESIAN_POINT ( 'NONE',  ( 35.00000000000000000, 4.705694406421931860E-17, -3.469127814946512892E-15 ) ) ;
#59498=CIRCLE ( 'NONE', #36116, 4.999999999999999112 ) ;
#59500=DIRECTION ( 'NONE',  ( 0.000000000000000000, 0.01356324068817998940, -0.9999080150203990547 ) ) ;
#59501=EDGE_CURVE ( 'NONE', #34799, #64644, #35044, .T. ) ;
#59503=ORIENTED_EDGE ( 'NONE', *, *, #9296, .T. ) ;
#59504=DIRECTION ( 'NONE',  ( 1.000000000000000000, 0.000000000000000000, 0.000000000000000000 ) ) ;
#59506=DIRECTION ( 'NONE',  ( -0.9854502544271372955, 0.000000000000000000, -0.1699641022377680610 ) ) ;
#59508=CARTESIAN_POINT ( 'NONE',  ( 35.00000000000000000, 10.99909370905164430, 5.246972444133898072 ) ) ;
#59511=ORIENTED_EDGE ( 'NONE', *, *, #16723, .F. ) ;
#59512=VECTOR ( 'NONE', #58724, 1000.000000000000000 ) ;
#59517=AXIS2_PLACEMENT_3D ( 'NONE', #6918, #58788, #37490 ) ;
#59518=FACE_OUTER_BOUND ( 'NONE', #35279, .T. ) ;
#59519=AXIS2_PLACEMENT_3D ( 'NONE', #8699, #29303, #14324 ) ;
#59520=CIRCLE ( 'NONE', #15861, 5.000000000000001776 ) ;
#59521=AXIS2_PLACEMENT_3D ( 'NONE', #40523, #10584, #60154 ) ;
#59524=CARTESIAN_POINT ( 'NONE',  ( -35.00000000000000000, -9.700295462048607931, -7.376655759824990000 ) ) ;
#59525=ORIENTED_EDGE ( 'NONE', *, *, #3625, .T. ) ;
#59527=DIRECTION ( 'NONE',  ( 0.000000000000000000, -0.01356324068817998940, 0.9999080150203990547 ) ) ;
#59528=CYLINDRICAL_SURFACE ( 'NONE', #33522, 8.549672981451799103 ) ;
#59530=ORIENTED_EDGE ( 'NONE', *, *, #59477, .F. ) ;
#59535=ORIENTED_EDGE ( 'NONE', *, *, #51506, .T. ) ;
#59536=ORIENTED_EDGE ( 'NONE', *, *, #50996, .F. ) ;
#59537=ORIENTED_EDGE ( 'NONE', *, *, #41849, .F. ) ;
#59538=CIRCLE ( 'NONE', #62693, 5.000000000000001776 ) ;
#59541=DIRECTION ( 'NONE',  ( 0.000000000000000000, -0.01356324068817998940, 0.9999080150203990547 ) ) ;
#59543=CARTESIAN_POINT ( 'NONE',  ( -35.00000000000000000, -7.817610399097453922, -8.766823244862070652 ) ) ;
#59545=AXIS2_PLACEMENT_3D ( 'NONE', #28467, #2233, #32465 ) ;
#59547=ORIENTED_EDGE ( 'NONE', *, *, #15999, .T. ) ;
#59549=CARTESIAN_POINT ( 'NONE',  ( -18.07087328174625895, -5.729890374228451044, -12.22671232969771715 ) ) ;
#59551=DIRECTION ( 'NONE',  ( 0.000000000000000000, 0.7196168960969766548, 0.6943713148249667233 ) ) ;
#59555=EDGE_CURVE ( 'NONE', #31409, #30664, #36137, .T. ) ;
#59556=ORIENTED_EDGE ( 'NONE', *, *, #31916, .T. ) ;
#59557=ORIENTED_EDGE ( 'NONE', *, *, #52799, .F. ) ;
#59560=VECTOR ( 'NONE', #54569, 1000.000000000000000 ) ;
#59561=VERTEX_POINT ( 'NONE', #43873 ) ;
#59562=CARTESIAN_POINT ( 'NONE',  ( -26.80268169419326085, -12.44861804319972265, 5.223704780996759389 ) ) ;
#59563=CARTESIAN_POINT ( 'NONE',  ( -37.00000000000000711, 1.771820996347319710, -11.61175578952784448 ) ) ;
#59564=CARTESIAN_POINT ( 'NONE',  ( -30.18541646480390384, -1.416020129149325513, 13.42553116244798517 ) ) ;
#59566=CARTESIAN_POINT ( 'NONE',  ( -2.924554904731178961, 11.04673857066214815, 4.702770982435475311 ) ) ;
#59567=VECTOR ( 'NONE', #57378, 1000.000000000000000 ) ;
#59568=CARTESIAN_POINT ( 'NONE',  ( 13.10189188732837628, 9.774122605474259373, -6.975859618942914508 ) ) ;
#59569=ORIENTED_EDGE ( 'NONE', *, *, #56543, .F. ) ;
#59572=AXIS2_PLACEMENT_3D ( 'NONE', #18115, #3505, #9416 ) ;
#59577=DIRECTION ( 'NONE',  ( -0.000000000000000000, -1.000000000000000000, -0.000000000000000000 ) ) ;
#59578=DIRECTION ( 'NONE',  ( 1.000000000000000000, 0.000000000000000000, 0.000000000000000000 ) ) ;
#59580=AXIS2_PLACEMENT_3D ( 'NONE', #57493, #47512, #41513 ) ;
#59581=CIRCLE ( 'NONE', #54279, 12.74999999999999822 ) ;
#59582=EDGE_CURVE ( 'NONE', #2444, #65068, #17030, .T. ) ;
#59584=CARTESIAN_POINT ( 'NONE',  ( 37.00000000000000711, 1.488153103996963100, -11.65150730582935523 ) ) ;
#59585=CIRCLE ( 'NONE', #30905, 4.999999999999999112 ) ;
#59586=CIRCLE ( 'NONE', #24550, 11.99999999999998579 ) ;
#59587=ADVANCED_FACE ( 'NONE', ( #39197 ), #19906, .T. ) ;
#59588=ORIENTED_EDGE ( 'NONE', *, *, #24116, .T. ) ;
#59592=DIRECTION ( 'NONE',  ( 1.000000000000000000, 0.000000000000000000, 0.000000000000000000 ) ) ;
#59593=ORIENTED_EDGE ( 'NONE', *, *, #32560, .T. ) ;
#59594=AXIS2_PLACEMENT_3D ( 'NONE', #22838, #22500, #7518 ) ;
#59596=VERTEX_POINT ( 'NONE', #55486 ) ;
#59597=VERTEX_POINT ( 'NONE', #14564 ) ;
#59600=ORIENTED_EDGE ( 'NONE', *, *, #45104, .T. ) ;
#59601=CARTESIAN_POINT ( 'NONE',  ( 35.00000000000000000, -7.251710744571640888, -9.240395740215610942 ) ) ;
#59602=CYLINDRICAL_SURFACE ( 'NONE', #35745, 5.000000000000000888 ) ;
#59604=AXIS2_PLACEMENT_3D ( 'NONE', #30981, #46606, #10364 ) ;
#59605=CARTESIAN_POINT ( 'NONE',  ( -47.00000000000000711, 0.000000000000000000, 0.000000000000000000 ) ) ;
#59607=DIRECTION ( 'NONE',  ( 0.000000000000000000, -0.8989688749565202253, -0.4380125133593882336 ) ) ;
#59609=DIRECTION ( 'NONE',  ( -1.000000000000000000, 0.000000000000000000, 0.000000000000000000 ) ) ;
#59610=CARTESIAN_POINT ( 'NONE',  ( 37.00000000000000711, -9.926225166346981155, 6.280308599560240346 ) ) ;
#59611=EDGE_LOOP ( 'NONE', ( #22986, #27886, #13279, #38311 ) ) ;
#59613=VECTOR ( 'NONE', #21130, 1000.000000000000000 ) ;
#59614=EDGE_CURVE ( 'NONE', #21230, #28220, #14258, .T. ) ;
#59616=ORIENTED_EDGE ( 'NONE', *, *, #561, .F. ) ;
#59617=DIRECTION ( 'NONE',  ( 0.000000000000000000, -0.01356324068817998940, 0.9999080150203990547 ) ) ;
#59618=ORIENTED_EDGE ( 'NONE', *, *, #19827, .F. ) ;
#59619=CARTESIAN_POINT ( 'NONE',  ( 37.00000000000000711, -4.603882218679472338, 10.80631716521671493 ) ) ;
#59621=ADVANCED_FACE ( 'NONE', ( #25545 ), #45837, .T. ) ;
#59622=DIRECTION ( 'NONE',  ( 1.000000000000000000, -0.000000000000000000, 0.000000000000000000 ) ) ;
#59624=VECTOR ( 'NONE', #39206, 1000.000000000000000 ) ;
#59625=AXIS2_PLACEMENT_3D ( 'NONE', #6829, #12433, #32396 ) ;
#59627=DIRECTION ( 'NONE',  ( -1.000000000000000000, 0.000000000000000000, -0.000000000000000000 ) ) ;
#59629=DIRECTION ( 'NONE',  ( -1.000000000000000000, 0.000000000000000000, 0.000000000000000000 ) ) ;
#59630=ORIENTED_EDGE ( 'NONE', *, *, #51300, .F. ) ;
#59632=ORIENTED_EDGE ( 'NONE', *, *, #5528, .F. ) ;
#59633=CARTESIAN_POINT ( 'NONE',  ( 36.00000000000000711, 8.624332853796058629, -9.390600770288022758 ) ) ;
#59634=ORIENTED_EDGE ( 'NONE', *, *, #53569, .T. ) ;
#59637=DIRECTION ( 'NONE',  ( 1.000000000000000000, 0.000000000000000000, -0.000000000000000000 ) ) ;
#59641=ADVANCED_FACE ( 'NONE', ( #56125 ), #61774, .T. ) ;
#59642=AXIS2_PLACEMENT_3D ( 'NONE', #23345, #39281, #3084 ) ;
#59644=CYLINDRICAL_SURFACE ( 'NONE', #40826, 4.999999999999999112 ) ;
#59646=EDGE_CURVE ( 'NONE', #19021, #53819, #20228, .T. ) ;
#59647=VERTEX_POINT ( 'NONE', #30524 ) ;
#59649=AXIS2_PLACEMENT_3D ( 'NONE', #4159, #50039, #24768 ) ;
#59650=DIRECTION ( 'NONE',  ( 1.000000000000000000, 0.000000000000000000, 0.000000000000000000 ) ) ;
#59652=ORIENTED_EDGE ( 'NONE', *, *, #51653, .F. ) ;
#59653=CIRCLE ( 'NONE', #49039, 12.18649999999999878 ) ;
#59654=CARTESIAN_POINT ( 'NONE',  ( -7.952749643240611732, -1.708398112507050204, 13.39193977470096542 ) ) ;
#59656=CIRCLE ( 'NONE', #34009, 12.18650000000000233 ) ;
#59657=AXIS2_PLACEMENT_3D ( 'NONE', #955, #30232, #51187 ) ;
#59658=ORIENTED_EDGE ( 'NONE', *, *, #14786, .F. ) ;
#59660=CARTESIAN_POINT ( 'NONE',  ( 29.03457606387295087, 4.854210015632069997, 10.97436308512422265 ) ) ;
#59661=CARTESIAN_POINT ( 'NONE',  ( -37.00000000000000711, 11.02904044024209185, -4.041347439435899247 ) ) ;
#59662=VECTOR ( 'NONE', #32730, 1000.000000000000000 ) ;
#59663=CIRCLE ( 'NONE', #1242, 12.18649999999999700 ) ;
#59664=AXIS2_PLACEMENT_3D ( 'NONE', #64311, #39042, #18114 ) ;
#59665=DIRECTION ( 'NONE',  ( 0.000000000000000000, 0.01356324068817991828, -0.9999080150203990547 ) ) ;
#59666=CARTESIAN_POINT ( 'NONE',  ( 35.00000000000000000, 8.295159312811978936, 8.927548052240801724 ) ) ;
#59668=ORIENTED_EDGE ( 'NONE', *, *, #44516, .F. ) ;
#59670=DIRECTION ( 'NONE',  ( 0.000000000000000000, 0.9999080150203989437, 0.01356324068818338426 ) ) ;
#59671=DIRECTION ( 'NONE',  ( 0.8405098440481681976, 0.000000000000000000, -0.5417962735734934698 ) ) ;
#59672=VERTEX_POINT ( 'NONE', #16566 ) ;
#59673=CYLINDRICAL_SURFACE ( 'NONE', #14870, 4.999999999999999112 ) ;
#59675=ORIENTED_EDGE ( 'NONE', *, *, #34046, .T. ) ;
#59676=ORIENTED_EDGE ( 'NONE', *, *, #14707, .F. ) ;
#59677=LINE ( 'NONE', #39374, #36343 ) ;
#59678=VECTOR ( 'NONE', #65263, 1000.000000000000000 ) ;
#59680=EDGE_LOOP ( 'NONE', ( #41627, #19540, #6771, #36307 ) ) ;
#59681=AXIS2_PLACEMENT_3D ( 'NONE', #24077, #45659, #35345 ) ;
#59683=DIRECTION ( 'NONE',  ( 0.000000000000000000, -0.8696919319575239227, -0.4935949184179166394 ) ) ;
#59684=CARTESIAN_POINT ( 'NONE',  ( -17.54726996257253191, 25.00000000000000000, 3.865003848717349033 ) ) ;
#59685=CARTESIAN_POINT ( 'NONE',  ( -47.00000000000000711, 0.000000000000000000, 0.000000000000000000 ) ) ;
#59686=VECTOR ( 'NONE', #29994, 1000.000000000000000 ) ;
#59688=DIRECTION ( 'NONE',  ( -0.8758382566188793739, 0.4826047536471247956, 0.000000000000000000 ) ) ;
#59695=VERTEX_POINT ( 'NONE', #51167 ) ;
#59696=DIRECTION ( 'NONE',  ( -0.9854502544271372955, 0.000000000000000000, -0.1699641022377680610 ) ) ;
#59699=CARTESIAN_POINT ( 'NONE',  ( -24.75879207840611684, 11.63908045720823736, 6.841945026260960461 ) ) ;
#59700=CARTESIAN_POINT ( 'NONE',  ( 22.86323487647331021, 2.804901635794770254, 11.66983792800902542 ) ) ;
#59703=ORIENTED_EDGE ( 'NONE', *, *, #64347, .F. ) ;
#59704=AXIS2_PLACEMENT_3D ( 'NONE', #29434, #13800, #34088 ) ;
#59706=DIRECTION ( 'NONE',  ( -1.000000000000000000, 0.000000000000000000, 0.000000000000000000 ) ) ;
#59707=ORIENTED_EDGE ( 'NONE', *, *, #43434, .T. ) ;
#59709=AXIS2_PLACEMENT_3D ( 'NONE', #53049, #37759, #32740 ) ;
#59710=CARTESIAN_POINT ( 'NONE',  ( -10.48620311856347875, -9.720786832536937538, 7.036071585506805448 ) ) ;
#59712=DIRECTION ( 'NONE',  ( 0.000000000000000000, -0.01356324068817992175, 0.9999080150203990547 ) ) ;
#59714=CIRCLE ( 'NONE', #31030, 12.75000000000000178 ) ;
#59715=DIRECTION ( 'NONE',  ( 0.000000000000000000, -0.01356324068818000848, 0.9999080150203990547 ) ) ;
#59716=VECTOR ( 'NONE', #62662, 1000.000000000000000 ) ;
#59717=CARTESIAN_POINT ( 'NONE',  ( 37.00000000000000711, -8.534258022646033837, 8.699265615723071221 ) ) ;
#59718=ORIENTED_EDGE ( 'NONE', *, *, #39032, .T. ) ;
#59719=VERTEX_POINT ( 'NONE', #40506 ) ;
#59720=CARTESIAN_POINT ( 'NONE',  ( -35.00000000000000000, 0.000000000000000000, 0.000000000000000000 ) ) ;
#59721=DIRECTION ( 'NONE',  ( 0.000000000000000000, -0.01356324068817991828, 0.9999080150203990547 ) ) ;
#59723=AXIS2_PLACEMENT_3D ( 'NONE', #1561, #17494, #42394 ) ;
#59724=EDGE_CURVE ( 'NONE', #12098, #60025, #25217, .T. ) ;
#59725=CIRCLE ( 'NONE', #39539, 12.18649999999999878 ) ;
#59726=DIRECTION ( 'NONE',  ( 0.000000000000000000, 0.01356324068817998940, -0.9999080150203990547 ) ) ;
#59727=DIRECTION ( 'NONE',  ( 0.000000000000000000, -0.01356324068817992175, 0.9999080150203990547 ) ) ;
#59729=CARTESIAN_POINT ( 'NONE',  ( -10.66166322600637173, -5.805694913916275901, -10.50405896137098161 ) ) ;
#59731=AXIS2_PLACEMENT_3D ( 'NONE', #54139, #58481, #27890 ) ;
#59732=CARTESIAN_POINT ( 'NONE',  ( 35.00000000000000000, 6.415447294506860132, 11.01837265713066039 ) ) ;
#59733=CYLINDRICAL_SURFACE ( 'NONE', #58389, 4.999999999999999112 ) ;
#59735=CARTESIAN_POINT ( 'NONE',  ( -36.00000000000000711, -12.38385022362079724, -3.033604067594711129 ) ) ;
#59736=CARTESIAN_POINT ( 'NONE',  ( -35.00000000000000000, -2.346765782874520312, 11.95840593935200680 ) ) ;
#59737=CYLINDRICAL_SURFACE ( 'NONE', #33327, 4.999999999999998224 ) ;
#59740=CARTESIAN_POINT ( 'NONE',  ( -27.45775109278351067, -8.499184579339635448, -8.471355351200609007 ) ) ;
#59741=EDGE_CURVE ( 'NONE', #35230, #15987, #46486, .T. ) ;
#59742=ORIENTED_EDGE ( 'NONE', *, *, #97, .T. ) ;
#59744=CARTESIAN_POINT ( 'NONE',  ( 37.00000000000000711, -11.70009620280412399, -1.039216533672868481 ) ) ;
#59746=ORIENTED_EDGE ( 'NONE', *, *, #57144, .F. ) ;
#59749=CARTESIAN_POINT ( 'NONE',  ( -28.24693446298985577, -12.60603044485271873, -4.840642766324885216 ) ) ;
#59750=DIRECTION ( 'NONE',  ( 1.000000000000000000, 0.000000000000000000, 0.000000000000000000 ) ) ;
#59752=AXIS2_PLACEMENT_3D ( 'NONE', #59204, #3026, #13621 ) ;
#59753=DIRECTION ( 'NONE',  ( -0.000000000000000000, -1.000000000000000000, -0.000000000000000000 ) ) ;
#59754=CARTESIAN_POINT ( 'NONE',  ( -7.971167194659495969, -8.542028475013285771, -10.47297933864158104 ) ) ;
#59758=ORIENTED_EDGE ( 'NONE', *, *, #24873, .F. ) ;
#59760=CARTESIAN_POINT ( 'NONE',  ( 35.00000000000000000, 3.093009498343925134, -11.78745411414841016 ) ) ;
#59761=DIRECTION ( 'NONE',  ( 0.000000000000000000, 0.7790879021242487212, -0.6269146997508011632 ) ) ;
#59766=CARTESIAN_POINT ( 'NONE',  ( -30.18541646480307961, -1.416020129149133888, -11.91616074890920807 ) ) ;
#59768=ORIENTED_EDGE ( 'NONE', *, *, #57948, .F. ) ;
#59770=CARTESIAN_POINT ( 'NONE',  ( -18.25006854224444908, -9.443202773001939221, -7.404452808139720510 ) ) ;
#59771=CIRCLE ( 'NONE', #8793, 12.18650000000000233 ) ;
#59772=ORIENTED_EDGE ( 'NONE', *, *, #35210, .T. ) ;
#59776=CARTESIAN_POINT ( 'NONE',  ( -18.10941110424452916, -9.537088721069792996, 9.555689318548472144 ) ) ;
#59777=VERTEX_POINT ( 'NONE', #6595 ) ;
#59779=DIRECTION ( 'NONE',  ( 1.000000000000000000, 0.000000000000000000, -0.000000000000000000 ) ) ;
#59780=DIRECTION ( 'NONE',  ( 1.000000000000000000, 0.000000000000000000, 0.000000000000000000 ) ) ;
#59781=VERTEX_POINT ( 'NONE', #58112 ) ;
#59782=ORIENTED_EDGE ( 'NONE', *, *, #15337, .T. ) ;
#59785=ORIENTED_EDGE ( 'NONE', *, *, #46244, .F. ) ;
#59786=CARTESIAN_POINT ( 'NONE',  ( -27.65870282641429867, -11.28224200227462859, -4.098090116028304308 ) ) ;
#59788=CARTESIAN_POINT ( 'NONE',  ( -19.55198024779261345, -3.902068674853249153, -11.34897822738861883 ) ) ;
#59789=CYLINDRICAL_SURFACE ( 'NONE', #11410, 6.095312090839646757 ) ;
#59791=PLANE ( 'NONE',  #9336 ) ;
#59793=ORIENTED_EDGE ( 'NONE', *, *, #55556, .T. ) ;
#59797=FACE_OUTER_BOUND ( 'NONE', #51677, .T. ) ;
#59798=AXIS2_PLACEMENT_3D ( 'NONE', #60479, #4313, #29894 ) ;
#59802=DIRECTION ( 'NONE',  ( -1.000000000000000000, 0.000000000000000000, 0.000000000000000000 ) ) ;
#59804=CARTESIAN_POINT ( 'NONE',  ( 35.00000000000000000, 4.705694406421931860E-17, -3.469127814946512892E-15 ) ) ;
#59805=AXIS2_PLACEMENT_3D ( 'NONE', #19991, #29623, #9672 ) ;
#59806=EDGE_CURVE ( 'NONE', #8415, #35879, #47851, .T. ) ;
#59807=AXIS2_PLACEMENT_3D ( 'NONE', #58548, #12973, #33590 ) ;
#59809=CARTESIAN_POINT ( 'NONE',  ( 37.00000000000000711, -4.018060380616318206, 11.50504120060946533 ) ) ;
#59811=ORIENTED_EDGE ( 'NONE', *, *, #52170, .F. ) ;
#59812=CARTESIAN_POINT ( 'NONE',  ( -30.18541646480307961, -1.416020129149133888, -11.91616074890920807 ) ) ;
#59815=AXIS2_PLACEMENT_3D ( 'NONE', #46969, #21707, #41960 ) ;
#59816=B_SPLINE_CURVE_WITH_KNOTS ( 'NONE', 3,
 ( #61165, #25250, #65791, #30559, #20263, #50863, #20608, #5656, #9616, #35557, #14597, #19938, #55852, #40544, #40886, #15595, #35859, #29913, #34877, #65475 ),
 .UNSPECIFIED., .F., .F.,
 ( 4, 2, 2, 2, 2, 2, 2, 2, 2, 4 ),
 ( 0.000000000000000000, 0.001138311071655714055, 0.002276622143311428110, 0.003414933214967142382, 0.004553244286622856220, 0.005691555358278570058, 0.006829866429934284763, 0.007399021965762139948, 0.007968177501589996867, 0.009106488573245712440 ),
 .UNSPECIFIED. ) ;
#59819=VERTEX_POINT ( 'NONE', #22191 ) ;
#59820=DIRECTION ( 'NONE',  ( -1.000000000000000000, -1.836970198721029688E-16, 0.000000000000000000 ) ) ;
#59822=CARTESIAN_POINT ( 'NONE',  ( 9.270078297875276263, 2.860737070136182059, 11.65636294989809407 ) ) ;
#59825=VECTOR ( 'NONE', #24173, 1000.000000000000000 ) ;
#59830=EDGE_CURVE ( 'NONE', #37175, #58284, #35085, .T. ) ;
#59831=AXIS2_PLACEMENT_3D ( 'NONE', #24961, #45233, #65491 ) ;
#59832=CARTESIAN_POINT ( 'NONE',  ( 35.00000000000000000, -5.556331110570486231, -11.47561260193575272 ) ) ;
#59833=ORIENTED_EDGE ( 'NONE', *, *, #42402, .F. ) ;
#59834=EDGE_CURVE ( 'NONE', #5900, #6107, #6459, .T. ) ;
#59835=CARTESIAN_POINT ( 'NONE',  ( -2.532614230583026593, 7.965877694534055031, 10.89930238848911337 ) ) ;
#59836=CARTESIAN_POINT ( 'NONE',  ( 35.00000000000000000, 7.561043153948098450, 9.557269938331469206 ) ) ;
#59838=CARTESIAN_POINT ( 'NONE',  ( -37.00000000000000711, -4.041347439435779343, -11.02904044024213270 ) ) ;
#59839=VECTOR ( 'NONE', #49972, 1000.000000000000000 ) ;
#59840=ORIENTED_EDGE ( 'NONE', *, *, #27825, .T. ) ;
#59841=ADVANCED_FACE ( 'NONE', ( #27844 ), #32805, .T. ) ;
#59843=CARTESIAN_POINT ( 'NONE',  ( 37.00000000000000711, -11.56998259273180274, -3.827046518385039064 ) ) ;
#59844=DIRECTION ( 'NONE',  ( -1.000000000000000000, 0.000000000000000000, 0.000000000000000000 ) ) ;
#59852=ORIENTED_EDGE ( 'NONE', *, *, #23660, .F. ) ;
#59858=AXIS2_PLACEMENT_3D ( 'NONE', #13684, #33964, #48965 ) ;
#59860=VERTEX_POINT ( 'NONE', #22870 ) ;
#59862=EDGE_CURVE ( 'NONE', #19519, #18553, #30825, .T. ) ;
#59863=CYLINDRICAL_SURFACE ( 'NONE', #58705, 11.99999999999999289 ) ;
#59865=CARTESIAN_POINT ( 'NONE',  ( -37.00000000000000711, 1.457575200925721237, -12.66641127287624435 ) ) ;
#59866=DIRECTION ( 'NONE',  ( 0.000000000000000000, -0.9987865678893271815, 0.04924826701375695226 ) ) ;
#59869=CIRCLE ( 'NONE', #38638, 12.18649999999999878 ) ;
#59871=EDGE_CURVE ( 'NONE', #433, #23887, #7218, .T. ) ;
#59872=CARTESIAN_POINT ( 'NONE',  ( 35.00000000000000000, 4.705694406421931860E-17, -3.469127814946512892E-15 ) ) ;
#59873=ORIENTED_EDGE ( 'NONE', *, *, #37572, .F. ) ;
#59874=CARTESIAN_POINT ( 'NONE',  ( 10.57567362079633355, 8.112553359107785411, 10.79197710481157557 ) ) ;
#59880=CIRCLE ( 'NONE', #3602, 12.74999999999999822 ) ;
#59882=CARTESIAN_POINT ( 'NONE',  ( -35.00000000000000000, 3.704519465651306742, 11.60979404548636218 ) ) ;
#59886=ORIENTED_EDGE ( 'NONE', *, *, #14548, .F. ) ;
#59887=CARTESIAN_POINT ( 'NONE',  ( -35.00000000000000000, -0.1414404973751245964, -12.74921544981111055 ) ) ;
#59888=VECTOR ( 'NONE', #64434, 1000.000000000000000 ) ;
#59889=FACE_OUTER_BOUND ( 'NONE', #22911, .T. ) ;
#59892=CARTESIAN_POINT ( 'NONE',  ( -35.00000000000000000, 0.000000000000000000, 0.000000000000000000 ) ) ;
#59894=ORIENTED_EDGE ( 'NONE', *, *, #14604, .F. ) ;
#59897=VECTOR ( 'NONE', #31235, 1000.000000000000000 ) ;
#59898=ORIENTED_EDGE ( 'NONE', *, *, #62834, .T. ) ;
#59901=DIRECTION ( 'NONE',  ( -1.000000000000000000, 0.000000000000000000, 0.000000000000000000 ) ) ;
#59903=CARTESIAN_POINT ( 'NONE',  ( 35.00000000000000000, 1.286231064351314624, -12.68495603654572257 ) ) ;
#59905=CARTESIAN_POINT ( 'NONE',  ( 13.33628443002342046, 11.16462474940892236, -4.404581277556346208 ) ) ;
#59907=CIRCLE ( 'NONE', #3631, 4.999999999999997335 ) ;
#59909=AXIS2_PLACEMENT_3D ( 'NONE', #56599, #26012, #2650 ) ;
#59910=CARTESIAN_POINT ( 'NONE',  ( -35.00000000000000000, -11.72195762423409349, -0.7536123767499773862 ) ) ;
#59912=AXIS2_PLACEMENT_3D ( 'NONE', #60234, #9683, #4740 ) ;
#59913=EDGE_CURVE ( 'NONE', #62432, #11383, #22535, .T. ) ;
#59914=DIRECTION ( 'NONE',  ( 1.000000000000000000, -0.000000000000000000, 0.000000000000000000 ) ) ;
#59915=CIRCLE ( 'NONE', #33318, 12.75000000000000178 ) ;
#59917=EDGE_CURVE ( 'NONE', #52994, #55534, #6412, .T. ) ;
#59919=CARTESIAN_POINT ( 'NONE',  ( -35.00000000000000000, 0.000000000000000000, 0.000000000000000000 ) ) ;
#59920=DIRECTION ( 'NONE',  ( 0.000000000000000000, 0.8827602140260332186, -0.4698238015817334245 ) ) ;
#59922=ORIENTED_EDGE ( 'NONE', *, *, #4121, .T. ) ;
#59923=CARTESIAN_POINT ( 'NONE',  ( 37.00000000000000711, 3.287724142101414504, -11.73463472867577373 ) ) ;
#59924=ORIENTED_EDGE ( 'NONE', *, *, #30170, .F. ) ;
#59925=CARTESIAN_POINT ( 'NONE',  ( -14.23149639848878678, 7.941839253138335941, -8.998400932456027235 ) ) ;
#59928=AXIS2_PLACEMENT_3D ( 'NONE', #25652, #10345, #24675 ) ;
#59929=EDGE_CURVE ( 'NONE', #58896, #49993, #19023, .T. ) ;
#59931=EDGE_LOOP ( 'NONE', ( #11574, #13514, #42039, #56873 ) ) ;
#59932=EDGE_LOOP ( 'NONE', ( #24972, #36264, #23712, #59175 ) ) ;
#59935=EDGE_CURVE ( 'NONE', #9125, #36890, #12215, .T. ) ;
#59936=AXIS2_PLACEMENT_3D ( 'NONE', #29677, #30020, #39996 ) ;
#59937=DIRECTION ( 'NONE',  ( -1.000000000000000000, 0.000000000000000000, 0.000000000000000000 ) ) ;
#59938=ORIENTED_EDGE ( 'NONE', *, *, #59003, .F. ) ;
#59939=ADVANCED_FACE ( 'NONE', ( #42132 ), #45101, .T. ) ;
#59944=EDGE_LOOP ( 'NONE', ( #31141, #51992, #17471, #28202 ) ) ;
#59947=CARTESIAN_POINT ( 'NONE',  ( -29.92777678363736626, -3.750539801530011985, 11.39883551934754635 ) ) ;
#59952=ORIENTED_EDGE ( 'NONE', *, *, #13883, .F. ) ;
#59953=AXIS2_PLACEMENT_3D ( 'NONE', #9777, #25402, #45682 ) ;
#59955=ORIENTED_EDGE ( 'NONE', *, *, #12914, .F. ) ;
#59956=CARTESIAN_POINT ( 'NONE',  ( 11.74548640120467979, 25.00000000000000000, -8.184666801472349817 ) ) ;
#59957=CARTESIAN_POINT ( 'NONE',  ( 12.34777221413211912, -11.79052471001755009, -2.240005522967919216 ) ) ;
#59959=CYLINDRICAL_SURFACE ( 'NONE', #2527, 12.18649999999999878 ) ;
#59961=CARTESIAN_POINT ( 'NONE',  ( -35.00000000000000000, 0.000000000000000000, 0.000000000000000000 ) ) ;
#59963=LINE ( 'NONE', #49654, #33133 ) ;
#59969=EDGE_LOOP ( 'NONE', ( #27496, #47533, #43198, #58370 ) ) ;
#59971=DIRECTION ( 'NONE',  ( -1.000000000000000000, -0.000000000000000000, 0.000000000000000000 ) ) ;
#59973=CARTESIAN_POINT ( 'NONE',  ( 36.00000000000000711, 8.017674001891782254, -9.913596905230145140 ) ) ;
#59974=DIRECTION ( 'NONE',  ( 1.000000000000000000, -0.000000000000000000, 0.000000000000000000 ) ) ;
#59975=VECTOR ( 'NONE', #44366, 1000.000000000000000 ) ;
#59978=CARTESIAN_POINT ( 'NONE',  ( 35.00000000000000000, 3.805206332242470513, -12.16893194857551386 ) ) ;
#59979=EDGE_CURVE ( 'NONE', #2869, #35192, #4668, .T. ) ;
#59981=CARTESIAN_POINT ( 'NONE',  ( -14.11589373245165469, 8.250315036047107142, 10.68561190601526611 ) ) ;
#59984=ORIENTED_EDGE ( 'NONE', *, *, #44574, .T. ) ;
#59985=EDGE_CURVE ( 'NONE', #57610, #52011, #25823, .T. ) ;
#59986=CIRCLE ( 'NONE', #7919, 12.74999999999999822 ) ;
#59988=CARTESIAN_POINT ( 'NONE',  ( -8.073144562555491177, -2.358972950292971049, 13.29271665687120674 ) ) ;
#59992=DIRECTION ( 'NONE',  ( -1.000000000000000000, 0.000000000000000000, 0.000000000000000000 ) ) ;
#59994=EDGE_CURVE ( 'NONE', #11634, #30317, #12790, .T. ) ;
#59995=CARTESIAN_POINT ( 'NONE',  ( 36.00000000000000711, -12.60630747491661374, 1.908798535168511057 ) ) ;
#59996=CARTESIAN_POINT ( 'NONE',  ( 35.00000000000000000, 4.705694406421931860E-17, -3.469127814946512892E-15 ) ) ;
#59997=ORIENTED_EDGE ( 'NONE', *, *, #11476, .F. ) ;
#60000=CARTESIAN_POINT ( 'NONE',  ( -37.00000000000000711, -4.400442035671033203, 11.96656215839367654 ) ) ;
#60001=ORIENTED_EDGE ( 'NONE', *, *, #64995, .T. ) ;
#60002=CARTESIAN_POINT ( 'NONE',  ( 35.00000000000000000, 6.891188680298960811, 9.512294188640820991 ) ) ;
#60003=DIRECTION ( 'NONE',  ( -0.8405098440481674205, 0.000000000000000000, -0.5417962735734949131 ) ) ;
#60004=VERTEX_POINT ( 'NONE', #10826 ) ;
#60007=CARTESIAN_POINT ( 'NONE',  ( 37.00000000000000711, -6.753013023069642351, 10.14433819232440825 ) ) ;
#60009=ORIENTED_EDGE ( 'NONE', *, *, #5249, .T. ) ;
#60010=ADVANCED_FACE ( 'NONE', ( #16147 ), #50431, .T. ) ;
#60011=DIRECTION ( 'NONE',  ( 1.000000000000000000, -0.000000000000000000, -0.000000000000000000 ) ) ;
#60012=CYLINDRICAL_SURFACE ( 'NONE', #4939, 12.18650000000000055 ) ;
#60017=CARTESIAN_POINT ( 'NONE',  ( -35.00000000000000000, -5.246972444134095248, 10.99909370905155370 ) ) ;
#60020=ADVANCED_FACE ( 'NONE', ( #10169 ), #41076, .T. ) ;
#60021=DIRECTION ( 'NONE',  ( -0.000000000000000000, -0.000000000000000000, -1.000000000000000000 ) ) ;
#60025=VERTEX_POINT ( 'NONE', #40766 ) ;
#60028=DIRECTION ( 'NONE',  ( -1.000000000000000000, 0.000000000000000000, 0.000000000000000000 ) ) ;
#60030=DIRECTION ( 'NONE',  ( -1.000000000000000000, 0.000000000000000000, -0.000000000000000000 ) ) ;
#60032=CARTESIAN_POINT ( 'NONE',  ( 37.00000000000000711, -4.309077947445731027, -10.92721691015454510 ) ) ;
#60035=VERTEX_POINT ( 'NONE', #15794 ) ;
#60039=VERTEX_POINT ( 'NONE', #30762 ) ;
#60044=LINE ( 'NONE', #34738, #1273 ) ;
#60045=DIRECTION ( 'NONE',  ( 0.000000000000000000, 0.01356324068817998073, -0.9999080150203990547 ) ) ;
#60046=EDGE_CURVE ( 'NONE', #19066, #49868, #46844, .T. ) ;
#60047=ORIENTED_EDGE ( 'NONE', *, *, #17508, .F. ) ;
#60048=AXIS2_PLACEMENT_3D ( 'NONE', #46253, #40588, #10641 ) ;
#60050=FACE_OUTER_BOUND ( 'NONE', #50223, .T. ) ;
#60052=CARTESIAN_POINT ( 'NONE',  ( -35.00000000000000000, 0.000000000000000000, 0.000000000000000000 ) ) ;
#60053=CIRCLE ( 'NONE', #28206, 5.000000000000001776 ) ;
#60056=CARTESIAN_POINT ( 'NONE',  ( -10.90165637462999726, -7.183754052287492975, -9.621202272021861290 ) ) ;
#60060=EDGE_CURVE ( 'NONE', #20098, #46347, #44683, .T. ) ;
#60061=ORIENTED_EDGE ( 'NONE', *, *, #22692, .F. ) ;
#60062=PLANE ( 'NONE',  #54780 ) ;
#60064=DIRECTION ( 'NONE',  ( 0.000000000000000000, -0.01356324068817999114, 0.9999080150203989437 ) ) ;
#60065=EDGE_CURVE ( 'NONE', #14286, #55534, #51425, .T. ) ;
#60066=CIRCLE ( 'NONE', #39886, 12.18649999999999878 ) ;
#60068=CARTESIAN_POINT ( 'NONE',  ( -17.87891481078358069, -12.92455976930239814, 3.899497271525862896 ) ) ;
#60069=ORIENTED_EDGE ( 'NONE', *, *, #40231, .T. ) ;
#60070=DIRECTION ( 'NONE',  ( -1.000000000000000000, 0.000000000000000000, -0.000000000000000000 ) ) ;
#60071=CARTESIAN_POINT ( 'NONE',  ( 27.73674564613515514, 12.76067307604452417, 4.417293456390572359 ) ) ;
#60074=DIRECTION ( 'NONE',  ( -1.000000000000000000, 0.000000000000000000, 0.000000000000000000 ) ) ;
#60075=CARTESIAN_POINT ( 'NONE',  ( -28.08468344552528606, -11.68084827141784565, -6.774767069026986555 ) ) ;
#60077=DIRECTION ( 'NONE',  ( 0.000000000000000000, -0.01356324068817998940, 0.9999080150203990547 ) ) ;
#60079=ADVANCED_FACE ( 'NONE', ( #46096 ), #543, .T. ) ;
#60080=CYLINDRICAL_SURFACE ( 'NONE', #38261, 5.000000000000000888 ) ;
#60081=VERTEX_POINT ( 'NONE', #5874 ) ;
#60082=CARTESIAN_POINT ( 'NONE',  ( 3.780834652287974773, 8.352030633203074927, -8.616471685210672860 ) ) ;
#60083=DIRECTION ( 'NONE',  ( 1.000000000000000000, -0.000000000000000000, 0.000000000000000000 ) ) ;
#60084=AXIS2_PLACEMENT_3D ( 'NONE', #57705, #22432, #16480 ) ;
#60085=DIRECTION ( 'NONE',  ( 1.000000000000000000, -0.000000000000000000, 0.000000000000000000 ) ) ;
#60087=DIRECTION ( 'NONE',  ( 1.000000000000000000, -0.000000000000000000, 0.000000000000000000 ) ) ;
#60088=FACE_OUTER_BOUND ( 'NONE', #40878, .T. ) ;
#60089=CYLINDRICAL_SURFACE ( 'NONE', #42460, 12.18650000000000055 ) ;
#60091=ORIENTED_EDGE ( 'NONE', *, *, #41651, .F. ) ;
#60092=CARTESIAN_POINT ( 'NONE',  ( -18.01363938508876927, -9.088990878694016118, -7.856193784715579831 ) ) ;
#60093=VERTEX_POINT ( 'NONE', #26130 ) ;
#60095=CIRCLE ( 'NONE', #18725, 5.000000000000000000 ) ;
#60098=CARTESIAN_POINT ( 'NONE',  ( -19.69476066079020171, -4.201994156881551312, 11.24025111398909615 ) ) ;
#60099=ORIENTED_EDGE ( 'NONE', *, *, #1635, .T. ) ;
#60100=CARTESIAN_POINT ( 'NONE',  ( -35.00000000000000000, 0.000000000000000000, 0.000000000000000000 ) ) ;
#60102=CARTESIAN_POINT ( 'NONE',  ( 23.98498522125079191, 2.278584884918189779, 13.31001393690969969 ) ) ;
#60103=EDGE_LOOP ( 'NONE', ( #29852, #38693, #37359, #42092 ) ) ;
#60106=ORIENTED_EDGE ( 'NONE', *, *, #48253, .T. ) ;
#60107=DIRECTION ( 'NONE',  ( -1.000000000000000000, 0.000000000000000000, 0.000000000000000000 ) ) ;
#60108=VERTEX_POINT ( 'NONE', #17788 ) ;
#60109=DIRECTION ( 'NONE',  ( 0.000000000000000000, -0.9651210252299822212, -0.2618041379715531636 ) ) ;
#60110=CARTESIAN_POINT ( 'NONE',  ( -29.25216940168754931, 1.557237388845396753, 11.90587590551118424 ) ) ;
#60111=FACE_OUTER_BOUND ( 'NONE', #4286, .T. ) ;
#60119=DIRECTION ( 'NONE',  ( 1.000000000000000000, 0.000000000000000000, 0.000000000000000000 ) ) ;
#60120=DIRECTION ( 'NONE',  ( 0.000000000000000000, 0.01356324068817991828, -0.9999080150203990547 ) ) ;
#60122=CARTESIAN_POINT ( 'NONE',  ( 24.08205593069842365, 1.039322572775280618, 13.46392217257402635 ) ) ;
#60124=CARTESIAN_POINT ( 'NONE',  ( 35.00000000000000000, -7.561043153948031836, -9.557269938331533154 ) ) ;
#60126=ORIENTED_EDGE ( 'NONE', *, *, #11029, .F. ) ;
#60127=EDGE_CURVE ( 'NONE', #46634, #10568, #92, .T. ) ;
#60128=CARTESIAN_POINT ( 'NONE',  ( -15.23244606078242214, 8.473308435344804934, -8.497338976891521511 ) ) ;
#60129=VECTOR ( 'NONE', #48318, 1000.000000000000000 ) ;
#60131=DIRECTION ( 'NONE',  ( -1.000000000000000000, -1.836970198721029688E-16, -0.000000000000000000 ) ) ;
#60132=DIRECTION ( 'NONE',  ( 1.000000000000000000, 0.000000000000000000, -0.000000000000000000 ) ) ;
#60133=DIRECTION ( 'NONE',  ( 1.000000000000000000, 0.000000000000000000, -0.000000000000000000 ) ) ;
#60136=EDGE_CURVE ( 'NONE', #44008, #32797, #65574, .T. ) ;
#60138=CARTESIAN_POINT ( 'NONE',  ( 35.00000000000000000, -9.896810808925339487, 7.110831038798382409 ) ) ;
#60140=CARTESIAN_POINT ( 'NONE',  ( 12.27748271067557617, 0.5231152287652744981, 11.98862020473568002 ) ) ;
#60143=ORIENTED_EDGE ( 'NONE', *, *, #47328, .F. ) ;
#60144=CARTESIAN_POINT ( 'NONE',  ( -35.00000000000000000, 0.000000000000000000, 0.000000000000000000 ) ) ;
#60145=ORIENTED_EDGE ( 'NONE', *, *, #60890, .T. ) ;
#60146=CARTESIAN_POINT ( 'NONE',  ( -4.975205859172449507, -1.416020129149132778, 13.42553116244733680 ) ) ;
#60147=DIRECTION ( 'NONE',  ( -1.000000000000000000, 0.000000000000000000, 0.000000000000000000 ) ) ;
#60149=DIRECTION ( 'NONE',  ( -1.000000000000000000, -0.000000000000000000, 0.000000000000000000 ) ) ;
#60150=ORIENTED_EDGE ( 'NONE', *, *, #34251, .T. ) ;
#60153=ORIENTED_EDGE ( 'NONE', *, *, #62031, .T. ) ;
#60154=DIRECTION ( 'NONE',  ( 0.000000000000000000, 0.01356324068817998940, -0.9999080150203990547 ) ) ;
#60155=DIRECTION ( 'NONE',  ( 0.000000000000000000, 0.9467777615094560284, 0.3218879778916007850 ) ) ;
#60156=FACE_OUTER_BOUND ( 'NONE', #20292, .T. ) ;
#60159=DIRECTION ( 'NONE',  ( -1.000000000000000000, -0.000000000000000000, -0.000000000000000000 ) ) ;
#60161=ORIENTED_EDGE ( 'NONE', *, *, #55953, .T. ) ;
#60162=CARTESIAN_POINT ( 'NONE',  ( -37.00000000000000711, 0.000000000000000000, 0.000000000000000000 ) ) ;
#60163=ORIENTED_EDGE ( 'NONE', *, *, #209, .T. ) ;
#60164=ORIENTED_EDGE ( 'NONE', *, *, #7281, .T. ) ;
#60165=VECTOR ( 'NONE', #22991, 1000.000000000000000 ) ;
#60166=LINE ( 'NONE', #39885, #22415 ) ;
#60167=EDGE_CURVE ( 'NONE', #1326, #31517, #9662, .T. ) ;
#60169=ORIENTED_EDGE ( 'NONE', *, *, #30102, .T. ) ;
#60171=CARTESIAN_POINT ( 'NONE',  ( 35.00000000000000000, 4.545979934229410269, -11.30684963584391234 ) ) ;
#60173=DIRECTION ( 'NONE',  ( -1.000000000000000000, -0.000000000000000000, 0.000000000000000000 ) ) ;
#60174=CARTESIAN_POINT ( 'NONE',  ( -35.00000000000000000, 1.738225594539995589, 12.63095688309029541 ) ) ;
#60175=DIRECTION ( 'NONE',  ( 1.000000000000000000, 0.000000000000000000, 0.000000000000000000 ) ) ;
#60177=ORIENTED_EDGE ( 'NONE', *, *, #59260, .T. ) ;
#60179=DIRECTION ( 'NONE',  ( 1.000000000000000000, -0.000000000000000000, 0.000000000000000000 ) ) ;
#60182=ORIENTED_EDGE ( 'NONE', *, *, #29680, .T. ) ;
#60183=ORIENTED_EDGE ( 'NONE', *, *, #28156, .F. ) ;
#60184=VERTEX_POINT ( 'NONE', #22109 ) ;
#60185=DIRECTION ( 'NONE',  ( -1.000000000000000000, 0.000000000000000000, -0.000000000000000000 ) ) ;
#60186=CARTESIAN_POINT ( 'NONE',  ( -36.00000000000000711, -8.624332853796127907, 9.390600770287960586 ) ) ;
#60187=ADVANCED_FACE ( 'NONE', ( #37737 ), #53027, .T. ) ;
#60188=CARTESIAN_POINT ( 'NONE',  ( -37.00000000000000711, -11.78977382767499194, 4.245927698352017110 ) ) ;
#60189=CARTESIAN_POINT ( 'NONE',  ( -35.00000000000000000, -9.821084925794513865, -7.215058775251364409 ) ) ;
#60190=ORIENTED_EDGE ( 'NONE', *, *, #29485, .T. ) ;
#60191=DIRECTION ( 'NONE',  ( 0.000000000000000000, 0.3554799084908899509, 0.9346839223284567622 ) ) ;
#60192=( BOUNDED_CURVE ( )  B_SPLINE_CURVE ( 3, ( #23263, #12612, #28258, #32890 ),
 .UNSPECIFIED., .F., .F. ) 
 B_SPLINE_CURVE_WITH_KNOTS ( ( 4, 4 ),
 ( 1.638716093112601024, 1.675879999089879613 ),
 .UNSPECIFIED. ) 
 CURVE ( )  GEOMETRIC_REPRESENTATION_ITEM ( )  RATIONAL_B_SPLINE_CURVE ( ( 1.000000000000000000, 0.9998849069861288630, 0.9998849069861288630, 1.000000000000000000 ) ) 
 REPRESENTATION_ITEM ( '' )  );
#60193=ORIENTED_EDGE ( 'NONE', *, *, #34790, .T. ) ;
#60194=CARTESIAN_POINT ( 'NONE',  ( 0.2851083653049504285, -0.4107471485392698018, 25.00000000000000000 ) ) ;
#60195=EDGE_CURVE ( 'NONE', #49313, #7701, #57434, .T. ) ;
#60196=CARTESIAN_POINT ( 'NONE',  ( -19.42992534460779908, -4.328069792619975154, -12.78809649950834171 ) ) ;
#60197=ADVANCED_FACE ( 'NONE', ( #27419 ), #47717, .T. ) ;
#60198=ORIENTED_EDGE ( 'NONE', *, *, #52590, .T. ) ;
#60206=AXIS2_PLACEMENT_3D ( 'NONE', #13097, #53676, #32380 ) ;
#60207=ORIENTED_EDGE ( 'NONE', *, *, #33644, .T. ) ;
#60208=EDGE_CURVE ( 'NONE', #15944, #63155, #14094, .T. ) ;
#60211=CARTESIAN_POINT ( 'NONE',  ( -47.00000000000000711, 0.000000000000000000, 0.000000000000000000 ) ) ;
#60212=CARTESIAN_POINT ( 'NONE',  ( -47.00000000000000711, 0.000000000000000000, 0.000000000000000000 ) ) ;
#60213=CARTESIAN_POINT ( 'NONE',  ( -37.00000000000000711, 0.000000000000000000, 0.000000000000000000 ) ) ;
#60215=DIRECTION ( 'NONE',  ( 0.000000000000000000, 0.01356324068817992175, -0.9999080150203990547 ) ) ;
#60216=DIRECTION ( 'NONE',  ( 0.000000000000000000, -0.01356324068817992175, 0.9999080150203990547 ) ) ;
#60217=CARTESIAN_POINT ( 'NONE',  ( 35.00000000000000000, 4.705694406421931860E-17, -3.469127814946512892E-15 ) ) ;
#60220=AXIS2_PLACEMENT_3D ( 'NONE', #31147, #26164, #39559 ) ;
#60221=EDGE_CURVE ( 'NONE', #59432, #8976, #43706, .T. ) ;
#60223=ADVANCED_FACE ( 'NONE', ( #44347 ), #63987, .T. ) ;
#60224=DIRECTION ( 'NONE',  ( 0.000000000000000000, 0.4380125133593912312, -0.8989688749565187820 ) ) ;
#60226=DIRECTION ( 'NONE',  ( 0.000000000000000000, 0.01356324068818000328, -0.9999080150203990547 ) ) ;
#60227=CARTESIAN_POINT ( 'NONE',  ( -19.69476066079020171, -4.201994156881551312, -12.82938989607585789 ) ) ;
#60230=CARTESIAN_POINT ( 'NONE',  ( -30.18541646480307250, -2.218019889705987957, 11.82085758638470629 ) ) ;
#60234=CARTESIAN_POINT ( 'NONE',  ( -37.00000000000000711, 5.391785509270962784, 10.43555801961477236 ) ) ;
#60237=ORIENTED_EDGE ( 'NONE', *, *, #28228, .F. ) ;
#60238=ORIENTED_EDGE ( 'NONE', *, *, #18836, .F. ) ;
#60240=CARTESIAN_POINT ( 'NONE',  ( -2.952869152607111136, -4.384817011589735358, 11.17020052527586138 ) ) ;
#60242=EDGE_CURVE ( 'NONE', #924, #5805, #54265, .T. ) ;
#60245=CARTESIAN_POINT ( 'NONE',  ( -35.00000000000000000, 6.307491713049167004, -9.908974237959577991 ) ) ;
#60248=DIRECTION ( 'NONE',  ( 1.000000000000000000, 0.000000000000000000, -0.000000000000000000 ) ) ;
#60250=CARTESIAN_POINT ( 'NONE',  ( -4.989057617119011745, -0.9162120371760335003, 25.00000000000000000 ) ) ;
#60251=DIRECTION ( 'NONE',  ( -1.000000000000000000, -0.000000000000000000, -0.000000000000000000 ) ) ;
#60252=VERTEX_POINT ( 'NONE', #28409 ) ;
#60253=FACE_OUTER_BOUND ( 'NONE', #36707, .T. ) ;
#60254=ORIENTED_EDGE ( 'NONE', *, *, #23363, .F. ) ;
#60259=VECTOR ( 'NONE', #34089, 1000.000000000000000 ) ;
#60260=FACE_OUTER_BOUND ( 'NONE', #8822, .T. ) ;
#60261=CARTESIAN_POINT ( 'NONE',  ( 12.57979501679909440, -8.984612513102003817, -7.965368934693056069 ) ) ;
#60262=CARTESIAN_POINT ( 'NONE',  ( -35.00000000000000000, 0.000000000000000000, 0.000000000000000000 ) ) ;
#60265=LINE ( 'NONE', #50956, #34617 ) ;
#60267=CARTESIAN_POINT ( 'NONE',  ( -35.00000000000000000, 11.56998259273177787, 3.827046518385122553 ) ) ;
#60271=ORIENTED_EDGE ( 'NONE', *, *, #33644, .F. ) ;
#60272=EDGE_LOOP ( 'NONE', ( #64792, #62752, #20431, #11854 ) ) ;
#60273=CARTESIAN_POINT ( 'NONE',  ( 12.68490744323399433, -13.22581700042956498, -2.713934262790095087 ) ) ;
#60275=EDGE_CURVE ( 'NONE', #35410, #26477, #4381, .T. ) ;
#60276=VERTEX_POINT ( 'NONE', #49687 ) ;
#60282=CARTESIAN_POINT ( 'NONE',  ( -37.00000000000000711, 11.17622378668011685, -3.614449339633368119 ) ) ;
#60283=VERTEX_POINT ( 'NONE', #34044 ) ;
#60284=EDGE_CURVE ( 'NONE', #10035, #6763, #16024, .T. ) ;
#60287=CARTESIAN_POINT ( 'NONE',  ( -19.17656007471153146, -3.894919239584830439, 12.92680134493071797 ) ) ;
#60289=ORIENTED_EDGE ( 'NONE', *, *, #13, .F. ) ;
#60291=AXIS2_PLACEMENT_3D ( 'NONE', #64027, #18513, #14133 ) ;
#60292=EDGE_CURVE ( 'NONE', #44595, #36164, #2235, .T. ) ;
#60296=EDGE_CURVE ( 'NONE', #38332, #8899, #37240, .T. ) ;
#60297=CARTESIAN_POINT ( 'NONE',  ( -7.539837441135050611, -2.057183563332125154, 13.34261549860323015 ) ) ;
#60299=AXIS2_PLACEMENT_3D ( 'NONE', #45379, #20449, #10790 ) ;
#60301=DIRECTION ( 'NONE',  ( 1.000000000000000000, 0.000000000000000000, 0.000000000000000000 ) ) ;
#60303=CARTESIAN_POINT ( 'NONE',  ( 3.848109687703774817, 8.028244186201112242, 8.930321068435377541 ) ) ;
#60304=AXIS2_PLACEMENT_3D ( 'NONE', #33701, #18090, #23401 ) ;
#60306=LINE ( 'NONE', #14093, #40518 ) ;
#60307=DIRECTION ( 'NONE',  ( -1.000000000000000000, -1.836970198721029688E-16, 0.000000000000000000 ) ) ;
#60310=DIRECTION ( 'NONE',  ( 1.000000000000000000, 0.000000000000000000, 0.000000000000000000 ) ) ;
#60311=CARTESIAN_POINT ( 'NONE',  ( -36.00000000000000711, 10.68873102412852560, -6.950793414699682593 ) ) ;
#60313=CARTESIAN_POINT ( 'NONE',  ( 11.39082382910284785, 0.2412655231989612459, 13.49807518737375744 ) ) ;
#60315=ORIENTED_EDGE ( 'NONE', *, *, #47646, .F. ) ;
#60316=EDGE_LOOP ( 'NONE', ( #27228, #20274, #746, #5562 ) ) ;
#60317=ORIENTED_EDGE ( 'NONE', *, *, #7516, .T. ) ;
#60318=EDGE_CURVE ( 'NONE', #21025, #17610, #4132, .T. ) ;
#60320=DIRECTION ( 'NONE',  ( -1.000000000000000000, 0.000000000000000000, -0.000000000000000000 ) ) ;
#60321=DIRECTION ( 'NONE',  ( 1.000000000000000000, 0.000000000000000000, 0.000000000000000000 ) ) ;
#60322=DIRECTION ( 'NONE',  ( 1.000000000000000000, 0.000000000000000000, 0.000000000000000000 ) ) ;
#60323=CARTESIAN_POINT ( 'NONE',  ( -3.740102306720532788, 25.00000000000000000, -6.044082642436763742 ) ) ;
#60325=DIRECTION ( 'NONE',  ( -1.000000000000000000, 0.000000000000000000, 0.000000000000000000 ) ) ;
#60326=CARTESIAN_POINT ( 'NONE',  ( -28.85619398320021745, 3.750539801530000439, 25.00000000000000000 ) ) ;
#60327=ORIENTED_EDGE ( 'NONE', *, *, #26594, .F. ) ;
#60328=CYLINDRICAL_SURFACE ( 'NONE', #60685, 12.74999999999999822 ) ;
#60329=VERTEX_POINT ( 'NONE', #64622 ) ;
#60331=ORIENTED_EDGE ( 'NONE', *, *, #44334, .F. ) ;
#60332=EDGE_CURVE ( 'NONE', #22711, #9287, #52122, .T. ) ;
#60333=ORIENTED_EDGE ( 'NONE', *, *, #51322, .T. ) ;
#60339=DIRECTION ( 'NONE',  ( 1.000000000000000000, 0.000000000000000000, 0.000000000000000000 ) ) ;
#60341=VERTEX_POINT ( 'NONE', #53704 ) ;
#60342=AXIS2_PLACEMENT_3D ( 'NONE', #40365, #40044, #55016 ) ;
#60344=FACE_OUTER_BOUND ( 'NONE', #22321, .T. ) ;
#60345=VERTEX_POINT ( 'NONE', #34384 ) ;
#60347=EDGE_LOOP ( 'NONE', ( #3715, #3769, #21084, #11478 ) ) ;
#60348=CARTESIAN_POINT ( 'NONE',  ( 35.00000000000000000, 1.262958560998929558, 12.12087942037208066 ) ) ;
#60349=AXIS2_PLACEMENT_3D ( 'NONE', #44819, #34817, #49820 ) ;
#60351=CARTESIAN_POINT ( 'NONE',  ( 17.10287315442671030, -9.289536693978741155, 7.615149052798787288 ) ) ;
#60352=EDGE_CURVE ( 'NONE', #58929, #30664, #23440, .T. ) ;
#60354=CARTESIAN_POINT ( 'NONE',  ( -10.87643784907710298, -4.898157848850412499, -10.96305477394234273 ) ) ;
#60355=DIRECTION ( 'NONE',  ( 1.000000000000000000, -0.000000000000000000, 0.000000000000000000 ) ) ;
#60356=ORIENTED_EDGE ( 'NONE', *, *, #51785, .F. ) ;
#60359=FACE_OUTER_BOUND ( 'NONE', #5393, .T. ) ;
#60360=DIRECTION ( 'NONE',  ( 0.000000000000000000, -0.01356324068817998940, 0.9999080150203990547 ) ) ;
#60362=CARTESIAN_POINT ( 'NONE',  ( -35.00000000000000000, -11.50504120060940316, -4.018060380616521599 ) ) ;
#60364=CARTESIAN_POINT ( 'NONE',  ( 37.00000000000000711, 4.705694406421931860E-17, -3.469127814946512892E-15 ) ) ;
#60365=ADVANCED_FACE ( 'NONE', ( #10744 ), #50998, .T. ) ;
#60366=CIRCLE ( 'NONE', #34859, 12.18649999999999878 ) ;
#60367=CARTESIAN_POINT ( 'NONE',  ( 6.812204945636112896, -4.138731716409435712, -12.84993773446340803 ) ) ;
#60369=EDGE_CURVE ( 'NONE', #15685, #6304, #11750, .T. ) ;
#60371=EDGE_LOOP ( 'NONE', ( #13942, #18686, #20618, #52779 ) ) ;
#60374=DIRECTION ( 'NONE',  ( 1.000000000000000000, 0.000000000000000000, -0.000000000000000000 ) ) ;
#60375=AXIS2_PLACEMENT_3D ( 'NONE', #12380, #32650, #9276 ) ;
#60378=CARTESIAN_POINT ( 'NONE',  ( 35.00000000000000000, 7.146664589317909488, -9.321877890560465119 ) ) ;
#60382=VERTEX_POINT ( 'NONE', #45667 ) ;
#60384=CARTESIAN_POINT ( 'NONE',  ( 27.08585833250204900, 12.95103964514429684, 3.823327208526503984 ) ) ;
#60386=ORIENTED_EDGE ( 'NONE', *, *, #36424, .T. ) ;
#60387=VECTOR ( 'NONE', #57260, 1000.000000000000000 ) ;
#60389=CYLINDRICAL_SURFACE ( 'NONE', #1309, 12.74999999999999822 ) ;
#60393=CARTESIAN_POINT ( 'NONE',  ( -14.23149639848878678, 7.941839253138341270, 8.998400932456021906 ) ) ;
#60394=CARTESIAN_POINT ( 'NONE',  ( 37.00000000000000711, -10.02106554660713833, -7.882940143791743459 ) ) ;
#60396=DIRECTION ( 'NONE',  ( -1.000000000000000000, 0.000000000000000000, 0.000000000000000000 ) ) ;
#60398=DIRECTION ( 'NONE',  ( -1.000000000000000000, -0.000000000000000000, 0.000000000000000000 ) ) ;
#60399=CARTESIAN_POINT ( 'NONE',  ( -14.37821012703996892, 8.339393263347453455, -10.61631806211926587 ) ) ;
#60400=DIRECTION ( 'NONE',  ( 1.000000000000000000, 0.000000000000000000, 0.000000000000000000 ) ) ;
#60401=FACE_OUTER_BOUND ( 'NONE', #63823, .T. ) ;
#60403=CYLINDRICAL_SURFACE ( 'NONE', #55695, 5.000000000000000888 ) ;
#60404=DIRECTION ( 'NONE',  ( 0.000000000000000000, -0.8515178078024813191, 0.5243256840888652626 ) ) ;
#60405=ORIENTED_EDGE ( 'NONE', *, *, #31424, .T. ) ;
#60406=ORIENTED_EDGE ( 'NONE', *, *, #17020, .F. ) ;
#60408=EDGE_LOOP ( 'NONE', ( #65771, #19650, #3022, #61635 ) ) ;
#60412=CIRCLE ( 'NONE', #49842, 12.74999999999999822 ) ;
#60414=VERTEX_POINT ( 'NONE', #40019 ) ;
#60415=CARTESIAN_POINT ( 'NONE',  ( 37.00000000000000711, -5.246972444133939817, 10.99909370905162298 ) ) ;
#60416=CARTESIAN_POINT ( 'NONE',  ( 10.88441259213023393, 11.89247429979993242, -1.605920490876132867 ) ) ;
#60418=DIRECTION ( 'NONE',  ( -1.000000000000000000, -0.000000000000000000, 0.000000000000000000 ) ) ;
#60420=ORIENTED_EDGE ( 'NONE', *, *, #269, .F. ) ;
#60422=EDGE_CURVE ( 'NONE', #30330, #47727, #3340, .T. ) ;
#60423=EDGE_CURVE ( 'NONE', #7557, #24932, #29882, .T. ) ;
#60424=ORIENTED_EDGE ( 'NONE', *, *, #28499, .T. ) ;
#60426=ORIENTED_EDGE ( 'NONE', *, *, #26044, .F. ) ;
#60428=AXIS2_PLACEMENT_3D ( 'NONE', #27852, #2616, #43129 ) ;
#60430=CARTESIAN_POINT ( 'NONE',  ( -29.68541646480307605, -1.201201861335963628, 11.94168801375079703 ) ) ;
#60431=CIRCLE ( 'NONE', #31744, 5.000000000000000000 ) ;
#60434=CARTESIAN_POINT ( 'NONE',  ( 35.00000000000000000, 10.25474254703961918, 6.584150480049438592 ) ) ;
#60435=ORIENTED_EDGE ( 'NONE', *, *, #34238, .F. ) ;
#60437=DIRECTION ( 'NONE',  ( 0.000000000000000000, 0.01356324068817992175, -0.9999080150203990547 ) ) ;
#60439=CARTESIAN_POINT ( 'NONE',  ( 12.73595680732062085, 12.88342186531470546, -4.037885783516507843 ) ) ;
#60442=LINE ( 'NONE', #25196, #15349 ) ;
#60444=EDGE_CURVE ( 'NONE', #14488, #37865, #24577, .T. ) ;
#60445=VERTEX_POINT ( 'NONE', #470 ) ;
#60446=CARTESIAN_POINT ( 'NONE',  ( -17.49774675589618411, 7.618938804295157574, -9.273320750912958488 ) ) ;
#60447=EDGE_CURVE ( 'NONE', #46217, #51182, #21181, .T. ) ;
#60449=CARTESIAN_POINT ( 'NONE',  ( 35.00000000000000000, -1.030638227056475120, 12.14284015767850811 ) ) ;
#60451=CARTESIAN_POINT ( 'NONE',  ( -18.08686583997217667, 5.372364593331139915, -12.38728941600954769 ) ) ;
#60452=CARTESIAN_POINT ( 'NONE',  ( 35.00000000000000000, 9.557269938331552694, -7.561043153948004303 ) ) ;
#60455=CARTESIAN_POINT ( 'NONE',  ( -35.00000000000000000, -10.02106554660702820, -7.882940143791882903 ) ) ;
#60457=CARTESIAN_POINT ( 'NONE',  ( 35.00000000000000000, 4.705694406421931860E-17, -3.469127814946512892E-15 ) ) ;
#60458=CARTESIAN_POINT ( 'NONE',  ( 47.00000000000000711, 4.705694406421931860E-17, -3.469127814946512892E-15 ) ) ;
#60460=CARTESIAN_POINT ( 'NONE',  ( -18.87003134133906102, -4.090855072109758517, 11.28365501786238490 ) ) ;
#60465=ORIENTED_EDGE ( 'NONE', *, *, #1512, .T. ) ;
#60468=CARTESIAN_POINT ( 'NONE',  ( -37.00000000000000711, 0.000000000000000000, -1.750000000000000000 ) ) ;
#60471=ORIENTED_EDGE ( 'NONE', *, *, #8980, .T. ) ;
#60473=ORIENTED_EDGE ( 'NONE', *, *, #39388, .T. ) ;
#60474=AXIS2_PLACEMENT_3D ( 'NONE', #25729, #5124, #46020 ) ;
#60477=CYLINDRICAL_SURFACE ( 'NONE', #3502, 4.999999999999999112 ) ;
#60479=CARTESIAN_POINT ( 'NONE',  ( 35.00000000000000000, -11.16627499335657703, -3.645068577059991988 ) ) ;
#60482=DIRECTION ( 'NONE',  ( 0.000000000000000000, -0.01356324068817998073, 0.9999080150203990547 ) ) ;
#60483=ORIENTED_EDGE ( 'NONE', *, *, #25601, .F. ) ;
#60485=ORIENTED_EDGE ( 'NONE', *, *, #31911, .T. ) ;
#60486=VECTOR ( 'NONE', #63512, 1000.000000000000000 ) ;
#60487=ORIENTED_EDGE ( 'NONE', *, *, #23547, .T. ) ;
#60488=DIRECTION ( 'NONE',  ( 0.000000000000000000, 0.04924826701373889726, 0.9987865678893281807 ) ) ;
#60490=EDGE_CURVE ( 'NONE', #35533, #36952, #56654, .T. ) ;
#60491=ORIENTED_EDGE ( 'NONE', *, *, #5447, .T. ) ;
#60492=DIRECTION ( 'NONE',  ( 1.000000000000000000, -0.000000000000000000, 0.000000000000000000 ) ) ;
#60493=ORIENTED_EDGE ( 'NONE', *, *, #9920, .F. ) ;
#60494=CARTESIAN_POINT ( 'NONE',  ( 36.00000000000000711, 1.286231064351314624, -12.68495603654572257 ) ) ;
#60496=CARTESIAN_POINT ( 'NONE',  ( 35.00000000000000000, -11.72397916322011824, 0.7214809346829776926 ) ) ;
#60497=CARTESIAN_POINT ( 'NONE',  ( 4.365482547053908924, -10.79959492482372241, 5.234344269312817488 ) ) ;
#60498=ORIENTED_EDGE ( 'NONE', *, *, #55475, .T. ) ;
#60501=VERTEX_POINT ( 'NONE', #46653 ) ;
#60503=ADVANCED_FACE ( 'NONE', ( #12372 ), #62581, .T. ) ;
#60504=DIRECTION ( 'NONE',  ( -1.000000000000000000, 0.000000000000000000, -0.000000000000000000 ) ) ;
#60505=ORIENTED_EDGE ( 'NONE', *, *, #47778, .F. ) ;
#60506=VERTEX_POINT ( 'NONE', #52647 ) ;
#60510=AXIS2_PLACEMENT_3D ( 'NONE', #13036, #27333, #18372 ) ;
#60511=CARTESIAN_POINT ( 'NONE',  ( 35.00000000000000000, 4.705694406421931860E-17, -3.469127814946512892E-15 ) ) ;
#60512=AXIS2_PLACEMENT_3D ( 'NONE', #63150, #27566, #6657 ) ;
#60513=CYLINDRICAL_SURFACE ( 'NONE', #46821, 7.115568257478080305 ) ;
#60515=VERTEX_POINT ( 'NONE', #26700 ) ;
#60517=VERTEX_POINT ( 'NONE', #1107 ) ;
#60518=AXIS2_PLACEMENT_3D ( 'NONE', #2063, #37959, #22327 ) ;
#60519=FACE_OUTER_BOUND ( 'NONE', #4208, .T. ) ;
#60520=CARTESIAN_POINT ( 'NONE',  ( 35.00000000000000000, 4.705694406421931860E-17, -3.469127814946512892E-15 ) ) ;
#60523=CARTESIAN_POINT ( 'NONE',  ( 26.83124887464803976, 11.22347478894700679, 4.259285346550930385 ) ) ;
#60525=CIRCLE ( 'NONE', #46761, 12.74999999999999822 ) ;
#60526=VERTEX_POINT ( 'NONE', #47638 ) ;
#60527=DIRECTION ( 'NONE',  ( 1.000000000000000000, 0.000000000000000000, -0.000000000000000000 ) ) ;
#60528=AXIS2_PLACEMENT_3D ( 'NONE', #22124, #47732, #62675 ) ;
#60529=ORIENTED_EDGE ( 'NONE', *, *, #59917, .F. ) ;
#60530=CARTESIAN_POINT ( 'NONE',  ( -10.64440273086534816, -9.782391350870085489, -6.950960968970274934 ) ) ;
#60531=DIRECTION ( 'NONE',  ( 0.000000000000000000, 0.2960891610144441022, 0.9551603052523501836 ) ) ;
#60533=CYLINDRICAL_SURFACE ( 'NONE', #20285, 12.18650000000000055 ) ;
#60534=CARTESIAN_POINT ( 'NONE',  ( 13.41118187415329643, 10.79912113741252178, -5.237416537976061548 ) ) ;
#60537=CYLINDRICAL_SURFACE ( 'NONE', #38783, 4.999999999999999112 ) ;
#60538=CARTESIAN_POINT ( 'NONE',  ( 36.00000000000000711, -12.68495603654572612, -1.286231064351273989 ) ) ;
#60539=CIRCLE ( 'NONE', #48839, 4.999999999999999112 ) ;
#60542=EDGE_CURVE ( 'NONE', #27686, #62900, #50078, .T. ) ;
#60545=CARTESIAN_POINT ( 'NONE',  ( -7.489022030332961322, -5.127957880411574187, -10.84914964302385521 ) ) ;
#60548=EDGE_CURVE ( 'NONE', #62086, #7910, #46901, .T. ) ;
#60549=VECTOR ( 'NONE', #51721, 1000.000000000000000 ) ;
#60552=EDGE_CURVE ( 'NONE', #61981, #21190, #38384, .T. ) ;
#60553=EDGE_LOOP ( 'NONE', ( #61256, #32810, #45151, #54031 ) ) ;
#60554=DIRECTION ( 'NONE',  ( -0.9748757316300199482, 0.000000000000000000, 0.2227494284590502138 ) ) ;
#60559=EDGE_CURVE ( 'NONE', #56061, #15944, #53710, .T. ) ;
#60560=ORIENTED_EDGE ( 'NONE', *, *, #4631, .T. ) ;
#60561=ORIENTED_EDGE ( 'NONE', *, *, #64246, .T. ) ;
#60563=CARTESIAN_POINT ( 'NONE',  ( 28.90977330190072792, -10.36490708579996678, 6.051299003903356954 ) ) ;
#60564=AXIS2_PLACEMENT_3D ( 'NONE', #58304, #57318, #22380 ) ;
#60565=FACE_OUTER_BOUND ( 'NONE', #51991, .T. ) ;
#60566=EDGE_CURVE ( 'NONE', #49238, #4915, #51369, .T. ) ;
#60567=ORIENTED_EDGE ( 'NONE', *, *, #22048, .F. ) ;
#60572=EDGE_LOOP ( 'NONE', ( #65398, #31305, #24298, #15766 ) ) ;
#60580=DIRECTION ( 'NONE',  ( -1.000000000000000000, 0.000000000000000000, -0.000000000000000000 ) ) ;
#60581=VERTEX_POINT ( 'NONE', #30223 ) ;
#60583=AXIS2_PLACEMENT_3D ( 'NONE', #1067, #7032, #21336 ) ;
#60586=DIRECTION ( 'NONE',  ( -1.000000000000000000, 0.000000000000000000, 0.000000000000000000 ) ) ;
#60587=DIRECTION ( 'NONE',  ( 0.000000000000000000, 0.01356324068817300540, -0.9999080150203989437 ) ) ;
#60589=CARTESIAN_POINT ( 'NONE',  ( 35.00000000000000000, -2.250029553613672295, 12.54989509947652770 ) ) ;
#60590=FACE_OUTER_BOUND ( 'NONE', #3634, .T. ) ;
#60591=B_SPLINE_CURVE_WITH_KNOTS ( 'NONE', 3,
 ( #20795, #35420, #20135, #5859, #51065, #45087, #41063, #35073, #46080, #40402, #24805, #40746, #50733, #41383, #10471, #40076, #61340, #46392, #20470, #30748, #840, #55726, #10157, #19817 ),
 .UNSPECIFIED., .F., .F.,
 ( 4, 2, 2, 2, 2, 2, 2, 2, 2, 2, 2, 4 ),
 ( 2.602085213965210642E-18, 0.001217752653192586071, 0.001826628979788878782, 0.002435505306385171709, 0.003044381632981464636, 0.003653257959577757129, 0.004871010612770343418, 0.006088763265962928405, 0.007306515919155514259, 0.008524268572348100981, 0.009133144898944393908, 0.009742021225540686835 ),
 .UNSPECIFIED. ) ;
#60592=CARTESIAN_POINT ( 'NONE',  ( 12.19547418290646590, 0.02891602860409012848, 11.99999999999999467 ) ) ;
#60593=DIRECTION ( 'NONE',  ( 0.000000000000000000, 0.01356324068817998767, -0.9999080150203990547 ) ) ;
#60595=CARTESIAN_POINT ( 'NONE',  ( 4.884421565153296285, -10.53113076414237703, 8.448016786630551778 ) ) ;
#60596=ORIENTED_EDGE ( 'NONE', *, *, #24083, .F. ) ;
#60597=B_SPLINE_CURVE_WITH_KNOTS ( 'NONE', 3,
 ( #3906, #49139, #59414, #3598, #18211, #39449, #34131, #38479, #64709, #23864 ),
 .UNSPECIFIED., .F., .F.,
 ( 4, 2, 2, 2, 4 ),
 ( 1.163687884334659274E-17, 0.002301662762293088353, 0.004603325524586164563, 0.006904988286879240773, 0.009206651049172318718 ),
 .UNSPECIFIED. ) ;
#60599=CARTESIAN_POINT ( 'NONE',  ( 36.00000000000000711, -12.08151691381187298, 4.074242145636130630 ) ) ;
#60602=CARTESIAN_POINT ( 'NONE',  ( 12.89830783111085566, -13.14232582968774388, -3.093048059426170227 ) ) ;
#60605=DIRECTION ( 'NONE',  ( -1.000000000000000000, -0.000000000000000000, 0.000000000000000000 ) ) ;
#60606=DIRECTION ( 'NONE',  ( 0.000000000000000000, 0.01356324068817991828, -0.9999080150203990547 ) ) ;
#60611=AXIS2_PLACEMENT_3D ( 'NONE', #36237, #365, #35899 ) ;
#60612=AXIS2_PLACEMENT_3D ( 'NONE', #49474, #7924, #38490 ) ;
#60613=PLANE ( 'NONE',  #18389 ) ;
#60615=ORIENTED_EDGE ( 'NONE', *, *, #61996, .T. ) ;
#60617=FACE_OUTER_BOUND ( 'NONE', #20867, .T. ) ;
#60619=ORIENTED_EDGE ( 'NONE', *, *, #48074, .T. ) ;
#60623=CARTESIAN_POINT ( 'NONE',  ( -35.00000000000000000, -3.511814412392038953, -11.66953048682403171 ) ) ;
#60624=AXIS2_PLACEMENT_3D ( 'NONE', #8744, #63269, #64568 ) ;
#60625=CARTESIAN_POINT ( 'NONE',  ( -10.82482511535300773, -8.491786248805359705, -10.49748912556531621 ) ) ;
#60628=DIRECTION ( 'NONE',  ( 1.000000000000000000, -0.000000000000000000, 0.000000000000000000 ) ) ;
#60630=CARTESIAN_POINT ( 'NONE',  ( -37.00000000000000711, -12.21925492305359562, -3.640372113593682624 ) ) ;
#60635=AXIS2_PLACEMENT_3D ( 'NONE', #63854, #43921, #34892 ) ;
#60636=ORIENTED_EDGE ( 'NONE', *, *, #26282, .T. ) ;
#60637=EDGE_CURVE ( 'NONE', #59860, #23486, #7592, .T. ) ;
#60639=CARTESIAN_POINT ( 'NONE',  ( 3.145174248154654517, 4.348535253017615787, -11.19168307967391129 ) ) ;
#60640=CARTESIAN_POINT ( 'NONE',  ( 37.00000000000000711, 4.705694406421931860E-17, -3.469127814946512892E-15 ) ) ;
#60641=ORIENTED_EDGE ( 'NONE', *, *, #59913, .T. ) ;
#60642=FACE_OUTER_BOUND ( 'NONE', #64516, .T. ) ;
#60643=CIRCLE ( 'NONE', #12843, 12.18650000000000411 ) ;
#60644=PLANE ( 'NONE',  #22428 ) ;
#60649=CIRCLE ( 'NONE', #8691, 4.999999999999999112 ) ;
#60650=CIRCLE ( 'NONE', #37296, 5.000000000000000888 ) ;
#60651=CIRCLE ( 'NONE', #55334, 12.18649999999999878 ) ;
#60653=CARTESIAN_POINT ( 'NONE',  ( -37.00000000000000711, 0.000000000000000000, 0.000000000000000000 ) ) ;
#60657=DIRECTION ( 'NONE',  ( -1.000000000000000000, 0.000000000000000000, 0.000000000000000000 ) ) ;
#60658=EDGE_CURVE ( 'NONE', #14915, #40547, #24576, .T. ) ;
#60660=B_SPLINE_CURVE_WITH_KNOTS ( 'NONE', 3,
 ( #31438, #36073, #1532, #16790, #57049, #16146, #27110, #26129, #11470, #51737, #21120, #26443, #16484, #12130, #32076, #36753, #57368, #31746 ),
 .UNSPECIFIED., .F., .F.,
 ( 4, 2, 2, 2, 2, 2, 2, 2, 4 ),
 ( 0.000000000000000000, 0.0007405344560050070241, 0.001481068912010014048, 0.002221603368015021181, 0.002962137824020028096, 0.003702672280025034578, 0.004443206736030042361, 0.005183741192035048843, 0.005924275648040054458 ),
 .UNSPECIFIED. ) ;
#60662=DIRECTION ( 'NONE',  ( 0.000000000000000000, -0.7196168960969868689, -0.6943713148249562872 ) ) ;
#60664=DIRECTION ( 'NONE',  ( 0.000000000000000000, 0.01356324068817998940, -0.9999080150203990547 ) ) ;
#60667=DIRECTION ( 'NONE',  ( -1.000000000000000000, 0.000000000000000000, 0.000000000000000000 ) ) ;
#60668=ORIENTED_EDGE ( 'NONE', *, *, #22969, .F. ) ;
#60669=EDGE_LOOP ( 'NONE', ( #60315, #26834, #42992, #34151 ) ) ;
#60671=EDGE_CURVE ( 'NONE', #52324, #53488, #52233, .T. ) ;
#60672=VECTOR ( 'NONE', #54724, 1000.000000000000000 ) ;
#60675=CIRCLE ( 'NONE', #51148, 12.18650000000000055 ) ;
#60677=FACE_OUTER_BOUND ( 'NONE', #39467, .T. ) ;
#60678=CYLINDRICAL_SURFACE ( 'NONE', #158, 12.75000000000000178 ) ;
#60679=CIRCLE ( 'NONE', #52242, 12.18650000000000411 ) ;
#60680=ADVANCED_FACE ( 'NONE', ( #65765 ), #44203, .T. ) ;
#60681=ORIENTED_EDGE ( 'NONE', *, *, #35720, .T. ) ;
#60682=EDGE_LOOP ( 'NONE', ( #39141, #38852, #20991, #23295 ) ) ;
#60684=ORIENTED_EDGE ( 'NONE', *, *, #29698, .F. ) ;
#60685=AXIS2_PLACEMENT_3D ( 'NONE', #25752, #45047, #40042 ) ;
#60687=ORIENTED_EDGE ( 'NONE', *, *, #27301, .F. ) ;
#60690=DIRECTION ( 'NONE',  ( 1.000000000000000000, 0.000000000000000000, 0.000000000000000000 ) ) ;
#60692=CARTESIAN_POINT ( 'NONE',  ( 17.87656210312829330, -6.543550415627087169, 10.06239431139154306 ) ) ;
#60696=AXIS2_PLACEMENT_3D ( 'NONE', #19560, #14528, #28222 ) ;
#60697=EDGE_LOOP ( 'NONE', ( #31328, #29564, #43895, #38853 ) ) ;
#60698=ORIENTED_EDGE ( 'NONE', *, *, #19755, .F. ) ;
#60700=CIRCLE ( 'NONE', #49043, 12.18650000000000411 ) ;
#60701=CARTESIAN_POINT ( 'NONE',  ( 10.48620311856346454, 8.250315036047107142, -10.68561190601526789 ) ) ;
#60704=ADVANCED_FACE ( 'NONE', ( #29880 ), #50192, .T. ) ;
#60705=AXIS2_PLACEMENT_3D ( 'NONE', #27303, #12339, #32604 ) ;
#60706=CARTESIAN_POINT ( 'NONE',  ( 35.00000000000000000, 7.474872387601131152, 9.060822531525964507 ) ) ;
#60707=AXIS2_PLACEMENT_3D ( 'NONE', #40018, #54989, #59665 ) ;
#60709=FACE_OUTER_BOUND ( 'NONE', #38248, .T. ) ;
#60710=CYLINDRICAL_SURFACE ( 'NONE', #42830, 13.50000000000000178 ) ;
#60712=ORIENTED_EDGE ( 'NONE', *, *, #14998, .F. ) ;
#60713=DIRECTION ( 'NONE',  ( 1.000000000000000000, 0.000000000000000000, 0.000000000000000000 ) ) ;
#60715=EDGE_CURVE ( 'NONE', #12171, #52971, #19270, .T. ) ;
#60718=AXIS2_PLACEMENT_3D ( 'NONE', #4464, #40329, #54681 ) ;
#60719=DIRECTION ( 'NONE',  ( 1.000000000000000000, -0.000000000000000000, 0.000000000000000000 ) ) ;
#60721=ORIENTED_EDGE ( 'NONE', *, *, #30960, .F. ) ;
#60725=ORIENTED_EDGE ( 'NONE', *, *, #5435, .F. ) ;
#60726=DIRECTION ( 'NONE',  ( -1.000000000000000000, 0.000000000000000000, -0.000000000000000000 ) ) ;
#60727=CARTESIAN_POINT ( 'NONE',  ( 35.00000000000000000, 12.02534193257720574, -4.237174932027271801 ) ) ;
#60729=EDGE_CURVE ( 'NONE', #23899, #11586, #31524, .T. ) ;
#60730=CIRCLE ( 'NONE', #32049, 12.18650000000000055 ) ;
#60731=CYLINDRICAL_SURFACE ( 'NONE', #27533, 5.000000000000000888 ) ;
#60732=ORIENTED_EDGE ( 'NONE', *, *, #43881, .T. ) ;
#60735=VERTEX_POINT ( 'NONE', #15249 ) ;
#60736=CIRCLE ( 'NONE', #40565, 4.999999999999999112 ) ;
#60737=CARTESIAN_POINT ( 'NONE',  ( -9.327891528110853869, 11.85922960855886821, -6.460470496795954531 ) ) ;
#60738=DIRECTION ( 'NONE',  ( 1.000000000000000000, 0.000000000000000000, 0.000000000000000000 ) ) ;
#60739=DIRECTION ( 'NONE',  ( 0.000000000000000000, -0.3554799084909036067, -0.9346839223284515441 ) ) ;
#60742=FACE_OUTER_BOUND ( 'NONE', #34959, .T. ) ;
#60743=ORIENTED_EDGE ( 'NONE', *, *, #5380, .F. ) ;
#60744=CARTESIAN_POINT ( 'NONE',  ( 35.00000000000000000, -11.66953048682396954, 3.511814412392239682 ) ) ;
#60745=ORIENTED_EDGE ( 'NONE', *, *, #53079, .T. ) ;
#60746=CIRCLE ( 'NONE', #10855, 12.74999999999999822 ) ;
#60748=EDGE_CURVE ( 'NONE', #31515, #64802, #44988, .T. ) ;
#60749=AXIS2_PLACEMENT_3D ( 'NONE', #53040, #27122, #63651 ) ;
#60751=CIRCLE ( 'NONE', #52129, 12.75000000000000178 ) ;
#60752=CIRCLE ( 'NONE', #20401, 5.000000000000001776 ) ;
#60753=ADVANCED_FACE ( 'NONE', ( #25899 ), #52154, .T. ) ;
#60755=ORIENTED_EDGE ( 'NONE', *, *, #12459, .F. ) ;
#60757=DIRECTION ( 'NONE',  ( 0.000000000000000000, 0.4698238015817365332, 0.8827602140260315533 ) ) ;
#60760=VERTEX_POINT ( 'NONE', #45847 ) ;
#60763=VERTEX_POINT ( 'NONE', #16576 ) ;
#60766=AXIS2_PLACEMENT_3D ( 'NONE', #40798, #878, #34788 ) ;
#60767=DIRECTION ( 'NONE',  ( 1.000000000000000000, 0.000000000000000000, 0.000000000000000000 ) ) ;
#60768=LINE ( 'NONE', #55112, #13542 ) ;
#60769=AXIS2_PLACEMENT_3D ( 'NONE', #54917, #35921, #40264 ) ;
#60770=CARTESIAN_POINT ( 'NONE',  ( 35.00000000000000000, 12.08216339958902630, 1.591260454995109930 ) ) ;
#60771=CARTESIAN_POINT ( 'NONE',  ( -35.00000000000000000, -7.561043153947899498, -9.557269938331636183 ) ) ;
#60773=ORIENTED_EDGE ( 'NONE', *, *, #21816, .F. ) ;
#60776=CARTESIAN_POINT ( 'NONE',  ( 21.94281256157706750, 11.68886982501328475, -2.741018260906308068 ) ) ;
#60777=CARTESIAN_POINT ( 'NONE',  ( 9.772170780982303739, 13.45371974242435442, -1.117788476161230227 ) ) ;
#60778=PLANE ( 'NONE',  #46706 ) ;
#60779=CARTESIAN_POINT ( 'NONE',  ( 37.00000000000000711, 8.017674001891784030, -9.913596905230145140 ) ) ;
#60780=DIRECTION ( 'NONE',  ( 0.000000000000000000, 0.2960891610144441022, 0.9551603052523501836 ) ) ;
#60781=FACE_OUTER_BOUND ( 'NONE', #28125, .T. ) ;
#60782=EDGE_CURVE ( 'NONE', #21703, #54954, #5470, .T. ) ;
#60784=CARTESIAN_POINT ( 'NONE',  ( 35.00000000000000000, 11.80185301892980299, -4.824807283154166626 ) ) ;
#60785=AXIS2_PLACEMENT_3D ( 'NONE', #27819, #47459, #53089 ) ;
#60786=EDGE_CURVE ( 'NONE', #6776, #40631, #56429, .T. ) ;
#60788=VERTEX_POINT ( 'NONE', #36843 ) ;
#60789=FACE_OUTER_BOUND ( 'NONE', #53727, .T. ) ;
#60791=CARTESIAN_POINT ( 'NONE',  ( -17.29753452029093097, 7.115740787999835781, -11.47405852577958107 ) ) ;
#60793=CARTESIAN_POINT ( 'NONE',  ( -37.00000000000000711, -10.43555801961479190, 5.391785509270926369 ) ) ;
#60795=DIRECTION ( 'NONE',  ( 1.000000000000000000, 0.000000000000000000, 0.000000000000000000 ) ) ;
#60797=ADVANCED_FACE ( 'NONE', ( #21893 ), #40859, .T. ) ;
#60799=DIRECTION ( 'NONE',  ( 0.000000000000000000, 0.01356324068817992175, -0.9999080150203990547 ) ) ;
#60801=AXIS2_PLACEMENT_3D ( 'NONE', #28902, #43523, #29234 ) ;
#60802=CARTESIAN_POINT ( 'NONE',  ( 9.773978258136098773, 6.946402228990928407, -11.57921718125522581 ) ) ;
#60804=ORIENTED_EDGE ( 'NONE', *, *, #57073, .T. ) ;
#60807=FACE_OUTER_BOUND ( 'NONE', #16601, .T. ) ;
#60810=CARTESIAN_POINT ( 'NONE',  ( 29.12753374973488363, -5.698473394425191074, 10.60092621982456862 ) ) ;
#60812=DIRECTION ( 'NONE',  ( -1.000000000000000000, 0.000000000000000000, 0.000000000000000000 ) ) ;
#60813=CIRCLE ( 'NONE', #54468, 5.000000000000001776 ) ;
#60814=VERTEX_POINT ( 'NONE', #37500 ) ;
#60816=CARTESIAN_POINT ( 'NONE',  ( 22.57855258442564761, -4.427776684447072952, 25.00000000000000000 ) ) ;
#60821=CYLINDRICAL_SURFACE ( 'NONE', #46894, 4.999999999999999112 ) ;
#60822=DIRECTION ( 'NONE',  ( 1.000000000000000000, 0.000000000000000000, 0.000000000000000000 ) ) ;
#60825=DIRECTION ( 'NONE',  ( -1.000000000000000000, 0.000000000000000000, 0.000000000000000000 ) ) ;
#60828=ORIENTED_EDGE ( 'NONE', *, *, #1831, .F. ) ;
#60829=CARTESIAN_POINT ( 'NONE',  ( 37.00000000000000711, 10.25474254703961918, 6.584150480049438592 ) ) ;
#60830=ADVANCED_FACE ( 'NONE', ( #57470 ), #16889, .T. ) ;
#60832=ORIENTED_EDGE ( 'NONE', *, *, #20847, .T. ) ;
#60834=FACE_BOUND ( 'NONE', #12808, .T. ) ;
#60835=EDGE_LOOP ( 'NONE', ( #8108, #4251, #52883, #16211 ) ) ;
#60836=CARTESIAN_POINT ( 'NONE',  ( -37.00000000000000711, 9.506317355798371338, 8.496612874013196759 ) ) ;
#60837=DIRECTION ( 'NONE',  ( 1.000000000000000000, 0.000000000000000000, 0.000000000000000000 ) ) ;
#60840=ORIENTED_EDGE ( 'NONE', *, *, #58103, .F. ) ;
#60841=ORIENTED_EDGE ( 'NONE', *, *, #62318, .T. ) ;
#60843=ORIENTED_EDGE ( 'NONE', *, *, #56534, .F. ) ;
#60845=ORIENTED_EDGE ( 'NONE', *, *, #60871, .T. ) ;
#60846=CIRCLE ( 'NONE', #47086, 12.18650000000000055 ) ;
#60848=AXIS2_PLACEMENT_3D ( 'NONE', #4583, #39810, #51457 ) ;
#60849=ORIENTED_EDGE ( 'NONE', *, *, #40224, .T. ) ;
#60850=VERTEX_POINT ( 'NONE', #37831 ) ;
#60853=AXIS2_PLACEMENT_3D ( 'NONE', #62741, #52476, #36153 ) ;
#60854=CIRCLE ( 'NONE', #1438, 5.000000000000000000 ) ;
#60855=DIRECTION ( 'NONE',  ( 1.000000000000000000, 0.000000000000000000, 0.000000000000000000 ) ) ;
#60856=CARTESIAN_POINT ( 'NONE',  ( -37.00000000000000711, 0.000000000000000000, 0.000000000000000000 ) ) ;
#60858=ORIENTED_EDGE ( 'NONE', *, *, #2552, .T. ) ;
#60859=DIRECTION ( 'NONE',  ( 1.000000000000000000, 0.000000000000000000, 0.000000000000000000 ) ) ;
#60860=ORIENTED_EDGE ( 'NONE', *, *, #28150, .T. ) ;
#60861=DIRECTION ( 'NONE',  ( 1.000000000000000000, -0.000000000000000000, -0.000000000000000000 ) ) ;
#60862=CIRCLE ( 'NONE', #13106, 5.000000000000001776 ) ;
#60864=VERTEX_POINT ( 'NONE', #37158 ) ;
#60865=CARTESIAN_POINT ( 'NONE',  ( -27.23368049396187374, 11.01758315594069870, -7.819524286938179358 ) ) ;
#60866=VECTOR ( 'NONE', #36246, 1000.000000000000000 ) ;
#60867=CARTESIAN_POINT ( 'NONE',  ( 29.16097531476821203, 8.613045793590645260, 8.368184035611974991 ) ) ;
#60868=DIRECTION ( 'NONE',  ( 0.6442147435043042991, 0.000000000000000000, 0.7648446667472313942 ) ) ;
#60869=VERTEX_POINT ( 'NONE', #63733 ) ;
#60870=CARTESIAN_POINT ( 'NONE',  ( -35.00000000000000000, 7.971186206369601734, -9.217970097227642157 ) ) ;
#60871=EDGE_CURVE ( 'NONE', #56061, #60283, #5042, .T. ) ;
#60874=CARTESIAN_POINT ( 'NONE',  ( -18.78786164167387085, -13.48564496196971874, -0.7125357888566099529 ) ) ;
#60879=ORIENTED_EDGE ( 'NONE', *, *, #19694, .F. ) ;
#60880=CYLINDRICAL_SURFACE ( 'NONE', #53651, 4.999999999999999112 ) ;
#60883=DIRECTION ( 'NONE',  ( -1.000000000000000000, 0.000000000000000000, -0.000000000000000000 ) ) ;
#60884=ADVANCED_FACE ( 'NONE', ( #28498 ), #12538, .T. ) ;
#60885=AXIS2_PLACEMENT_3D ( 'NONE', #39429, #29769, #14475 ) ;
#60890=EDGE_CURVE ( 'NONE', #2445, #35323, #60649, .T. ) ;
#60891=DIRECTION ( 'NONE',  ( 1.000000000000000000, 0.000000000000000000, 0.000000000000000000 ) ) ;
#60892=CARTESIAN_POINT ( 'NONE',  ( -37.00000000000000711, 9.621072037177118119, -8.366449238204259231 ) ) ;
#60894=VECTOR ( 'NONE', #3794, 1000.000000000000000 ) ;
#60897=ORIENTED_EDGE ( 'NONE', *, *, #27487, .F. ) ;
#60898=ORIENTED_EDGE ( 'NONE', *, *, #47465, .F. ) ;
#60900=FACE_OUTER_BOUND ( 'NONE', #17869, .T. ) ;
#60902=AXIS2_PLACEMENT_3D ( 'NONE', #17622, #21945, #16947 ) ;
#60903=DIRECTION ( 'NONE',  ( -1.000000000000000000, 0.000000000000000000, 0.000000000000000000 ) ) ;
#60904=EDGE_LOOP ( 'NONE', ( #15729, #12220, #51158, #19915 ) ) ;
#60905=CIRCLE ( 'NONE', #32228, 12.75000000000000178 ) ;
#60907=ORIENTED_EDGE ( 'NONE', *, *, #63059, .F. ) ;
#60909=EDGE_CURVE ( 'NONE', #32398, #9122, #13990, .T. ) ;
#60910=VECTOR ( 'NONE', #5137, 1000.000000000000000 ) ;
#60912=EDGE_LOOP ( 'NONE', ( #36845, #7754, #65073, #26417 ) ) ;
#60913=DIRECTION ( 'NONE',  ( -1.000000000000000000, 0.000000000000000000, 0.000000000000000000 ) ) ;
#60914=CARTESIAN_POINT ( 'NONE',  ( 35.00000000000000000, 4.705694406421931860E-17, -3.469127814946512892E-15 ) ) ;
#60919=CIRCLE ( 'NONE', #20526, 4.999999999999999112 ) ;
#60921=DIRECTION ( 'NONE',  ( 1.000000000000000000, 0.000000000000000000, 0.000000000000000000 ) ) ;
#60922=ORIENTED_EDGE ( 'NONE', *, *, #43203, .T. ) ;
#60923=CARTESIAN_POINT ( 'NONE',  ( -37.00000000000000711, 0.000000000000000000, 0.000000000000000000 ) ) ;
#60926=ORIENTED_EDGE ( 'NONE', *, *, #45220, .T. ) ;
#60927=DIRECTION ( 'NONE',  ( 0.000000000000000000, -0.01356324068817998940, 0.9999080150203990547 ) ) ;
#60929=FACE_OUTER_BOUND ( 'NONE', #40903, .T. ) ;
#60931=DIRECTION ( 'NONE',  ( -1.000000000000000000, 0.000000000000000000, 0.000000000000000000 ) ) ;
#60933=CARTESIAN_POINT ( 'NONE',  ( 11.12599276166011464, 0.3473812333126252150, 11.99566059042195754 ) ) ;
#60934=DIRECTION ( 'NONE',  ( 1.000000000000000000, 0.000000000000000000, 0.000000000000000000 ) ) ;
#60936=CARTESIAN_POINT ( 'NONE',  ( 47.00000000000000711, 4.705694406421931860E-17, -3.469127814946512892E-15 ) ) ;
#60937=ORIENTED_EDGE ( 'NONE', *, *, #6714, .F. ) ;
#60938=DIRECTION ( 'NONE',  ( 0.000000000000000000, -0.2006870767258961963, 0.9796553971857727694 ) ) ;
#60940=DIRECTION ( 'NONE',  ( 0.000000000000000000, 0.3807014730195219521, -0.9246979985058723095 ) ) ;
#60941=VERTEX_POINT ( 'NONE', #19840 ) ;
#60942=CARTESIAN_POINT ( 'NONE',  ( 37.00000000000000711, 4.309077947445811851, 10.92721691015450780 ) ) ;
#60944=ORIENTED_EDGE ( 'NONE', *, *, #57455, .T. ) ;
#60946=AXIS2_PLACEMENT_3D ( 'NONE', #5625, #50188, #65130 ) ;
#60948=CYLINDRICAL_SURFACE ( 'NONE', #6826, 12.75000000000000178 ) ;
#60949=DIRECTION ( 'NONE',  ( -1.000000000000000000, 0.000000000000000000, 0.000000000000000000 ) ) ;
#60952=EDGE_LOOP ( 'NONE', ( #14833, #14441, #26262, #30610 ) ) ;
#60953=DIRECTION ( 'NONE',  ( -0.9015184547431841500, -0.4327406564646559262, 0.000000000000000000 ) ) ;
#60954=EDGE_CURVE ( 'NONE', #48650, #60581, #49050, .T. ) ;
#60955=CIRCLE ( 'NONE', #15277, 12.75000000000000178 ) ;
#60956=VERTEX_POINT ( 'NONE', #40100 ) ;
#60958=AXIS2_PLACEMENT_3D ( 'NONE', #47468, #2587, #17850 ) ;
#60959=DIRECTION ( 'NONE',  ( -1.000000000000000000, 0.000000000000000000, 0.000000000000000000 ) ) ;
#60960=EDGE_CURVE ( 'NONE', #21860, #27364, #9757, .T. ) ;
#60961=CARTESIAN_POINT ( 'NONE',  ( -29.92777678363736626, -3.750539801530011985, -12.96855624952674724 ) ) ;
#60962=EDGE_LOOP ( 'NONE', ( #28557, #10109, #28126, #53156 ) ) ;
#60963=CIRCLE ( 'NONE', #6810, 5.000000000000000888 ) ;
#60965=CIRCLE ( 'NONE', #53570, 12.18650000000000055 ) ;
#60968=CARTESIAN_POINT ( 'NONE',  ( -4.975205859172449507, -1.416020129149132778, 13.42553116244733680 ) ) ;
#60974=AXIS2_PLACEMENT_3D ( 'NONE', #12024, #1742, #2056 ) ;
#60976=LINE ( 'NONE', #5455, #38443 ) ;
#60978=( BOUNDED_CURVE ( )  B_SPLINE_CURVE ( 3, ( #45648, #20385, #40663, #10725 ),
 .UNSPECIFIED., .F., .F. ) 
 B_SPLINE_CURVE_WITH_KNOTS ( ( 4, 4 ),
 ( 5.851531777320561289, 5.909121302884260629 ),
 .UNSPECIFIED. ) 
 CURVE ( )  GEOMETRIC_REPRESENTATION_ITEM ( )  RATIONAL_B_SPLINE_CURVE ( ( 1.000000000000000000, 0.9997236396413186066, 0.9997236396413186066, 1.000000000000000000 ) ) 
 REPRESENTATION_ITEM ( '' )  );
#60981=CARTESIAN_POINT ( 'NONE',  ( 1.585986311398264403, 1.432643833071485906, -11.91909886592589451 ) ) ;
#60983=ORIENTED_EDGE ( 'NONE', *, *, #11270, .T. ) ;
#60984=CARTESIAN_POINT ( 'NONE',  ( -18.45334481119305892, 4.188336017657096733, 11.24834648941091864 ) ) ;
#60987=AXIS2_PLACEMENT_3D ( 'NONE', #2857, #64325, #44361 ) ;
#60988=AXIS2_PLACEMENT_3D ( 'NONE', #61439, #32488, #42136 ) ;
#60991=ORIENTED_EDGE ( 'NONE', *, *, #48537, .T. ) ;
#60992=DIRECTION ( 'NONE',  ( 0.000000000000000000, 0.01356324068817998940, -0.9999080150203990547 ) ) ;
#60994=DIRECTION ( 'NONE',  ( -1.000000000000000000, 0.000000000000000000, 0.000000000000000000 ) ) ;
#60995=DIRECTION ( 'NONE',  ( -1.000000000000000000, 0.000000000000000000, 0.000000000000000000 ) ) ;
#60998=CARTESIAN_POINT ( 'NONE',  ( 22.88594695219327235, -4.822122601967141264, -12.60940655271284427 ) ) ;
#61003=DIRECTION ( 'NONE',  ( 1.000000000000000000, 0.000000000000000000, 0.000000000000000000 ) ) ;
#61004=EDGE_LOOP ( 'NONE', ( #22116, #37428, #21390, #26255 ) ) ;
#61005=ORIENTED_EDGE ( 'NONE', *, *, #17201, .T. ) ;
#61008=AXIS2_PLACEMENT_3D ( 'NONE', #873, #1215, #20508 ) ;
#61010=ADVANCED_FACE ( 'NONE', ( #54774 ), #38817, .T. ) ;
#61011=CARTESIAN_POINT ( 'NONE',  ( 37.00000000000000711, -6.307491713048959170, 9.908974237959705889 ) ) ;
#61014=ORIENTED_EDGE ( 'NONE', *, *, #25830, .T. ) ;
#61015=ORIENTED_EDGE ( 'NONE', *, *, #894, .F. ) ;
#61016=DIRECTION ( 'NONE',  ( 0.000000000000000000, -0.01356324068817998940, 0.9999080150203990547 ) ) ;
#61017=ORIENTED_EDGE ( 'NONE', *, *, #30587, .T. ) ;
#61018=CIRCLE ( 'NONE', #32323, 12.18650000000000055 ) ;
#61020=DIRECTION ( 'NONE',  ( 0.000000000000000000, -1.000000000000000000, 0.000000000000000000 ) ) ;
#61026=VECTOR ( 'NONE', #33219, 1000.000000000000000 ) ;
#61027=EDGE_CURVE ( 'NONE', #62196, #26384, #7977, .T. ) ;
#61029=EDGE_CURVE ( 'NONE', #22470, #13538, #17179, .T. ) ;
#61031=EDGE_CURVE ( 'NONE', #27642, #28605, #44850, .T. ) ;
#61032=CARTESIAN_POINT ( 'NONE',  ( -35.00000000000000000, 0.000000000000000000, 0.000000000000000000 ) ) ;
#61033=CIRCLE ( 'NONE', #10094, 5.000000000000000000 ) ;
#61034=CARTESIAN_POINT ( 'NONE',  ( 10.48620311856346454, 8.250315036047107142, 25.00000000000000000 ) ) ;
#61035=DIRECTION ( 'NONE',  ( 0.000000000000000000, -0.01356324068817991828, 0.9999080150203990547 ) ) ;
#61037=CARTESIAN_POINT ( 'NONE',  ( 3.388896915696421708, -10.79019736087639281, 5.264843862020491372 ) ) ;
#61038=ADVANCED_FACE ( 'NONE', ( #14183 ), #4888, .T. ) ;
#61040=LINE ( 'NONE', #25792, #5472 ) ;
#61042=CARTESIAN_POINT ( 'NONE',  ( 0.2851083653049504285, -0.4107471485392698018, -11.99296822225284131 ) ) ;
#61044=VERTEX_POINT ( 'NONE', #11485 ) ;
#61048=CIRCLE ( 'NONE', #30295, 4.999999999999999112 ) ;
#61052=VERTEX_POINT ( 'NONE', #36441 ) ;
#61053=CARTESIAN_POINT ( 'NONE',  ( -17.37319572219799113, -6.065883689981585114, -12.06447225982703486 ) ) ;
#61054=DIRECTION ( 'NONE',  ( 0.000000000000000000, -0.4698238015817426949, -0.8827602140260283337 ) ) ;
#61057=ORIENTED_EDGE ( 'NONE', *, *, #54093, .T. ) ;
#61058=CYLINDRICAL_SURFACE ( 'NONE', #7934, 4.999999999999999112 ) ;
#61059=CARTESIAN_POINT ( 'NONE',  ( -17.15720051295231485, 7.250774436309729509, -9.563211349854379151 ) ) ;
#61061=CARTESIAN_POINT ( 'NONE',  ( -32.00000000000000711, 12.00000000000000000, 1.469576158976823553E-15 ) ) ;
#61062=ORIENTED_EDGE ( 'NONE', *, *, #43077, .F. ) ;
#61063=DIRECTION ( 'NONE',  ( -1.000000000000000000, 0.000000000000000000, 0.000000000000000000 ) ) ;
#61064=VECTOR ( 'NONE', #25870, 1000.000000000000000 ) ;
#61066=ORIENTED_EDGE ( 'NONE', *, *, #17641, .F. ) ;
#61068=CARTESIAN_POINT ( 'NONE',  ( -35.00000000000000000, -8.699265615722922007, -8.534258022646191932 ) ) ;
#61069=CARTESIAN_POINT ( 'NONE',  ( 24.08299418260464719, 1.037082133578634213, -11.95962290153675056 ) ) ;
#61070=CARTESIAN_POINT ( 'NONE',  ( 8.437200413559441614, 4.669230153606584111, -12.66846808887212106 ) ) ;
#61071=CARTESIAN_POINT ( 'NONE',  ( 0.1900979142430823110, -0.2738684153833558232, -13.49791647769710679 ) ) ;
#61072=CARTESIAN_POINT ( 'NONE',  ( -18.58686583997219088, 4.910876720226735159, 12.57779378420807781 ) ) ;
#61074=ORIENTED_EDGE ( 'NONE', *, *, #12809, .F. ) ;
#61075=DIRECTION ( 'NONE',  ( -0.000000000000000000, -0.000000000000000000, -1.000000000000000000 ) ) ;
#61076=ORIENTED_EDGE ( 'NONE', *, *, #34731, .F. ) ;
#61079=ADVANCED_FACE ( 'NONE', ( #35452 ), #21482, .T. ) ;
#61080=EDGE_CURVE ( 'NONE', #27549, #2404, #1290, .T. ) ;
#61081=EDGE_LOOP ( 'NONE', ( #8549, #14372, #43537, #34303 ) ) ;
#61083=DIRECTION ( 'NONE',  ( 1.000000000000000000, 0.000000000000000000, 0.000000000000000000 ) ) ;
#61084=CARTESIAN_POINT ( 'NONE',  ( 35.00000000000000000, -9.321877890560486435, -7.146664589317880178 ) ) ;
#61089=VERTEX_POINT ( 'NONE', #41087 ) ;
#61090=DIRECTION ( 'NONE',  ( 0.000000000000000000, -0.9718671068226434340, 0.2355298848897617037 ) ) ;
#61092=FACE_OUTER_BOUND ( 'NONE', #40237, .T. ) ;
#61093=VECTOR ( 'NONE', #29742, 1000.000000000000000 ) ;
#61094=CARTESIAN_POINT ( 'NONE',  ( 35.00000000000000000, 10.32377448871667625, -6.475373545682339582 ) ) ;
#61095=CARTESIAN_POINT ( 'NONE',  ( 36.00000000000000711, 12.42372387097886488, 2.865935305911484043 ) ) ;
#61096=FACE_OUTER_BOUND ( 'NONE', #20434, .T. ) ;
#61099=ORIENTED_EDGE ( 'NONE', *, *, #62016, .T. ) ;
#61100=CARTESIAN_POINT ( 'NONE',  ( 37.00000000000000711, 11.32068061209303522, 5.865551165830957814 ) ) ;
#61101=CARTESIAN_POINT ( 'NONE',  ( 23.20721382908649488, 9.991207635573182699, -6.653344022984436279 ) ) ;
#61102=EDGE_CURVE ( 'NONE', #40994, #14607, #11848, .T. ) ;
#61104=CARTESIAN_POINT ( 'NONE',  ( -18.92121795399529915, 13.50133162273161069, 0.2605718306269828033 ) ) ;
#61105=CARTESIAN_POINT ( 'NONE',  ( -2.952869152607111136, 7.581333670610111319, 11.17020052527586138 ) ) ;
#61106=CARTESIAN_POINT ( 'NONE',  ( 2.354167843600960097, -6.278647867796540716, 25.00000000000000000 ) ) ;
#61108=DIRECTION ( 'NONE',  ( 1.000000000000000000, 0.000000000000000000, 0.000000000000000000 ) ) ;
#61110=ORIENTED_EDGE ( 'NONE', *, *, #31910, .T. ) ;
#61111=CARTESIAN_POINT ( 'NONE',  ( -7.489022030332961322, -5.127957880411574187, -10.84914964302385521 ) ) ;
#61112=ORIENTED_EDGE ( 'NONE', *, *, #45409, .F. ) ;
#61113=CARTESIAN_POINT ( 'NONE',  ( -3.322308238815765868, -10.53368969201583916, 5.762262606413962374 ) ) ;
#61115=ADVANCED_FACE ( 'NONE', ( #40782 ), #15492, .T. ) ;
#61116=DIRECTION ( 'NONE',  ( 0.000000000000000000, -0.01356324068817998940, 0.9999080150203990547 ) ) ;
#61118=DIRECTION ( 'NONE',  ( -1.000000000000000000, 0.000000000000000000, 0.000000000000000000 ) ) ;
#61127=EDGE_CURVE ( 'NONE', #47727, #37018, #56056, .T. ) ;
#61130=DIRECTION ( 'NONE',  ( -1.000000000000000000, 0.000000000000000000, 0.000000000000000000 ) ) ;
#61131=AXIS2_PLACEMENT_3D ( 'NONE', #45486, #60795, #12207 ) ;
#61132=ORIENTED_EDGE ( 'NONE', *, *, #34210, .F. ) ;
#61133=DIRECTION ( 'NONE',  ( -1.000000000000000000, 0.000000000000000000, -0.000000000000000000 ) ) ;
#61134=EDGE_CURVE ( 'NONE', #55855, #53922, #11176, .T. ) ;
#61135=VERTEX_POINT ( 'NONE', #47418 ) ;
#61138=CARTESIAN_POINT ( 'NONE',  ( 29.03457606387295087, -4.854210015632035358, 10.97436308512422265 ) ) ;
#61139=CARTESIAN_POINT ( 'NONE',  ( -5.804292984923859144, -1.481750644001851525, 11.90855073620921267 ) ) ;
#61140=CIRCLE ( 'NONE', #32453, 4.999999999999997335 ) ;
#61142=ORIENTED_EDGE ( 'NONE', *, *, #48382, .T. ) ;
#61144=ORIENTED_EDGE ( 'NONE', *, *, #39277, .T. ) ;
#61146=CARTESIAN_POINT ( 'NONE',  ( 35.00000000000000000, -9.063649021438894948, 8.146229107149494553 ) ) ;
#61147=CARTESIAN_POINT ( 'NONE',  ( 47.00000000000000711, 4.705694406421931860E-17, -3.469127814946512892E-15 ) ) ;
#61150=FACE_OUTER_BOUND ( 'NONE', #25392, .T. ) ;
#61151=CARTESIAN_POINT ( 'NONE',  ( -11.24844400926880716, -6.045701199311597662, 10.37522813442839009 ) ) ;
#61152=ORIENTED_EDGE ( 'NONE', *, *, #64674, .T. ) ;
#61153=DIRECTION ( 'NONE',  ( 0.000000000000000000, 0.3554799084908970563, 0.9346839223284539866 ) ) ;
#61154=ORIENTED_EDGE ( 'NONE', *, *, #9794, .F. ) ;
#61157=CARTESIAN_POINT ( 'NONE',  ( -35.00000000000000000, -11.91791701451264629, -2.544412758415973030 ) ) ;
#61158=EDGE_CURVE ( 'NONE', #42345, #33595, #13136, .T. ) ;
#61161=DIRECTION ( 'NONE',  ( -1.836970198721029688E-16, 1.000000000000000000, 0.000000000000000000 ) ) ;
#61162=EDGE_CURVE ( 'NONE', #45235, #24100, #22496, .T. ) ;
#61164=DIRECTION ( 'NONE',  ( 1.000000000000000000, 0.000000000000000000, 0.000000000000000000 ) ) ;
#61165=CARTESIAN_POINT ( 'NONE',  ( 6.361445718264521432, -4.355102044641763648, -12.77822703589027320 ) ) ;
#61168=ORIENTED_EDGE ( 'NONE', *, *, #40381, .F. ) ;
#61172=CARTESIAN_POINT ( 'NONE',  ( 37.00000000000000711, -12.71517666308947092, 0.9416912585475696318 ) ) ;
#61173=ORIENTED_EDGE ( 'NONE', *, *, #52853, .T. ) ;
#61174=EDGE_CURVE ( 'NONE', #15952, #51800, #62350, .T. ) ;
#61175=VERTEX_POINT ( 'NONE', #11806 ) ;
#61178=DIRECTION ( 'NONE',  ( -1.000000000000000000, 0.000000000000000000, 0.000000000000000000 ) ) ;
#61179=CARTESIAN_POINT ( 'NONE',  ( 35.00000000000000000, -9.348667969174460524, -7.817492529713823579 ) ) ;
#61183=VECTOR ( 'NONE', #37703, 1000.000000000000000 ) ;
#61184=CARTESIAN_POINT ( 'NONE',  ( -28.41827485489077532, 3.509237424706437292, 11.47541949982830722 ) ) ;
#61185=VECTOR ( 'NONE', #10405, 1000.000000000000000 ) ;
#61186=ORIENTED_EDGE ( 'NONE', *, *, #60242, .T. ) ;
#61189=DIRECTION ( 'NONE',  ( 1.000000000000000000, -0.000000000000000000, 0.000000000000000000 ) ) ;
#61191=EDGE_CURVE ( 'NONE', #47785, #9350, #27767, .T. ) ;
#61196=ORIENTED_EDGE ( 'NONE', *, *, #39529, .T. ) ;
#61197=LINE ( 'NONE', #60870, #8835 ) ;
#61200=CARTESIAN_POINT ( 'NONE',  ( -35.00000000000000000, -11.42599468261432527, 4.237620530777758354 ) ) ;
#61201=CARTESIAN_POINT ( 'NONE',  ( 36.00000000000000711, 8.366449238204499039, 9.621072037176899627 ) ) ;
#61203=ORIENTED_EDGE ( 'NONE', *, *, #31834, .F. ) ;
#61204=CARTESIAN_POINT ( 'NONE',  ( 37.00000000000000711, 1.171570255487609291, 11.68758509253246380 ) ) ;
#61205=DIRECTION ( 'NONE',  ( 0.000000000000000000, -0.5767582926624852391, -0.8169148498130358593 ) ) ;
#61206=CARTESIAN_POINT ( 'NONE',  ( -37.00000000000000711, 0.000000000000000000, 0.000000000000000000 ) ) ;
#61209=EDGE_CURVE ( 'NONE', #50989, #7512, #48070, .T. ) ;
#61213=EDGE_CURVE ( 'NONE', #37677, #34871, #52277, .T. ) ;
#61215=LINE ( 'NONE', #65523, #15546 ) ;
#61217=EDGE_CURVE ( 'NONE', #48103, #44068, #44785, .T. ) ;
#61218=ORIENTED_EDGE ( 'NONE', *, *, #50744, .F. ) ;
#61219=CIRCLE ( 'NONE', #30417, 12.18650000000000055 ) ;
#61220=ORIENTED_EDGE ( 'NONE', *, *, #32685, .F. ) ;
#61223=DIRECTION ( 'NONE',  ( -1.000000000000000000, 0.000000000000000000, 0.000000000000000000 ) ) ;
#61225=ORIENTED_EDGE ( 'NONE', *, *, #5858, .T. ) ;
#61226=VERTEX_POINT ( 'NONE', #47731 ) ;
#61227=ORIENTED_EDGE ( 'NONE', *, *, #41048, .F. ) ;
#61228=CARTESIAN_POINT ( 'NONE',  ( 29.26291958553499484, -9.868730160957575492, 6.831222511614969406 ) ) ;
#61229=CARTESIAN_POINT ( 'NONE',  ( -21.04906020170784586, -11.41231286973902215, -3.710994071045400133 ) ) ;
#61231=DIRECTION ( 'NONE',  ( 0.000000000000000000, 0.01356324068817998940, -0.9999080150203989437 ) ) ;
#61232=DIRECTION ( 'NONE',  ( 0.000000000000000000, -0.01356324068817992175, 0.9999080150203990547 ) ) ;
#61234=ORIENTED_EDGE ( 'NONE', *, *, #1831, .T. ) ;
#61237=CARTESIAN_POINT ( 'NONE',  ( -35.00000000000000000, 0.000000000000000000, 0.000000000000000000 ) ) ;
#61238=EDGE_LOOP ( 'NONE', ( #27973, #29669, #56822, #23955 ) ) ;
#61239=CYLINDRICAL_SURFACE ( 'NONE', #36325, 4.999999999999999112 ) ;
#61242=VERTEX_POINT ( 'NONE', #22452 ) ;
#61244=DIRECTION ( 'NONE',  ( 0.000000000000000000, 0.8827602140260332186, -0.4698238015817334245 ) ) ;
#61245=CARTESIAN_POINT ( 'NONE',  ( 12.93723047338301058, 4.476360154859203355, 25.00000000000000000 ) ) ;
#61246=LINE ( 'NONE', #51940, #6038 ) ;
#61249=CARTESIAN_POINT ( 'NONE',  ( -32.00000000000000000, 15.00000000000000000, 1.836970198721029589E-15 ) ) ;
#61251=CARTESIAN_POINT ( 'NONE',  ( 36.00000000000000711, -5.865551165831000446, 11.32068061209301035 ) ) ;
#61254=ORIENTED_EDGE ( 'NONE', *, *, #43979, .F. ) ;
#61256=ORIENTED_EDGE ( 'NONE', *, *, #45473, .F. ) ;
#61261=CARTESIAN_POINT ( 'NONE',  ( -35.00000000000000000, -4.946702696913093611, -11.13736569743279681 ) ) ;
#61262=LINE ( 'NONE', #56951, #14868 ) ;
#61263=DIRECTION ( 'NONE',  ( 1.000000000000000000, 0.000000000000000000, -0.000000000000000000 ) ) ;
#61265=DIRECTION ( 'NONE',  ( -1.000000000000000000, 0.000000000000000000, -0.000000000000000000 ) ) ;
#61266=ADVANCED_FACE ( 'NONE', ( #58717 ), #33419, .T. ) ;
#61268=ORIENTED_EDGE ( 'NONE', *, *, #7345, .F. ) ;
#61269=CIRCLE ( 'NONE', #62300, 12.74999999999999822 ) ;
#61272=DIRECTION ( 'NONE',  ( -1.000000000000000000, -1.836970198721029688E-16, 0.000000000000000000 ) ) ;
#61273=DIRECTION ( 'NONE',  ( 1.000000000000000000, 0.000000000000000000, 0.000000000000000000 ) ) ;
#61275=ORIENTED_EDGE ( 'NONE', *, *, #57958, .F. ) ;
#61276=DIRECTION ( 'NONE',  ( 1.000000000000000000, -0.000000000000000000, -0.000000000000000000 ) ) ;
#61279=DIRECTION ( 'NONE',  ( -1.000000000000000000, -0.000000000000000000, 0.000000000000000000 ) ) ;
#61282=ORIENTED_EDGE ( 'NONE', *, *, #8392, .F. ) ;
#61283=DIRECTION ( 'NONE',  ( 0.000000000000000000, -0.01356324068817998940, 0.9999080150203990547 ) ) ;
#61285=CARTESIAN_POINT ( 'NONE',  ( -35.00000000000000000, -12.70128625845193682, 1.113475361586445889 ) ) ;
#61286=EDGE_CURVE ( 'NONE', #42768, #32729, #43758, .T. ) ;
#61292=DIRECTION ( 'NONE',  ( 1.000000000000000000, -0.000000000000000000, 0.000000000000000000 ) ) ;
#61298=AXIS2_PLACEMENT_3D ( 'NONE', #54483, #64120, #3637 ) ;
#61299=ORIENTED_EDGE ( 'NONE', *, *, #6848, .F. ) ;
#61300=LINE ( 'NONE', #61967, #62416 ) ;
#61301=ORIENTED_EDGE ( 'NONE', *, *, #818, .T. ) ;
#61304=CARTESIAN_POINT ( 'NONE',  ( -35.00000000000000000, -6.753013023069787124, 10.14433819232432477 ) ) ;
#61306=ADVANCED_FACE ( 'NONE', ( #16804 ), #43054, .T. ) ;
#61310=DIRECTION ( 'NONE',  ( 0.000000000000000000, -0.4935949184179321825, 0.8696919319575150409 ) ) ;
#61311=VERTEX_POINT ( 'NONE', #58367 ) ;
#61312=EDGE_CURVE ( 'NONE', #31078, #2293, #32012, .T. ) ;
#61313=FACE_OUTER_BOUND ( 'NONE', #9558, .T. ) ;
#61314=ORIENTED_EDGE ( 'NONE', *, *, #60782, .F. ) ;
#61315=CARTESIAN_POINT ( 'NONE',  ( -47.00000000000000711, 0.000000000000000000, 0.000000000000000000 ) ) ;
#61321=ADVANCED_FACE ( 'NONE', ( #28420 ), #8470, .T. ) ;
#61326=ORIENTED_EDGE ( 'NONE', *, *, #51967, .F. ) ;
#61327=DIRECTION ( 'NONE',  ( -0.000000000000000000, -0.000000000000000000, -1.000000000000000000 ) ) ;
#61328=VERTEX_POINT ( 'NONE', #60007 ) ;
#61329=EDGE_CURVE ( 'NONE', #21190, #21166, #40616, .T. ) ;
#61331=CARTESIAN_POINT ( 'NONE',  ( -37.00000000000000711, 10.62137734850268345, 5.015831474386344802 ) ) ;
#61334=DIRECTION ( 'NONE',  ( 1.000000000000000000, 0.000000000000000000, 0.000000000000000000 ) ) ;
#61336=DIRECTION ( 'NONE',  ( 0.000000000000000000, -0.01356324068817991828, 0.9999080150203990547 ) ) ;
#61337=AXIS2_PLACEMENT_3D ( 'NONE', #3645, #64436, #32862 ) ;
#61338=VERTEX_POINT ( 'NONE', #59037 ) ;
#61339=DIRECTION ( 'NONE',  ( -1.000000000000000000, 0.000000000000000000, -0.000000000000000000 ) ) ;
#61340=CARTESIAN_POINT ( 'NONE',  ( 5.376045869553820467, -9.552872917373893102, 7.269855246128603454 ) ) ;
#61341=DIRECTION ( 'NONE',  ( -1.000000000000000000, -0.000000000000000000, 0.000000000000000000 ) ) ;
#61345=LINE ( 'NONE', #21110, #4604 ) ;
#61348=EDGE_CURVE ( 'NONE', #63981, #8085, #53355, .T. ) ;
#61351=CARTESIAN_POINT ( 'NONE',  ( 36.00000000000000711, 3.473736367725426266, 12.26766708251987836 ) ) ;
#61355=ORIENTED_EDGE ( 'NONE', *, *, #13236, .T. ) ;
#61357=CYLINDRICAL_SURFACE ( 'NONE', #37543, 12.18649999999999878 ) ;
#61359=ORIENTED_EDGE ( 'NONE', *, *, #40669, .T. ) ;
#61360=CYLINDRICAL_SURFACE ( 'NONE', #22785, 13.50000000000000178 ) ;
#61362=CARTESIAN_POINT ( 'NONE',  ( 36.00000000000000711, 2.696588552979229725, 12.46157735505186004 ) ) ;
#61363=FACE_OUTER_BOUND ( 'NONE', #34628, .T. ) ;
#61364=ORIENTED_EDGE ( 'NONE', *, *, #35711, .T. ) ;
#61366=AXIS2_PLACEMENT_3D ( 'NONE', #20273, #10289, #34575 ) ;
#61367=EDGE_CURVE ( 'NONE', #311, #44305, #1343, .T. ) ;
#61369=ORIENTED_EDGE ( 'NONE', *, *, #39102, .T. ) ;
#61370=DIRECTION ( 'NONE',  ( 0.000000000000000000, -0.9246979985058680906, -0.3807014730195321661 ) ) ;
#61372=FACE_OUTER_BOUND ( 'NONE', #58706, .T. ) ;
#61373=CARTESIAN_POINT ( 'NONE',  ( 8.676227275390266058, 5.971235288444897371, -12.11418353888797661 ) ) ;
#61374=EDGE_CURVE ( 'NONE', #63634, #14535, #8808, .T. ) ;
#61376=ADVANCED_FACE ( 'NONE', ( #29096 ), #49401, .T. ) ;
#61377=CARTESIAN_POINT ( 'NONE',  ( -18.56098820112710968, 4.668070274350404780, 12.66988895734626297 ) ) ;
#61378=CYLINDRICAL_SURFACE ( 'NONE', #10, 5.000000000000000888 ) ;
#61380=EDGE_CURVE ( 'NONE', #64240, #19313, #59677, .T. ) ;
#61381=ORIENTED_EDGE ( 'NONE', *, *, #62320, .T. ) ;
#61383=EDGE_LOOP ( 'NONE', ( #55586, #27616, #60009, #27009 ) ) ;
#61385=CYLINDRICAL_SURFACE ( 'NONE', #13498, 5.000000000000000888 ) ;
#61387=ADVANCED_FACE ( 'NONE', ( #54029 ), #9123, .T. ) ;
#61388=CARTESIAN_POINT ( 'NONE',  ( 35.00000000000000000, 0.01609748574445066943, -11.74614673114903773 ) ) ;
#61391=DIRECTION ( 'NONE',  ( 0.000000000000000000, -0.04924826701375277505, -0.9987865678893275145 ) ) ;
#61392=LINE ( 'NONE', #31155, #40400 ) ;
#61393=EDGE_CURVE ( 'NONE', #35473, #45350, #18340, .T. ) ;
#61396=CARTESIAN_POINT ( 'NONE',  ( 35.00000000000000000, 10.12742074351896271, -7.745827850123049529 ) ) ;
#61398=EDGE_LOOP ( 'NONE', ( #46755, #25945, #39251, #3191 ) ) ;
#61399=CARTESIAN_POINT ( 'NONE',  ( 22.64436338924570080, -10.50028284738791839, -5.818370998278716399 ) ) ;
#61402=CARTESIAN_POINT ( 'NONE',  ( 37.00000000000000711, 11.72195762423409704, 0.7536123767498881243 ) ) ;
#61404=CARTESIAN_POINT ( 'NONE',  ( -36.00000000000000711, 5.710938531231713355, 11.39945968423473666 ) ) ;
#61405=ADVANCED_FACE ( 'NONE', ( #18482 ), #29404, .T. ) ;
#61406=CARTESIAN_POINT ( 'NONE',  ( 35.00000000000000000, 7.110831038798420600, 9.896810808925309288 ) ) ;
#61409=CIRCLE ( 'NONE', #1957, 12.18650000000000233 ) ;
#61410=CARTESIAN_POINT ( 'NONE',  ( 22.22111349864275809, 11.93717068860222774, -1.276428617110490382 ) ) ;
#61411=CARTESIAN_POINT ( 'NONE',  ( -37.00000000000000711, 11.91791701451266405, 2.544412758415886877 ) ) ;
#61414=DIRECTION ( 'NONE',  ( 0.000000000000000000, 0.01356324068817998073, -0.9999080150203990547 ) ) ;
#61415=LINE ( 'NONE', #22093, #17501 ) ;
#61417=AXIS2_PLACEMENT_3D ( 'NONE', #23907, #53516, #54487 ) ;
#61418=VERTEX_POINT ( 'NONE', #33732 ) ;
#61420=DIRECTION ( 'NONE',  ( -1.000000000000000000, 0.000000000000000000, 0.000000000000000000 ) ) ;
#61421=AXIS2_PLACEMENT_3D ( 'NONE', #25539, #10562, #56122 ) ;
#61422=VECTOR ( 'NONE', #46682, 1000.000000000000000 ) ;
#61423=VERTEX_POINT ( 'NONE', #27651 ) ;
#61429=CYLINDRICAL_SURFACE ( 'NONE', #58738, 12.18649999999999878 ) ;
#61430=CARTESIAN_POINT ( 'NONE',  ( 35.00000000000000000, -6.946017217730008575, -10.01317267707884184 ) ) ;
#61432=FACE_OUTER_BOUND ( 'NONE', #155, .T. ) ;
#61434=DIRECTION ( 'NONE',  ( -1.000000000000000000, 0.000000000000000000, 0.000000000000000000 ) ) ;
#61437=DIRECTION ( 'NONE',  ( -1.000000000000000000, 0.000000000000000000, 0.000000000000000000 ) ) ;
#61438=ORIENTED_EDGE ( 'NONE', *, *, #55567, .F. ) ;
#61439=CARTESIAN_POINT ( 'NONE',  ( 35.00000000000000000, 4.705694406421931860E-17, -3.469127814946512892E-15 ) ) ;
#61440=CARTESIAN_POINT ( 'NONE',  ( -35.00000000000000000, 0.000000000000000000, 0.000000000000000000 ) ) ;
#61441=CARTESIAN_POINT ( 'NONE',  ( 27.76533532700122464, -10.82083892906157629, 5.202369787004509583 ) ) ;
#61445=ORIENTED_EDGE ( 'NONE', *, *, #56803, .T. ) ;
#61449=CARTESIAN_POINT ( 'NONE',  ( -35.00000000000000000, 0.000000000000000000, 0.000000000000000000 ) ) ;
#61450=CARTESIAN_POINT ( 'NONE',  ( 0.000000000000000000, -1.734723475976807094E-15, -13.50000000000000178 ) ) ;
#61453=CIRCLE ( 'NONE', #6329, 12.18650000000000055 ) ;
#61458=ORIENTED_EDGE ( 'NONE', *, *, #12852, .T. ) ;
#61459=ADVANCED_FACE ( 'NONE', ( #52935 ), #37962, .T. ) ;
#61461=ORIENTED_EDGE ( 'NONE', *, *, #9083, .T. ) ;
#61464=AXIS2_PLACEMENT_3D ( 'NONE', #52330, #62273, #11408 ) ;
#61465=CARTESIAN_POINT ( 'NONE',  ( 17.86670421114028073, 9.033888303652016560, 10.06012754632461004 ) ) ;
#61469=EDGE_LOOP ( 'NONE', ( #994, #43836, #9591, #65609 ) ) ;
#61470=DIRECTION ( 'NONE',  ( -0.000000000000000000, -1.000000000000000000, -0.000000000000000000 ) ) ;
#61472=DIRECTION ( 'NONE',  ( 0.000000000000000000, 0.000000000000000000, -1.000000000000000000 ) ) ;
#61473=EDGE_CURVE ( 'NONE', #32620, #45080, #4525, .T. ) ;
#61477=AXIS2_PLACEMENT_3D ( 'NONE', #997, #15935, #37206 ) ;
#61478=DIRECTION ( 'NONE',  ( 0.000000000000000000, 0.01356324068817998940, -0.9999080150203990547 ) ) ;
#61479=ADVANCED_FACE ( 'NONE', ( #48620 ), #22691, .T. ) ;
#61480=VERTEX_POINT ( 'NONE', #28323 ) ;
#61482=ORIENTED_EDGE ( 'NONE', *, *, #37051, .F. ) ;
#61486=EDGE_CURVE ( 'NONE', #3067, #44205, #13031, .T. ) ;
#61487=CARTESIAN_POINT ( 'NONE',  ( 37.00000000000000711, 4.705694406421931860E-17, -3.469127814946512892E-15 ) ) ;
#61492=ORIENTED_EDGE ( 'NONE', *, *, #53517, .F. ) ;
#61493=EDGE_CURVE ( 'NONE', #55501, #34288, #59044, .T. ) ;
#61495=ORIENTED_EDGE ( 'NONE', *, *, #30239, .F. ) ;
#61496=DIRECTION ( 'NONE',  ( 1.000000000000000000, 0.000000000000000000, 0.000000000000000000 ) ) ;
#61498=EDGE_CURVE ( 'NONE', #27716, #18175, #58417, .T. ) ;
#61501=CARTESIAN_POINT ( 'NONE',  ( 29.21915657715117121, 6.866533784549974762, 9.851962652288564826 ) ) ;
#61502=LINE ( 'NONE', #52546, #24902 ) ;
#61505=DIRECTION ( 'NONE',  ( -1.000000000000000000, 0.000000000000000000, 0.000000000000000000 ) ) ;
#61506=VECTOR ( 'NONE', #27992, 1000.000000000000000 ) ;
#61507=ORIENTED_EDGE ( 'NONE', *, *, #16922, .F. ) ;
#61508=CARTESIAN_POINT ( 'NONE',  ( -10.95212338237647920, -9.902220863987562183, -6.778349501228825069 ) ) ;
#61509=CARTESIAN_POINT ( 'NONE',  ( -35.00000000000000000, -3.640372113593638215, 12.21925492305360983 ) ) ;
#61511=DIRECTION ( 'NONE',  ( 0.000000000000000000, -0.01356324068817998940, 0.9999080150203990547 ) ) ;
#61512=DIRECTION ( 'NONE',  ( 1.000000000000000000, -0.000000000000000000, 0.000000000000000000 ) ) ;
#61514=CARTESIAN_POINT ( 'NONE',  ( 35.00000000000000000, 6.280308599560279426, 9.926225166346956286 ) ) ;
#61515=CARTESIAN_POINT ( 'NONE',  ( -35.00000000000000000, 4.018060380616562455, -11.50504120060938718 ) ) ;
#61516=CARTESIAN_POINT ( 'NONE',  ( 35.00000000000000000, 4.946702696913328090, 11.13736569743268845 ) ) ;
#61517=CARTESIAN_POINT ( 'NONE',  ( 24.44374455839395921, -11.03111509265887591, -7.786461916442146247 ) ) ;
#61518=CIRCLE ( 'NONE', #967, 4.999999999999999112 ) ;
#61519=EDGE_CURVE ( 'NONE', #62927, #55740, #19368, .T. ) ;
#61520=CIRCLE ( 'NONE', #9482, 12.74999999999999822 ) ;
#61521=LINE ( 'NONE', #30942, #62632 ) ;
#61522=DIRECTION ( 'NONE',  ( 0.000000000000000000, -0.9937233664769772323, 0.1118654143051511785 ) ) ;
#61525=DIRECTION ( 'NONE',  ( 0.000000000000000000, -0.1740410799127471153, -0.9847383929261642743 ) ) ;
#61526=EDGE_CURVE ( 'NONE', #6547, #25804, #38629, .T. ) ;
#61527=AXIS2_PLACEMENT_3D ( 'NONE', #5310, #56162, #45215 ) ;
#61528=ORIENTED_EDGE ( 'NONE', *, *, #31797, .F. ) ;
#61529=( BOUNDED_CURVE ( )  B_SPLINE_CURVE ( 3, ( #15577, #11264, #50530, #55838 ),
 .UNSPECIFIED., .F., .F. ) 
 B_SPLINE_CURVE_WITH_KNOTS ( ( 4, 4 ),
 ( 5.368938899291405775, 5.390737220995221790 ),
 .UNSPECIFIED. ) 
 CURVE ( )  GEOMETRIC_REPRESENTATION_ITEM ( )  RATIONAL_B_SPLINE_CURVE ( ( 1.000000000000000000, 0.9999604031562251416, 0.9999604031562251416, 1.000000000000000000 ) ) 
 REPRESENTATION_ITEM ( '' )  );
#61530=ORIENTED_EDGE ( 'NONE', *, *, #31834, .T. ) ;
#61531=CARTESIAN_POINT ( 'NONE',  ( 37.00000000000000711, 4.705694406421931860E-17, -3.469127814946512892E-15 ) ) ;
#61533=CARTESIAN_POINT ( 'NONE',  ( 35.00000000000000000, 10.07641281632177588, -6.036400161834603928 ) ) ;
#61534=DIRECTION ( 'NONE',  ( -1.000000000000000000, 0.000000000000000000, 0.000000000000000000 ) ) ;
#61535=ORIENTED_EDGE ( 'NONE', *, *, #10217, .T. ) ;
#61539=DIRECTION ( 'NONE',  ( 1.000000000000000000, 0.000000000000000000, 0.000000000000000000 ) ) ;
#61541=CARTESIAN_POINT ( 'NONE',  ( 37.00000000000000711, 9.752226076388984310, 6.547236723513913503 ) ) ;
#61542=VECTOR ( 'NONE', #65735, 1000.000000000000000 ) ;
#61543=ORIENTED_EDGE ( 'NONE', *, *, #34295, .F. ) ;
#61544=CARTESIAN_POINT ( 'NONE',  ( 6.511276587883018330, -4.283181266385642338, 12.80273922584868629 ) ) ;
#61545=CARTESIAN_POINT ( 'NONE',  ( -35.00000000000000000, 11.07407352312212723, 3.916263239775389149 ) ) ;
#61547=DIRECTION ( 'NONE',  ( -1.000000000000000000, -0.000000000000000000, 0.000000000000000000 ) ) ;
#61551=ORIENTED_EDGE ( 'NONE', *, *, #13358, .T. ) ;
#61552=LINE ( 'NONE', #35941, #25646 ) ;
#61554=FACE_OUTER_BOUND ( 'NONE', #3430, .T. ) ;
#61556=DIRECTION ( 'NONE',  ( 0.000000000000000000, -0.01356324068817998940, 0.9999080150203990547 ) ) ;
#61557=EDGE_CURVE ( 'NONE', #22685, #44279, #22546, .T. ) ;
#61558=DIRECTION ( 'NONE',  ( 0.000000000000000000, 0.2618041379715635442, -0.9651210252299794456 ) ) ;
#61561=B_SPLINE_CURVE_WITH_KNOTS ( 'NONE', 3,
 ( #51588, #12527, #31595, #26294, #46908, #63725, #48795, #56563 ),
 .UNSPECIFIED., .F., .F.,
 ( 4, 2, 2, 4 ),
 ( 0.004035003267135223344, 0.006329346555864282138, 0.007476518200228814137, 0.008623689844593347004 ),
 .UNSPECIFIED. ) ;
#61562=CARTESIAN_POINT ( 'NONE',  ( -7.489022030332961322, 5.127957880411581293, -10.84914964302385521 ) ) ;
#61566=CARTESIAN_POINT ( 'NONE',  ( -17.68536118190054651, 2.866363609320780270, -13.19378535958787069 ) ) ;
#61567=VERTEX_POINT ( 'NONE', #12952 ) ;
#61568=EDGE_CURVE ( 'NONE', #40799, #40241, #3968, .T. ) ;
#61569=CIRCLE ( 'NONE', #62599, 5.000000000000000000 ) ;
#61570=DIRECTION ( 'NONE',  ( 1.000000000000000000, 0.000000000000000000, 0.000000000000000000 ) ) ;
#61571=VERTEX_POINT ( 'NONE', #53195 ) ;
#61573=CARTESIAN_POINT ( 'NONE',  ( 37.00000000000000711, -11.29812557209478996, -3.213188559034203529 ) ) ;
#61576=CARTESIAN_POINT ( 'NONE',  ( 37.00000000000000711, 4.705694406421931860E-17, -3.469127814946512892E-15 ) ) ;
#61577=DIRECTION ( 'NONE',  ( 0.000000000000000000, 0.01356324068817998940, -0.9999080150203990547 ) ) ;
#61581=CARTESIAN_POINT ( 'NONE',  ( -35.00000000000000000, -7.718225330433740261, -9.430788938294131896 ) ) ;
#61582=ORIENTED_EDGE ( 'NONE', *, *, #34216, .F. ) ;
#61583=LINE ( 'NONE', #62246, #55549 ) ;
#61585=CARTESIAN_POINT ( 'NONE',  ( -37.00000000000000711, 0.000000000000000000, 0.000000000000000000 ) ) ;
#61586=DIRECTION ( 'NONE',  ( 1.000000000000000000, 0.000000000000000000, 0.000000000000000000 ) ) ;
#61587=CARTESIAN_POINT ( 'NONE',  ( -35.00000000000000000, 0.000000000000000000, 0.000000000000000000 ) ) ;
#61588=VERTEX_POINT ( 'NONE', #43200 ) ;
#61590=EDGE_CURVE ( 'NONE', #3506, #48302, #59714, .T. ) ;
#61591=AXIS2_PLACEMENT_3D ( 'NONE', #35151, #21185, #25194 ) ;
#61592=ADVANCED_FACE ( 'NONE', ( #44192 ), #63475, .T. ) ;
#61595=CARTESIAN_POINT ( 'NONE',  ( 37.00000000000000711, 4.705694406421931860E-17, -3.469127814946512892E-15 ) ) ;
#61599=DIRECTION ( 'NONE',  ( 0.000000000000000000, -0.01356324068817999114, 0.9999080150203989437 ) ) ;
#61600=EDGE_CURVE ( 'NONE', #58586, #16833, #6660, .T. ) ;
#61602=CARTESIAN_POINT ( 'NONE',  ( -16.15337078595565501, 7.823288771779902007, 11.00216753322003704 ) ) ;
#61604=CIRCLE ( 'NONE', #22311, 5.000000000000000000 ) ;
#61605=ORIENTED_EDGE ( 'NONE', *, *, #1987, .F. ) ;
#61606=LINE ( 'NONE', #46998, #7732 ) ;
#61607=CARTESIAN_POINT ( 'NONE',  ( 3.485421372826590591, 6.960100877362279448, -9.812747699357830200 ) ) ;
#61611=DIRECTION ( 'NONE',  ( -0.000000000000000000, -0.000000000000000000, -1.000000000000000000 ) ) ;
#61612=VERTEX_POINT ( 'NONE', #7642 ) ;
#61613=EDGE_CURVE ( 'NONE', #3310, #19106, #15697, .T. ) ;
#61614=EDGE_CURVE ( 'NONE', #64143, #13395, #10858, .T. ) ;
#61615=CIRCLE ( 'NONE', #4300, 5.000000000000000888 ) ;
#61616=CARTESIAN_POINT ( 'NONE',  ( 35.00000000000000000, 11.35427606708806003, -4.426194442447284771 ) ) ;
#61618=VERTEX_POINT ( 'NONE', #48869 ) ;
#61624=CARTESIAN_POINT ( 'NONE',  ( 36.00000000000000711, -4.983891302653661981, -11.73555825188274682 ) ) ;
#61626=CARTESIAN_POINT ( 'NONE',  ( 10.47337281987918267, 7.645786758740480415, 9.252117967043277602 ) ) ;
#61632=ORIENTED_EDGE ( 'NONE', *, *, #13397, .T. ) ;
#61633=DIRECTION ( 'NONE',  ( 0.000000000000000000, -0.01356324068817998940, 0.9999080150203990547 ) ) ;
#61634=AXIS2_PLACEMENT_3D ( 'NONE', #59685, #33738, #27775 ) ;
#61635=ORIENTED_EDGE ( 'NONE', *, *, #41975, .T. ) ;
#61636=CARTESIAN_POINT ( 'NONE',  ( 37.00000000000000711, -5.672855678558609505, 10.28547182238013669 ) ) ;
#61637=ORIENTED_EDGE ( 'NONE', *, *, #47403, .F. ) ;
#61638=ORIENTED_EDGE ( 'NONE', *, *, #62730, .T. ) ;
#61641=EDGE_CURVE ( 'NONE', #51910, #55560, #29981, .T. ) ;
#61642=DIRECTION ( 'NONE',  ( 1.000000000000000000, 0.000000000000000000, 0.000000000000000000 ) ) ;
#61644=EDGE_LOOP ( 'NONE', ( #5853, #22797, #39441, #61144 ) ) ;
#61645=CIRCLE ( 'NONE', #38235, 12.18649999999999878 ) ;
#61647=AXIS2_PLACEMENT_3D ( 'NONE', #49861, #34227, #38904 ) ;
#61648=CARTESIAN_POINT ( 'NONE',  ( 10.48620311856346454, 8.250315036047107142, 8.713914264323181058 ) ) ;
#61649=CARTESIAN_POINT ( 'NONE',  ( -17.97077823246242900, -9.629623312810577929, -9.462431742398621282 ) ) ;
#61650=VERTEX_POINT ( 'NONE', #44498 ) ;
#61651=EDGE_CURVE ( 'NONE', #18427, #29827, #13286, .T. ) ;
#61654=VERTEX_POINT ( 'NONE', #53544 ) ;
#61655=ORIENTED_EDGE ( 'NONE', *, *, #10751, .T. ) ;
#61656=DIRECTION ( 'NONE',  ( 0.000000000000000000, 0.9903235168508544017, 0.1387779952735853917 ) ) ;
#61659=CARTESIAN_POINT ( 'NONE',  ( -21.17861794710831091, -13.00977982294134883, -3.604945070120774808 ) ) ;
#61661=AXIS2_PLACEMENT_3D ( 'NONE', #49639, #4079, #14369 ) ;
#61666=VERTEX_POINT ( 'NONE', #39191 ) ;
#61668=CIRCLE ( 'NONE', #18165, 4.999999999999999112 ) ;
#61669=FACE_OUTER_BOUND ( 'NONE', #38985, .T. ) ;
#61671=CIRCLE ( 'NONE', #29820, 12.74999999999999822 ) ;
#61673=CARTESIAN_POINT ( 'NONE',  ( 24.39765525450732753, -1.078022420954182437, -13.46171517445628041 ) ) ;
#61676=AXIS2_PLACEMENT_3D ( 'NONE', #11172, #62666, #46417 ) ;
#61677=EDGE_LOOP ( 'NONE', ( #905, #50966, #51819, #4918 ) ) ;
#61678=DIRECTION ( 'NONE',  ( 0.000000000000000000, -0.01356324068817998940, 0.9999080150203990547 ) ) ;
#61680=CARTESIAN_POINT ( 'NONE',  ( 35.00000000000000000, 5.927257550915316919, -10.64792938439757641 ) ) ;
#61681=VECTOR ( 'NONE', #3831, 1000.000000000000000 ) ;
#61687=ORIENTED_EDGE ( 'NONE', *, *, #34777, .T. ) ;
#61688=LINE ( 'NONE', #36429, #31236 ) ;
#61689=DIRECTION ( 'NONE',  ( 0.000000000000000000, -0.1387779952735886391, 0.9903235168508540687 ) ) ;
#61691=EDGE_LOOP ( 'NONE', ( #57641, #44287, #47636, #49411 ) ) ;
#61692=CARTESIAN_POINT ( 'NONE',  ( -28.85619398320021745, 3.750539801530000439, -12.96855624952673836 ) ) ;
#61693=DIRECTION ( 'NONE',  ( -1.000000000000000000, 0.000000000000000000, -0.000000000000000000 ) ) ;
#61696=FACE_OUTER_BOUND ( 'NONE', #1320, .T. ) ;
#61698=DIRECTION ( 'NONE',  ( 1.000000000000000000, -0.000000000000000000, -0.000000000000000000 ) ) ;
#61700=CIRCLE ( 'NONE', #53277, 12.75000000000000178 ) ;
#61702=ORIENTED_EDGE ( 'NONE', *, *, #22467, .T. ) ;
#61703=AXIS2_PLACEMENT_3D ( 'NONE', #62825, #52556, #57535 ) ;
#61704=DIRECTION ( 'NONE',  ( 0.000000000000000000, -0.3218879778916040602, 0.9467777615094549182 ) ) ;
#61705=CARTESIAN_POINT ( 'NONE',  ( -37.00000000000000711, 0.000000000000000000, 0.000000000000000000 ) ) ;
#61706=CARTESIAN_POINT ( 'NONE',  ( 24.18338352651159084, -2.157158703131657695, -11.80984941100301810 ) ) ;
#61708=CARTESIAN_POINT ( 'NONE',  ( -9.632141019976685925, 11.15750179195580394, -4.437120446396224160 ) ) ;
#61710=DIRECTION ( 'NONE',  ( -1.000000000000000000, 0.000000000000000000, 0.000000000000000000 ) ) ;
#61711=CARTESIAN_POINT ( 'NONE',  ( -37.00000000000000711, -7.110831038798204773, -9.896810808925470937 ) ) ;
#61714=CARTESIAN_POINT ( 'NONE',  ( 37.00000000000000711, 11.30684963584395675, 4.545979934229284147 ) ) ;
#61716=EDGE_LOOP ( 'NONE', ( #22578, #41193, #20747, #15599 ) ) ;
#61718=CARTESIAN_POINT ( 'NONE',  ( -35.00000000000000000, 12.09831040184926287, -1.463443770872647542 ) ) ;
#61720=CARTESIAN_POINT ( 'NONE',  ( -18.06493064879303034, 4.742646137938961282, 11.02526057695991923 ) ) ;
#61722=ORIENTED_EDGE ( 'NONE', *, *, #44579, .T. ) ;
#61725=DIRECTION ( 'NONE',  ( -0.000000000000000000, -1.000000000000000000, -0.000000000000000000 ) ) ;
#61728=CARTESIAN_POINT ( 'NONE',  ( 29.14505760361227260, -8.530938414384094060, 10.47125003768023888 ) ) ;
#61729=AXIS2_PLACEMENT_3D ( 'NONE', #21579, #36850, #51835 ) ;
#61731=CARTESIAN_POINT ( 'NONE',  ( 22.48820342141346984, -10.66318017514404914, -5.515879813209774163 ) ) ;
#61732=DIRECTION ( 'NONE',  ( -1.000000000000000000, 0.000000000000000000, 0.000000000000000000 ) ) ;
#61733=DIRECTION ( 'NONE',  ( -1.000000000000000000, 0.000000000000000000, 0.000000000000000000 ) ) ;
#61736=AXIS2_PLACEMENT_3D ( 'NONE', #32168, #11892, #1931 ) ;
#61737=AXIS2_PLACEMENT_3D ( 'NONE', #30751, #20472, #65666 ) ;
#61739=CARTESIAN_POINT ( 'NONE',  ( 35.00000000000000000, 8.017674001891782254, -9.913596905230143363 ) ) ;
#61742=ORIENTED_EDGE ( 'NONE', *, *, #29003, .F. ) ;
#61746=CARTESIAN_POINT ( 'NONE',  ( -27.22214261968804294, 12.41558776886551740, 5.304269109247361058 ) ) ;
#61748=DIRECTION ( 'NONE',  ( 1.000000000000000000, 0.000000000000000000, 0.000000000000000000 ) ) ;
#61749=CARTESIAN_POINT ( 'NONE',  ( 35.00000000000000000, -11.54110654723647400, 2.185196060784003524 ) ) ;
#61750=DIRECTION ( 'NONE',  ( -1.000000000000000000, 0.000000000000000000, 0.000000000000000000 ) ) ;
#61752=ORIENTED_EDGE ( 'NONE', *, *, #27654, .F. ) ;
#61756=EDGE_CURVE ( 'NONE', #10568, #55595, #14254, .T. ) ;
#61757=ORIENTED_EDGE ( 'NONE', *, *, #50336, .F. ) ;
#61758=EDGE_CURVE ( 'NONE', #31935, #38476, #20566, .T. ) ;
#61761=AXIS2_PLACEMENT_3D ( 'NONE', #62607, #12079, #42647 ) ;
#61763=EDGE_CURVE ( 'NONE', #58057, #38611, #32213, .T. ) ;
#61765=VERTEX_POINT ( 'NONE', #54833 ) ;
#61767=CARTESIAN_POINT ( 'NONE',  ( 12.47628546223243617, 0.000000000000000000, 11.99999999999999645 ) ) ;
#61769=FACE_OUTER_BOUND ( 'NONE', #33536, .T. ) ;
#61771=EDGE_CURVE ( 'NONE', #63912, #33199, #5270, .T. ) ;
#61772=CARTESIAN_POINT ( 'NONE',  ( 12.10998784662220729, -8.443435280036764468, -8.526922110106905706 ) ) ;
#61773=AXIS2_PLACEMENT_3D ( 'NONE', #49984, #46237, #9088 ) ;
#61774=CYLINDRICAL_SURFACE ( 'NONE', #20209, 12.18650000000000055 ) ;
#61776=DIRECTION ( 'NONE',  ( 1.000000000000000000, -0.000000000000000000, 0.000000000000000000 ) ) ;
#61777=ORIENTED_EDGE ( 'NONE', *, *, #45712, .F. ) ;
#61778=DIRECTION ( 'NONE',  ( 1.000000000000000000, 0.000000000000000000, 0.000000000000000000 ) ) ;
#61779=DIRECTION ( 'NONE',  ( 0.000000000000000000, -0.01356324068817998940, 0.9999080150203990547 ) ) ;
#61780=CARTESIAN_POINT ( 'NONE',  ( -47.00000000000000711, 0.000000000000000000, 0.000000000000000000 ) ) ;
#61781=DIRECTION ( 'NONE',  ( 0.000000000000000000, -0.01356324068817999114, 0.9999080150203989437 ) ) ;
#61783=CARTESIAN_POINT ( 'NONE',  ( -10.66894337560421135, -5.799424265809170365, 10.51297739570658685 ) ) ;
#61784=AXIS2_PLACEMENT_3D ( 'NONE', #64082, #34135, #34471 ) ;
#61785=AXIS2_PLACEMENT_3D ( 'NONE', #14729, #55661, #14416 ) ;
#61786=ORIENTED_EDGE ( 'NONE', *, *, #26763, .T. ) ;
#61787=ORIENTED_EDGE ( 'NONE', *, *, #6592, .T. ) ;
#61790=EDGE_LOOP ( 'NONE', ( #42695, #58912, #22656, #17363 ) ) ;
#61792=DIRECTION ( 'NONE',  ( 1.000000000000000000, -0.000000000000000000, -0.000000000000000000 ) ) ;
#61793=CYLINDRICAL_SURFACE ( 'NONE', #59657, 6.842778212674966554 ) ;
#61795=CARTESIAN_POINT ( 'NONE',  ( -37.00000000000000711, 11.67026961469348123, 4.564151185897115326 ) ) ;
#61796=CARTESIAN_POINT ( 'NONE',  ( 10.57504247840391010, 8.113525156875745381, -8.843426623829302002 ) ) ;
#61797=DIRECTION ( 'NONE',  ( -1.000000000000000000, -0.000000000000000000, 0.000000000000000000 ) ) ;
#61800=VERTEX_POINT ( 'NONE', #19256 ) ;
#61801=AXIS2_PLACEMENT_3D ( 'NONE', #62618, #27710, #52682 ) ;
#61803=DIRECTION ( 'NONE',  ( 0.000000000000000000, -0.01356324068817991481, 0.9999080150203990547 ) ) ;
#61805=AXIS2_PLACEMENT_3D ( 'NONE', #41976, #36335, #25713 ) ;
#61808=VERTEX_POINT ( 'NONE', #29534 ) ;
#61809=CARTESIAN_POINT ( 'NONE',  ( 37.00000000000000711, 4.705694406421931860E-17, -3.469127814946512892E-15 ) ) ;
#61811=DIRECTION ( 'NONE',  ( 0.000000000000000000, -0.04924826701375277505, -0.9987865678893272925 ) ) ;
#61814=CIRCLE ( 'NONE', #25704, 5.000000000000000000 ) ;
#61815=ORIENTED_EDGE ( 'NONE', *, *, #11066, .F. ) ;
#61816=DIRECTION ( 'NONE',  ( -1.000000000000000000, 0.000000000000000000, 0.000000000000000000 ) ) ;
#61820=ORIENTED_EDGE ( 'NONE', *, *, #5335, .T. ) ;
#61821=ORIENTED_EDGE ( 'NONE', *, *, #816, .F. ) ;
#61825=EDGE_CURVE ( 'NONE', #5002, #56493, #16177, .T. ) ;
#61826=DIRECTION ( 'NONE',  ( 0.000000000000000000, 0.7790879021242528291, -0.6269146997507959451 ) ) ;
#61828=CARTESIAN_POINT ( 'NONE',  ( 37.00000000000000711, 12.02534193257720574, -4.237174932027271801 ) ) ;
#61831=VECTOR ( 'NONE', #57522, 1000.000000000000000 ) ;
#61832=VERTEX_POINT ( 'NONE', #7212 ) ;
#61833=DIRECTION ( 'NONE',  ( 0.000000000000000000, 0.01356324068818000848, -0.9999080150203990547 ) ) ;
#61834=CARTESIAN_POINT ( 'NONE',  ( -3.515176343547850468, 10.77627674567199634, 8.139927681337322696 ) ) ;
#61838=CARTESIAN_POINT ( 'NONE',  ( 35.00000000000000000, 4.705694406421931860E-17, -3.469127814946512892E-15 ) ) ;
#61839=AXIS2_PLACEMENT_3D ( 'NONE', #43464, #34145, #49152 ) ;
#61840=CIRCLE ( 'NONE', #33164, 5.000000000000001776 ) ;
#61842=EDGE_LOOP ( 'NONE', ( #4249, #5977, #49575, #42550 ) ) ;
#61843=CARTESIAN_POINT ( 'NONE',  ( -18.08686583997218733, 5.151216734910788908, -10.83812558286602012 ) ) ;
#61844=ORIENTED_EDGE ( 'NONE', *, *, #34060, .T. ) ;
#61845=EDGE_CURVE ( 'NONE', #31785, #13407, #10911, .T. ) ;
#61850=EDGE_CURVE ( 'NONE', #63179, #53475, #47476, .T. ) ;
#61856=DIRECTION ( 'NONE',  ( 0.000000000000000000, -0.01356324068817998940, 0.9999080150203990547 ) ) ;
#61857=CIRCLE ( 'NONE', #39537, 12.18649999999999878 ) ;
#61858=AXIS2_PLACEMENT_3D ( 'NONE', #18858, #13836, #64708 ) ;
#61861=CIRCLE ( 'NONE', #49118, 5.000000000000000000 ) ;
#61862=ADVANCED_FACE ( 'NONE', ( #41470 ), #36507, .T. ) ;
#61867=EDGE_CURVE ( 'NONE', #26214, #32335, #33222, .T. ) ;
#61870=EDGE_CURVE ( 'NONE', #58250, #21512, #32156, .T. ) ;
#61871=CIRCLE ( 'NONE', #7723, 12.75000000000000178 ) ;
#61872=ORIENTED_EDGE ( 'NONE', *, *, #63421, .T. ) ;
#61877=LINE ( 'NONE', #6358, #43473 ) ;
#61879=AXIS2_PLACEMENT_3D ( 'NONE', #44670, #64961, #25389 ) ;
#61880=AXIS2_PLACEMENT_3D ( 'NONE', #53226, #17324, #7673 ) ;
#61881=ORIENTED_EDGE ( 'NONE', *, *, #16548, .F. ) ;
#61883=DIRECTION ( 'NONE',  ( -1.000000000000000000, 0.000000000000000000, 0.000000000000000000 ) ) ;
#61886=VECTOR ( 'NONE', #4399, 1000.000000000000000 ) ;
#61887=ORIENTED_EDGE ( 'NONE', *, *, #51322, .F. ) ;
#61889=CARTESIAN_POINT ( 'NONE',  ( 36.00000000000000711, 6.265926637539650734, 11.10408318471052347 ) ) ;
#61890=ORIENTED_EDGE ( 'NONE', *, *, #2408, .T. ) ;
#61891=CARTESIAN_POINT ( 'NONE',  ( -19.47984447937493613, -3.750539801530005768, 25.00000000000000000 ) ) ;
#61893=CARTESIAN_POINT ( 'NONE',  ( 24.85820284700998428, 0.06691071362158636238, 12.00631040446440778 ) ) ;
#61894=VERTEX_POINT ( 'NONE', #61767 ) ;
#61896=ORIENTED_EDGE ( 'NONE', *, *, #37899, .T. ) ;
#61898=VECTOR ( 'NONE', #50734, 1000.000000000000000 ) ;
#61901=AXIS2_PLACEMENT_3D ( 'NONE', #42217, #21967, #7311 ) ;
#61902=CARTESIAN_POINT ( 'NONE',  ( 37.00000000000000711, -6.475373545682373333, -10.32377448871666026 ) ) ;
#61903=ADVANCED_FACE ( 'NONE', ( #16225 ), #16872, .T. ) ;
#61904=ADVANCED_FACE ( 'NONE', ( #62109 ), #61429, .T. ) ;
#61905=CARTESIAN_POINT ( 'NONE',  ( 35.00000000000000000, -1.903127969211267700, -11.59095880812007628 ) ) ;
#61907=LINE ( 'NONE', #32938, #17530 ) ;
#61909=VERTEX_POINT ( 'NONE', #27182 ) ;
#61910=DIRECTION ( 'NONE',  ( -1.000000000000000000, -0.000000000000000000, 0.000000000000000000 ) ) ;
#61911=EDGE_LOOP ( 'NONE', ( #16268, #57055, #59130, #10816 ) ) ;
#61913=AXIS2_PLACEMENT_3D ( 'NONE', #54062, #38433, #8496 ) ;
#61914=DIRECTION ( 'NONE',  ( 0.000000000000000000, -0.01356324068817999114, 0.9999080150203989437 ) ) ;
#61915=ORIENTED_EDGE ( 'NONE', *, *, #64676, .F. ) ;
#61917=DIRECTION ( 'NONE',  ( -1.000000000000000000, 0.000000000000000000, 0.000000000000000000 ) ) ;
#61919=CARTESIAN_POINT ( 'NONE',  ( 35.00000000000000000, -10.91072401419414462, -5.428340790341669830 ) ) ;
#61920=CARTESIAN_POINT ( 'NONE',  ( -37.00000000000000711, 0.000000000000000000, 0.000000000000000000 ) ) ;
#61922=CIRCLE ( 'NONE', #57709, 12.74999999999999822 ) ;
#61923=EDGE_CURVE ( 'NONE', #21512, #16453, #36829, .T. ) ;
#61924=ORIENTED_EDGE ( 'NONE', *, *, #43667, .F. ) ;
#61925=CARTESIAN_POINT ( 'NONE',  ( -18.87381964659587297, -4.101229939362269761, -11.27785301288100506 ) ) ;
#61927=CARTESIAN_POINT ( 'NONE',  ( 35.00000000000000000, 11.59605747147793586, 5.300372733891518529 ) ) ;
#61928=DIRECTION ( 'NONE',  ( 0.000000000000000000, 0.7196168960969767658, 0.6943713148249667233 ) ) ;
#61931=ORIENTED_EDGE ( 'NONE', *, *, #61771, .F. ) ;
#61933=VECTOR ( 'NONE', #42828, 1000.000000000000000 ) ;
#61935=AXIS2_PLACEMENT_3D ( 'NONE', #11468, #12440, #18110 ) ;
#61936=CIRCLE ( 'NONE', #55585, 5.000000000000000888 ) ;
#61938=DIRECTION ( 'NONE',  ( 0.000000000000000000, 0.01356324068817991828, -0.9999080150203990547 ) ) ;
#61941=AXIS2_PLACEMENT_3D ( 'NONE', #5344, #40579, #36232 ) ;
#61944=ADVANCED_FACE ( 'NONE', ( #47159 ), #1608, .T. ) ;
#61945=CARTESIAN_POINT ( 'NONE',  ( 35.00000000000000000, 2.936739658819871313, -11.37311665002364869 ) ) ;
#61946=CARTESIAN_POINT ( 'NONE',  ( -37.00000000000000711, 0.000000000000000000, 0.000000000000000000 ) ) ;
#61949=EDGE_CURVE ( 'NONE', #34626, #33925, #42127, .T. ) ;
#61950=CIRCLE ( 'NONE', #53474, 12.74999999999999822 ) ;
#61951=ORIENTED_EDGE ( 'NONE', *, *, #33284, .T. ) ;
#61953=CARTESIAN_POINT ( 'NONE',  ( -15.92735611090874848, 7.887070990759704969, 10.95653452613623102 ) ) ;
#61954=DIRECTION ( 'NONE',  ( 1.000000000000000000, -0.000000000000000000, 0.000000000000000000 ) ) ;
#61957=CARTESIAN_POINT ( 'NONE',  ( 3.382263751109486627, 5.483660712610938681, -10.67588914012733348 ) ) ;
#61958=VECTOR ( 'NONE', #59153, 1000.000000000000000 ) ;
#61959=CARTESIAN_POINT ( 'NONE',  ( 37.00000000000000711, 11.61175578952788356, 1.771820996347031940 ) ) ;
#61961=EDGE_CURVE ( 'NONE', #12164, #49077, #62922, .T. ) ;
#61963=ORIENTED_EDGE ( 'NONE', *, *, #1884, .F. ) ;
#61964=CARTESIAN_POINT ( 'NONE',  ( -35.00000000000000000, -9.076753354954062658, 8.954052073409570767 ) ) ;
#61965=ORIENTED_EDGE ( 'NONE', *, *, #44726, .F. ) ;
#61967=CARTESIAN_POINT ( 'NONE',  ( 12.52750123246316072, 0.4973700281276248192, 25.00000000000000000 ) ) ;
#61968=VECTOR ( 'NONE', #61470, 1000.000000000000000 ) ;
#61969=ORIENTED_EDGE ( 'NONE', *, *, #16454, .T. ) ;
#61970=CARTESIAN_POINT ( 'NONE',  ( -25.56972390839818843, -10.04380371306811881, 6.568580827850054149 ) ) ;
#61973=DIRECTION ( 'NONE',  ( 1.000000000000000000, 0.000000000000000000, 0.000000000000000000 ) ) ;
#61974=ORIENTED_EDGE ( 'NONE', *, *, #58044, .T. ) ;
#61978=DIRECTION ( 'NONE',  ( 0.000000000000000000, -0.4698238015817237101, -0.8827602140260384367 ) ) ;
#61979=ORIENTED_EDGE ( 'NONE', *, *, #31470, .F. ) ;
#61980=CARTESIAN_POINT ( 'NONE',  ( -28.07033260158857857, 9.867324763291481560, -6.836013876802826239 ) ) ;
#61981=VERTEX_POINT ( 'NONE', #54435 ) ;
#61982=AXIS2_PLACEMENT_3D ( 'NONE', #22098, #53358, #27096 ) ;
#61983=DIRECTION ( 'NONE',  ( 0.000000000000000000, -0.9970832820307047317, -0.07632122047555414679 ) ) ;
#61985=ORIENTED_EDGE ( 'NONE', *, *, #3729, .F. ) ;
#61987=CARTESIAN_POINT ( 'NONE',  ( -35.00000000000000000, 0.000000000000000000, 0.000000000000000000 ) ) ;
#61988=AXIS2_PLACEMENT_3D ( 'NONE', #40935, #62193, #25636 ) ;
#61991=EDGE_CURVE ( 'NONE', #2019, #18023, #22602, .T. ) ;
#61993=CARTESIAN_POINT ( 'NONE',  ( -35.00000000000000000, -11.70009620280410978, -1.039216533673027243 ) ) ;
#61995=ORIENTED_EDGE ( 'NONE', *, *, #3771, .T. ) ;
#61996=EDGE_CURVE ( 'NONE', #30317, #35454, #28478, .T. ) ;
#61998=DIRECTION ( 'NONE',  ( -1.000000000000000000, 0.000000000000000000, 0.000000000000000000 ) ) ;
#61999=ORIENTED_EDGE ( 'NONE', *, *, #56532, .F. ) ;
#62000=VECTOR ( 'NONE', #35505, 1000.000000000000000 ) ;
#62001=ORIENTED_EDGE ( 'NONE', *, *, #49275, .T. ) ;
#62002=CIRCLE ( 'NONE', #38644, 4.999999999999999112 ) ;
#62008=CARTESIAN_POINT ( 'NONE',  ( 35.00000000000000000, 4.705694406421931860E-17, -3.469127814946512892E-15 ) ) ;
#62009=CIRCLE ( 'NONE', #54619, 5.000000000000000000 ) ;
#62011=DIRECTION ( 'NONE',  ( -1.000000000000000000, -0.000000000000000000, 0.000000000000000000 ) ) ;
#62012=DIRECTION ( 'NONE',  ( 0.000000000000000000, 0.01356324068817998940, -0.9999080150203990547 ) ) ;
#62015=DIRECTION ( 'NONE',  ( 1.000000000000000000, 0.000000000000000000, 0.000000000000000000 ) ) ;
#62016=EDGE_CURVE ( 'NONE', #53424, #33400, #40668, .T. ) ;
#62018=CARTESIAN_POINT ( 'NONE',  ( 12.47628546223243617, 0.000000000000000000, -11.99999999999998224 ) ) ;
#62019=CIRCLE ( 'NONE', #35471, 12.18650000000000055 ) ;
#62021=DIRECTION ( 'NONE',  ( 0.000000000000000000, -0.01356324068817991828, 0.9999080150203990547 ) ) ;
#62022=CARTESIAN_POINT ( 'NONE',  ( 2.750171585628739646, 2.206612499183723486, -11.80217412294446788 ) ) ;
#62024=EDGE_LOOP ( 'NONE', ( #6233, #21548, #44232, #10027 ) ) ;
#62028=LINE ( 'NONE', #42359, #49198 ) ;
#62029=CIRCLE ( 'NONE', #56736, 12.18649999999999878 ) ;
#62030=LINE ( 'NONE', #61680, #54566 ) ;
#62031=EDGE_CURVE ( 'NONE', #42381, #53925, #30034, .T. ) ;
#62034=CARTESIAN_POINT ( 'NONE',  ( -25.37693896798699456, -11.65917517926966873, 6.807023274763674081 ) ) ;
#62035=ORIENTED_EDGE ( 'NONE', *, *, #31704, .F. ) ;
#62036=DIRECTION ( 'NONE',  ( 0.000000000000000000, -0.01356324068817998940, 0.9999080150203990547 ) ) ;
#62037=CARTESIAN_POINT ( 'NONE',  ( -27.41041641377506011, -11.32519648962278680, -7.368711486028817426 ) ) ;
#62039=ORIENTED_EDGE ( 'NONE', *, *, #13856, .F. ) ;
#62040=EDGE_CURVE ( 'NONE', #42133, #32028, #13138, .T. ) ;
#62042=CARTESIAN_POINT ( 'NONE',  ( -17.31450763390795800, 7.097772087455203938, -9.677943051329000568 ) ) ;
#62043=FACE_OUTER_BOUND ( 'NONE', #30562, .T. ) ;
#62044=CIRCLE ( 'NONE', #18543, 4.999999999999999112 ) ;
#62045=CARTESIAN_POINT ( 'NONE',  ( -37.00000000000000711, 0.000000000000000000, 0.000000000000000000 ) ) ;
#62046=VERTEX_POINT ( 'NONE', #202 ) ;
#62048=CIRCLE ( 'NONE', #33381, 12.74999999999999822 ) ;
#62049=AXIS2_PLACEMENT_3D ( 'NONE', #53528, #48529, #31891 ) ;
#62050=LINE ( 'NONE', #20163, #20180 ) ;
#62051=VERTEX_POINT ( 'NONE', #15148 ) ;
#62053=DIRECTION ( 'NONE',  ( -1.000000000000000000, 0.000000000000000000, -0.000000000000000000 ) ) ;
#62055=DIRECTION ( 'NONE',  ( 0.000000000000000000, -0.01356324068817992001, 0.9999080150203990547 ) ) ;
#62056=CARTESIAN_POINT ( 'NONE',  ( 37.00000000000000711, 4.705694406421931860E-17, -3.469127814946512892E-15 ) ) ;
#62057=AXIS2_PLACEMENT_3D ( 'NONE', #48983, #34315, #38663 ) ;
#62058=LINE ( 'NONE', #36777, #6854 ) ;
#62060=ORIENTED_EDGE ( 'NONE', *, *, #64602, .F. ) ;
#62061=VERTEX_POINT ( 'NONE', #59736 ) ;
#62062=CARTESIAN_POINT ( 'NONE',  ( 23.19458397200137867, -4.581538694898370068, -11.09407635438899931 ) ) ;
#62067=AXIS2_PLACEMENT_3D ( 'NONE', #27911, #2671, #47864 ) ;
#62068=DIRECTION ( 'NONE',  ( 1.000000000000000000, 0.000000000000000000, 0.000000000000000000 ) ) ;
#62070=DIRECTION ( 'NONE',  ( 0.000000000000000000, -0.01356324068817998940, 0.9999080150203990547 ) ) ;
#62071=ADVANCED_FACE ( 'NONE', ( #65360 ), #49755, .T. ) ;
#62073=FACE_OUTER_BOUND ( 'NONE', #14319, .T. ) ;
#62074=ORIENTED_EDGE ( 'NONE', *, *, #8811, .F. ) ;
#62076=ORIENTED_EDGE ( 'NONE', *, *, #50688, .F. ) ;
#62078=AXIS2_PLACEMENT_3D ( 'NONE', #27360, #63263, #6124 ) ;
#62079=ORIENTED_EDGE ( 'NONE', *, *, #21995, .F. ) ;
#62080=DIRECTION ( 'NONE',  ( -1.000000000000000000, 0.000000000000000000, -0.000000000000000000 ) ) ;
#62081=CARTESIAN_POINT ( 'NONE',  ( 9.105023507364348845, 3.304801514924585959, 13.09129911384226652 ) ) ;
#62082=DIRECTION ( 'NONE',  ( -1.000000000000000000, -0.000000000000000000, 0.000000000000000000 ) ) ;
#62083=CARTESIAN_POINT ( 'NONE',  ( 9.687175622948609899, 13.48729812737144940, -0.5854820436212360146 ) ) ;
#62086=VERTEX_POINT ( 'NONE', #14799 ) ;
#62088=CARTESIAN_POINT ( 'NONE',  ( -35.00000000000000000, 4.237174932027226504, 12.02534193257722350 ) ) ;
#62089=ORIENTED_EDGE ( 'NONE', *, *, #56688, .T. ) ;
#62090=DIRECTION ( 'NONE',  ( 0.000000000000000000, 0.01356324068817992001, -0.9999080150203990547 ) ) ;
#62092=DIRECTION ( 'NONE',  ( 1.000000000000000000, -0.000000000000000000, 0.000000000000000000 ) ) ;
#62093=LINE ( 'NONE', #601, #4089 ) ;
#62095=CARTESIAN_POINT ( 'NONE',  ( -36.00000000000000711, 11.73555825188283741, -4.983891302653458588 ) ) ;
#62096=CARTESIAN_POINT ( 'NONE',  ( 36.00000000000000711, -12.38385022362083987, -3.033604067594536602 ) ) ;
#62097=EDGE_CURVE ( 'NONE', #14797, #63500, #16105, .T. ) ;
#62100=ORIENTED_EDGE ( 'NONE', *, *, #37821, .F. ) ;
#62102=ORIENTED_EDGE ( 'NONE', *, *, #61174, .F. ) ;
#62103=FACE_OUTER_BOUND ( 'NONE', #41049, .T. ) ;
#62104=DIRECTION ( 'NONE',  ( 0.000000000000000000, 0.9999080150203989437, 0.01356324068818338426 ) ) ;
#62107=ORIENTED_EDGE ( 'NONE', *, *, #45736, .F. ) ;
#62109=FACE_OUTER_BOUND ( 'NONE', #31478, .T. ) ;
#62110=CARTESIAN_POINT ( 'NONE',  ( -37.00000000000000711, 0.000000000000000000, 0.000000000000000000 ) ) ;
#62111=LINE ( 'NONE', #16563, #4109 ) ;
#62112=EDGE_CURVE ( 'NONE', #8415, #27274, #17281, .T. ) ;
#62113=DIRECTION ( 'NONE',  ( 1.000000000000000000, -0.000000000000000000, 0.000000000000000000 ) ) ;
#62115=VERTEX_POINT ( 'NONE', #10164 ) ;
#62116=DIRECTION ( 'NONE',  ( 1.000000000000000000, -0.000000000000000000, 0.000000000000000000 ) ) ;
#62121=CARTESIAN_POINT ( 'NONE',  ( 28.46403053133689198, -10.24654051476648497, 6.260428664560219403 ) ) ;
#62122=CARTESIAN_POINT ( 'NONE',  ( -8.606002450955907435, -2.738469685186787128, 11.68403320950772795 ) ) ;
#62124=ORIENTED_EDGE ( 'NONE', *, *, #20439, .T. ) ;
#62125=ORIENTED_EDGE ( 'NONE', *, *, #59614, .F. ) ;
#62126=DIRECTION ( 'NONE',  ( 0.000000000000000000, -0.9467777615094604693, -0.3218879778915875178 ) ) ;
#62127=ORIENTED_EDGE ( 'NONE', *, *, #41972, .T. ) ;
#62128=CARTESIAN_POINT ( 'NONE',  ( 3.425926600331120397, 5.853248163474676247, 10.47781994178590104 ) ) ;
#62129=DIRECTION ( 'NONE',  ( -1.000000000000000000, 0.000000000000000000, 0.000000000000000000 ) ) ;
#62134=CARTESIAN_POINT ( 'NONE',  ( -35.00000000000000000, -0.7008968033237865658, -12.16632754454237819 ) ) ;
#62136=ORIENTED_EDGE ( 'NONE', *, *, #32286, .T. ) ;
#62137=FACE_OUTER_BOUND ( 'NONE', #37762, .T. ) ;
#62138=ORIENTED_EDGE ( 'NONE', *, *, #60284, .T. ) ;
#62139=DIRECTION ( 'NONE',  ( 0.000000000000000000, -0.7196168960969868689, -0.6943713148249562872 ) ) ;
#62140=DIRECTION ( 'NONE',  ( 1.000000000000000000, 0.000000000000000000, 0.000000000000000000 ) ) ;
#62142=DIRECTION ( 'NONE',  ( 0.000000000000000000, 0.2960891610144441022, 0.9551603052523501836 ) ) ;
#62143=ORIENTED_EDGE ( 'NONE', *, *, #16605, .T. ) ;
#62144=CARTESIAN_POINT ( 'NONE',  ( -35.00000000000000000, -10.80478261802186246, 5.636262487437281976 ) ) ;
#62149=ORIENTED_EDGE ( 'NONE', *, *, #33094, .T. ) ;
#62150=CARTESIAN_POINT ( 'NONE',  ( 0.6705955404150230059, 0.5055564190250056988, 13.49364205544756423 ) ) ;
#62153=DIRECTION ( 'NONE',  ( 0.000000000000000000, 0.01356324068817998940, -0.9999080150203990547 ) ) ;
#62154=ORIENTED_EDGE ( 'NONE', *, *, #40016, .T. ) ;
#62155=VERTEX_POINT ( 'NONE', #9832 ) ;
#62156=ORIENTED_EDGE ( 'NONE', *, *, #36258, .T. ) ;
#62159=VECTOR ( 'NONE', #18697, 1000.000000000000000 ) ;
#62160=CARTESIAN_POINT ( 'NONE',  ( -20.74858375370908803, -11.60713604139673905, -3.059550090777561682 ) ) ;
#62161=CARTESIAN_POINT ( 'NONE',  ( -35.00000000000000000, 9.430788938294162094, -7.718225330433707398 ) ) ;
#62163=CYLINDRICAL_SURFACE ( 'NONE', #26355, 5.000000000000000888 ) ;
#62165=CARTESIAN_POINT ( 'NONE',  ( 37.00000000000000711, 11.71932350927024657, -3.511386971104992760 ) ) ;
#62167=CARTESIAN_POINT ( 'NONE',  ( -10.64311535907470230, -9.781890035361625380, -9.304428041637391900 ) ) ;
#62168=CARTESIAN_POINT ( 'NONE',  ( -2.798074428798408952, 8.529348309608609568, 10.48748355420409339 ) ) ;
#62173=CARTESIAN_POINT ( 'NONE',  ( -27.45775109278351067, 25.00000000000000000, -1.989333891161980894 ) ) ;
#62176=DIRECTION ( 'NONE',  ( -1.000000000000000000, -0.000000000000000000, 0.000000000000000000 ) ) ;
#62182=DIRECTION ( 'NONE',  ( -1.000000000000000000, 0.000000000000000000, 0.000000000000000000 ) ) ;
#62184=ORIENTED_EDGE ( 'NONE', *, *, #63224, .F. ) ;
#62185=CARTESIAN_POINT ( 'NONE',  ( 37.00000000000000711, 4.705694406421931860E-17, -3.469127814946512892E-15 ) ) ;
#62187=CARTESIAN_POINT ( 'NONE',  ( 35.00000000000000000, -11.50504120060945645, -4.018060380616356397 ) ) ;
#62189=CIRCLE ( 'NONE', #4861, 12.18649999999999878 ) ;
#62190=CYLINDRICAL_SURFACE ( 'NONE', #20160, 12.74999999999999822 ) ;
#62193=DIRECTION ( 'NONE',  ( 1.000000000000000000, 0.000000000000000000, 0.000000000000000000 ) ) ;
#62194=EDGE_CURVE ( 'NONE', #40279, #36481, #6697, .T. ) ;
#62195=ORIENTED_EDGE ( 'NONE', *, *, #41562, .F. ) ;
#62196=VERTEX_POINT ( 'NONE', #40411 ) ;
#62197=CARTESIAN_POINT ( 'NONE',  ( -37.00000000000000711, 1.113475361586490298, 12.70128625845193326 ) ) ;
#62199=CYLINDRICAL_SURFACE ( 'NONE', #53457, 4.500030059823568074 ) ;
#62200=DIRECTION ( 'NONE',  ( 1.000000000000000000, 0.000000000000000000, 0.000000000000000000 ) ) ;
#62201=ORIENTED_EDGE ( 'NONE', *, *, #13856, .T. ) ;
#62202=ORIENTED_EDGE ( 'NONE', *, *, #2832, .F. ) ;
#62204=CARTESIAN_POINT ( 'NONE',  ( 37.00000000000000711, 10.49591321039688019, 5.273331777780226659 ) ) ;
#62205=FACE_OUTER_BOUND ( 'NONE', #2674, .T. ) ;
#62206=EDGE_CURVE ( 'NONE', #44869, #11584, #8922, .T. ) ;
#62208=AXIS2_PLACEMENT_3D ( 'NONE', #32601, #52909, #36298 ) ;
#62209=CARTESIAN_POINT ( 'NONE',  ( 35.00000000000000000, 4.705694406421931860E-17, -3.469127814946512892E-15 ) ) ;
#62210=FACE_OUTER_BOUND ( 'NONE', #47681, .T. ) ;
#62214=EDGE_CURVE ( 'NONE', #29569, #39344, #34262, .T. ) ;
#62216=CYLINDRICAL_SURFACE ( 'NONE', #1692, 4.999999999999999112 ) ;
#62217=ORIENTED_EDGE ( 'NONE', *, *, #49756, .F. ) ;
#62218=DIRECTION ( 'NONE',  ( 1.000000000000000000, -0.000000000000000000, 0.000000000000000000 ) ) ;
#62220=EDGE_LOOP ( 'NONE', ( #64408, #54565, #48969, #22488 ) ) ;
#62222=ORIENTED_EDGE ( 'NONE', *, *, #55887, .F. ) ;
#62223=DIRECTION ( 'NONE',  ( -1.000000000000000000, 0.000000000000000000, -0.000000000000000000 ) ) ;
#62224=VECTOR ( 'NONE', #56698, 1000.000000000000000 ) ;
#62226=LINE ( 'NONE', #38254, #59145 ) ;
#62228=CARTESIAN_POINT ( 'NONE',  ( -35.00000000000000000, 0.000000000000000000, 0.000000000000000000 ) ) ;
#62229=EDGE_CURVE ( 'NONE', #21159, #29920, #37436, .T. ) ;
#62231=DIRECTION ( 'NONE',  ( 1.000000000000000000, -0.000000000000000000, 0.000000000000000000 ) ) ;
#62232=ORIENTED_EDGE ( 'NONE', *, *, #57795, .T. ) ;
#62233=CARTESIAN_POINT ( 'NONE',  ( -37.00000000000000711, 0.6593684648222315481, -12.73293890771482850 ) ) ;
#62235=DIRECTION ( 'NONE',  ( -1.000000000000000000, 0.000000000000000000, 0.000000000000000000 ) ) ;
#62237=CARTESIAN_POINT ( 'NONE',  ( 35.00000000000000000, 8.624332853796058629, -9.390600770288020982 ) ) ;
#62238=ORIENTED_EDGE ( 'NONE', *, *, #37897, .T. ) ;
#62239=B_SPLINE_CURVE_WITH_KNOTS ( 'NONE', 3,
 ( #56367, #37056, #1522, #6175, #57039, #52386, #41068, #17118, #12121, #46398, #32397, #31430, #36066, #42355, #51729, #1835, #26769, #56730 ),
 .UNSPECIFIED., .F., .F.,
 ( 4, 2, 2, 2, 2, 2, 2, 2, 4 ),
 ( 0.005052247689395389027, 0.005881123449897000116, 0.006709999210398609470, 0.007538874970900218825, 0.008367750731401828179, 0.009196626491903437534, 0.01002550225240504515, 0.01085437801290665451, 0.01168325377340826386 ),
 .UNSPECIFIED. ) ;
#62241=DIRECTION ( 'NONE',  ( 1.000000000000000000, -0.000000000000000000, 0.000000000000000000 ) ) ;
#62242=DIRECTION ( 'NONE',  ( -1.000000000000000000, 0.000000000000000000, -0.000000000000000000 ) ) ;
#62244=ORIENTED_EDGE ( 'NONE', *, *, #35527, .F. ) ;
#62245=ORIENTED_EDGE ( 'NONE', *, *, #18199, .T. ) ;
#62246=CARTESIAN_POINT ( 'NONE',  ( 36.00000000000000711, -9.733281772932102172, 8.235637554476744171 ) ) ;
#62247=EDGE_CURVE ( 'NONE', #29901, #41167, #42740, .T. ) ;
#62248=ORIENTED_EDGE ( 'NONE', *, *, #15879, .F. ) ;
#62250=EDGE_CURVE ( 'NONE', #43149, #39558, #53408, .T. ) ;
#62251=CARTESIAN_POINT ( 'NONE',  ( -37.00000000000000711, 11.72195762423408816, 0.7536123767500589876 ) ) ;
#62252=DIRECTION ( 'NONE',  ( 0.3509218304786018705, 0.9364047569793457759, 0.000000000000000000 ) ) ;
#62253=ORIENTED_EDGE ( 'NONE', *, *, #38267, .T. ) ;
#62255=CARTESIAN_POINT ( 'NONE',  ( -35.00000000000000000, -12.15823808070322087, -0.8294751490780611913 ) ) ;
#62256=CYLINDRICAL_SURFACE ( 'NONE', #11792, 5.000000000000000888 ) ;
#62257=CARTESIAN_POINT ( 'NONE',  ( 11.74548640120467979, 10.73597826697114677, -8.184666801472349817 ) ) ;
#62258=DIRECTION ( 'NONE',  ( -1.000000000000000000, 0.000000000000000000, 0.000000000000000000 ) ) ;
#62259=CYLINDRICAL_SURFACE ( 'NONE', #18200, 4.999999999999999112 ) ;
#62262=EDGE_CURVE ( 'NONE', #54132, #21703, #18380, .T. ) ;
#62263=ORIENTED_EDGE ( 'NONE', *, *, #31725, .T. ) ;
#62265=DIRECTION ( 'NONE',  ( 0.000000000000000000, 0.01356324068817998940, -0.9999080150203990547 ) ) ;
#62272=EDGE_CURVE ( 'NONE', #32962, #39957, #62028, .T. ) ;
#62273=DIRECTION ( 'NONE',  ( -1.000000000000000000, 0.000000000000000000, 0.000000000000000000 ) ) ;
#62275=EDGE_LOOP ( 'NONE', ( #45027, #42936, #5827, #31140 ) ) ;
#62277=ADVANCED_FACE ( 'NONE', ( #37061 ), #26440, .T. ) ;
#62278=EDGE_LOOP ( 'NONE', ( #51981, #64885, #51087, #60804 ) ) ;
#62281=DIRECTION ( 'NONE',  ( 0.000000000000000000, -0.01356324068817998940, 0.9999080150203990547 ) ) ;
#62289=CARTESIAN_POINT ( 'NONE',  ( 35.00000000000000000, 11.73463472867580393, 3.287724142101285274 ) ) ;
#62290=EDGE_CURVE ( 'NONE', #17119, #61052, #57633, .T. ) ;
#62291=VERTEX_POINT ( 'NONE', #6179 ) ;
#62292=DIRECTION ( 'NONE',  ( -1.000000000000000000, -0.000000000000000000, 0.000000000000000000 ) ) ;
#62293=ORIENTED_EDGE ( 'NONE', *, *, #22895, .T. ) ;
#62294=AXIS2_PLACEMENT_3D ( 'NONE', #51623, #50954, #25674 ) ;
#62295=CARTESIAN_POINT ( 'NONE',  ( 21.77067674801237374, -10.88489934719429719, -5.055603271500189955 ) ) ;
#62296=DIRECTION ( 'NONE',  ( 1.000000000000000000, -0.000000000000000000, 0.000000000000000000 ) ) ;
#62298=ORIENTED_EDGE ( 'NONE', *, *, #30526, .F. ) ;
#62300=AXIS2_PLACEMENT_3D ( 'NONE', #60914, #8738, #26311 ) ;
#62305=ORIENTED_EDGE ( 'NONE', *, *, #28426, .F. ) ;
#62307=ORIENTED_EDGE ( 'NONE', *, *, #57899, .F. ) ;
#62309=ADVANCED_FACE ( 'NONE', ( #6835 ), #57043, .T. ) ;
#62310=ORIENTED_EDGE ( 'NONE', *, *, #53934, .F. ) ;
#62311=CARTESIAN_POINT ( 'NONE',  ( -35.00000000000000000, 4.545979934229578134, -11.30684963584384128 ) ) ;
#62313=CARTESIAN_POINT ( 'NONE',  ( 35.00000000000000000, 11.44858830469736333, -2.627174906297124135 ) ) ;
#62317=CARTESIAN_POINT ( 'NONE',  ( -35.00000000000000000, -11.07407352312210058, -3.916263239775468197 ) ) ;
#62318=EDGE_CURVE ( 'NONE', #56972, #45989, #48145, .T. ) ;
#62319=CARTESIAN_POINT ( 'NONE',  ( 37.00000000000000711, 4.705694406421931860E-17, -3.469127814946512892E-15 ) ) ;
#62320=EDGE_CURVE ( 'NONE', #43224, #40174, #22644, .T. ) ;
#62322=ORIENTED_EDGE ( 'NONE', *, *, #34488, .F. ) ;
#62323=EDGE_CURVE ( 'NONE', #55188, #53297, #65105, .T. ) ;
#62325=CARTESIAN_POINT ( 'NONE',  ( -2.952869152607106251, -11.39722960915210592, 3.755417052241485365 ) ) ;
#62326=FACE_OUTER_BOUND ( 'NONE', #7390, .T. ) ;
#62328=CARTESIAN_POINT ( 'NONE',  ( -35.00000000000000000, 0.06441628369853458214, -12.18632975068353019 ) ) ;
#62331=LINE ( 'NONE', #7454, #48267 ) ;
#62332=DIRECTION ( 'NONE',  ( -0.000000000000000000, -0.000000000000000000, -1.000000000000000000 ) ) ;
#62335=CIRCLE ( 'NONE', #24141, 5.000000000000000000 ) ;
#62336=EDGE_CURVE ( 'NONE', #44318, #2190, #7456, .T. ) ;
#62338=CARTESIAN_POINT ( 'NONE',  ( -26.09336990274247015, 10.32957149698990662, 6.108314406108311445 ) ) ;
#62340=ORIENTED_EDGE ( 'NONE', *, *, #58276, .F. ) ;
#62341=CARTESIAN_POINT ( 'NONE',  ( -37.00000000000000711, 11.47561260193585042, -5.556331110570289056 ) ) ;
#62342=CARTESIAN_POINT ( 'NONE',  ( -27.75607595719766252, -12.49444088651119245, -5.120525247301848992 ) ) ;
#62346=DIRECTION ( 'NONE',  ( 0.000000000000000000, -0.8827602140260264463, 0.4698238015817460256 ) ) ;
#62347=ADVANCED_FACE ( 'NONE', ( #58028 ), #48051, .T. ) ;
#62348=DIRECTION ( 'NONE',  ( 1.000000000000000000, 0.000000000000000000, 0.000000000000000000 ) ) ;
#62350=LINE ( 'NONE', #57381, #59662 ) ;
#62351=CARTESIAN_POINT ( 'NONE',  ( -35.00000000000000000, 10.49591321039680736, 5.273331777780375873 ) ) ;
#62352=VERTEX_POINT ( 'NONE', #62999 ) ;
#62354=DIRECTION ( 'NONE',  ( -1.000000000000000000, 0.000000000000000000, 0.000000000000000000 ) ) ;
#62361=ADVANCED_FACE ( 'NONE', ( #49048 ), #53700, .T. ) ;
#62362=ORIENTED_EDGE ( 'NONE', *, *, #15090, .T. ) ;
#62363=CARTESIAN_POINT ( 'NONE',  ( 35.00000000000000000, 1.171570255487609291, 11.68758509253246380 ) ) ;
#62364=VERTEX_POINT ( 'NONE', #17460 ) ;
#62369=DIRECTION ( 'NONE',  ( 0.000000000000000000, 0.01356324068817998940, -0.9999080150203989437 ) ) ;
#62371=CARTESIAN_POINT ( 'NONE',  ( 35.00000000000000000, -11.78745411414841726, -3.093009498343884722 ) ) ;
#62373=ORIENTED_EDGE ( 'NONE', *, *, #45352, .T. ) ;
#62375=CARTESIAN_POINT ( 'NONE',  ( 26.44133037087954108, -12.90712213389093144, 3.963402434803054319 ) ) ;
#62377=CARTESIAN_POINT ( 'NONE',  ( 35.00000000000000000, 4.705694406421931860E-17, -3.469127814946512892E-15 ) ) ;
#62378=FACE_OUTER_BOUND ( 'NONE', #6318, .T. ) ;
#62381=EDGE_CURVE ( 'NONE', #20489, #48808, #49241, .T. ) ;
#62384=CARTESIAN_POINT ( 'NONE',  ( -35.00000000000000000, 8.496612874013292682, -9.506317355798284296 ) ) ;
#62387=CARTESIAN_POINT ( 'NONE',  ( 35.00000000000000000, -9.240395740215580744, 7.251710744571670197 ) ) ;
#62388=ORIENTED_EDGE ( 'NONE', *, *, #20957, .T. ) ;
#62389=DIRECTION ( 'NONE',  ( -1.000000000000000000, 0.000000000000000000, 0.000000000000000000 ) ) ;
#62390=ORIENTED_EDGE ( 'NONE', *, *, #48074, .F. ) ;
#62391=ADVANCED_FACE ( 'NONE', ( #7814 ), #28097, .T. ) ;
#62392=CARTESIAN_POINT ( 'NONE',  ( 37.00000000000000711, 5.814360711498443912, 10.70999494708485678 ) ) ;
#62393=DIRECTION ( 'NONE',  ( 1.000000000000000000, 0.000000000000000000, 0.000000000000000000 ) ) ;
#62394=CARTESIAN_POINT ( 'NONE',  ( -35.00000000000000000, 0.000000000000000000, 0.000000000000000000 ) ) ;
#62395=CARTESIAN_POINT ( 'NONE',  ( -35.00000000000000000, -9.926225166347071749, 6.280308599560108007 ) ) ;
#62397=LINE ( 'NONE', #62096, #12818 ) ;
#62402=DIRECTION ( 'NONE',  ( 1.000000000000000000, 0.000000000000000000, 0.000000000000000000 ) ) ;
#62403=CYLINDRICAL_SURFACE ( 'NONE', #4873, 5.000000000000000888 ) ;
#62408=DIRECTION ( 'NONE',  ( 0.000000000000000000, -0.01356324068817991828, 0.9999080150203990547 ) ) ;
#62409=CARTESIAN_POINT ( 'NONE',  ( -28.62233190725736520, 3.138911663004114949, -13.13561239495938793 ) ) ;
#62410=DIRECTION ( 'NONE',  ( 0.000000000000000000, -1.000000000000000000, 0.000000000000000000 ) ) ;
#62411=CIRCLE ( 'NONE', #44376, 12.75000000000000178 ) ;
#62412=EDGE_CURVE ( 'NONE', #20824, #51886, #21016, .T. ) ;
#62414=ADVANCED_FACE ( 'NONE', ( #35004 ), #40333, .T. ) ;
#62415=CARTESIAN_POINT ( 'NONE',  ( 9.575800908719084958, -11.95193887484098028, -1.072919909436247154 ) ) ;
#62416=VECTOR ( 'NONE', #16729, 1000.000000000000000 ) ;
#62418=DIRECTION ( 'NONE',  ( 1.000000000000000000, 0.000000000000000000, 0.000000000000000000 ) ) ;
#62420=AXIS2_PLACEMENT_3D ( 'NONE', #8764, #53984, #43664 ) ;
#62421=CARTESIAN_POINT ( 'NONE',  ( 10.66646312117316420, 7.972760762573109616, -10.89565866104123515 ) ) ;
#62422=CARTESIAN_POINT ( 'NONE',  ( -35.00000000000000000, -4.309077947445573820, -10.92721691015460550 ) ) ;
#62424=B_SPLINE_CURVE_WITH_KNOTS ( 'NONE', 3,
 ( #47477, #32154, #22866, #27840, #63393, #1915, #17861, #12520, #62409, #12209 ),
 .UNSPECIFIED., .F., .F.,
 ( 4, 2, 2, 2, 4 ),
 ( 0.002277974501771297573, 0.003563696101339898156, 0.004849417700908497872, 0.006135139300477097588, 0.007420860900045698171 ),
 .UNSPECIFIED. ) ;
#62425=EDGE_CURVE ( 'NONE', #22366, #57124, #24777, .T. ) ;
#62426=VECTOR ( 'NONE', #39014, 1000.000000000000000 ) ;
#62427=CARTESIAN_POINT ( 'NONE',  ( -28.85619398320021745, 3.750539801530000439, -12.96855624952673836 ) ) ;
#62429=ORIENTED_EDGE ( 'NONE', *, *, #53366, .T. ) ;
#62430=ORIENTED_EDGE ( 'NONE', *, *, #64460, .F. ) ;
#62431=DIRECTION ( 'NONE',  ( 0.000000000000000000, -0.4134677391718577510, -0.9105187689795923855 ) ) ;
#62432=VERTEX_POINT ( 'NONE', #60630 ) ;
#62433=CARTESIAN_POINT ( 'NONE',  ( 3.352489165639872315, 5.289728451004561904, 10.77323605601821122 ) ) ;
#62434=CARTESIAN_POINT ( 'NONE',  ( 3.427805754086258982, 7.593281694980515972, -11.19290452534897540 ) ) ;
#62435=CARTESIAN_POINT ( 'NONE',  ( -37.00000000000000711, 2.220215194441898632, 11.98254675519229195 ) ) ;
#62436=FACE_OUTER_BOUND ( 'NONE', #59969, .T. ) ;
#62437=DIRECTION ( 'NONE',  ( 1.000000000000000000, 0.000000000000000000, -0.000000000000000000 ) ) ;
#62440=ORIENTED_EDGE ( 'NONE', *, *, #25720, .F. ) ;
#62441=EDGE_CURVE ( 'NONE', #51508, #7867, #18441, .T. ) ;
#62446=ADVANCED_FACE ( 'NONE', ( #13752 ), #54685, .T. ) ;
#62447=CARTESIAN_POINT ( 'NONE',  ( 21.48131883620574101, -13.31057713625612671, -2.288337088862757440 ) ) ;
#62449=FACE_OUTER_BOUND ( 'NONE', #12512, .T. ) ;
#62450=ORIENTED_EDGE ( 'NONE', *, *, #49656, .F. ) ;
#62451=DIRECTION ( 'NONE',  ( -1.000000000000000000, -0.000000000000000000, 0.000000000000000000 ) ) ;
#62453=AXIS2_PLACEMENT_3D ( 'NONE', #30174, #20191, #61090 ) ;
#62454=DIRECTION ( 'NONE',  ( -1.000000000000000000, 0.000000000000000000, 0.000000000000000000 ) ) ;
#62457=FACE_OUTER_BOUND ( 'NONE', #22458, .T. ) ;
#62460=EDGE_LOOP ( 'NONE', ( #11259, #26068, #33655, #5388 ) ) ;
#62461=EDGE_LOOP ( 'NONE', ( #15683, #12825, #56500, #64843 ) ) ;
#62463=EDGE_CURVE ( 'NONE', #12785, #17303, #44936, .T. ) ;
#62464=DIRECTION ( 'NONE',  ( -1.000000000000000000, 0.000000000000000000, 0.000000000000000000 ) ) ;
#62465=AXIS2_PLACEMENT_3D ( 'NONE', #11935, #32217, #37200 ) ;
#62466=CARTESIAN_POINT ( 'NONE',  ( -15.27729454824424948, 5.151216734910788908, 25.00000000000000000 ) ) ;
#62468=DIRECTION ( 'NONE',  ( 1.000000000000000000, 0.000000000000000000, 0.000000000000000000 ) ) ;
#62469=VERTEX_POINT ( 'NONE', #5117 ) ;
#62470=EDGE_CURVE ( 'NONE', #35654, #1814, #55584, .T. ) ;
#62472=VECTOR ( 'NONE', #37813, 1000.000000000000000 ) ;
#62473=AXIS2_PLACEMENT_3D ( 'NONE', #805, #47027, #32362 ) ;
#62474=ORIENTED_EDGE ( 'NONE', *, *, #29566, .F. ) ;
#62475=CARTESIAN_POINT ( 'NONE',  ( -35.00000000000000000, -11.05394794832833583, 5.130401251914692651 ) ) ;
#62481=CIRCLE ( 'NONE', #22142, 5.000000000000000888 ) ;
#62483=CARTESIAN_POINT ( 'NONE',  ( -35.00000000000000000, -11.99999999999999289, 0.000000000000000000 ) ) ;
#62484=EDGE_CURVE ( 'NONE', #28276, #36620, #3585, .T. ) ;
#62485=ORIENTED_EDGE ( 'NONE', *, *, #38751, .F. ) ;
#62487=DIRECTION ( 'NONE',  ( 0.000000000000000000, -0.8169148498130212044, 0.5767582926625058892 ) ) ;
#62491=ORIENTED_EDGE ( 'NONE', *, *, #22989, .F. ) ;
#62492=DIRECTION ( 'NONE',  ( -1.000000000000000000, 0.000000000000000000, 0.000000000000000000 ) ) ;
#62493=CARTESIAN_POINT ( 'NONE',  ( -37.00000000000000711, -12.42372387097880626, -2.865935305911759379 ) ) ;
#62495=CARTESIAN_POINT ( 'NONE',  ( -3.351502423664876495, 12.75501326137288771, 4.438561732491696610 ) ) ;
#62496=CIRCLE ( 'NONE', #4129, 5.000000000000001776 ) ;
#62497=ADVANCED_FACE ( 'NONE', ( #39698 ), #49387, .T. ) ;
#62499=ORIENTED_EDGE ( 'NONE', *, *, #23791, .F. ) ;
#62500=VECTOR ( 'NONE', #32379, 1000.000000000000000 ) ;
#62505=CIRCLE ( 'NONE', #52985, 5.000000000000000000 ) ;
#62508=AXIS2_PLACEMENT_3D ( 'NONE', #43116, #42792, #17212 ) ;
#62509=ORIENTED_EDGE ( 'NONE', *, *, #15216, .F. ) ;
#62513=DIRECTION ( 'NONE',  ( 0.000000000000000000, -0.01356324068817999114, 0.9999080150203989437 ) ) ;
#62514=CIRCLE ( 'NONE', #33855, 4.999999999999999112 ) ;
#62518=ORIENTED_EDGE ( 'NONE', *, *, #59029, .F. ) ;
#62519=AXIS2_PLACEMENT_3D ( 'NONE', #41380, #41720, #11456 ) ;
#62521=CARTESIAN_POINT ( 'NONE',  ( 35.00000000000000000, 9.821084925794670184, 7.215058775251142364 ) ) ;
#62522=LINE ( 'NONE', #6698, #65046 ) ;
#62523=VERTEX_POINT ( 'NONE', #21379 ) ;
#62524=CARTESIAN_POINT ( 'NONE',  ( -18.06530682554817702, 4.745038755617106752, -11.02423958223924139 ) ) ;
#62525=DIRECTION ( 'NONE',  ( -1.000000000000000000, 0.000000000000000000, -0.000000000000000000 ) ) ;
#62531=LINE ( 'NONE', #52600, #48022 ) ;
#62532=ORIENTED_EDGE ( 'NONE', *, *, #29389, .F. ) ;
#62533=CARTESIAN_POINT ( 'NONE',  ( -37.00000000000000711, -12.57916205664480103, -2.080187960898693511 ) ) ;
#62534=CARTESIAN_POINT ( 'NONE',  ( -18.73860168220982914, -4.849834184236166301, 12.60028275727231772 ) ) ;
#62535=FACE_OUTER_BOUND ( 'NONE', #8146, .T. ) ;
#62536=DIRECTION ( 'NONE',  ( 1.000000000000000000, 0.000000000000000000, 0.000000000000000000 ) ) ;
#62537=CIRCLE ( 'NONE', #32817, 12.74999999999999822 ) ;
#62539=CARTESIAN_POINT ( 'NONE',  ( 35.00000000000000000, 4.705694406421931860E-17, -3.469127814946512892E-15 ) ) ;
#62540=CARTESIAN_POINT ( 'NONE',  ( 37.00000000000000711, 4.705694406421931860E-17, -3.469127814946512892E-15 ) ) ;
#62542=VERTEX_POINT ( 'NONE', #16404 ) ;
#62547=DIRECTION ( 'NONE',  ( 0.000000000000000000, -0.9346839223284579834, 0.3554799084908866202 ) ) ;
#62548=VERTEX_POINT ( 'NONE', #21037 ) ;
#62549=CARTESIAN_POINT ( 'NONE',  ( 35.00000000000000000, -1.039216533672818299, 11.70009620280412399 ) ) ;
#62550=CARTESIAN_POINT ( 'NONE',  ( -35.00000000000000000, -11.32068061209291265, -5.865551165831199398 ) ) ;
#62552=ORIENTED_EDGE ( 'NONE', *, *, #34746, .T. ) ;
#62553=EDGE_CURVE ( 'NONE', #43307, #60788, #46987, .T. ) ;
#62554=ORIENTED_EDGE ( 'NONE', *, *, #39463, .T. ) ;
#62559=DIRECTION ( 'NONE',  ( -1.000000000000000000, 0.000000000000000000, 0.000000000000000000 ) ) ;
#62560=FACE_OUTER_BOUND ( 'NONE', #54046, .T. ) ;
#62562=CARTESIAN_POINT ( 'NONE',  ( -7.181456785175555524, 5.890186129966279438, -10.45493698471458188 ) ) ;
#62564=CIRCLE ( 'NONE', #2069, 12.75000000000000178 ) ;
#62565=DIRECTION ( 'NONE',  ( -1.000000000000000000, -0.000000000000000000, 0.000000000000000000 ) ) ;
#62568=CARTESIAN_POINT ( 'NONE',  ( 3.291290029914074378, 8.250315036047103590, 8.713914264323182834 ) ) ;
#62569=CYLINDRICAL_SURFACE ( 'NONE', #57491, 12.18650000000000055 ) ;
#62570=ADVANCED_FACE ( 'NONE', ( #57291 ), #31995, .T. ) ;
#62572=DIRECTION ( 'NONE',  ( 1.000000000000000000, 0.000000000000000000, 0.000000000000000000 ) ) ;
#62573=EDGE_CURVE ( 'NONE', #14653, #37445, #52316, .T. ) ;
#62574=CARTESIAN_POINT ( 'NONE',  ( -9.351388602708162523, -11.42638970207761950, -3.665735721005252135 ) ) ;
#62577=AXIS2_PLACEMENT_3D ( 'NONE', #39850, #13588, #39519 ) ;
#62581=PLANE ( 'NONE',  #22435 ) ;
#62582=EDGE_LOOP ( 'NONE', ( #23789, #59588, #36941, #22863, #18666, #47825 ) ) ;
#62583=CIRCLE ( 'NONE', #33935, 12.18650000000000055 ) ;
#62585=EDGE_CURVE ( 'NONE', #39733, #14759, #32212, .T. ) ;
#62587=VERTEX_POINT ( 'NONE', #61285 ) ;
#62589=VERTEX_POINT ( 'NONE', #56648 ) ;
#62590=DIRECTION ( 'NONE',  ( -1.000000000000000000, 0.000000000000000000, 0.000000000000000000 ) ) ;
#62592=EDGE_LOOP ( 'NONE', ( #25708, #31464, #12342, #1771 ) ) ;
#62594=CYLINDRICAL_SURFACE ( 'NONE', #14617, 5.000000000000000888 ) ;
#62595=ORIENTED_EDGE ( 'NONE', *, *, #30117, .T. ) ;
#62599=AXIS2_PLACEMENT_3D ( 'NONE', #5797, #26064, #41326 ) ;
#62607=CARTESIAN_POINT ( 'NONE',  ( -35.00000000000000000, 2.936739658820028520, -11.37311665002360783 ) ) ;
#62609=CARTESIAN_POINT ( 'NONE',  ( -35.00000000000000000, 11.73463472867576129, 3.287724142101457137 ) ) ;
#62611=ORIENTED_EDGE ( 'NONE', *, *, #30193, .T. ) ;
#62612=CARTESIAN_POINT ( 'NONE',  ( 22.61346430089559334, -9.960673739116366221, -6.702005469580054609 ) ) ;
#62613=FACE_OUTER_BOUND ( 'NONE', #12517, .T. ) ;
#62614=DIRECTION ( 'NONE',  ( 1.000000000000000000, -0.000000000000000000, 0.000000000000000000 ) ) ;
#62615=ORIENTED_EDGE ( 'NONE', *, *, #3771, .F. ) ;
#62616=DIRECTION ( 'NONE',  ( 1.000000000000000000, -0.000000000000000000, 0.000000000000000000 ) ) ;
#62617=CARTESIAN_POINT ( 'NONE',  ( -4.975205859172452172, -1.416020129149132778, -11.91616074890918675 ) ) ;
#62618=CARTESIAN_POINT ( 'NONE',  ( -35.00000000000000000, 0.000000000000000000, 0.000000000000000000 ) ) ;
#62619=EDGE_LOOP ( 'NONE', ( #25241, #39198, #54076, #12448 ) ) ;
#62620=VERTEX_POINT ( 'NONE', #35992 ) ;
#62622=ORIENTED_EDGE ( 'NONE', *, *, #28426, .T. ) ;
#62624=ORIENTED_EDGE ( 'NONE', *, *, #45132, .F. ) ;
#62625=FACE_OUTER_BOUND ( 'NONE', #25821, .T. ) ;
#62628=CARTESIAN_POINT ( 'NONE',  ( 36.00000000000000711, -2.696588552979145348, -12.46157735505188491 ) ) ;
#62629=FACE_OUTER_BOUND ( 'NONE', #48819, .T. ) ;
#62631=DIRECTION ( 'NONE',  ( -1.000000000000000000, 0.000000000000000000, 0.000000000000000000 ) ) ;
#62632=VECTOR ( 'NONE', #35909, 1000.000000000000000 ) ;
#62633=CIRCLE ( 'NONE', #61591, 4.999999999999999112 ) ;
#62634=CARTESIAN_POINT ( 'NONE',  ( 22.68150004936238773, 3.158880575389232614, -11.57756885178368478 ) ) ;
#62636=DIRECTION ( 'NONE',  ( 0.000000000000000000, 0.01356324068817998940, -0.9999080150203990547 ) ) ;
#62637=DIRECTION ( 'NONE',  ( 0.000000000000000000, 0.000000000000000000, -1.000000000000000000 ) ) ;
#62638=AXIS2_PLACEMENT_3D ( 'NONE', #2189, #13148, #63663 ) ;
#62642=DIRECTION ( 'NONE',  ( -1.000000000000000000, 0.000000000000000000, -0.000000000000000000 ) ) ;
#62644=CARTESIAN_POINT ( 'NONE',  ( 22.57855258442564761, -4.427776684447072952, -12.75322679295976691 ) ) ;
#62646=PLANE ( 'NONE',  #58612 ) ;
#62647=EDGE_CURVE ( 'NONE', #50772, #8493, #42283, .T. ) ;
#62651=CARTESIAN_POINT ( 'NONE',  ( -37.00000000000000711, 4.603882218679707705, -10.80631716521661900 ) ) ;
#62653=AXIS2_PLACEMENT_3D ( 'NONE', #31784, #20843, #582 ) ;
#62656=CARTESIAN_POINT ( 'NONE',  ( -24.95436193843509187, -11.16571467309113075, 7.594604397006440522 ) ) ;
#62657=AXIS2_PLACEMENT_3D ( 'NONE', #19378, #60248, #9699 ) ;
#62658=ORIENTED_EDGE ( 'NONE', *, *, #12428, .T. ) ;
#62660=CARTESIAN_POINT ( 'NONE',  ( -27.73793999403614663, -12.15445282031313035, -5.902762415843590738 ) ) ;
#62662=DIRECTION ( 'NONE',  ( 1.000000000000000000, 0.000000000000000000, 0.000000000000000000 ) ) ;
#62666=DIRECTION ( 'NONE',  ( 1.000000000000000000, -0.000000000000000000, 0.000000000000000000 ) ) ;
#62667=EDGE_CURVE ( 'NONE', #57486, #65758, #20550, .T. ) ;
#62668=CARTESIAN_POINT ( 'NONE',  ( -37.00000000000000711, -7.215058775251327994, 9.821084925794545839 ) ) ;
#62669=VERTEX_POINT ( 'NONE', #27662 ) ;
#62672=CIRCLE ( 'NONE', #8527, 5.000000000000000000 ) ;
#62673=AXIS2_PLACEMENT_3D ( 'NONE', #57604, #12347, #13017 ) ;
#62674=VECTOR ( 'NONE', #33899, 1000.000000000000000 ) ;
#62675=DIRECTION ( 'NONE',  ( 0.000000000000000000, -0.9551603052523447435, 0.2960891610144610886 ) ) ;
#62677=EDGE_CURVE ( 'NONE', #10925, #43149, #3755, .T. ) ;
#62678=CARTESIAN_POINT ( 'NONE',  ( -37.00000000000000711, 3.511814412392118445, 11.66953048682401040 ) ) ;
#62679=LINE ( 'NONE', #41758, #30881 ) ;
#62682=DIRECTION ( 'NONE',  ( -1.000000000000000000, 0.000000000000000000, 0.000000000000000000 ) ) ;
#62684=CARTESIAN_POINT ( 'NONE',  ( 35.00000000000000000, 7.094637218249506994, 10.59380114696461739 ) ) ;
#62686=ORIENTED_EDGE ( 'NONE', *, *, #50892, .F. ) ;
#62687=CARTESIAN_POINT ( 'NONE',  ( 9.147009959156623182, 5.797999425567116560, 12.19668806932873295 ) ) ;
#62689=CARTESIAN_POINT ( 'NONE',  ( 37.00000000000000711, -5.130401251914806338, -11.05394794832827898 ) ) ;
#62690=ORIENTED_EDGE ( 'NONE', *, *, #55883, .F. ) ;
#62692=DIRECTION ( 'NONE',  ( 1.000000000000000000, 0.000000000000000000, 0.000000000000000000 ) ) ;
#62693=AXIS2_PLACEMENT_3D ( 'NONE', #9442, #31694, #61978 ) ;
#62694=CARTESIAN_POINT ( 'NONE',  ( 37.00000000000000711, -7.110831038798346881, -9.896810808925367908 ) ) ;
#62696=CARTESIAN_POINT ( 'NONE',  ( 35.00000000000000000, 4.705694406421931860E-17, -3.469127814946512892E-15 ) ) ;
#62697=VECTOR ( 'NONE', #61276, 1000.000000000000000 ) ;
#62698=ORIENTED_EDGE ( 'NONE', *, *, #45762, .F. ) ;
#62701=CYLINDRICAL_SURFACE ( 'NONE', #33999, 4.999999999999999112 ) ;
#62702=ORIENTED_EDGE ( 'NONE', *, *, #16363, .F. ) ;
#62703=ORIENTED_EDGE ( 'NONE', *, *, #8242, .F. ) ;
#62705=ORIENTED_EDGE ( 'NONE', *, *, #37164, .T. ) ;
#62706=AXIS2_PLACEMENT_3D ( 'NONE', #50236, #9001, #25600 ) ;
#62707=DIRECTION ( 'NONE',  ( 0.000000000000000000, 0.01356324068817991828, -0.9999080150203990547 ) ) ;
#62709=CARTESIAN_POINT ( 'NONE',  ( 12.47628546223243617, 0.000000000000000000, 11.99999999999999645 ) ) ;
#62710=DIRECTION ( 'NONE',  ( -1.000000000000000000, 0.000000000000000000, -0.000000000000000000 ) ) ;
#62711=EDGE_CURVE ( 'NONE', #56883, #27273, #44933, .T. ) ;
#62714=DIRECTION ( 'NONE',  ( 1.000000000000000000, 0.000000000000000000, 0.000000000000000000 ) ) ;
#62715=CIRCLE ( 'NONE', #43592, 5.000000000000000888 ) ;
#62719=AXIS2_PLACEMENT_3D ( 'NONE', #6523, #36449, #26798 ) ;
#62720=CARTESIAN_POINT ( 'NONE',  ( -35.00000000000000000, 11.02904044024209185, -4.041347439435899247 ) ) ;
#62721=CARTESIAN_POINT ( 'NONE',  ( -35.00000000000000000, -12.17626345777664021, 0.4993900848166987760 ) ) ;
#62723=ADVANCED_FACE ( 'NONE', ( #55237 ), #29314, .T. ) ;
#62725=CARTESIAN_POINT ( 'NONE',  ( -35.00000000000000000, 12.14284015767850100, 1.030638227056609679 ) ) ;
#62727=CIRCLE ( 'NONE', #49988, 4.999999999999999112 ) ;
#62728=ORIENTED_EDGE ( 'NONE', *, *, #4375, .T. ) ;
#62729=CIRCLE ( 'NONE', #22394, 5.000000000000000000 ) ;
#62730=EDGE_CURVE ( 'NONE', #2869, #42754, #43962, .T. ) ;
#62732=VERTEX_POINT ( 'NONE', #19018 ) ;
#62733=CIRCLE ( 'NONE', #29840, 12.74999999999999822 ) ;
#62735=CARTESIAN_POINT ( 'NONE',  ( 37.00000000000000711, 9.321877890560537949, 7.146664589317804683 ) ) ;
#62738=EDGE_CURVE ( 'NONE', #54185, #54568, #39619, .T. ) ;
#62739=EDGE_LOOP ( 'NONE', ( #13780, #57175, #5150, #57743 ) ) ;
#62740=CYLINDRICAL_SURFACE ( 'NONE', #40954, 4.999999999999998224 ) ;
#62741=CARTESIAN_POINT ( 'NONE',  ( -35.00000000000000000, 0.000000000000000000, 0.000000000000000000 ) ) ;
#62743=CARTESIAN_POINT ( 'NONE',  ( 145.1370849898475797, 3.309064568108273190E-14, 0.000000000000000000 ) ) ;
#62744=AXIS2_PLACEMENT_3D ( 'NONE', #44790, #65072, #29190 ) ;
#62745=AXIS2_PLACEMENT_3D ( 'NONE', #53698, #44662, #54354 ) ;
#62746=AXIS2_PLACEMENT_3D ( 'NONE', #52225, #58182, #6025 ) ;
#62747=CARTESIAN_POINT ( 'NONE',  ( -17.83419946441818027, -9.720786832536937538, 7.036071585506806336 ) ) ;
#62748=DIRECTION ( 'NONE',  ( 0.000000000000000000, -0.01356324068817998940, 0.9999080150203990547 ) ) ;
#62749=ORIENTED_EDGE ( 'NONE', *, *, #47986, .F. ) ;
#62750=AXIS2_PLACEMENT_3D ( 'NONE', #5933, #1254, #36132 ) ;
#62752=ORIENTED_EDGE ( 'NONE', *, *, #39092, .F. ) ;
#62753=CARTESIAN_POINT ( 'NONE',  ( -35.00000000000000000, -11.73463472867573643, -3.287724142101541958 ) ) ;
#62754=DIRECTION ( 'NONE',  ( 1.000000000000000000, 0.000000000000000000, 0.000000000000000000 ) ) ;
#62755=FACE_OUTER_BOUND ( 'NONE', #7232, .T. ) ;
#62758=CARTESIAN_POINT ( 'NONE',  ( 3.386626873725977038, -10.78029969106401253, 8.130803614474325869 ) ) ;
#62759=ADVANCED_FACE ( 'NONE', ( #39616 ), #65524, .T. ) ;
#62763=EDGE_CURVE ( 'NONE', #31335, #36681, #44584, .T. ) ;
#62764=ORIENTED_EDGE ( 'NONE', *, *, #16363, .T. ) ;
#62765=CIRCLE ( 'NONE', #33001, 14.99999999999998757 ) ;
#62767=LINE ( 'NONE', #954, #359 ) ;
#62768=DIRECTION ( 'NONE',  ( 1.000000000000000000, 0.000000000000000000, 0.000000000000000000 ) ) ;
#62769=DIRECTION ( 'NONE',  ( -1.000000000000000000, 0.000000000000000000, 0.000000000000000000 ) ) ;
#62770=CARTESIAN_POINT ( 'NONE',  ( 37.00000000000000711, 4.041347439436019151, 11.02904044024204211 ) ) ;
#62775=AXIS2_PLACEMENT_3D ( 'NONE', #860, #16800, #37078 ) ;
#62778=ORIENTED_EDGE ( 'NONE', *, *, #36805, .T. ) ;
#62780=CARTESIAN_POINT ( 'NONE',  ( 24.48433763888825965, -10.56700585905174705, -8.404709212046528322 ) ) ;
#62781=CYLINDRICAL_SURFACE ( 'NONE', #47046, 4.999999999999999112 ) ;
#62782=CIRCLE ( 'NONE', #34103, 12.74999999999999822 ) ;
#62785=DIRECTION ( 'NONE',  ( 0.000000000000000000, 0.01356324068817998940, -0.9999080150203990547 ) ) ;
#62788=ORIENTED_EDGE ( 'NONE', *, *, #57118, .T. ) ;
#62789=ORIENTED_EDGE ( 'NONE', *, *, #20516, .F. ) ;
#62791=ORIENTED_EDGE ( 'NONE', *, *, #53079, .F. ) ;
#62792=ORIENTED_EDGE ( 'NONE', *, *, #63400, .F. ) ;
#62793=CARTESIAN_POINT ( 'NONE',  ( -36.00000000000000711, -3.473736367725172247, -12.26766708251995475 ) ) ;
#62795=ORIENTED_EDGE ( 'NONE', *, *, #49286, .T. ) ;
#62796=AXIS2_PLACEMENT_3D ( 'NONE', #38346, #63606, #23392 ) ;
#62798=CARTESIAN_POINT ( 'NONE',  ( -37.00000000000000711, -12.26766708251994409, 3.473736367725208662 ) ) ;
#62800=EDGE_CURVE ( 'NONE', #11272, #6611, #17375, .T. ) ;
#62801=CARTESIAN_POINT ( 'NONE',  ( -35.00000000000000000, -11.68758509253249223, 1.171570255487406786 ) ) ;
#62804=VECTOR ( 'NONE', #37140, 1000.000000000000000 ) ;
#62805=CARTESIAN_POINT ( 'NONE',  ( 17.11293024090986492, 12.19363187244997881, 5.793609989425340778 ) ) ;
#62806=ADVANCED_FACE ( 'NONE', ( #35274 ), #29966, .T. ) ;
#62808=CARTESIAN_POINT ( 'NONE',  ( 35.00000000000000000, 4.705694406421931860E-17, -3.469127814946512892E-15 ) ) ;
#62810=AXIS2_PLACEMENT_3D ( 'NONE', #36025, #35379, #30070 ) ;
#62812=CARTESIAN_POINT ( 'NONE',  ( 35.00000000000000000, 10.43555801961475282, -5.391785509271000087 ) ) ;
#62813=DIRECTION ( 'NONE',  ( -1.000000000000000000, 0.000000000000000000, -0.000000000000000000 ) ) ;
#62814=CIRCLE ( 'NONE', #34132, 5.000000000000002665 ) ;
#62815=CARTESIAN_POINT ( 'NONE',  ( -28.71060117729525984, 3.670315194194624375, -12.99175741217617386 ) ) ;
#62817=EDGE_LOOP ( 'NONE', ( #63521, #6641, #52611, #50872 ) ) ;
#62820=VERTEX_POINT ( 'NONE', #60227 ) ;
#62824=AXIS2_PLACEMENT_3D ( 'NONE', #17410, #37686, #52972 ) ;
#62825=CARTESIAN_POINT ( 'NONE',  ( -35.00000000000000000, 0.000000000000000000, 0.000000000000000000 ) ) ;
#62826=CIRCLE ( 'NONE', #47940, 5.000000000000000000 ) ;
#62829=VERTEX_POINT ( 'NONE', #28655 ) ;
#62830=CARTESIAN_POINT ( 'NONE',  ( 37.00000000000000711, -11.26103545359853264, 3.340853584269647847 ) ) ;
#62833=CARTESIAN_POINT ( 'NONE',  ( -37.00000000000000711, 0.000000000000000000, 0.000000000000000000 ) ) ;
#62834=EDGE_CURVE ( 'NONE', #25804, #34326, #44998, .T. ) ;
#62835=AXIS2_PLACEMENT_3D ( 'NONE', #46420, #65691, #20159 ) ;
#62837=CIRCLE ( 'NONE', #50131, 4.999999999999999112 ) ;
#62838=DIRECTION ( 'NONE',  ( 1.000000000000000000, 0.000000000000000000, -0.000000000000000000 ) ) ;
#62839=EDGE_LOOP ( 'NONE', ( #35560, #9311, #15198, #21053 ) ) ;
#62843=EDGE_CURVE ( 'NONE', #10126, #21470, #18710, .T. ) ;
#62845=VERTEX_POINT ( 'NONE', #8718 ) ;
#62848=ORIENTED_EDGE ( 'NONE', *, *, #56944, .T. ) ;
#62849=CARTESIAN_POINT ( 'NONE',  ( -18.15255838926453080, 3.492896982859142518, 11.48290758289192937 ) ) ;
#62851=CYLINDRICAL_SURFACE ( 'NONE', #21601, 4.999999999999999112 ) ;
#62855=VERTEX_POINT ( 'NONE', #49308 ) ;
#62856=CIRCLE ( 'NONE', #21326, 5.000000000000001776 ) ;
#62867=CYLINDRICAL_SURFACE ( 'NONE', #8433, 4.999999999999999112 ) ;
#62868=CARTESIAN_POINT ( 'NONE',  ( 24.90125186782636035, -0.3305283664803125299, 12.00214278619375285 ) ) ;
#62869=ORIENTED_EDGE ( 'NONE', *, *, #60065, .T. ) ;
#62870=ORIENTED_EDGE ( 'NONE', *, *, #48168, .T. ) ;
#62871=CARTESIAN_POINT ( 'NONE',  ( -35.00000000000000000, 0.6593684648222323252, -12.73293890771482495 ) ) ;
#62874=CIRCLE ( 'NONE', #3586, 5.000000000000000000 ) ;
#62875=CARTESIAN_POINT ( 'NONE',  ( 35.00000000000000000, 5.130401251914885385, 11.05394794832823813 ) ) ;
#62877=DIRECTION ( 'NONE',  ( 1.000000000000000000, 0.000000000000000000, 0.000000000000000000 ) ) ;
#62879=DIRECTION ( 'NONE',  ( 0.000000000000000000, 0.4698238015817302049, 0.8827602140260349950 ) ) ;
#62880=AXIS2_PLACEMENT_3D ( 'NONE', #59584, #14344, #34933 ) ;
#62881=CARTESIAN_POINT ( 'NONE',  ( -30.18541646480309026, -1.416020129149132334, -13.42553116244734746 ) ) ;
#62882=CARTESIAN_POINT ( 'NONE',  ( 6.361445718264521432, -4.355102044641763648, -11.18181944858513077 ) ) ;
#62883=ORIENTED_EDGE ( 'NONE', *, *, #13962, .F. ) ;
#62884=LINE ( 'NONE', #47294, #47066 ) ;
#62890=CARTESIAN_POINT ( 'NONE',  ( -18.55545074886880386, 5.671797102417516001, 10.57879050686813116 ) ) ;
#62893=AXIS2_PLACEMENT_3D ( 'NONE', #62363, #16512, #22473 ) ;
#62894=VERTEX_POINT ( 'NONE', #46574 ) ;
#62895=CIRCLE ( 'NONE', #55450, 4.999999999999999112 ) ;
#62896=EDGE_CURVE ( 'NONE', #27449, #3878, #51380, .T. ) ;
#62897=ORIENTED_EDGE ( 'NONE', *, *, #30914, .T. ) ;
#62898=CARTESIAN_POINT ( 'NONE',  ( -35.00000000000000000, 0.000000000000000000, 0.000000000000000000 ) ) ;
#62899=AXIS2_PLACEMENT_3D ( 'NONE', #22066, #6457, #42653 ) ;
#62900=VERTEX_POINT ( 'NONE', #60892 ) ;
#62901=FACE_OUTER_BOUND ( 'NONE', #42080, .T. ) ;
#62902=AXIS2_PLACEMENT_3D ( 'NONE', #45141, #40128, #50784 ) ;
#62904=CARTESIAN_POINT ( 'NONE',  ( -3.439258850808092571, -11.96382994935912514, 6.264996690403261681 ) ) ;
#62905=CARTESIAN_POINT ( 'NONE',  ( -19.16330044134494415, -4.498325028293125527, 11.12691725379990082 ) ) ;
#62906=EDGE_CURVE ( 'NONE', #10959, #47299, #50337, .T. ) ;
#62909=EDGE_CURVE ( 'NONE', #33373, #53424, #20964, .T. ) ;
#62910=AXIS2_PLACEMENT_3D ( 'NONE', #31174, #40478, #6236 ) ;
#62912=( BOUNDED_CURVE ( )  B_SPLINE_CURVE ( 3, ( #6528, #2188, #22468, #32429 ),
 .UNSPECIFIED., .F., .F. ) 
 B_SPLINE_CURVE_WITH_KNOTS ( ( 4, 4 ),
 ( 0.7473423473803021411, 0.7669100185107887713 ),
 .UNSPECIFIED. ) 
 CURVE ( )  GEOMETRIC_REPRESENTATION_ITEM ( )  RATIONAL_B_SPLINE_CURVE ( ( 1.000000000000000000, 0.9999680924417370109, 0.9999680924417370109, 1.000000000000000000 ) ) 
 REPRESENTATION_ITEM ( '' )  );
#62913=FACE_OUTER_BOUND ( 'NONE', #2881, .T. ) ;
#62914=CARTESIAN_POINT ( 'NONE',  ( 22.98437084614390713, 11.91223824963345024, -6.360283269683757901 ) ) ;
#62916=DIRECTION ( 'NONE',  ( -1.000000000000000000, 0.000000000000000000, -0.000000000000000000 ) ) ;
#62919=CIRCLE ( 'NONE', #27907, 12.75000000000000178 ) ;
#62920=CIRCLE ( 'NONE', #39574, 12.18650000000000411 ) ;
#62922=CIRCLE ( 'NONE', #52373, 4.999999999999999112 ) ;
#62923=AXIS2_PLACEMENT_3D ( 'NONE', #6112, #46656, #16720 ) ;
#62924=ORIENTED_EDGE ( 'NONE', *, *, #53768, .F. ) ;
#62926=CARTESIAN_POINT ( 'NONE',  ( 5.043734429376389272, -9.821217208287897904, 9.263622243474671336 ) ) ;
#62927=VERTEX_POINT ( 'NONE', #35914 ) ;
#62928=LINE ( 'NONE', #2087, #56573 ) ;
#62929=CYLINDRICAL_SURFACE ( 'NONE', #20461, 12.18650000000000055 ) ;
#62930=VERTEX_POINT ( 'NONE', #15967 ) ;
#62933=ORIENTED_EDGE ( 'NONE', *, *, #15582, .T. ) ;
#62934=CIRCLE ( 'NONE', #5627, 5.000000000000000000 ) ;
#62935=CARTESIAN_POINT ( 'NONE',  ( -36.00000000000000711, 3.307597835713245171, 12.31350058095524425 ) ) ;
#62936=ORIENTED_EDGE ( 'NONE', *, *, #62320, .F. ) ;
#62937=ORIENTED_EDGE ( 'NONE', *, *, #48722, .F. ) ;
#62938=ADVANCED_FACE ( 'NONE', ( #11003, #15332 ), #51589, .F. ) ;
#62939=AXIS2_PLACEMENT_3D ( 'NONE', #64797, #34856, #55836 ) ;
#62944=DIRECTION ( 'NONE',  ( -1.000000000000000000, -1.836970198721029688E-16, -0.000000000000000000 ) ) ;
#62947=DIRECTION ( 'NONE',  ( 0.000000000000000000, 0.01356324068817998940, -0.9999080150203989437 ) ) ;
#62948=VECTOR ( 'NONE', #8836, 1000.000000000000000 ) ;
#62951=CARTESIAN_POINT ( 'NONE',  ( -24.33265139114022091, 8.847575708096826475, 8.109868413052772951 ) ) ;
#62952=ORIENTED_EDGE ( 'NONE', *, *, #2579, .T. ) ;
#62953=FACE_OUTER_BOUND ( 'NONE', #16714, .T. ) ;
#62954=ORIENTED_EDGE ( 'NONE', *, *, #29442, .F. ) ;
#62955=CARTESIAN_POINT ( 'NONE',  ( -35.00000000000000000, -1.286231064351400555, 12.68495603654571369 ) ) ;
#62956=ORIENTED_EDGE ( 'NONE', *, *, #13236, .F. ) ;
#62957=DIRECTION ( 'NONE',  ( -1.000000000000000000, 0.000000000000000000, 0.000000000000000000 ) ) ;
#62960=VERTEX_POINT ( 'NONE', #41909 ) ;
#62962=DIRECTION ( 'NONE',  ( 0.000000000000000000, -0.01356324068818000848, 0.9999080150203990547 ) ) ;
#62964=ORIENTED_EDGE ( 'NONE', *, *, #15911, .T. ) ;
#62965=EDGE_CURVE ( 'NONE', #9350, #2029, #2530, .T. ) ;
#62969=ADVANCED_FACE ( 'NONE', ( #31288 ), #20315, .T. ) ;
#62970=AXIS2_PLACEMENT_3D ( 'NONE', #27867, #62769, #48173 ) ;
#62972=DIRECTION ( 'NONE',  ( -0.000000000000000000, -1.000000000000000000, -0.000000000000000000 ) ) ;
#62973=CIRCLE ( 'NONE', #34300, 5.000000000000000888 ) ;
#62974=DIRECTION ( 'NONE',  ( 1.000000000000000000, 0.000000000000000000, 0.000000000000000000 ) ) ;
#62975=DIRECTION ( 'NONE',  ( 0.000000000000000000, 0.4134677391718512007, 0.9105187689795953832 ) ) ;
#62979=CARTESIAN_POINT ( 'NONE',  ( -35.00000000000000000, -9.196955404009360180, 8.830544224262913744 ) ) ;
#62982=DIRECTION ( 'NONE',  ( 1.000000000000000000, 0.000000000000000000, 0.000000000000000000 ) ) ;
#62985=FACE_OUTER_BOUND ( 'NONE', #43406, .T. ) ;
#62990=FACE_OUTER_BOUND ( 'NONE', #8317, .T. ) ;
#62992=AXIS2_PLACEMENT_3D ( 'NONE', #47348, #61973, #31383 ) ;
#62993=CARTESIAN_POINT ( 'NONE',  ( 17.11293024090985071, -12.19363187244996105, 5.793609989425343443 ) ) ;
#62995=CARTESIAN_POINT ( 'NONE',  ( 12.03305870789770360, 0.5719181555549518459, -11.98657499750327915 ) ) ;
#62997=DIRECTION ( 'NONE',  ( 0.000000000000000000, -0.01356324068817991828, 0.9999080150203990547 ) ) ;
#62998=CYLINDRICAL_SURFACE ( 'NONE', #25111, 12.18650000000000055 ) ;
#62999=CARTESIAN_POINT ( 'NONE',  ( -35.00000000000000000, 11.80185301892987582, -4.824807283153994319 ) ) ;
#63000=CARTESIAN_POINT ( 'NONE',  ( -18.04274061274178109, -13.45660803163010755, 1.263225231962421313 ) ) ;
#63001=CARTESIAN_POINT ( 'NONE',  ( -27.27855387000350262, 10.59660315834921640, 5.631341004100471892 ) ) ;
#63002=CARTESIAN_POINT ( 'NONE',  ( 35.00000000000000000, -6.280308599560208371, -9.926225166347007800 ) ) ;
#63004=CARTESIAN_POINT ( 'NONE',  ( 18.43933328720107667, -6.457919038062313710, 10.12447623701847554 ) ) ;
#63005=CARTESIAN_POINT ( 'NONE',  ( -35.00000000000000000, 0.000000000000000000, 0.000000000000000000 ) ) ;
#63008=ORIENTED_EDGE ( 'NONE', *, *, #51401, .T. ) ;
#63009=CARTESIAN_POINT ( 'NONE',  ( 24.48320719723312777, 10.56747877308070827, -8.404134578084967444 ) ) ;
#63010=DIRECTION ( 'NONE',  ( 1.000000000000000000, 0.000000000000000000, 0.000000000000000000 ) ) ;
#63011=ORIENTED_EDGE ( 'NONE', *, *, #18166, .F. ) ;
#63012=VECTOR ( 'NONE', #57698, 1000.000000000000000 ) ;
#63013=AXIS2_PLACEMENT_3D ( 'NONE', #9454, #14445, #40719 ) ;
#63014=EDGE_LOOP ( 'NONE', ( #54330, #47886, #3099, #33276 ) ) ;
#63016=AXIS2_PLACEMENT_3D ( 'NONE', #41399, #1537, #61689 ) ;
#63022=DIRECTION ( 'NONE',  ( 0.000000000000000000, -0.01356324068817998940, 0.9999080150203990547 ) ) ;
#63023=CARTESIAN_POINT ( 'NONE',  ( -7.489022030332961322, 25.00000000000000000, -10.84914964302385521 ) ) ;
#63024=CARTESIAN_POINT ( 'NONE',  ( -35.00000000000000000, 2.220215194441899076, 11.98254675519229195 ) ) ;
#63026=DIRECTION ( 'NONE',  ( 1.000000000000000000, 0.000000000000000000, 0.000000000000000000 ) ) ;
#63028=ORIENTED_EDGE ( 'NONE', *, *, #41048, .T. ) ;
#63030=ORIENTED_EDGE ( 'NONE', *, *, #8774, .T. ) ;
#63031=CARTESIAN_POINT ( 'NONE',  ( 24.88399796223642468, -1.143778065019554813, -11.94702019429119844 ) ) ;
#63040=CARTESIAN_POINT ( 'NONE',  ( 36.00000000000000711, -1.113475361586579337, -12.70128625845192616 ) ) ;
#63041=ORIENTED_EDGE ( 'NONE', *, *, #29862, .T. ) ;
#63042=AXIS2_PLACEMENT_3D ( 'NONE', #24682, #40622, #29336 ) ;
#63047=AXIS2_PLACEMENT_3D ( 'NONE', #64362, #63060, #13182 ) ;
#63049=CARTESIAN_POINT ( 'NONE',  ( -37.00000000000000711, 12.38385022362082033, 3.033604067594621867 ) ) ;
#63050=ADVANCED_FACE ( 'NONE', ( #24158 ), #28489, .F. ) ;
#63052=DIRECTION ( 'NONE',  ( -1.000000000000000000, 0.000000000000000000, -0.000000000000000000 ) ) ;
#63054=LINE ( 'NONE', #17517, #17217 ) ;
#63057=DIRECTION ( 'NONE',  ( -1.000000000000000000, 0.000000000000000000, 0.000000000000000000 ) ) ;
#63058=VECTOR ( 'NONE', #38165, 1000.000000000000000 ) ;
#63059=EDGE_CURVE ( 'NONE', #63385, #27449, #55640, .T. ) ;
#63060=DIRECTION ( 'NONE',  ( -1.000000000000000000, 0.000000000000000000, 0.000000000000000000 ) ) ;
#63062=CARTESIAN_POINT ( 'NONE',  ( -47.00000000000000711, 0.000000000000000000, 0.000000000000000000 ) ) ;
#63063=ADVANCED_FACE ( 'NONE', ( #8219 ), #33494, .T. ) ;
#63064=EDGE_LOOP ( 'NONE', ( #65782, #25024, #24787, #25624 ) ) ;
#63066=CARTESIAN_POINT ( 'NONE',  ( -8.650525597369476571, -10.29405175124346172, -8.740411465918450418 ) ) ;
#63067=DIRECTION ( 'NONE',  ( 1.000000000000000000, 0.000000000000000000, -0.000000000000000000 ) ) ;
#63069=CARTESIAN_POINT ( 'NONE',  ( 11.74548640120467979, 8.775604215601129354, -8.184666801472349817 ) ) ;
#63071=VERTEX_POINT ( 'NONE', #43794 ) ;
#63072=DIRECTION ( 'NONE',  ( 1.000000000000000000, 0.000000000000000000, -0.000000000000000000 ) ) ;
#63073=ADVANCED_FACE ( 'NONE', ( #12528 ), #54098, .T. ) ;
#63074=AXIS2_PLACEMENT_3D ( 'NONE', #30770, #51090, #5546 ) ;
#63075=ORIENTED_EDGE ( 'NONE', *, *, #32320, .T. ) ;
#63077=CARTESIAN_POINT ( 'NONE',  ( -35.00000000000000000, 10.25474254703952859, 6.584150480049587806 ) ) ;
#63078=CIRCLE ( 'NONE', #23797, 4.999999999999999112 ) ;
#63079=EDGE_CURVE ( 'NONE', #48921, #29332, #21745, .T. ) ;
#63081=DIRECTION ( 'NONE',  ( -1.000000000000000000, -0.000000000000000000, -0.000000000000000000 ) ) ;
#63083=AXIS2_PLACEMENT_3D ( 'NONE', #33704, #8775, #8439 ) ;
#63085=CARTESIAN_POINT ( 'NONE',  ( 18.50973545861780423, 8.752035742591949941, 10.30270490042575737 ) ) ;
#63088=DIRECTION ( 'NONE',  ( -0.000000000000000000, -1.000000000000000000, -0.000000000000000000 ) ) ;
#63093=ORIENTED_EDGE ( 'NONE', *, *, #7115, .T. ) ;
#63094=CARTESIAN_POINT ( 'NONE',  ( 36.00000000000000711, 11.66664283989686979, 5.143145423404152261 ) ) ;
#63095=DIRECTION ( 'NONE',  ( -1.000000000000000000, 0.000000000000000000, -0.000000000000000000 ) ) ;
#63097=DIRECTION ( 'NONE',  ( 0.000000000000000000, 0.01356324068818000328, -0.9999080150203990547 ) ) ;
#63099=EDGE_CURVE ( 'NONE', #16693, #3390, #34765, .T. ) ;
#63105=CARTESIAN_POINT ( 'NONE',  ( 3.780834652287974773, 8.352030633203074927, 25.00000000000000000 ) ) ;
#63112=DIRECTION ( 'NONE',  ( 1.000000000000000000, 0.000000000000000000, 0.000000000000000000 ) ) ;
#63113=VERTEX_POINT ( 'NONE', #44758 ) ;
#63114=VERTEX_POINT ( 'NONE', #25145 ) ;
#63115=EDGE_CURVE ( 'NONE', #34249, #32729, #41805, .T. ) ;
#63116=CIRCLE ( 'NONE', #51468, 12.75000000000000178 ) ;
#63119=CARTESIAN_POINT ( 'NONE',  ( 47.00000000000000711, 4.705694406421931860E-17, -3.469127814946512892E-15 ) ) ;
#63122=DIRECTION ( 'NONE',  ( 1.000000000000000000, -0.000000000000000000, 0.000000000000000000 ) ) ;
#63123=ORIENTED_EDGE ( 'NONE', *, *, #55843, .T. ) ;
#63129=EDGE_CURVE ( 'NONE', #44861, #39718, #45414, .T. ) ;
#63130=EDGE_LOOP ( 'NONE', ( #27293, #63915, #49591, #54371 ) ) ;
#63134=VERTEX_POINT ( 'NONE', #30765 ) ;
#63135=CYLINDRICAL_SURFACE ( 'NONE', #43689, 12.18649999999999878 ) ;
#63136=AXIS2_PLACEMENT_3D ( 'NONE', #44137, #13229, #33516 ) ;
#63137=DIRECTION ( 'NONE',  ( -1.000000000000000000, -0.000000000000000000, 0.000000000000000000 ) ) ;
#63138=CARTESIAN_POINT ( 'NONE',  ( 37.00000000000000711, 4.705694406421931860E-17, -3.469127814946512892E-15 ) ) ;
#63140=CARTESIAN_POINT ( 'NONE',  ( 36.00000000000000711, -12.46157735505187247, 2.696588552979187536 ) ) ;
#63143=ORIENTED_EDGE ( 'NONE', *, *, #8060, .F. ) ;
#63147=CARTESIAN_POINT ( 'NONE',  ( -35.00000000000000000, -2.220215194441821360, -11.98254675519230794 ) ) ;
#63149=CARTESIAN_POINT ( 'NONE',  ( 29.60113888844488272, 8.983404872736210578, 7.970891106847078689 ) ) ;
#63150=CARTESIAN_POINT ( 'NONE',  ( 37.00000000000000711, 10.92721691015455754, -4.309077947445693724 ) ) ;
#63152=CARTESIAN_POINT ( 'NONE',  ( -28.41827485489077532, 3.509237424706437292, -13.03592162821790801 ) ) ;
#63153=EDGE_CURVE ( 'NONE', #16086, #27902, #12089, .T. ) ;
#63155=VERTEX_POINT ( 'NONE', #39443 ) ;
#63157=EDGE_CURVE ( 'NONE', #52994, #12978, #26955, .T. ) ;
#63159=CARTESIAN_POINT ( 'NONE',  ( -35.00000000000000000, 0.000000000000000000, 0.000000000000000000 ) ) ;
#63161=DIRECTION ( 'NONE',  ( 0.000000000000000000, 0.01356324068817998940, -0.9999080150203990547 ) ) ;
#63162=ADVANCED_FACE ( 'NONE', ( #9185 ), #29463, .T. ) ;
#63163=CARTESIAN_POINT ( 'NONE',  ( -37.00000000000000711, -4.824807283154036952, -11.80185301892985805 ) ) ;
#63166=AXIS2_PLACEMENT_3D ( 'NONE', #38668, #53959, #38320 ) ;
#63168=CARTESIAN_POINT ( 'NONE',  ( 35.00000000000000000, 12.21925492305367200, 3.640372113593418391 ) ) ;
#63169=CARTESIAN_POINT ( 'NONE',  ( -37.00000000000000711, 9.493370459201697642, 6.917234959366862057 ) ) ;
#63170=DIRECTION ( 'NONE',  ( -1.000000000000000000, 0.000000000000000000, 0.000000000000000000 ) ) ;
#63172=CIRCLE ( 'NONE', #24922, 5.000000000000001776 ) ;
#63173=ORIENTED_EDGE ( 'NONE', *, *, #34120, .T. ) ;
#63176=AXIS2_PLACEMENT_3D ( 'NONE', #26995, #17346, #42249 ) ;
#63178=EDGE_CURVE ( 'NONE', #6530, #46064, #18483, .T. ) ;
#63179=VERTEX_POINT ( 'NONE', #1846 ) ;
#63180=CARTESIAN_POINT ( 'NONE',  ( -36.00000000000000711, 12.66641127287626034, 1.457575200925590453 ) ) ;
#63181=VERTEX_POINT ( 'NONE', #20811 ) ;
#63185=CARTESIAN_POINT ( 'NONE',  ( -35.00000000000000000, 0.000000000000000000, 0.000000000000000000 ) ) ;
#63187=EDGE_CURVE ( 'NONE', #45883, #39718, #28099, .T. ) ;
#63191=VECTOR ( 'NONE', #52302, 1000.000000000000000 ) ;
#63194=DIRECTION ( 'NONE',  ( -1.000000000000000000, -1.836970198721029688E-16, 0.000000000000000000 ) ) ;
#63197=LINE ( 'NONE', #22294, #64049 ) ;
#63198=CARTESIAN_POINT ( 'NONE',  ( -36.00000000000000711, 8.235637554476644695, 9.733281772932192766 ) ) ;
#63200=ORIENTED_EDGE ( 'NONE', *, *, #56588, .T. ) ;
#63203=EDGE_CURVE ( 'NONE', #12979, #15531, #21813, .T. ) ;
#63204=ORIENTED_EDGE ( 'NONE', *, *, #25445, .F. ) ;
#63206=ORIENTED_EDGE ( 'NONE', *, *, #51971, .T. ) ;
#63207=LINE ( 'NONE', #43243, #48972 ) ;
#63211=CARTESIAN_POINT ( 'NONE',  ( 37.00000000000000711, 8.830544224263075392, 9.196955404009196755 ) ) ;
#63214=CARTESIAN_POINT ( 'NONE',  ( 6.787498709350838766, -5.788853919323486252, -10.51921472689792658 ) ) ;
#63219=DIRECTION ( 'NONE',  ( 0.000000000000000000, 0.9937233664769756780, -0.1118654143051654171 ) ) ;
#63220=VERTEX_POINT ( 'NONE', #6186 ) ;
#63221=CARTESIAN_POINT ( 'NONE',  ( 35.00000000000000000, 2.185196060784047045, 11.54110654723646157 ) ) ;
#63222=FACE_OUTER_BOUND ( 'NONE', #1247, .T. ) ;
#63224=EDGE_CURVE ( 'NONE', #8907, #50922, #11475, .T. ) ;
#63225=CIRCLE ( 'NONE', #25028, 5.000000000000000000 ) ;
#63227=ORIENTED_EDGE ( 'NONE', *, *, #30522, .F. ) ;
#63229=ADVANCED_FACE ( 'NONE', ( #32410 ), #36757, .F. ) ;
#63232=DIRECTION ( 'NONE',  ( -1.000000000000000000, 0.000000000000000000, -0.000000000000000000 ) ) ;
#63233=EDGE_CURVE ( 'NONE', #18752, #32907, #40764, .T. ) ;
#63235=CARTESIAN_POINT ( 'NONE',  ( -17.68548993317135398, -8.030202814678021994, 8.922382581021231829 ) ) ;
#63236=ORIENTED_EDGE ( 'NONE', *, *, #22619, .F. ) ;
#63237=DIRECTION ( 'NONE',  ( -1.000000000000000000, 0.000000000000000000, 0.000000000000000000 ) ) ;
#63238=AXIS2_PLACEMENT_3D ( 'NONE', #48231, #17627, #33229 ) ;
#63239=ADVANCED_FACE ( 'NONE', ( #47721 ), #61357, .T. ) ;
#63242=CARTESIAN_POINT ( 'NONE',  ( 37.00000000000000711, 2.021542716731571154, 12.01765980939839196 ) ) ;
#63246=EDGE_LOOP ( 'NONE', ( #53037, #59668, #61931, #13648 ) ) ;
#63248=EDGE_CURVE ( 'NONE', #16664, #35283, #16150, .T. ) ;
#63250=DIRECTION ( 'NONE',  ( 1.000000000000000000, 0.000000000000000000, 0.000000000000000000 ) ) ;
#63253=EDGE_LOOP ( 'NONE', ( #9231, #20450, #60164, #41125 ) ) ;
#63255=ORIENTED_EDGE ( 'NONE', *, *, #52424, .F. ) ;
#63258=EDGE_LOOP ( 'NONE', ( #6892, #15681, #64701, #38784 ) ) ;
#63259=DIRECTION ( 'NONE',  ( -1.000000000000000000, -0.000000000000000000, 0.000000000000000000 ) ) ;
#63260=CIRCLE ( 'NONE', #5965, 5.000000000000000888 ) ;
#63262=VERTEX_POINT ( 'NONE', #52397 ) ;
#63263=DIRECTION ( 'NONE',  ( -1.000000000000000000, 0.000000000000000000, -0.000000000000000000 ) ) ;
#63264=DIRECTION ( 'NONE',  ( 1.000000000000000000, 0.000000000000000000, 0.000000000000000000 ) ) ;
#63266=CARTESIAN_POINT ( 'NONE',  ( 19.08014163997884083, 3.539499929403262968, 11.50397527077400106 ) ) ;
#63269=DIRECTION ( 'NONE',  ( 1.000000000000000000, -0.000000000000000000, 0.000000000000000000 ) ) ;
#63271=DIRECTION ( 'NONE',  ( -1.000000000000000000, -0.000000000000000000, -0.000000000000000000 ) ) ;
#63272=ORIENTED_EDGE ( 'NONE', *, *, #62206, .F. ) ;
#63273=CARTESIAN_POINT ( 'NONE',  ( -28.25740157508035821, 10.82141011665706465, -5.195967623798041224 ) ) ;
#63274=EDGE_CURVE ( 'NONE', #2632, #63113, #25872, .T. ) ;
#63275=EDGE_CURVE ( 'NONE', #57020, #60276, #13041, .T. ) ;
#63276=ORIENTED_EDGE ( 'NONE', *, *, #53772, .T. ) ;
#63283=LINE ( 'NONE', #17753, #56689 ) ;
#63284=CARTESIAN_POINT ( 'NONE',  ( -17.83419946441818027, -9.720786832536937538, 25.00000000000000000 ) ) ;
#63290=EDGE_LOOP ( 'NONE', ( #59952, #39822, #56906, #59315 ) ) ;
#63291=ORIENTED_EDGE ( 'NONE', *, *, #45645, .F. ) ;
#63292=DIRECTION ( 'NONE',  ( 1.000000000000000000, -0.000000000000000000, -0.000000000000000000 ) ) ;
#63294=CARTESIAN_POINT ( 'NONE',  ( -37.00000000000000711, 10.02106554660708859, 7.882940143791811849 ) ) ;
#63296=DIRECTION ( 'NONE',  ( 1.000000000000000000, -0.000000000000000000, 0.000000000000000000 ) ) ;
#63297=ADVANCED_FACE ( 'NONE', ( #31442 ), #51741, .T. ) ;
#63299=DIRECTION ( 'NONE',  ( 0.000000000000000000, -0.8515178078024924213, 0.5243256840888473880 ) ) ;
#63302=ORIENTED_EDGE ( 'NONE', *, *, #27879, .T. ) ;
#63304=DIRECTION ( 'NONE',  ( -1.000000000000000000, 0.000000000000000000, 0.000000000000000000 ) ) ;
#63305=B_SPLINE_CURVE_WITH_KNOTS ( 'NONE', 3,
 ( #18473, #3510, #7825, #59337, #29395, #64963, #39704, #38731, #13442, #3167, #39368, #49394 ),
 .UNSPECIFIED., .F., .F.,
 ( 4, 2, 2, 2, 2, 4 ),
 ( 0.006954109192215124878, 0.007747514422417968276, 0.008144217037519390842, 0.008540919652620814276, 0.009334324882823661143, 0.01012773011302650801 ),
 .UNSPECIFIED. ) ;
#63308=FACE_OUTER_BOUND ( 'NONE', #33302, .T. ) ;
#63311=CARTESIAN_POINT ( 'NONE',  ( -29.92777678363736626, -3.750539801530011985, 25.00000000000000000 ) ) ;
#63312=VERTEX_POINT ( 'NONE', #17468 ) ;
#63314=FACE_OUTER_BOUND ( 'NONE', #58201, .T. ) ;
#63317=DIRECTION ( 'NONE',  ( 0.000000000000000000, 0.01356324068817998940, -0.9999080150203989437 ) ) ;
#63320=EDGE_LOOP ( 'NONE', ( #45213, #11692, #60498, #31620 ) ) ;
#63321=CARTESIAN_POINT ( 'NONE',  ( -37.00000000000000711, -11.72397916322012890, 0.7214809346828189307 ) ) ;
#63324=CARTESIAN_POINT ( 'NONE',  ( -37.00000000000000711, 0.000000000000000000, 0.000000000000000000 ) ) ;
#63325=ORIENTED_EDGE ( 'NONE', *, *, #26344, .F. ) ;
#63329=ORIENTED_EDGE ( 'NONE', *, *, #34238, .T. ) ;
#63330=ORIENTED_EDGE ( 'NONE', *, *, #32847, .F. ) ;
#63332=CARTESIAN_POINT ( 'NONE',  ( 35.00000000000000000, 2.905556151562782574, 11.38112321385047210 ) ) ;
#63334=CIRCLE ( 'NONE', #48519, 5.000000000000000888 ) ;
#63335=FACE_OUTER_BOUND ( 'NONE', #48254, .T. ) ;
#63336=EDGE_LOOP ( 'NONE', ( #57963, #2985, #26518, #26903 ) ) ;
#63337=CARTESIAN_POINT ( 'NONE',  ( -47.00000000000000711, 0.000000000000000000, 0.000000000000000000 ) ) ;
#63339=CARTESIAN_POINT ( 'NONE',  ( 35.00000000000000000, 12.73293890771483738, 0.6593684648219080291 ) ) ;
#63341=CARTESIAN_POINT ( 'NONE',  ( -27.63833054859100002, 10.11270778234927548, -6.466741440011825937 ) ) ;
#63345=CARTESIAN_POINT ( 'NONE',  ( -37.00000000000000711, -8.146229107149334681, -9.063649021439044162 ) ) ;
#63346=EDGE_CURVE ( 'NONE', #31517, #53149, #8783, .T. ) ;
#63348=VERTEX_POINT ( 'NONE', #17791 ) ;
#63349=CARTESIAN_POINT ( 'NONE',  ( 26.34661844826604593, 13.08594712317291986, 3.317828791472332117 ) ) ;
#63350=ORIENTED_EDGE ( 'NONE', *, *, #64460, .T. ) ;
#63352=CARTESIAN_POINT ( 'NONE',  ( -14.11589373245165469, 8.250315036047107142, 10.68561190601526611 ) ) ;
#63354=CARTESIAN_POINT ( 'NONE',  ( -3.385148144206586274, 5.981256269455808905, 10.44061326340053775 ) ) ;
#63356=CARTESIAN_POINT ( 'NONE',  ( 22.57855258442565116, 3.026812727784649493, 13.15630665159948975 ) ) ;
#63357=ORIENTED_EDGE ( 'NONE', *, *, #65487, .T. ) ;
#63359=CARTESIAN_POINT ( 'NONE',  ( 37.00000000000000711, 1.738225594540171670, 12.63095688309027054 ) ) ;
#63360=CARTESIAN_POINT ( 'NONE',  ( 35.00000000000000000, 7.110831038798420600, 9.896810808925309288 ) ) ;
#63361=ORIENTED_EDGE ( 'NONE', *, *, #5034, .T. ) ;
#63364=VERTEX_POINT ( 'NONE', #27758 ) ;
#63365=CYLINDRICAL_SURFACE ( 'NONE', #42265, 5.000000000000000888 ) ;
#63367=CARTESIAN_POINT ( 'NONE',  ( 11.32888944540964360, 0.8054644877949781456, 13.47643349399415058 ) ) ;
#63370=CARTESIAN_POINT ( 'NONE',  ( -29.54343203963513886, 0.2941795591554937084, 13.49847162130717493 ) ) ;
#63371=CARTESIAN_POINT ( 'NONE',  ( -35.00000000000000000, -9.557269938331609538, 7.561043153947932360 ) ) ;
#63372=VERTEX_POINT ( 'NONE', #63643 ) ;
#63373=CARTESIAN_POINT ( 'NONE',  ( 17.27839441901508977, 12.20388373500084711, 5.771933972472493402 ) ) ;
#63375=ORIENTED_EDGE ( 'NONE', *, *, #32937, .F. ) ;
#63376=CARTESIAN_POINT ( 'NONE',  ( -9.328146843779920871, -11.86223754448519507, -6.454750433817429744 ) ) ;
#63377=EDGE_CURVE ( 'NONE', #41285, #52499, #62919, .T. ) ;
#63378=CYLINDRICAL_SURFACE ( 'NONE', #1047, 2.977897737712716708 ) ;
#63381=EDGE_CURVE ( 'NONE', #40353, #45412, #22922, .T. ) ;
#63384=AXIS2_PLACEMENT_3D ( 'NONE', #9695, #64893, #34634 ) ;
#63385=VERTEX_POINT ( 'NONE', #7822 ) ;
#63390=ORIENTED_EDGE ( 'NONE', *, *, #2080, .T. ) ;
#63393=CARTESIAN_POINT ( 'NONE',  ( -29.46823373269320712, 0.7215570029219251502, -13.48712589208137125 ) ) ;
#63394=CARTESIAN_POINT ( 'NONE',  ( -35.00000000000000000, 2.220215194441899076, 11.98254675519229195 ) ) ;
#63395=ADVANCED_FACE ( 'NONE', ( #8799 ), #2845, .F. ) ;
#63398=EDGE_CURVE ( 'NONE', #28034, #44608, #35121, .T. ) ;
#63400=EDGE_CURVE ( 'NONE', #46189, #25502, #30032, .T. ) ;
#63404=VERTEX_POINT ( 'NONE', #14733 ) ;
#63405=EDGE_CURVE ( 'NONE', #56864, #42378, #5613, .T. ) ;
#63406=CARTESIAN_POINT ( 'NONE',  ( -7.954836218480799026, -1.696952596288976434, -13.39419882916700644 ) ) ;
#63408=DIRECTION ( 'NONE',  ( -0.000000000000000000, -1.000000000000000000, -0.000000000000000000 ) ) ;
#63410=CARTESIAN_POINT ( 'NONE',  ( 35.00000000000000000, 4.725891942574903304, 10.75351884295722193 ) ) ;
#63411=ORIENTED_EDGE ( 'NONE', *, *, #25445, .T. ) ;
#63415=ORIENTED_EDGE ( 'NONE', *, *, #13789, .T. ) ;
#63419=FACE_OUTER_BOUND ( 'NONE', #20321, .T. ) ;
#63421=EDGE_CURVE ( 'NONE', #30828, #10832, #36396, .T. ) ;
#63423=CARTESIAN_POINT ( 'NONE',  ( -32.00000000000000711, 5.510910596163084625E-16, 0.000000000000000000 ) ) ;
#63424=ORIENTED_EDGE ( 'NONE', *, *, #28534, .F. ) ;
#63425=ORIENTED_EDGE ( 'NONE', *, *, #38256, .F. ) ;
#63426=DIRECTION ( 'NONE',  ( 0.000000000000000000, 0.8369827122275363962, 0.5472293298355243030 ) ) ;
#63427=ORIENTED_EDGE ( 'NONE', *, *, #29003, .T. ) ;
#63432=EDGE_CURVE ( 'NONE', #32449, #433, #2428, .T. ) ;
#63438=VERTEX_POINT ( 'NONE', #49690 ) ;
#63439=ORIENTED_EDGE ( 'NONE', *, *, #44522, .F. ) ;
#63443=VERTEX_POINT ( 'NONE', #50677 ) ;
#63444=B_SPLINE_CURVE_WITH_KNOTS ( 'NONE', 3,
 ( #7168, #62062, #6867, #12163, #16171, #22814, #27138, #16821, #1869, #63031, #51766, #27784, #43071, #57075, #36456, #21835, #21498, #53055, #42082, #12473 ),
 .UNSPECIFIED., .F., .F.,
 ( 4, 2, 2, 2, 2, 2, 2, 2, 2, 4 ),
 ( 0.000000000000000000, 0.001199198029652149286, 0.002398396059304298573, 0.003597594088956448076, 0.004197193103782522611, 0.004796792118608597146, 0.005995990148260746215, 0.007195188177912896152, 0.008394386207565045221, 0.009593584237217194291 ),
 .UNSPECIFIED. ) ;
#63448=DIRECTION ( 'NONE',  ( -1.000000000000000000, 0.000000000000000000, 0.000000000000000000 ) ) ;
#63456=DIRECTION ( 'NONE',  ( 0.000000000000000000, -0.01356324068817998940, 0.9999080150203990547 ) ) ;
#63462=CIRCLE ( 'NONE', #64544, 4.999999999999999112 ) ;
#63463=EDGE_CURVE ( 'NONE', #52684, #23475, #55664, .T. ) ;
#63465=DIRECTION ( 'NONE',  ( 1.000000000000000000, 0.000000000000000000, 0.000000000000000000 ) ) ;
#63466=AXIS2_PLACEMENT_3D ( 'NONE', #2762, #47959, #63550 ) ;
#63467=VERTEX_POINT ( 'NONE', #30048 ) ;
#63470=CARTESIAN_POINT ( 'NONE',  ( 35.00000000000000000, 4.705694406421931860E-17, -3.469127814946512892E-15 ) ) ;
#63471=CARTESIAN_POINT ( 'NONE',  ( -25.75517367794919465, -7.863739964200362031, 10.97545609339455019 ) ) ;
#63473=ORIENTED_EDGE ( 'NONE', *, *, #21039, .F. ) ;
#63474=CYLINDRICAL_SURFACE ( 'NONE', #8040, 5.000000000000000888 ) ;
#63475=CYLINDRICAL_SURFACE ( 'NONE', #43803, 13.50000000000000178 ) ;
#63478=CARTESIAN_POINT ( 'NONE',  ( -3.167941684595230623, 12.87051617182347130, 4.089067520392708488 ) ) ;
#63479=EDGE_CURVE ( 'NONE', #50867, #45916, #25771, .T. ) ;
#63481=( BOUNDED_CURVE ( )  B_SPLINE_CURVE ( 3, ( #48126, #28159, #53093, #39095 ),
 .UNSPECIFIED., .F., .F. ) 
 B_SPLINE_CURVE_WITH_KNOTS ( ( 4, 4 ),
 ( 3.532417926517623652, 3.558043830773766736 ),
 .UNSPECIFIED. ) 
 CURVE ( )  GEOMETRIC_REPRESENTATION_ITEM ( )  RATIONAL_B_SPLINE_CURVE ( ( 1.000000000000000000, 0.9999452768345937770, 0.9999452768345937770, 1.000000000000000000 ) ) 
 REPRESENTATION_ITEM ( '' )  );
#63482=ORIENTED_EDGE ( 'NONE', *, *, #46641, .T. ) ;
#63483=EDGE_CURVE ( 'NONE', #63404, #42570, #29393, .T. ) ;
#63484=CYLINDRICAL_SURFACE ( 'NONE', #64684, 12.18650000000000055 ) ;
#63486=DIRECTION ( 'NONE',  ( 0.000000000000000000, -0.01356324068817998940, 0.9999080150203990547 ) ) ;
#63488=EDGE_LOOP ( 'NONE', ( #52726, #57582, #60177, #46086 ) ) ;
#63489=CARTESIAN_POINT ( 'NONE',  ( 8.937200413559443390, 4.476360154859203355, -11.13383131558893346 ) ) ;
#63490=ORIENTED_EDGE ( 'NONE', *, *, #41123, .T. ) ;
#63491=CARTESIAN_POINT ( 'NONE',  ( 37.00000000000000711, 2.143131898507868297E-16, 1.750000000000000000 ) ) ;
#63494=CYLINDRICAL_SURFACE ( 'NONE', #27958, 12.74999999999999822 ) ;
#63499=ORIENTED_EDGE ( 'NONE', *, *, #58352, .T. ) ;
#63500=VERTEX_POINT ( 'NONE', #10413 ) ;
#63501=CARTESIAN_POINT ( 'NONE',  ( 35.00000000000000000, -4.561791185930327508, 11.90598845858537835 ) ) ;
#63503=CIRCLE ( 'NONE', #35916, 5.000000000000001776 ) ;
#63504=DIRECTION ( 'NONE',  ( 0.000000000000000000, 0.3218879778915972878, -0.9467777615094571386 ) ) ;
#63506=DIRECTION ( 'NONE',  ( 1.000000000000000000, -0.000000000000000000, 0.000000000000000000 ) ) ;
#63508=DIRECTION ( 'NONE',  ( -1.000000000000000000, -0.000000000000000000, 0.000000000000000000 ) ) ;
#63510=ORIENTED_EDGE ( 'NONE', *, *, #63735, .F. ) ;
#63511=LINE ( 'NONE', #27613, #54532 ) ;
#63512=DIRECTION ( 'NONE',  ( 1.000000000000000000, 0.000000000000000000, 0.000000000000000000 ) ) ;
#63516=EDGE_CURVE ( 'NONE', #39606, #60329, #61606, .T. ) ;
#63517=AXIS2_PLACEMENT_3D ( 'NONE', #4438, #55945, #56262 ) ;
#63518=CARTESIAN_POINT ( 'NONE',  ( 37.00000000000000711, 4.705694406421931860E-17, -3.469127814946512892E-15 ) ) ;
#63519=ORIENTED_EDGE ( 'NONE', *, *, #16220, .T. ) ;
#63520=CARTESIAN_POINT ( 'NONE',  ( 35.00000000000000000, -9.896810808925339487, 7.110831038798382409 ) ) ;
#63521=ORIENTED_EDGE ( 'NONE', *, *, #3503, .F. ) ;
#63522=VECTOR ( 'NONE', #25048, 1000.000000000000000 ) ;
#63523=DIRECTION ( 'NONE',  ( -1.000000000000000000, 0.000000000000000000, 0.000000000000000000 ) ) ;
#63524=DIRECTION ( 'NONE',  ( -1.000000000000000000, -0.000000000000000000, 0.000000000000000000 ) ) ;
#63526=DIRECTION ( 'NONE',  ( -1.000000000000000000, 0.000000000000000000, -0.000000000000000000 ) ) ;
#63528=CARTESIAN_POINT ( 'NONE',  ( 145.1370849898475797, 3.309064568108273190E-14, 0.000000000000000000 ) ) ;
#63530=ORIENTED_EDGE ( 'NONE', *, *, #54895, .F. ) ;
#63531=DIRECTION ( 'NONE',  ( -1.000000000000000000, 0.000000000000000000, -0.000000000000000000 ) ) ;
#63532=VERTEX_POINT ( 'NONE', #51669 ) ;
#63533=CARTESIAN_POINT ( 'NONE',  ( -36.00000000000000711, -5.556331110570328136, -11.47561260193582733 ) ) ;
#63535=CYLINDRICAL_SURFACE ( 'NONE', #3240, 6.615568257478080305 ) ;
#63537=VERTEX_POINT ( 'NONE', #46017 ) ;
#63538=EDGE_CURVE ( 'NONE', #18920, #56695, #56298, .T. ) ;
#63541=PLANE ( 'NONE',  #36451 ) ;
#63542=CIRCLE ( 'NONE', #18950, 12.74999999999999822 ) ;
#63543=VERTEX_POINT ( 'NONE', #37327 ) ;
#63544=DIRECTION ( 'NONE',  ( 1.000000000000000000, 0.000000000000000000, -0.000000000000000000 ) ) ;
#63550=DIRECTION ( 'NONE',  ( 0.000000000000000000, -0.01356324068817998940, 0.9999080150203990547 ) ) ;
#63551=CIRCLE ( 'NONE', #61464, 5.000000000000001776 ) ;
#63553=CIRCLE ( 'NONE', #19011, 5.000000000000000000 ) ;
#63554=VECTOR ( 'NONE', #53728, 1000.000000000000000 ) ;
#63557=DIRECTION ( 'NONE',  ( 1.000000000000000000, -0.000000000000000000, -0.000000000000000000 ) ) ;
#63563=VECTOR ( 'NONE', #41452, 1000.000000000000000 ) ;
#63566=ORIENTED_EDGE ( 'NONE', *, *, #5431, .T. ) ;
#63567=CARTESIAN_POINT ( 'NONE',  ( -35.00000000000000000, -2.497432891016921008, 11.47758908105693720 ) ) ;
#63571=DIRECTION ( 'NONE',  ( 0.000000000000000000, 0.000000000000000000, -1.000000000000000000 ) ) ;
#63573=CARTESIAN_POINT ( 'NONE',  ( -35.00000000000000000, -0.3137578094508303161, -12.74613886779085448 ) ) ;
#63574=EDGE_LOOP ( 'NONE', ( #48609, #13410, #54433, #34572 ) ) ;
#63578=ADVANCED_FACE ( 'NONE', ( #16719 ), #51985, .T. ) ;
#63580=ORIENTED_EDGE ( 'NONE', *, *, #49636, .F. ) ;
#63581=EDGE_CURVE ( 'NONE', #42983, #9845, #42732, .T. ) ;
#63583=DIRECTION ( 'NONE',  ( -1.000000000000000000, -1.836970198721029688E-16, -0.000000000000000000 ) ) ;
#63585=DIRECTION ( 'NONE',  ( -1.000000000000000000, 0.000000000000000000, -0.000000000000000000 ) ) ;
#63586=ORIENTED_EDGE ( 'NONE', *, *, #50012, .F. ) ;
#63587=DIRECTION ( 'NONE',  ( -0.000000000000000000, -0.000000000000000000, -1.000000000000000000 ) ) ;
#63588=AXIS2_PLACEMENT_3D ( 'NONE', #21781, #42338, #57023 ) ;
#63590=DIRECTION ( 'NONE',  ( -0.000000000000000000, -1.000000000000000000, -0.000000000000000000 ) ) ;
#63591=CARTESIAN_POINT ( 'NONE',  ( -35.00000000000000000, 0.000000000000000000, 0.000000000000000000 ) ) ;
#63592=ORIENTED_EDGE ( 'NONE', *, *, #16660, .T. ) ;
#63594=CYLINDRICAL_SURFACE ( 'NONE', #49032, 6.615568257478080305 ) ;
#63595=ORIENTED_EDGE ( 'NONE', *, *, #57973, .F. ) ;
#63599=AXIS2_PLACEMENT_3D ( 'NONE', #25774, #51048, #57682 ) ;
#63601=AXIS2_PLACEMENT_3D ( 'NONE', #1303, #5975, #21228 ) ;
#63605=CARTESIAN_POINT ( 'NONE',  ( -37.00000000000000711, 0.000000000000000000, 0.000000000000000000 ) ) ;
#63606=DIRECTION ( 'NONE',  ( -1.000000000000000000, 0.000000000000000000, 0.000000000000000000 ) ) ;
#63609=LINE ( 'NONE', #34348, #48640 ) ;
#63611=VERTEX_POINT ( 'NONE', #30690 ) ;
#63614=CIRCLE ( 'NONE', #34930, 12.75000000000000178 ) ;
#63617=DIRECTION ( 'NONE',  ( -0.000000000000000000, -0.000000000000000000, -1.000000000000000000 ) ) ;
#63618=EDGE_CURVE ( 'NONE', #5644, #21398, #52325, .T. ) ;
#63621=VERTEX_POINT ( 'NONE', #28663 ) ;
#63622=CARTESIAN_POINT ( 'NONE',  ( 37.00000000000000711, 2.968224442958566911, 11.81949347079743440 ) ) ;
#63628=AXIS2_PLACEMENT_3D ( 'NONE', #34451, #54753, #9487 ) ;
#63629=CIRCLE ( 'NONE', #47706, 4.999999999999999112 ) ;
#63630=CARTESIAN_POINT ( 'NONE',  ( -11.36165340985849426, -6.759379395737725282, 11.68799443367750612 ) ) ;
#63631=CARTESIAN_POINT ( 'NONE',  ( -10.89441910033722571, -7.164245653068409325, 11.44400242214513241 ) ) ;
#63633=EDGE_CURVE ( 'NONE', #41254, #4226, #12057, .T. ) ;
#63634=VERTEX_POINT ( 'NONE', #43292 ) ;
#63635=CYLINDRICAL_SURFACE ( 'NONE', #43614, 12.74999999999999822 ) ;
#63636=CARTESIAN_POINT ( 'NONE',  ( 35.00000000000000000, 8.052525312709883920, -8.551552972817113130 ) ) ;
#63637=EDGE_CURVE ( 'NONE', #6620, #45368, #62928, .T. ) ;
#63640=DIRECTION ( 'NONE',  ( 0.000000000000000000, -0.01356324068817992175, 0.9999080150203990547 ) ) ;
#63641=VECTOR ( 'NONE', #43539, 1000.000000000000000 ) ;
#63643=CARTESIAN_POINT ( 'NONE',  ( -37.00000000000000711, -9.621072037177057723, 8.366449238204328509 ) ) ;
#63644=DIRECTION ( 'NONE',  ( -1.000000000000000000, 0.000000000000000000, 0.000000000000000000 ) ) ;
#63645=DIRECTION ( 'NONE',  ( 0.000000000000000000, -0.01356324068817998940, 0.9999080150203990547 ) ) ;
#63646=EDGE_LOOP ( 'NONE', ( #49245, #50232, #8044, #14100 ) ) ;
#63648=DIRECTION ( 'NONE',  ( 0.000000000000000000, -0.01356324068817998593, 0.9999080150203990547 ) ) ;
#63649=ORIENTED_EDGE ( 'NONE', *, *, #8449, .F. ) ;
#63650=ORIENTED_EDGE ( 'NONE', *, *, #65600, .F. ) ;
#63651=DIRECTION ( 'NONE',  ( 0.000000000000000000, 0.01356324068817998940, -0.9999080150203990547 ) ) ;
#63657=DIRECTION ( 'NONE',  ( 1.000000000000000000, 0.000000000000000000, -0.000000000000000000 ) ) ;
#63659=DIRECTION ( 'NONE',  ( 0.000000000000000000, -0.4380125133594039433, 0.8989688749565125647 ) ) ;
#63661=CYLINDRICAL_SURFACE ( 'NONE', #2385, 12.18650000000000055 ) ;
#63663=DIRECTION ( 'NONE',  ( 0.000000000000000000, 0.01356324068817991828, -0.9999080150203990547 ) ) ;
#63665=DIRECTION ( 'NONE',  ( 1.000000000000000000, 0.000000000000000000, -0.000000000000000000 ) ) ;
#63667=LINE ( 'NONE', #44371, #17922 ) ;
#63669=ORIENTED_EDGE ( 'NONE', *, *, #17856, .F. ) ;
#63670=CARTESIAN_POINT ( 'NONE',  ( -17.65983200964312516, 7.462298296871543002, 11.25245064142463747 ) ) ;
#63673=CARTESIAN_POINT ( 'NONE',  ( -24.67543046828737729, 11.54621877779729289, 6.997874691641950307 ) ) ;
#63675=CARTESIAN_POINT ( 'NONE',  ( 22.85860294180936947, -4.209476205790071646, 11.23990550851312342 ) ) ;
#63677=DIRECTION ( 'NONE',  ( 1.000000000000000000, 0.000000000000000000, 0.000000000000000000 ) ) ;
#63678=LINE ( 'NONE', #57751, #38399 ) ;
#63682=CIRCLE ( 'NONE', #16949, 12.74999999999999822 ) ;
#63685=ORIENTED_EDGE ( 'NONE', *, *, #40531, .T. ) ;
#63688=CARTESIAN_POINT ( 'NONE',  ( 37.00000000000000711, 4.400442035670943497, -11.96656215839370851 ) ) ;
#63689=CARTESIAN_POINT ( 'NONE',  ( -10.71060692978931783, -9.068875453414413812, 7.876602834927732388 ) ) ;
#63690=FACE_OUTER_BOUND ( 'NONE', #28358, .T. ) ;
#63692=CIRCLE ( 'NONE', #35005, 5.000000000000000000 ) ;
#63693=DIRECTION ( 'NONE',  ( 0.000000000000000000, 0.9796553971857735466, 0.2006870767258926436 ) ) ;
#63697=ADVANCED_FACE ( 'NONE', ( #43969 ), #23354, .T. ) ;
#63699=DIRECTION ( 'NONE',  ( 1.000000000000000000, -0.000000000000000000, 0.000000000000000000 ) ) ;
#63700=ORIENTED_EDGE ( 'NONE', *, *, #25341, .T. ) ;
#63704=CARTESIAN_POINT ( 'NONE',  ( -35.00000000000000000, -11.72195762423409349, -0.7536123767499773862 ) ) ;
#63705=VERTEX_POINT ( 'NONE', #3092 ) ;
#63707=CARTESIAN_POINT ( 'NONE',  ( 35.00000000000000000, 4.603882218679549609, -10.80631716521668828 ) ) ;
#63708=ORIENTED_EDGE ( 'NONE', *, *, #39280, .F. ) ;
#63711=DIRECTION ( 'NONE',  ( 0.000000000000000000, 0.8989688749565143411, 0.4380125133594006681 ) ) ;
#63712=DIRECTION ( 'NONE',  ( 0.000000000000000000, -0.01356324068817998940, 0.9999080150203990547 ) ) ;
#63714=ORIENTED_EDGE ( 'NONE', *, *, #43234, .T. ) ;
#63715=CARTESIAN_POINT ( 'NONE',  ( -47.00000000000000711, 0.000000000000000000, 0.000000000000000000 ) ) ;
#63719=EDGE_CURVE ( 'NONE', #7910, #44848, #39290, .T. ) ;
#63720=VECTOR ( 'NONE', #41571, 1000.000000000000000 ) ;
#63725=CARTESIAN_POINT ( 'NONE',  ( -20.32764961709473184, -11.53253557995959788, -3.332158659635061859 ) ) ;
#63726=CARTESIAN_POINT ( 'NONE',  ( 28.77117211474471503, 12.20468600494871403, 5.784778099440913479 ) ) ;
#63728=VERTEX_POINT ( 'NONE', #55591 ) ;
#63732=FACE_OUTER_BOUND ( 'NONE', #49425, .T. ) ;
#63733=CARTESIAN_POINT ( 'NONE',  ( -35.00000000000000000, 6.475373545682302279, 10.32377448871670467 ) ) ;
#63734=VECTOR ( 'NONE', #46677, 1000.000000000000000 ) ;
#63735=EDGE_CURVE ( 'NONE', #27041, #1393, #19420, .T. ) ;
#63736=EDGE_LOOP ( 'NONE', ( #7079, #18558, #55987, #24784 ) ) ;
#63738=ORIENTED_EDGE ( 'NONE', *, *, #46672, .T. ) ;
#63740=DIRECTION ( 'NONE',  ( 1.000000000000000000, -0.000000000000000000, -0.000000000000000000 ) ) ;
#63742=CARTESIAN_POINT ( 'NONE',  ( 35.00000000000000000, 12.70128625845192616, -1.113475361586538481 ) ) ;
#63744=LINE ( 'NONE', #39462, #52272 ) ;
#63750=ORIENTED_EDGE ( 'NONE', *, *, #28548, .T. ) ;
#63752=EDGE_CURVE ( 'NONE', #54995, #50756, #24022, .T. ) ;
#63753=CYLINDRICAL_SURFACE ( 'NONE', #35339, 2.809571291727933851 ) ;
#63754=LINE ( 'NONE', #53813, #23459 ) ;
#63756=DIRECTION ( 'NONE',  ( 0.000000000000000000, 0.4380125133593975595, -0.8989688749565157844 ) ) ;
#63758=CARTESIAN_POINT ( 'NONE',  ( -35.00000000000000000, 5.015831474386455824, -10.62137734850263016 ) ) ;
#63759=ORIENTED_EDGE ( 'NONE', *, *, #24987, .F. ) ;
#63760=ORIENTED_EDGE ( 'NONE', *, *, #4882, .F. ) ;
#63762=VECTOR ( 'NONE', #44774, 1000.000000000000000 ) ;
#63766=ORIENTED_EDGE ( 'NONE', *, *, #20161, .T. ) ;
#63767=CARTESIAN_POINT ( 'NONE',  ( 35.00000000000000000, -11.42599468261425955, 4.237620530777920003 ) ) ;
#63768=EDGE_CURVE ( 'NONE', #48033, #3518, #17277, .T. ) ;
#63773=DIRECTION ( 'NONE',  ( -1.000000000000000000, 0.000000000000000000, -0.000000000000000000 ) ) ;
#63775=CIRCLE ( 'NONE', #43603, 5.000000000000000888 ) ;
#63777=EDGE_CURVE ( 'NONE', #27211, #44463, #48250, .T. ) ;
#63778=ORIENTED_EDGE ( 'NONE', *, *, #41270, .T. ) ;
#63779=DIRECTION ( 'NONE',  ( 1.000000000000000000, 0.000000000000000000, -0.000000000000000000 ) ) ;
#63783=CARTESIAN_POINT ( 'NONE',  ( -35.00000000000000000, 0.000000000000000000, 0.000000000000000000 ) ) ;
#63784=CARTESIAN_POINT ( 'NONE',  ( 29.66268546517093796, 8.643908359168339217, 8.338268269882382455 ) ) ;
#63787=DIRECTION ( 'NONE',  ( 1.000000000000000000, -0.000000000000000000, -0.000000000000000000 ) ) ;
#63790=AXIS2_PLACEMENT_3D ( 'NONE', #29076, #34378, #49385 ) ;
#63794=AXIS2_PLACEMENT_3D ( 'NONE', #15136, #39761, #24458 ) ;
#63795=ORIENTED_EDGE ( 'NONE', *, *, #40026, .T. ) ;
#63796=CARTESIAN_POINT ( 'NONE',  ( -10.95212338237647920, -9.902220863987562183, 6.778349501228839280 ) ) ;
#63798=CARTESIAN_POINT ( 'NONE',  ( 12.67279215479052112, -12.94353850923882909, -3.840530738146114675 ) ) ;
#63799=AXIS2_PLACEMENT_3D ( 'NONE', #61749, #41801, #16854 ) ;
#63800=LINE ( 'NONE', #23927, #13950 ) ;
#63802=EDGE_CURVE ( 'NONE', #37649, #12199, #50273, .T. ) ;
#63803=ORIENTED_EDGE ( 'NONE', *, *, #18866, .T. ) ;
#63810=CIRCLE ( 'NONE', #17115, 5.000000000000000888 ) ;
#63811=CARTESIAN_POINT ( 'NONE',  ( 35.00000000000000000, -12.01765980939840439, 2.021542716731525413 ) ) ;
#63812=VERTEX_POINT ( 'NONE', #20323 ) ;
#63813=DIRECTION ( 'NONE',  ( 0.000000000000000000, -0.01356324068817991828, 0.9999080150203990547 ) ) ;
#63814=AXIS2_PLACEMENT_3D ( 'NONE', #51747, #31119, #1199 ) ;
#63817=VECTOR ( 'NONE', #3162, 1000.000000000000000 ) ;
#63818=VECTOR ( 'NONE', #31428, 1000.000000000000000 ) ;
#63819=AXIS2_PLACEMENT_3D ( 'NONE', #33960, #61434, #56465 ) ;
#63821=ORIENTED_EDGE ( 'NONE', *, *, #6470, .T. ) ;
#63823=EDGE_LOOP ( 'NONE', ( #61461, #57060, #13139, #64285 ) ) ;
#63824=CARTESIAN_POINT ( 'NONE',  ( -37.00000000000000711, 6.307491713049167004, -9.908974237959577991 ) ) ;
#63826=AXIS2_PLACEMENT_3D ( 'NONE', #1887, #17176, #57762 ) ;
#63830=ORIENTED_EDGE ( 'NONE', *, *, #20942, .F. ) ;
#63831=EDGE_LOOP ( 'NONE', ( #18542, #65166, #44916, #58884 ) ) ;
#63835=ADVANCED_FACE ( 'NONE', ( #29631 ), #49938, .T. ) ;
#63838=CARTESIAN_POINT ( 'NONE',  ( -35.00000000000000000, -1.039216533672986387, 11.70009620280411333 ) ) ;
#63839=AXIS2_PLACEMENT_3D ( 'NONE', #65017, #14471, #19816 ) ;
#63841=ORIENTED_EDGE ( 'NONE', *, *, #18854, .T. ) ;
#63844=DIRECTION ( 'NONE',  ( -1.000000000000000000, -0.000000000000000000, -0.000000000000000000 ) ) ;
#63847=ORIENTED_EDGE ( 'NONE', *, *, #15516, .F. ) ;
#63850=CARTESIAN_POINT ( 'NONE',  ( -18.49080574448724690, 11.99999999999999645, 2.510045011421233839E-15 ) ) ;
#63854=CARTESIAN_POINT ( 'NONE',  ( 37.00000000000000711, 4.705694406421931860E-17, -3.469127814946512892E-15 ) ) ;
#63856=CYLINDRICAL_SURFACE ( 'NONE', #12562, 12.75000000000000178 ) ;
#63858=DIRECTION ( 'NONE',  ( 0.9207114435679737419, 0.000000000000000000, -0.3902440745007897949 ) ) ;
#63859=DIRECTION ( 'NONE',  ( -1.000000000000000000, -0.000000000000000000, 0.000000000000000000 ) ) ;
#63860=ORIENTED_EDGE ( 'NONE', *, *, #4596, .F. ) ;
#63862=AXIS2_PLACEMENT_3D ( 'NONE', #61487, #46226, #667 ) ;
#63863=ORIENTED_EDGE ( 'NONE', *, *, #60422, .F. ) ;
#63866=CARTESIAN_POINT ( 'NONE',  ( -35.00000000000000000, 0.000000000000000000, 0.000000000000000000 ) ) ;
#63868=AXIS2_PLACEMENT_3D ( 'NONE', #785, #6767, #26067 ) ;
#63869=ADVANCED_FACE ( 'NONE', ( #60900 ), #714, .T. ) ;
#63870=ORIENTED_EDGE ( 'NONE', *, *, #13296, .F. ) ;
#63872=DIRECTION ( 'NONE',  ( 0.000000000000000000, 0.000000000000000000, -1.000000000000000000 ) ) ;
#63875=VECTOR ( 'NONE', #31210, 1000.000000000000000 ) ;
#63876=AXIS2_PLACEMENT_3D ( 'NONE', #5325, #6313, #61826 ) ;
#63877=AXIS2_PLACEMENT_3D ( 'NONE', #39699, #64621, #30045 ) ;
#63878=VERTEX_POINT ( 'NONE', #11653 ) ;
#63879=EDGE_CURVE ( 'NONE', #58896, #46955, #31294, .T. ) ;
#63880=DIRECTION ( 'NONE',  ( -0.8758382566188793739, 0.4826047536471247956, 0.000000000000000000 ) ) ;
#63882=ORIENTED_EDGE ( 'NONE', *, *, #10552, .F. ) ;
#63884=DIRECTION ( 'NONE',  ( 0.000000000000000000, -0.9551603052523448545, 0.2960891610144612551 ) ) ;
#63885=DIRECTION ( 'NONE',  ( 1.000000000000000000, 0.000000000000000000, 0.000000000000000000 ) ) ;
#63888=CARTESIAN_POINT ( 'NONE',  ( -35.00000000000000000, 3.213188559034398040, -11.29812557209473667 ) ) ;
#63889=ORIENTED_EDGE ( 'NONE', *, *, #23067, .T. ) ;
#63890=B_SPLINE_CURVE_WITH_KNOTS ( 'NONE', 3,
 ( #43518, #23594, #13908, #39187, #64771, #53540 ),
 .UNSPECIFIED., .F., .F.,
 ( 4, 2, 4 ),
 ( 9.965227682168975268E-18, 0.001456900940518678468, 0.002913801881037346962 ),
 .UNSPECIFIED. ) ;
#63892=ADVANCED_FACE ( 'NONE', ( #52577 ), #62851, .T. ) ;
#63893=CIRCLE ( 'NONE', #53275, 5.000000000000000000 ) ;
#63894=CIRCLE ( 'NONE', #29905, 12.74999999999999822 ) ;
#63895=CIRCLE ( 'NONE', #28820, 5.000000000000000000 ) ;
#63896=EDGE_CURVE ( 'NONE', #37836, #58571, #42218, .T. ) ;
#63899=EDGE_CURVE ( 'NONE', #7557, #48895, #52880, .T. ) ;
#63900=CARTESIAN_POINT ( 'NONE',  ( -28.71071236259717807, 3.670376459565063421, 11.42521152978763155 ) ) ;
#63901=FACE_OUTER_BOUND ( 'NONE', #11658, .T. ) ;
#63903=CARTESIAN_POINT ( 'NONE',  ( 7.265852764334843172, -6.972182010717725476, -9.777817421782533103 ) ) ;
#63905=AXIS2_PLACEMENT_3D ( 'NONE', #57344, #32693, #38024 ) ;
#63906=ORIENTED_EDGE ( 'NONE', *, *, #52381, .T. ) ;
#63907=CARTESIAN_POINT ( 'NONE',  ( 12.48116093077668154, -11.51604155625666515, -3.378324846013889715 ) ) ;
#63908=ORIENTED_EDGE ( 'NONE', *, *, #10282, .T. ) ;
#63911=CARTESIAN_POINT ( 'NONE',  ( 12.10998784662220729, 25.00000000000000000, -8.526922110106905706 ) ) ;
#63912=VERTEX_POINT ( 'NONE', #37593 ) ;
#63913=CARTESIAN_POINT ( 'NONE',  ( -27.30970368864377207, 11.82098433594889109, -2.066507538000780464 ) ) ;
#63915=ORIENTED_EDGE ( 'NONE', *, *, #16447, .F. ) ;
#63916=CIRCLE ( 'NONE', #16173, 12.18649999999999878 ) ;
#63917=ORIENTED_EDGE ( 'NONE', *, *, #14260, .F. ) ;
#63919=CARTESIAN_POINT ( 'NONE',  ( 29.70647529080776650, -10.34008595192405977, 8.691137256207259298 ) ) ;
#63921=EDGE_CURVE ( 'NONE', #9046, #25109, #42547, .T. ) ;
#63922=AXIS2_PLACEMENT_3D ( 'NONE', #56089, #30491, #10528 ) ;
#63923=ADVANCED_FACE ( 'NONE', ( #32573 ), #16973, .T. ) ;
#63924=B_SPLINE_CURVE_WITH_KNOTS ( 'NONE', 3,
 ( #36756, #545, #57052, #35440, #20810, #55741, #41078, #15798, #10171, #36076, #26447, #61053, #30451, #25465, #10828, #31113, #15483, #35749, #51428, #5876, #26132, #854 ),
 .UNSPECIFIED., .F., .F.,
 ( 4, 2, 2, 2, 2, 2, 2, 2, 2, 2, 4 ),
 ( 0.000000000000000000, 0.0009985635585561321737, 0.001497845337834194032, 0.001997127117112255674, 0.002496408896390317749, 0.002995690675668379391, 0.003994254234224500939, 0.004992817792780622488, 0.005991381351336744036, 0.006989944909892865585, 0.007988508468448986266 ),
 .UNSPECIFIED. ) ;
#63925=AXIS2_PLACEMENT_3D ( 'NONE', #3830, #48056, #32716 ) ;
#63926=VERTEX_POINT ( 'NONE', #27946 ) ;
#63928=CARTESIAN_POINT ( 'NONE',  ( 1.937341776064131160, 1.073324468469882165, 13.46190213546479875 ) ) ;
#63929=CARTESIAN_POINT ( 'NONE',  ( 19.67311005600952711, -0.7004819783312107306, 25.00000000000000000 ) ) ;
#63930=DIRECTION ( 'NONE',  ( 0.000000000000000000, 0.01356324068817998940, -0.9999080150203990547 ) ) ;
#63932=CARTESIAN_POINT ( 'NONE',  ( -37.00000000000000711, 0.000000000000000000, 0.000000000000000000 ) ) ;
#63934=CARTESIAN_POINT ( 'NONE',  ( -29.51989888335948820, -3.283075202658972902, -11.54828650488808250 ) ) ;
#63935=CARTESIAN_POINT ( 'NONE',  ( 37.00000000000000711, 4.705694406421931860E-17, -3.469127814946512892E-15 ) ) ;
#63936=EDGE_LOOP ( 'NONE', ( #50614, #6439, #25590, #39921 ) ) ;
#63938=ORIENTED_EDGE ( 'NONE', *, *, #23683, .T. ) ;
#63941=ORIENTED_EDGE ( 'NONE', *, *, #19697, .T. ) ;
#63943=AXIS2_PLACEMENT_3D ( 'NONE', #39985, #55279, #13406 ) ;
#63946=CARTESIAN_POINT ( 'NONE',  ( 35.00000000000000000, -5.636262487437393887, -10.80478261802180207 ) ) ;
#63955=EDGE_CURVE ( 'NONE', #57557, #60039, #34299, .T. ) ;
#63959=CARTESIAN_POINT ( 'NONE',  ( 35.00000000000000000, 4.705694406421931860E-17, -3.469127814946512892E-15 ) ) ;
#63962=CARTESIAN_POINT ( 'NONE',  ( -47.00000000000000711, 0.000000000000000000, 0.000000000000000000 ) ) ;
#63964=ORIENTED_EDGE ( 'NONE', *, *, #43146, .F. ) ;
#63967=LINE ( 'NONE', #34029, #65329 ) ;
#63968=B_SPLINE_CURVE_WITH_KNOTS ( 'NONE', 3,
 ( #42579, #41619, #36638, #62881 ),
 .UNSPECIFIED., .F., .F.,
 ( 4, 4 ),
 ( 0.000000000000000000, 0.002391677032556851785 ),
 .UNSPECIFIED. ) ;
#63970=EDGE_CURVE ( 'NONE', #20003, #60501, #42900, .T. ) ;
#63972=ADVANCED_FACE ( 'NONE', ( #58204 ), #12625, .T. ) ;
#63973=AXIS2_PLACEMENT_3D ( 'NONE', #53272, #58259, #57619 ) ;
#63976=AXIS2_PLACEMENT_3D ( 'NONE', #5257, #29849, #14546 ) ;
#63978=CARTESIAN_POINT ( 'NONE',  ( -7.757791118878088810, -1.606844526199946221, 13.40434846090924204 ) ) ;
#63979=EDGE_CURVE ( 'NONE', #35317, #54327, #33258, .T. ) ;
#63980=CARTESIAN_POINT ( 'NONE',  ( -9.921280308801140535, -4.188103626763136411, 12.83514249654943207 ) ) ;
#63981=VERTEX_POINT ( 'NONE', #8971 ) ;
#63984=DIRECTION ( 'NONE',  ( 0.000000000000000000, 0.6269146997507930585, 0.7790879021242551605 ) ) ;
#63985=AXIS2_PLACEMENT_3D ( 'NONE', #64481, #18948, #38224 ) ;
#63986=DIRECTION ( 'NONE',  ( -1.000000000000000000, 0.000000000000000000, 0.000000000000000000 ) ) ;
#63987=CYLINDRICAL_SURFACE ( 'NONE', #20254, 12.18649999999999878 ) ;
#63988=AXIS2_PLACEMENT_3D ( 'NONE', #41263, #46593, #56236 ) ;
#63989=VERTEX_POINT ( 'NONE', #54539 ) ;
#63990=DIRECTION ( 'NONE',  ( 0.000000000000000000, 0.9987865678893279586, -0.04924826701374244303 ) ) ;
#63991=CARTESIAN_POINT ( 'NONE',  ( -8.966652592027504198, -7.722572881235366005, -9.193810145090301589 ) ) ;
#63992=CIRCLE ( 'NONE', #55508, 12.18649999999999878 ) ;
#63993=PLANE ( 'NONE',  #19060 ) ;
#63994=ORIENTED_EDGE ( 'NONE', *, *, #27405, .F. ) ;
#63997=VERTEX_POINT ( 'NONE', #64798 ) ;
#63999=DIRECTION ( 'NONE',  ( -1.000000000000000000, 0.000000000000000000, -0.000000000000000000 ) ) ;
#64000=EDGE_CURVE ( 'NONE', #17645, #11684, #24587, .T. ) ;
#64001=ORIENTED_EDGE ( 'NONE', *, *, #59646, .T. ) ;
#64003=ADVANCED_FACE ( 'NONE', ( #23951 ), #29253, .T. ) ;
#64004=CARTESIAN_POINT ( 'NONE',  ( -21.04919400413958996, -12.98042452237757161, -3.710884547572582459 ) ) ;
#64005=FACE_OUTER_BOUND ( 'NONE', #46057, .T. ) ;
#64006=DIRECTION ( 'NONE',  ( -1.000000000000000000, 0.000000000000000000, 0.000000000000000000 ) ) ;
#64008=FACE_OUTER_BOUND ( 'NONE', #9676, .T. ) ;
#64011=ORIENTED_EDGE ( 'NONE', *, *, #36386, .F. ) ;
#64012=CYLINDRICAL_SURFACE ( 'NONE', #21086, 5.000000000000000888 ) ;
#64013=EDGE_LOOP ( 'NONE', ( #21357, #18996, #46269, #63227 ) ) ;
#64014=EDGE_CURVE ( 'NONE', #29486, #47095, #56633, .T. ) ;
#64015=AXIS2_PLACEMENT_3D ( 'NONE', #12248, #1951, #22223 ) ;
#64017=CARTESIAN_POINT ( 'NONE',  ( -15.49418265353465785, 8.465735697530092807, 10.51590495851239915 ) ) ;
#64019=AXIS2_PLACEMENT_3D ( 'NONE', #35741, #14480, #39434 ) ;
#64020=DIRECTION ( 'NONE',  ( 0.000000000000000000, -0.1387779952735677669, 0.9903235168508569553 ) ) ;
#64022=DIRECTION ( 'NONE',  ( 1.000000000000000000, 0.000000000000000000, 0.000000000000000000 ) ) ;
#64025=CYLINDRICAL_SURFACE ( 'NONE', #16645, 13.50000000000000178 ) ;
#64027=CARTESIAN_POINT ( 'NONE',  ( -35.00000000000000000, 0.000000000000000000, 0.000000000000000000 ) ) ;
#64028=EDGE_LOOP ( 'NONE', ( #54970, #42496, #46015, #36807 ) ) ;
#64030=CARTESIAN_POINT ( 'NONE',  ( -35.00000000000000000, 0.000000000000000000, 0.000000000000000000 ) ) ;
#64036=CYLINDRICAL_SURFACE ( 'NONE', #59704, 4.999999999999999112 ) ;
#64041=DIRECTION ( 'NONE',  ( -1.000000000000000000, -0.000000000000000000, -0.000000000000000000 ) ) ;
#64042=ORIENTED_EDGE ( 'NONE', *, *, #29269, .F. ) ;
#64043=ORIENTED_EDGE ( 'NONE', *, *, #43343, .F. ) ;
#64049=VECTOR ( 'NONE', #32587, 1000.000000000000000 ) ;
#64050=DIRECTION ( 'NONE',  ( -1.000000000000000000, 0.000000000000000000, 0.000000000000000000 ) ) ;
#64051=EDGE_CURVE ( 'NONE', #35661, #18660, #50202, .T. ) ;
#64052=ORIENTED_EDGE ( 'NONE', *, *, #17715, .F. ) ;
#64053=CARTESIAN_POINT ( 'NONE',  ( 5.982824234232984928, -9.655473559075929302, -9.442377055868243829 ) ) ;
#64054=CARTESIAN_POINT ( 'NONE',  ( -35.00000000000000000, -12.21925492305359562, -3.640372113593682624 ) ) ;
#64057=CYLINDRICAL_SURFACE ( 'NONE', #18035, 12.74999999999999822 ) ;
#64059=CIRCLE ( 'NONE', #36486, 12.74999999999999822 ) ;
#64060=CARTESIAN_POINT ( 'NONE',  ( -36.00000000000000711, 12.60630747491665993, -1.908798535168239718 ) ) ;
#64062=CIRCLE ( 'NONE', #24816, 5.000000000000000888 ) ;
#64063=DIRECTION ( 'NONE',  ( 1.000000000000000000, -0.000000000000000000, 0.000000000000000000 ) ) ;
#64065=AXIS2_PLACEMENT_3D ( 'NONE', #46335, #774, #61599 ) ;
#64066=AXIS2_PLACEMENT_3D ( 'NONE', #51527, #15899, #34860 ) ;
#64071=VERTEX_POINT ( 'NONE', #30233 ) ;
#64073=DIRECTION ( 'NONE',  ( 0.000000000000000000, 0.01356324068817992175, -0.9999080150203990547 ) ) ;
#64074=CIRCLE ( 'NONE', #32223, 5.000000000000000000 ) ;
#64076=ORIENTED_EDGE ( 'NONE', *, *, #47684, .F. ) ;
#64078=CYLINDRICAL_SURFACE ( 'NONE', #54423, 12.75000000000000178 ) ;
#64079=LINE ( 'NONE', #19177, #54239 ) ;
#64080=CIRCLE ( 'NONE', #39631, 12.74999999999999822 ) ;
#64082=CARTESIAN_POINT ( 'NONE',  ( 35.00000000000000000, 10.28547182238015978, 5.672855678558568648 ) ) ;
#64083=AXIS2_PLACEMENT_3D ( 'NONE', #40356, #29724, #39721 ) ;
#64084=CARTESIAN_POINT ( 'NONE',  ( -37.00000000000000711, 0.000000000000000000, 0.000000000000000000 ) ) ;
#64085=ORIENTED_EDGE ( 'NONE', *, *, #55046, .F. ) ;
#64086=DIRECTION ( 'NONE',  ( -1.000000000000000000, 0.000000000000000000, -0.000000000000000000 ) ) ;
#64087=EDGE_CURVE ( 'NONE', #56264, #41059, #61529, .T. ) ;
#64094=AXIS2_PLACEMENT_3D ( 'NONE', #23315, #23655, #18000 ) ;
#64095=DIRECTION ( 'NONE',  ( 1.000000000000000000, 0.000000000000000000, -0.000000000000000000 ) ) ;
#64096=CARTESIAN_POINT ( 'NONE',  ( -17.19065538327509657, 2.658487034042159802, -13.23633903133955414 ) ) ;
#64097=VERTEX_POINT ( 'NONE', #33901 ) ;
#64098=ORIENTED_EDGE ( 'NONE', *, *, #23293, .F. ) ;
#64100=ORIENTED_EDGE ( 'NONE', *, *, #54503, .T. ) ;
#64105=ORIENTED_EDGE ( 'NONE', *, *, #17502, .T. ) ;
#64106=DIRECTION ( 'NONE',  ( -1.000000000000000000, 0.000000000000000000, -0.000000000000000000 ) ) ;
#64107=DIRECTION ( 'NONE',  ( 1.000000000000000000, 0.000000000000000000, -0.000000000000000000 ) ) ;
#64112=EDGE_CURVE ( 'NONE', #47275, #59432, #4613, .T. ) ;
#64113=VECTOR ( 'NONE', #60396, 1000.000000000000000 ) ;
#64114=DIRECTION ( 'NONE',  ( 1.000000000000000000, -0.000000000000000000, 0.000000000000000000 ) ) ;
#64115=CIRCLE ( 'NONE', #57777, 12.18650000000000055 ) ;
#64117=VERTEX_POINT ( 'NONE', #4973 ) ;
#64118=CARTESIAN_POINT ( 'NONE',  ( -35.00000000000000000, -2.772148766916031182, -11.86701198550359315 ) ) ;
#64119=EDGE_CURVE ( 'NONE', #9450, #14653, #60846, .T. ) ;
#64120=DIRECTION ( 'NONE',  ( -1.000000000000000000, -0.000000000000000000, 0.000000000000000000 ) ) ;
#64121=VECTOR ( 'NONE', #42059, 1000.000000000000000 ) ;
#64123=CARTESIAN_POINT ( 'NONE',  ( -37.00000000000000711, -7.146664589317976102, 9.321877890560418933 ) ) ;
#64125=CARTESIAN_POINT ( 'NONE',  ( -37.00000000000000711, -8.235637554476577193, -9.733281772932249609 ) ) ;
#64126=VERTEX_POINT ( 'NONE', #46833 ) ;
#64127=CIRCLE ( 'NONE', #48211, 12.18649999999999878 ) ;
#64128=DIRECTION ( 'NONE',  ( 1.000000000000000000, -0.000000000000000000, -0.000000000000000000 ) ) ;
#64129=AXIS2_PLACEMENT_3D ( 'NONE', #63707, #47147, #32144 ) ;
#64131=FACE_OUTER_BOUND ( 'NONE', #988, .T. ) ;
#64132=DIRECTION ( 'NONE',  ( 1.000000000000000000, 0.000000000000000000, 0.000000000000000000 ) ) ;
#64133=CARTESIAN_POINT ( 'NONE',  ( 29.73648668909451587, 7.552544575588006737, 9.338272984228474627 ) ) ;
#64136=DIRECTION ( 'NONE',  ( 1.000000000000000000, 0.000000000000000000, 0.000000000000000000 ) ) ;
#64138=DIRECTION ( 'NONE',  ( -0.8514458006899927600, 0.000000000000000000, -0.5244426074294281648 ) ) ;
#64140=VECTOR ( 'NONE', #62140, 1000.000000000000000 ) ;
#64141=VERTEX_POINT ( 'NONE', #21580 ) ;
#64143=VERTEX_POINT ( 'NONE', #41498 ) ;
#64144=CARTESIAN_POINT ( 'NONE',  ( -35.00000000000000000, 9.512294188641000403, -6.891188680298720115 ) ) ;
#64146=VECTOR ( 'NONE', #31798, 1000.000000000000000 ) ;
#64147=LINE ( 'NONE', #32880, #57947 ) ;
#64148=CARTESIAN_POINT ( 'NONE',  ( 35.00000000000000000, 4.705694406421931860E-17, -3.469127814946512892E-15 ) ) ;
#64149=DIRECTION ( 'NONE',  ( -1.000000000000000000, 0.000000000000000000, 0.000000000000000000 ) ) ;
#64150=ORIENTED_EDGE ( 'NONE', *, *, #27308, .F. ) ;
#64154=DIRECTION ( 'NONE',  ( 0.000000000000000000, -0.01356324068817998940, 0.9999080150203990547 ) ) ;
#64157=AXIS2_PLACEMENT_3D ( 'NONE', #7788, #28072, #64288 ) ;
#64161=VERTEX_POINT ( 'NONE', #35843 ) ;
#64163=DIRECTION ( 'NONE',  ( -1.000000000000000000, 0.000000000000000000, -0.000000000000000000 ) ) ;
#64164=CIRCLE ( 'NONE', #35480, 12.18650000000000055 ) ;
#64167=CARTESIAN_POINT ( 'NONE',  ( 6.401101480914875630, -8.123926338959122972, 10.78346351568197470 ) ) ;
#64168=EDGE_LOOP ( 'NONE', ( #12243, #14549, #55589, #61301 ) ) ;
#64169=ORIENTED_EDGE ( 'NONE', *, *, #30056, .T. ) ;
#64174=CARTESIAN_POINT ( 'NONE',  ( 35.00000000000000000, 10.91536515067648239, 4.339012074899986970 ) ) ;
#64177=EDGE_CURVE ( 'NONE', #35942, #54366, #16586, .T. ) ;
#64178=ORIENTED_EDGE ( 'NONE', *, *, #7586, .T. ) ;
#64181=CARTESIAN_POINT ( 'NONE',  ( -35.00000000000000000, 10.91072401419410554, 5.428340790341743549 ) ) ;
#64182=CIRCLE ( 'NONE', #35503, 12.18650000000000055 ) ;
#64183=DIRECTION ( 'NONE',  ( 0.000000000000000000, -0.5243256840888623760, -0.8515178078024829844 ) ) ;
#64185=ORIENTED_EDGE ( 'NONE', *, *, #8383, .T. ) ;
#64188=VERTEX_POINT ( 'NONE', #36852 ) ;
#64190=CIRCLE ( 'NONE', #59928, 12.75000000000000178 ) ;
#64191=CARTESIAN_POINT ( 'NONE',  ( -35.00000000000000000, -3.827046518385164742, 11.56998259273176188 ) ) ;
#64193=ORIENTED_EDGE ( 'NONE', *, *, #30380, .T. ) ;
#64194=ORIENTED_EDGE ( 'NONE', *, *, #24711, .F. ) ;
#64195=CARTESIAN_POINT ( 'NONE',  ( -4.989057617119011745, -0.9162120371760335003, 11.96497202265570259 ) ) ;
#64198=ADVANCED_FACE ( 'NONE', ( #30866 ), #56144, .T. ) ;
#64199=DIRECTION ( 'NONE',  ( 0.000000000000000000, 0.01356324068817992175, -0.9999080150203990547 ) ) ;
#64200=ORIENTED_EDGE ( 'NONE', *, *, #48114, .F. ) ;
#64201=ORIENTED_EDGE ( 'NONE', *, *, #45696, .F. ) ;
#64203=LINE ( 'NONE', #50234, #42583 ) ;
#64204=CARTESIAN_POINT ( 'NONE',  ( 35.00000000000000000, 6.564808257521768553, -10.93004082984021075 ) ) ;
#64205=VECTOR ( 'NONE', #34521, 1000.000000000000000 ) ;
#64206=DIRECTION ( 'NONE',  ( 0.000000000000000000, 0.2618041379715562722, -0.9651210252299813330 ) ) ;
#64209=ORIENTED_EDGE ( 'NONE', *, *, #134, .F. ) ;
#64210=CARTESIAN_POINT ( 'NONE',  ( 37.00000000000000711, -11.17622378668003691, 3.614449339633606595 ) ) ;
#64212=CARTESIAN_POINT ( 'NONE',  ( 37.00000000000000711, 9.557269938331552694, -7.561043153948004303 ) ) ;
#64214=ORIENTED_EDGE ( 'NONE', *, *, #18431, .T. ) ;
#64215=DIRECTION ( 'NONE',  ( 1.000000000000000000, -0.000000000000000000, 0.000000000000000000 ) ) ;
#64218=ORIENTED_EDGE ( 'NONE', *, *, #59741, .T. ) ;
#64221=VERTEX_POINT ( 'NONE', #15260 ) ;
#64222=CARTESIAN_POINT ( 'NONE',  ( -24.75896104215371096, -11.63928102839248879, 6.841611787138283773 ) ) ;
#64226=ORIENTED_EDGE ( 'NONE', *, *, #18942, .T. ) ;
#64227=DIRECTION ( 'NONE',  ( 0.000000000000000000, -0.1118654143051476951, -0.9937233664769775654 ) ) ;
#64228=AXIS2_PLACEMENT_3D ( 'NONE', #24346, #63590, #29341 ) ;
#64231=CARTESIAN_POINT ( 'NONE',  ( 9.022832866668583307, 5.316194047393634214, -12.41044072607060400 ) ) ;
#64234=CARTESIAN_POINT ( 'NONE',  ( 4.838183347715137472, -10.56890113247325047, -5.693500808758303222 ) ) ;
#64235=CARTESIAN_POINT ( 'NONE',  ( -36.00000000000000711, -0.1414404973751254013, -12.74921544981111410 ) ) ;
#64240=VERTEX_POINT ( 'NONE', #42819 ) ;
#64241=DIRECTION ( 'NONE',  ( -0.02770351589312032917, 0.9996161839461982224, 0.000000000000000000 ) ) ;
#64244=DIRECTION ( 'NONE',  ( -1.000000000000000000, -0.000000000000000000, -0.000000000000000000 ) ) ;
#64246=EDGE_CURVE ( 'NONE', #36643, #27041, #26853, .T. ) ;
#64247=ORIENTED_EDGE ( 'NONE', *, *, #62425, .T. ) ;
#64249=ORIENTED_EDGE ( 'NONE', *, *, #24025, .F. ) ;
#64250=ORIENTED_EDGE ( 'NONE', *, *, #62214, .T. ) ;
#64251=CARTESIAN_POINT ( 'NONE',  ( -36.00000000000000711, 0.6593684648222306599, -12.73293890771482850 ) ) ;
#64253=EDGE_CURVE ( 'NONE', #35323, #21896, #55531, .T. ) ;
#64254=ORIENTED_EDGE ( 'NONE', *, *, #16861, .F. ) ;
#64257=CARTESIAN_POINT ( 'NONE',  ( 24.82652845881425208, 10.42385221765396608, -8.578654028722157321 ) ) ;
#64259=ORIENTED_EDGE ( 'NONE', *, *, #15424, .T. ) ;
#64260=CARTESIAN_POINT ( 'NONE',  ( 35.00000000000000000, 11.65554240571056788, -1.456211999474385843 ) ) ;
#64262=CYLINDRICAL_SURFACE ( 'NONE', #112, 5.000000000000000888 ) ;
#64263=FACE_OUTER_BOUND ( 'NONE', #7076, .T. ) ;
#64265=ORIENTED_EDGE ( 'NONE', *, *, #10751, .F. ) ;
#64267=ORIENTED_EDGE ( 'NONE', *, *, #10656, .F. ) ;
#64268=CARTESIAN_POINT ( 'NONE',  ( -35.00000000000000000, -11.10408318471063716, 6.265926637539457111 ) ) ;
#64270=ORIENTED_EDGE ( 'NONE', *, *, #30754, .T. ) ;
#64271=CARTESIAN_POINT ( 'NONE',  ( -36.00000000000000711, -7.094637218249278732, -10.59380114696477904 ) ) ;
#64273=CIRCLE ( 'NONE', #49444, 5.000000000000000000 ) ;
#64277=CARTESIAN_POINT ( 'NONE',  ( -35.00000000000000000, 1.908798535168378274, 12.60630747491664039 ) ) ;
#64278=CARTESIAN_POINT ( 'NONE',  ( 11.67759032571662736, 13.41004018116123042, -1.561691431055280299 ) ) ;
#64279=EDGE_CURVE ( 'NONE', #40664, #47275, #32151, .T. ) ;
#64282=CARTESIAN_POINT ( 'NONE',  ( 36.00000000000000711, 6.415447294506860132, 11.01837265713066039 ) ) ;
#64283=ORIENTED_EDGE ( 'NONE', *, *, #59253, .F. ) ;
#64285=ORIENTED_EDGE ( 'NONE', *, *, #17675, .T. ) ;
#64288=DIRECTION ( 'NONE',  ( 0.000000000000000000, 0.01356324068817992001, -0.9999080150203990547 ) ) ;
#64289=B_SPLINE_CURVE_WITH_KNOTS ( 'NONE', 3,
 ( #45186, #56150, #55844, #46202, #25570, #45203, #45515, #25915, #30873, #56845, #51842, #31537, #40877, #50537, #15904, #14913 ),
 .UNSPECIFIED., .F., .F.,
 ( 4, 2, 2, 2, 2, 2, 2, 4 ),
 ( 9.697399036122160616E-18, 0.002292800386316098255, 0.003439200579474143912, 0.004585600772632189570, 0.005732000965790236963, 0.006878401158948284355, 0.008024801352106331748, 0.009171201545264380875 ),
 .UNSPECIFIED. ) ;
#64291=FACE_OUTER_BOUND ( 'NONE', #27513, .T. ) ;
#64293=VECTOR ( 'NONE', #7981, 1000.000000000000000 ) ;
#64294=FACE_OUTER_BOUND ( 'NONE', #49067, .T. ) ;
#64296=DIRECTION ( 'NONE',  ( 1.000000000000000000, -0.000000000000000000, 0.000000000000000000 ) ) ;
#64298=DIRECTION ( 'NONE',  ( -1.000000000000000000, -0.000000000000000000, 0.000000000000000000 ) ) ;
#64301=VECTOR ( 'NONE', #21198, 1000.000000000000000 ) ;
#64302=EDGE_CURVE ( 'NONE', #44696, #42318, #17318, .T. ) ;
#64303=CARTESIAN_POINT ( 'NONE',  ( -10.84719144215113218, -4.830053348895781085, 12.61335488639389446 ) ) ;
#64304=CARTESIAN_POINT ( 'NONE',  ( 9.102085259661365058, 3.314740859770817227, -11.53545134040598796 ) ) ;
#64305=EDGE_LOOP ( 'NONE', ( #38352, #34571, #14087, #8573 ) ) ;
#64306=DIRECTION ( 'NONE',  ( 0.000000000000000000, -0.8169148498130338609, 0.5767582926624880146 ) ) ;
#64308=ADVANCED_FACE ( 'NONE', ( #7238 ), #47499, .F. ) ;
#64310=ADVANCED_FACE ( 'NONE', ( #63419 ), #17889, .T. ) ;
#64311=CARTESIAN_POINT ( 'NONE',  ( -35.00000000000000000, 0.000000000000000000, 0.000000000000000000 ) ) ;
#64313=ORIENTED_EDGE ( 'NONE', *, *, #2929, .F. ) ;
#64314=EDGE_CURVE ( 'NONE', #11411, #2844, #18222, .T. ) ;
#64315=CARTESIAN_POINT ( 'NONE',  ( 35.00000000000000000, 9.700295462048766026, 7.376655759824770620 ) ) ;
#64316=CARTESIAN_POINT ( 'NONE',  ( -37.00000000000000711, 0.000000000000000000, 0.000000000000000000 ) ) ;
#64317=ORIENTED_EDGE ( 'NONE', *, *, #14987, .F. ) ;
#64318=CARTESIAN_POINT ( 'NONE',  ( 22.19367488060846227, 12.07937757942956658, -6.038551727115931911 ) ) ;
#64319=DIRECTION ( 'NONE',  ( -1.000000000000000000, 0.000000000000000000, 0.000000000000000000 ) ) ;
#64320=ADVANCED_FACE ( 'NONE', ( #62436 ), #31849, .F. ) ;
#64321=VERTEX_POINT ( 'NONE', #8891 ) ;
#64322=ORIENTED_EDGE ( 'NONE', *, *, #27839, .T. ) ;
#64323=DIRECTION ( 'NONE',  ( 0.000000000000000000, 0.01356324068817998073, -0.9999080150203990547 ) ) ;
#64324=ORIENTED_EDGE ( 'NONE', *, *, #27777, .T. ) ;
#64325=DIRECTION ( 'NONE',  ( 1.000000000000000000, 0.000000000000000000, 0.000000000000000000 ) ) ;
#64326=DIRECTION ( 'NONE',  ( 1.000000000000000000, 0.000000000000000000, -0.000000000000000000 ) ) ;
#64330=DIRECTION ( 'NONE',  ( 0.000000000000000000, 0.2618041379715633776, -0.9651210252299794456 ) ) ;
#64333=DIRECTION ( 'NONE',  ( 0.000000000000000000, 0.01356324068817998940, -0.9999080150203990547 ) ) ;
#64335=ORIENTED_EDGE ( 'NONE', *, *, #26941, .T. ) ;
#64337=ORIENTED_EDGE ( 'NONE', *, *, #62843, .T. ) ;
#64338=VERTEX_POINT ( 'NONE', #9200 ) ;
#64339=DIRECTION ( 'NONE',  ( 0.000000000000000000, -0.01356324068818000848, 0.9999080150203990547 ) ) ;
#64342=DIRECTION ( 'NONE',  ( 0.000000000000000000, -0.9651210252299767811, -0.2618041379715732031 ) ) ;
#64343=CARTESIAN_POINT ( 'NONE',  ( 24.34326217128684888, -1.446676816449340208, 11.91385012721646319 ) ) ;
#64344=CARTESIAN_POINT ( 'NONE',  ( 3.388896915696422152, -10.79019736087639458, -5.264843862020488707 ) ) ;
#64345=EDGE_CURVE ( 'NONE', #14524, #21230, #53506, .T. ) ;
#64346=DIRECTION ( 'NONE',  ( -1.000000000000000000, -0.000000000000000000, 0.000000000000000000 ) ) ;
#64347=EDGE_CURVE ( 'NONE', #36171, #25992, #19501, .T. ) ;
#64348=ORIENTED_EDGE ( 'NONE', *, *, #24185, .T. ) ;
#64351=EDGE_LOOP ( 'NONE', ( #34396, #16602, #37299, #30733 ) ) ;
#64352=DIRECTION ( 'NONE',  ( 0.000000000000000000, 0.9346839223284527653, -0.3554799084909002205 ) ) ;
#64355=ORIENTED_EDGE ( 'NONE', *, *, #3130, .F. ) ;
#64358=CARTESIAN_POINT ( 'NONE',  ( 12.10998784662220729, -10.46621227226782835, -8.526922110106905706 ) ) ;
#64362=CARTESIAN_POINT ( 'NONE',  ( -35.00000000000000000, -1.456211999474261054, -11.65554240571058742 ) ) ;
#64363=ORIENTED_EDGE ( 'NONE', *, *, #11090, .T. ) ;
#64367=CARTESIAN_POINT ( 'NONE',  ( -10.95212338237647920, -9.902220863987562183, 6.778349501228839280 ) ) ;
#64369=DIRECTION ( 'NONE',  ( 0.000000000000000000, -0.01356324068818685717, 0.9999080150203989437 ) ) ;
#64370=DIRECTION ( 'NONE',  ( -1.000000000000000000, 0.000000000000000000, 0.000000000000000000 ) ) ;
#64371=CYLINDRICAL_SURFACE ( 'NONE', #7594, 12.75000000000000178 ) ;
#64372=CARTESIAN_POINT ( 'NONE',  ( -35.00000000000000000, -9.040300684349640292, -7.499679039484155041 ) ) ;
#64374=DIRECTION ( 'NONE',  ( 1.000000000000000000, 0.000000000000000000, 0.000000000000000000 ) ) ;
#64375=EDGE_LOOP ( 'NONE', ( #12064, #44661, #55832, #26539 ) ) ;
#64378=EDGE_CURVE ( 'NONE', #47095, #50460, #8236, .T. ) ;
#64380=AXIS2_PLACEMENT_3D ( 'NONE', #32095, #6858, #2534 ) ;
#64383=CIRCLE ( 'NONE', #7058, 12.74999999999999822 ) ;
#64386=CARTESIAN_POINT ( 'NONE',  ( 28.55105714595230637, 12.36547357143752990, 5.429635869807071025 ) ) ;
#64388=ORIENTED_EDGE ( 'NONE', *, *, #39194, .T. ) ;
#64390=DIRECTION ( 'NONE',  ( 1.000000000000000000, 0.000000000000000000, 0.000000000000000000 ) ) ;
#64392=EDGE_CURVE ( 'NONE', #47265, #30454, #57720, .T. ) ;
#64394=DIRECTION ( 'NONE',  ( 0.000000000000000000, 0.01356324068818000328, -0.9999080150203990547 ) ) ;
#64395=CARTESIAN_POINT ( 'NONE',  ( 36.00000000000000711, 12.60630747491662973, -1.908798535168425792 ) ) ;
#64396=ORIENTED_EDGE ( 'NONE', *, *, #34136, .T. ) ;
#64397=DIRECTION ( 'NONE',  ( 0.000000000000000000, 0.9970832820307036215, 0.07632122047556835764 ) ) ;
#64402=CARTESIAN_POINT ( 'NONE',  ( 35.00000000000000000, 4.986700593229853595, 10.63508530065516311 ) ) ;
#64403=DIRECTION ( 'NONE',  ( 0.000000000000000000, -0.01356324068817998940, 0.9999080150203990547 ) ) ;
#64405=ORIENTED_EDGE ( 'NONE', *, *, #18431, .F. ) ;
#64406=EDGE_LOOP ( 'NONE', ( #3644, #10170, #14587, #5998 ) ) ;
#64408=ORIENTED_EDGE ( 'NONE', *, *, #24959, .F. ) ;
#64409=B_SPLINE_CURVE_WITH_KNOTS ( 'NONE', 3,
 ( #28225, #22586, #26916, #42850, #1330, #62160, #58160, #32856 ),
 .UNSPECIFIED., .F., .F.,
 ( 4, 2, 2, 4 ),
 ( 0.004099133380581623104, 0.006211397827347840857, 0.007267530050730946697, 0.008323662274114053405 ),
 .UNSPECIFIED. ) ;
#64413=DIRECTION ( 'NONE',  ( 0.000000000000000000, -0.8009703041134234036, -0.5987040770935587730 ) ) ;
#64416=ORIENTED_EDGE ( 'NONE', *, *, #38751, .T. ) ;
#64419=FACE_OUTER_BOUND ( 'NONE', #29601, .T. ) ;
#64422=EDGE_CURVE ( 'NONE', #56824, #17810, #26908, .T. ) ;
#64423=CARTESIAN_POINT ( 'NONE',  ( -37.00000000000000711, 6.547236723514155976, -9.752226076388824438 ) ) ;
#64424=CARTESIAN_POINT ( 'NONE',  ( 35.00000000000000000, 4.705694406421931860E-17, -3.469127814946512892E-15 ) ) ;
#64425=ORIENTED_EDGE ( 'NONE', *, *, #61758, .F. ) ;
#64426=AXIS2_PLACEMENT_3D ( 'NONE', #53741, #8174, #28447 ) ;
#64428=FACE_OUTER_BOUND ( 'NONE', #51203, .T. ) ;
#64431=CARTESIAN_POINT ( 'NONE',  ( -7.389643752995847414, 8.206056478905821905, -10.72177447465196209 ) ) ;
#64432=DIRECTION ( 'NONE',  ( -1.000000000000000000, 0.000000000000000000, -0.000000000000000000 ) ) ;
#64433=AXIS2_PLACEMENT_3D ( 'NONE', #34323, #24339, #45601 ) ;
#64434=DIRECTION ( 'NONE',  ( -1.000000000000000000, 0.000000000000000000, 0.000000000000000000 ) ) ;
#64435=ORIENTED_EDGE ( 'NONE', *, *, #34750, .F. ) ;
#64436=DIRECTION ( 'NONE',  ( -1.000000000000000000, 0.000000000000000000, 0.000000000000000000 ) ) ;
#64438=CARTESIAN_POINT ( 'NONE',  ( -35.00000000000000000, 6.415447294506704701, 11.01837265713075453 ) ) ;
#64442=CARTESIAN_POINT ( 'NONE',  ( 37.00000000000000711, 3.033604067594577902, -12.38385022362083454 ) ) ;
#64443=DIRECTION ( 'NONE',  ( -0.000000000000000000, -0.000000000000000000, -1.000000000000000000 ) ) ;
#64444=DIRECTION ( 'NONE',  ( 0.000000000000000000, 0.01356324068817992175, -0.9999080150203990547 ) ) ;
#64447=VERTEX_POINT ( 'NONE', #22421 ) ;
#64452=DIRECTION ( 'NONE',  ( 1.000000000000000000, 0.000000000000000000, 0.000000000000000000 ) ) ;
#64453=CYLINDRICAL_SURFACE ( 'NONE', #42541, 12.18649999999999878 ) ;
#64454=CYLINDRICAL_SURFACE ( 'NONE', #63238, 12.18649999999999878 ) ;
#64457=ORIENTED_EDGE ( 'NONE', *, *, #36780, .T. ) ;
#64458=DIRECTION ( 'NONE',  ( 0.000000000000000000, -1.000000000000000000, 0.000000000000000000 ) ) ;
#64459=CARTESIAN_POINT ( 'NONE',  ( 145.1370849898475797, 3.309064568108273190E-14, 0.000000000000000000 ) ) ;
#64460=EDGE_CURVE ( 'NONE', #26477, #6288, #48039, .T. ) ;
#64465=ORIENTED_EDGE ( 'NONE', *, *, #47388, .T. ) ;
#64466=LINE ( 'NONE', #24905, #5244 ) ;
#64467=EDGE_LOOP ( 'NONE', ( #41610, #59718, #22757, #20521 ) ) ;
#64470=EDGE_CURVE ( 'NONE', #21573, #35230, #8862, .T. ) ;
#64472=CIRCLE ( 'NONE', #61298, 12.18650000000000055 ) ;
#64473=LINE ( 'NONE', #9264, #16142 ) ;
#64474=ADVANCED_FACE ( 'NONE', ( #2501 ), #6825, .T. ) ;
#64475=CARTESIAN_POINT ( 'NONE',  ( 6.776630524595501193, -5.710973591730284404, 12.23820960985696793 ) ) ;
#64477=VECTOR ( 'NONE', #24115, 1000.000000000000000 ) ;
#64478=ORIENTED_EDGE ( 'NONE', *, *, #62262, .T. ) ;
#64481=CARTESIAN_POINT ( 'NONE',  ( 37.00000000000000711, 4.705694406421931860E-17, -3.469127814946512892E-15 ) ) ;
#64483=DIRECTION ( 'NONE',  ( 0.000000000000000000, 0.01356324068817998940, -0.9999080150203989437 ) ) ;
#64484=CARTESIAN_POINT ( 'NONE',  ( -35.00000000000000000, 2.627174906296914525, 11.44858830469741129 ) ) ;
#64485=VERTEX_POINT ( 'NONE', #12117 ) ;
#64486=ORIENTED_EDGE ( 'NONE', *, *, #36752, .F. ) ;
#64489=ADVANCED_FACE ( 'NONE', ( #63308 ), #37726, .T. ) ;
#64492=CYLINDRICAL_SURFACE ( 'NONE', #39003, 5.000000000000000888 ) ;
#64494=CYLINDRICAL_SURFACE ( 'NONE', #6678, 6.595312090839647645 ) ;
#64496=DIRECTION ( 'NONE',  ( 1.000000000000000000, 0.000000000000000000, 0.000000000000000000 ) ) ;
#64498=DIRECTION ( 'NONE',  ( -0.000000000000000000, -0.000000000000000000, -1.000000000000000000 ) ) ;
#64499=VERTEX_POINT ( 'NONE', #13427 ) ;
#64500=ORIENTED_EDGE ( 'NONE', *, *, #37462, .T. ) ;
#64501=CARTESIAN_POINT ( 'NONE',  ( -35.00000000000000000, 2.497432891017006718, -11.47758908105691766 ) ) ;
#64502=ORIENTED_EDGE ( 'NONE', *, *, #53787, .F. ) ;
#64504=ORIENTED_EDGE ( 'NONE', *, *, #7957, .T. ) ;
#64509=AXIS2_PLACEMENT_3D ( 'NONE', #40630, #30334, #39652 ) ;
#64512=CARTESIAN_POINT ( 'NONE',  ( -37.00000000000000711, -11.02904044024211849, 4.041347439435823752 ) ) ;
#64513=ORIENTED_EDGE ( 'NONE', *, *, #16761, .T. ) ;
#64516=EDGE_LOOP ( 'NONE', ( #42951, #55902, #56242, #20221 ) ) ;
#64517=DIRECTION ( 'NONE',  ( -1.000000000000000000, 0.000000000000000000, -0.000000000000000000 ) ) ;
#64518=CARTESIAN_POINT ( 'NONE',  ( -17.64417118620952252, -7.220089482685009052, -11.41077800675886245 ) ) ;
#64521=CARTESIAN_POINT ( 'NONE',  ( 37.00000000000000711, -6.564808257521689505, 10.93004082984025160 ) ) ;
#64524=ORIENTED_EDGE ( 'NONE', *, *, #48493, .F. ) ;
#64526=CIRCLE ( 'NONE', #12360, 4.999999999999999112 ) ;
#64528=ADVANCED_FACE ( 'NONE', ( #3151 ), #17112, .T. ) ;
#64529=ORIENTED_EDGE ( 'NONE', *, *, #17636, .T. ) ;
#64531=DIRECTION ( 'NONE',  ( -1.000000000000000000, -0.000000000000000000, 0.000000000000000000 ) ) ;
#64532=CARTESIAN_POINT ( 'NONE',  ( -30.18541646480308671, -0.9647385960114739367, 13.47312881255922257 ) ) ;
#64534=DIRECTION ( 'NONE',  ( 0.000000000000000000, 0.9970832820307041766, 0.07632122047556143263 ) ) ;
#64537=CARTESIAN_POINT ( 'NONE',  ( -30.18541646480390384, -1.416020129149325513, 13.42553116244798517 ) ) ;
#64538=EDGE_CURVE ( 'NONE', #786, #4699, #34350, .T. ) ;
#64544=AXIS2_PLACEMENT_3D ( 'NONE', #21250, #30894, #25933 ) ;
#64546=ORIENTED_EDGE ( 'NONE', *, *, #4648, .T. ) ;
#64547=CARTESIAN_POINT ( 'NONE',  ( -35.00000000000000000, 12.00000000000000000, 1.469576158976823947E-15 ) ) ;
#64550=CARTESIAN_POINT ( 'NONE',  ( 22.36482863261543486, 25.00000000000000000, -0.9234811557364158707 ) ) ;
#64554=CARTESIAN_POINT ( 'NONE',  ( 37.00000000000000711, 0.000000000000000000, 0.000000000000000000 ) ) ;
#64557=AXIS2_PLACEMENT_3D ( 'NONE', #16023, #43183, #63456 ) ;
#64558=EDGE_LOOP ( 'NONE', ( #30061, #18276, #59676, #31212 ) ) ;
#64560=EDGE_CURVE ( 'NONE', #52347, #51211, #32704, .T. ) ;
#64563=DIRECTION ( 'NONE',  ( -1.000000000000000000, 0.000000000000000000, 0.000000000000000000 ) ) ;
#64565=CARTESIAN_POINT ( 'NONE',  ( 21.90174657591892071, 11.97747433400151884, -0.7349207973210698519 ) ) ;
#64568=DIRECTION ( 'NONE',  ( 0.000000000000000000, 0.01356324068817998940, -0.9999080150203990547 ) ) ;
#64569=CARTESIAN_POINT ( 'NONE',  ( 37.00000000000000711, -6.891188680298889757, -9.512294188640879611 ) ) ;
#64571=ORIENTED_EDGE ( 'NONE', *, *, #57858, .F. ) ;
#64574=DIRECTION ( 'NONE',  ( -0.000000000000000000, -0.000000000000000000, -1.000000000000000000 ) ) ;
#64575=VERTEX_POINT ( 'NONE', #27407 ) ;
#64576=LINE ( 'NONE', #64271, #707 ) ;
#64580=EDGE_CURVE ( 'NONE', #31862, #21361, #29048, .T. ) ;
#64584=CARTESIAN_POINT ( 'NONE',  ( 10.54028985821272180, 13.47274386308714256, -0.8611671757873611277 ) ) ;
#64586=B_SPLINE_CURVE_WITH_KNOTS ( 'NONE', 3,
 ( #59000, #18754, #27392, #37712, #58007, #2819, #58675, #47689 ),
 .UNSPECIFIED., .F., .F.,
 ( 4, 2, 2, 4 ),
 ( 4.336808689942017736E-19, 0.002017501633567611672, 0.003026252450351417291, 0.004035003267135222477 ),
 .UNSPECIFIED. ) ;
#64587=VERTEX_POINT ( 'NONE', #7448 ) ;
#64589=ORIENTED_EDGE ( 'NONE', *, *, #16344, .F. ) ;
#64591=CARTESIAN_POINT ( 'NONE',  ( 47.00000000000000711, 4.705694406421931860E-17, -3.469127814946512892E-15 ) ) ;
#64592=DIRECTION ( 'NONE',  ( 1.000000000000000000, -0.000000000000000000, 0.000000000000000000 ) ) ;
#64593=DIRECTION ( 'NONE',  ( 0.000000000000000000, -0.9718671068226435450, 0.2355298848897615926 ) ) ;
#64595=CARTESIAN_POINT ( 'NONE',  ( 35.00000000000000000, 0.7008968033240532414, 12.16632754454235332 ) ) ;
#64596=AXIS2_PLACEMENT_3D ( 'NONE', #6647, #1663, #21611 ) ;
#64599=CARTESIAN_POINT ( 'NONE',  ( -35.00000000000000000, 0.000000000000000000, 0.000000000000000000 ) ) ;
#64601=AXIS2_PLACEMENT_3D ( 'NONE', #11119, #62292, #1798 ) ;
#64602=EDGE_CURVE ( 'NONE', #47144, #18362, #64059, .T. ) ;
#64603=VERTEX_POINT ( 'NONE', #8131 ) ;
#64604=FACE_OUTER_BOUND ( 'NONE', #54847, .T. ) ;
#64606=AXIS2_PLACEMENT_3D ( 'NONE', #55548, #55206, #30271 ) ;
#64608=CARTESIAN_POINT ( 'NONE',  ( -17.37148431026360740, -6.070708735758810093, 12.06204800037487246 ) ) ;
#64610=CIRCLE ( 'NONE', #35929, 12.18649999999999878 ) ;
#64611=EDGE_CURVE ( 'NONE', #49200, #2142, #23743, .T. ) ;
#64612=CARTESIAN_POINT ( 'NONE',  ( -9.378203292903490862, -2.735599985537505940, 13.22402823059322863 ) ) ;
#64614=CARTESIAN_POINT ( 'NONE',  ( -5.388074842124701114, -1.427462443323999741, 13.42432431655054970 ) ) ;
#64616=CYLINDRICAL_SURFACE ( 'NONE', #18151, 12.74999999999999822 ) ;
#64617=CARTESIAN_POINT ( 'NONE',  ( -37.00000000000000711, 0.000000000000000000, 0.000000000000000000 ) ) ;
#64618=DIRECTION ( 'NONE',  ( 0.000000000000000000, 0.07632122047556488820, -0.9970832820307038435 ) ) ;
#64620=EDGE_CURVE ( 'NONE', #30956, #22366, #45918, .T. ) ;
#64621=DIRECTION ( 'NONE',  ( 1.000000000000000000, 0.000000000000000000, 0.000000000000000000 ) ) ;
#64622=CARTESIAN_POINT ( 'NONE',  ( -37.00000000000000711, 11.78745411414839950, 3.093009498343969099 ) ) ;
#64623=ORIENTED_EDGE ( 'NONE', *, *, #23404, .F. ) ;
#64624=CARTESIAN_POINT ( 'NONE',  ( -37.00000000000000711, 0.000000000000000000, 0.000000000000000000 ) ) ;
#64625=CARTESIAN_POINT ( 'NONE',  ( -9.351388602708162523, -11.42638970207761950, -3.665735721005252135 ) ) ;
#64627=ORIENTED_EDGE ( 'NONE', *, *, #16389, .T. ) ;
#64628=CARTESIAN_POINT ( 'NONE',  ( 21.44698719852729596, 13.04659800062481523, -3.493617502577392120 ) ) ;
#64629=CYLINDRICAL_SURFACE ( 'NONE', #6551, 12.18650000000000055 ) ;
#64630=ORIENTED_EDGE ( 'NONE', *, *, #46024, .F. ) ;
#64633=DIRECTION ( 'NONE',  ( 1.000000000000000000, 0.000000000000000000, -0.000000000000000000 ) ) ;
#64634=AXIS2_PLACEMENT_3D ( 'NONE', #33768, #38442, #58758 ) ;
#64636=CARTESIAN_POINT ( 'NONE',  ( 18.98898312442695158, 6.102278294184976914, 12.04338967756598144 ) ) ;
#64637=CARTESIAN_POINT ( 'NONE',  ( -27.19357181888462094, 10.84410562793473431, 5.138615876886901468 ) ) ;
#64638=AXIS2_PLACEMENT_3D ( 'NONE', #62743, #52139, #62410 ) ;
#64639=CARTESIAN_POINT ( 'NONE',  ( -35.00000000000000000, -2.865935305911712749, 12.42372387097881514 ) ) ;
#64640=CARTESIAN_POINT ( 'NONE',  ( 35.00000000000000000, 4.705694406421931860E-17, -3.469127814946512892E-15 ) ) ;
#64643=FACE_OUTER_BOUND ( 'NONE', #48614, .T. ) ;
#64644=VERTEX_POINT ( 'NONE', #4724 ) ;
#64645=CIRCLE ( 'NONE', #35979, 5.000000000000000000 ) ;
#64648=EDGE_LOOP ( 'NONE', ( #38445, #61268, #14161, #32982 ) ) ;
#64650=ORIENTED_EDGE ( 'NONE', *, *, #34019, .F. ) ;
#64652=ORIENTED_EDGE ( 'NONE', *, *, #22036, .F. ) ;
#64657=CARTESIAN_POINT ( 'NONE',  ( 24.22861315122816706, -1.970758474066428345, 11.83836876581584185 ) ) ;
#64658=CARTESIAN_POINT ( 'NONE',  ( 37.00000000000000711, 8.389074212634284322, -8.839356091080075473 ) ) ;
#64659=CARTESIAN_POINT ( 'NONE',  ( 36.00000000000000711, -6.018036132182079889, 11.24036214326526562 ) ) ;
#64661=EDGE_LOOP ( 'NONE', ( #2828, #64042, #28739, #51644 ) ) ;
#64663=ORIENTED_EDGE ( 'NONE', *, *, #4952, .F. ) ;
#64666=LINE ( 'NONE', #8842, #45897 ) ;
#64667=CARTESIAN_POINT ( 'NONE',  ( -36.00000000000000711, 12.63095688309031495, -1.738225594539863472 ) ) ;
#64669=AXIS2_PLACEMENT_3D ( 'NONE', #50258, #54901, #45253 ) ;
#64672=ORIENTED_EDGE ( 'NONE', *, *, #35006, .F. ) ;
#64673=CIRCLE ( 'NONE', #40281, 12.18650000000000055 ) ;
#64674=EDGE_CURVE ( 'NONE', #63181, #52362, #42841, .T. ) ;
#64676=EDGE_CURVE ( 'NONE', #50460, #58025, #39670, .T. ) ;
#64679=CARTESIAN_POINT ( 'NONE',  ( -36.00000000000000711, -3.033604067594665832, 12.38385022362080967 ) ) ;
#64680=AXIS2_PLACEMENT_3D ( 'NONE', #41161, #40858, #61781 ) ;
#64681=DIRECTION ( 'NONE',  ( 1.000000000000000000, 0.000000000000000000, -0.000000000000000000 ) ) ;
#64682=DIRECTION ( 'NONE',  ( 0.000000000000000000, 0.01356324068817998940, -0.9999080150203990547 ) ) ;
#64683=EDGE_CURVE ( 'NONE', #853, #13869, #5030, .T. ) ;
#64684=AXIS2_PLACEMENT_3D ( 'NONE', #24569, #23608, #54526 ) ;
#64685=CARTESIAN_POINT ( 'NONE',  ( -6.614609636016250072, -1.684350297699918286, -11.88140433430720933 ) ) ;
#64686=EDGE_CURVE ( 'NONE', #21596, #2181, #55571, .T. ) ;
#64687=DIRECTION ( 'NONE',  ( 1.000000000000000000, 0.000000000000000000, 0.000000000000000000 ) ) ;
#64688=CARTESIAN_POINT ( 'NONE',  ( 37.00000000000000711, 11.26103545359850955, -3.340853584269734000 ) ) ;
#64690=VERTEX_POINT ( 'NONE', #20652 ) ;
#64691=CARTESIAN_POINT ( 'NONE',  ( -37.00000000000000711, -1.039216533672986387, 11.70009620280411333 ) ) ;
#64694=CARTESIAN_POINT ( 'NONE',  ( 22.36482863261543486, 13.46837713145128923, -0.9234811557364158707 ) ) ;
#64695=CIRCLE ( 'NONE', #44527, 12.18650000000000055 ) ;
#64696=EDGE_CURVE ( 'NONE', #53805, #54601, #51249, .T. ) ;
#64697=VECTOR ( 'NONE', #36227, 1000.000000000000000 ) ;
#64699=CARTESIAN_POINT ( 'NONE',  ( -35.00000000000000000, -10.70999494708497046, 5.814360711498253842 ) ) ;
#64700=CARTESIAN_POINT ( 'NONE',  ( 3.455078800971972619, 8.284346402942340148, 10.65933643386987484 ) ) ;
#64701=ORIENTED_EDGE ( 'NONE', *, *, #49069, .F. ) ;
#64702=DIRECTION ( 'NONE',  ( -0.000000000000000000, -1.000000000000000000, -0.000000000000000000 ) ) ;
#64703=DIRECTION ( 'NONE',  ( 0.000000000000000000, 0.8515178078024850938, -0.5243256840888592674 ) ) ;
#64705=EDGE_CURVE ( 'NONE', #60283, #32649, #35262, .T. ) ;
#64707=CARTESIAN_POINT ( 'NONE',  ( 37.00000000000000711, 11.74226168163341377, 0.3025107581129941048 ) ) ;
#64708=DIRECTION ( 'NONE',  ( 0.000000000000000000, -0.4134677391718576955, -0.9105187689795926076 ) ) ;
#64709=CARTESIAN_POINT ( 'NONE',  ( 18.66452694970452697, -6.623337850070971200, 11.78786257686909700 ) ) ;
#64712=AXIS2_PLACEMENT_3D ( 'NONE', #36503, #46168, #31507 ) ;
#64717=CARTESIAN_POINT ( 'NONE',  ( -15.21472318775516008, 8.472363384278436271, -10.51049469413687198 ) ) ;
#64720=AXIS2_PLACEMENT_3D ( 'NONE', #16544, #46461, #26187 ) ;
#64722=DIRECTION ( 'NONE',  ( 0.000000000000000000, -0.5767582926624851281, -0.8169148498130359703 ) ) ;
#64725=ORIENTED_EDGE ( 'NONE', *, *, #32374, .F. ) ;
#64726=CARTESIAN_POINT ( 'NONE',  ( -19.55532226645861726, -4.268374217007646187, -11.21543595443842456 ) ) ;
#64727=VERTEX_POINT ( 'NONE', #10642 ) ;
#64728=CIRCLE ( 'NONE', #19140, 12.75000000000000178 ) ;
#64729=CARTESIAN_POINT ( 'NONE',  ( 35.00000000000000000, 9.913596905230225076, 8.017674001891672120 ) ) ;
#64730=ADVANCED_FACE ( 'NONE', ( #25971 ), #15324, .T. ) ;
#64731=EDGE_CURVE ( 'NONE', #18732, #60108, #59907, .T. ) ;
#64734=DIRECTION ( 'NONE',  ( 1.000000000000000000, -0.000000000000000000, 0.000000000000000000 ) ) ;
#64735=CARTESIAN_POINT ( 'NONE',  ( -37.00000000000000711, -6.547236723514086698, 9.752226076388870624 ) ) ;
#64737=VERTEX_POINT ( 'NONE', #44029 ) ;
#64740=DIRECTION ( 'NONE',  ( 0.000000000000000000, -0.01356324068817992522, 0.9999080150203990547 ) ) ;
#64741=EDGE_CURVE ( 'NONE', #52228, #27224, #65207, .T. ) ;
#64745=ORIENTED_EDGE ( 'NONE', *, *, #16681, .T. ) ;
#64749=DIRECTION ( 'NONE',  ( 0.000000000000000000, 0.9937233664769765662, -0.1118654143051581590 ) ) ;
#64752=VERTEX_POINT ( 'NONE', #62493 ) ;
#64754=CARTESIAN_POINT ( 'NONE',  ( -14.29135464769095520, 7.782112657557433089, 9.134479874907178498 ) ) ;
#64758=CARTESIAN_POINT ( 'NONE',  ( 9.575800908719084958, 13.45729701195361372, -1.072919909436246266 ) ) ;
#64761=DIRECTION ( 'NONE',  ( -1.000000000000000000, 0.000000000000000000, 0.000000000000000000 ) ) ;
#64762=DIRECTION ( 'NONE',  ( 0.000000000000000000, -0.4698238015817425839, -0.8827602140260283337 ) ) ;
#64763=AXIS2_PLACEMENT_3D ( 'NONE', #37581, #43205, #17302 ) ;
#64764=AXIS2_PLACEMENT_3D ( 'NONE', #54078, #29444, #8510 ) ;
#64768=DIRECTION ( 'NONE',  ( -1.000000000000000000, 0.000000000000000000, 0.000000000000000000 ) ) ;
#64769=DIRECTION ( 'NONE',  ( -1.000000000000000000, 0.000000000000000000, 0.000000000000000000 ) ) ;
#64770=DIRECTION ( 'NONE',  ( 0.000000000000000000, -0.9903235168508535136, -0.1387779952735919697 ) ) ;
#64771=CARTESIAN_POINT ( 'NONE',  ( -10.90165637462999726, -7.918284569530332107, 10.94501414979677456 ) ) ;
#64772=DIRECTION ( 'NONE',  ( 0.000000000000000000, 0.04924826701374598187, 0.9987865678893278476 ) ) ;
#64773=ORIENTED_EDGE ( 'NONE', *, *, #30170, .T. ) ;
#64776=CARTESIAN_POINT ( 'NONE',  ( -35.00000000000000000, 0.000000000000000000, 0.000000000000000000 ) ) ;
#64777=DIRECTION ( 'NONE',  ( 0.000000000000000000, -0.01356324068818000328, 0.9999080150203990547 ) ) ;
#64779=AXIS2_PLACEMENT_3D ( 'NONE', #17240, #63112, #37844 ) ;
#64780=EDGE_CURVE ( 'NONE', #25468, #50714, #11318, .T. ) ;
#64783=ORIENTED_EDGE ( 'NONE', *, *, #26416, .T. ) ;
#64784=CARTESIAN_POINT ( 'NONE',  ( -18.22913673819321190, 11.73512385886278686, 2.593994127463341126 ) ) ;
#64785=ADVANCED_FACE ( 'NONE', ( #1020 ), #16638, .T. ) ;
#64789=AXIS2_PLACEMENT_3D ( 'NONE', #65396, #29823, #50135 ) ;
#64792=ORIENTED_EDGE ( 'NONE', *, *, #14322, .F. ) ;
#64793=VERTEX_POINT ( 'NONE', #47879 ) ;
#64794=CARTESIAN_POINT ( 'NONE',  ( 35.00000000000000000, 11.50504120060948487, 4.018060380616274685 ) ) ;
#64795=CIRCLE ( 'NONE', #79, 12.74999999999999822 ) ;
#64797=CARTESIAN_POINT ( 'NONE',  ( 35.00000000000000000, -3.213188559034160452, 11.29812557209479706 ) ) ;
#64798=CARTESIAN_POINT ( 'NONE',  ( 37.00000000000000711, -2.220215194441986561, -11.98254675519227597 ) ) ;
#64799=CARTESIAN_POINT ( 'NONE',  ( -35.00000000000000000, -11.71932350927023414, 3.511386971104904386 ) ) ;
#64801=CARTESIAN_POINT ( 'NONE',  ( -18.47110435980187049, -11.89396356225322648, 1.625996358069915049 ) ) ;
#64802=VERTEX_POINT ( 'NONE', #41900 ) ;
#64804=ORIENTED_EDGE ( 'NONE', *, *, #41872, .F. ) ;
#64809=AXIS2_PLACEMENT_3D ( 'NONE', #36410, #20792, #56359 ) ;
#64811=ORIENTED_EDGE ( 'NONE', *, *, #8335, .T. ) ;
#64812=CARTESIAN_POINT ( 'NONE',  ( 37.00000000000000711, 4.705694406421931860E-17, -3.469127814946512892E-15 ) ) ;
#64813=CARTESIAN_POINT ( 'NONE',  ( 35.00000000000000000, -2.865935305911542663, 12.42372387097884534 ) ) ;
#64814=EDGE_CURVE ( 'NONE', #50945, #54151, #36908, .T. ) ;
#64815=VERTEX_POINT ( 'NONE', #63168 ) ;
#64817=LINE ( 'NONE', #9969, #6397 ) ;
#64818=CARTESIAN_POINT ( 'NONE',  ( 7.195872910760210850, -7.348025474021660841, 9.498045278114711110 ) ) ;
#64820=VERTEX_POINT ( 'NONE', #57209 ) ;
#64822=ORIENTED_EDGE ( 'NONE', *, *, #27736, .T. ) ;
#64824=ORIENTED_EDGE ( 'NONE', *, *, #17102, .F. ) ;
#64825=EDGE_CURVE ( 'NONE', #62364, #40488, #11636, .T. ) ;
#64827=ORIENTED_EDGE ( 'NONE', *, *, #29721, .T. ) ;
#64832=DIRECTION ( 'NONE',  ( 0.000000000000000000, -0.07632122047557186872, 0.9970832820307033995 ) ) ;
#64834=AXIS2_PLACEMENT_3D ( 'NONE', #63704, #18183, #38451 ) ;
#64836=CIRCLE ( 'NONE', #4352, 12.75000000000000178 ) ;
#64839=DIRECTION ( 'NONE',  ( 1.000000000000000000, 0.000000000000000000, 0.000000000000000000 ) ) ;
#64840=CARTESIAN_POINT ( 'NONE',  ( -18.12306279865811476, -9.252926135531010843, -9.833831937096134013 ) ) ;
#64842=EDGE_CURVE ( 'NONE', #34385, #6738, #10009, .T. ) ;
#64843=ORIENTED_EDGE ( 'NONE', *, *, #38899, .F. ) ;
#64845=CARTESIAN_POINT ( 'NONE',  ( -35.00000000000000000, 5.273331777780488672, -10.49591321039675229 ) ) ;
#64849=EDGE_LOOP ( 'NONE', ( #11751, #20772, #5879, #18617 ) ) ;
#64851=ORIENTED_EDGE ( 'NONE', *, *, #3897, .T. ) ;
#64852=CARTESIAN_POINT ( 'NONE',  ( 37.00000000000000711, 12.74068829017553917, 0.4871980014161897410 ) ) ;
#64853=DIRECTION ( 'NONE',  ( 0.000000000000000000, 0.01356324068817998940, -0.9999080150203990547 ) ) ;
#64855=CARTESIAN_POINT ( 'NONE',  ( 37.00000000000000711, -4.824807283154208370, -11.80185301892979410 ) ) ;
#64858=VERTEX_POINT ( 'NONE', #22616 ) ;
#64860=DIRECTION ( 'NONE',  ( 0.000000000000000000, -0.01356324068817992175, 0.9999080150203990547 ) ) ;
#64861=EDGE_CURVE ( 'NONE', #27211, #31372, #42879, .T. ) ;
#64863=CIRCLE ( 'NONE', #21300, 12.18650000000000055 ) ;
#64864=AXIS2_PLACEMENT_3D ( 'NONE', #5291, #25561, #4654 ) ;
#64865=EDGE_CURVE ( 'NONE', #30718, #31243, #37584, .T. ) ;
#64870=CARTESIAN_POINT ( 'NONE',  ( 22.88594695219327235, 3.421158645304719137, 13.05931366970166962 ) ) ;
#64877=VECTOR ( 'NONE', #62182, 1000.000000000000000 ) ;
#64879=ORIENTED_EDGE ( 'NONE', *, *, #44910, .F. ) ;
#64881=DIRECTION ( 'NONE',  ( 1.000000000000000000, 0.000000000000000000, 0.000000000000000000 ) ) ;
#64882=DIRECTION ( 'NONE',  ( 0.000000000000000000, 0.01356324068817998940, -0.9999080150203989437 ) ) ;
#64885=ORIENTED_EDGE ( 'NONE', *, *, #14260, .T. ) ;
#64886=CIRCLE ( 'NONE', #37274, 5.000000000000000000 ) ;
#64888=ORIENTED_EDGE ( 'NONE', *, *, #15919, .F. ) ;
#64890=DIRECTION ( 'NONE',  ( 0.000000000000000000, -0.01356324068817991828, 0.9999080150203990547 ) ) ;
#64891=VERTEX_POINT ( 'NONE', #34139 ) ;
#64892=DIRECTION ( 'NONE',  ( 1.000000000000000000, 0.000000000000000000, 0.000000000000000000 ) ) ;
#64893=DIRECTION ( 'NONE',  ( 1.000000000000000000, 0.000000000000000000, 0.000000000000000000 ) ) ;
#64894=CARTESIAN_POINT ( 'NONE',  ( -36.00000000000000711, -2.250029553613845934, 12.54989509947650284 ) ) ;
#64895=AXIS2_PLACEMENT_3D ( 'NONE', #32768, #1239, #37453 ) ;
#64897=ADVANCED_FACE ( 'NONE', ( #18568 ), #28837, .T. ) ;
#64898=ORIENTED_EDGE ( 'NONE', *, *, #10217, .F. ) ;
#64899=DIRECTION ( 'NONE',  ( 0.000000000000000000, 0.4698238015817303159, 0.8827602140260348840 ) ) ;
#64902=DIRECTION ( 'NONE',  ( -1.000000000000000000, 0.000000000000000000, -0.000000000000000000 ) ) ;
#64903=VERTEX_POINT ( 'NONE', #65054 ) ;
#64905=VERTEX_POINT ( 'NONE', #19530 ) ;
#64906=DIRECTION ( 'NONE',  ( 0.000000000000000000, 0.01356324068817992175, -0.9999080150203990547 ) ) ;
#64907=ORIENTED_EDGE ( 'NONE', *, *, #32633, .T. ) ;
#64908=CARTESIAN_POINT ( 'NONE',  ( -36.00000000000000711, 12.70128625845194392, -1.113475361586356627 ) ) ;
#64909=CARTESIAN_POINT ( 'NONE',  ( 13.37010864853758285, -11.07599950531897370, -4.623143634268777724 ) ) ;
#64910=CARTESIAN_POINT ( 'NONE',  ( 37.00000000000000711, 4.705694406421931860E-17, -3.469127814946512892E-15 ) ) ;
#64911=CARTESIAN_POINT ( 'NONE',  ( 35.00000000000000000, 4.705694406421931860E-17, -3.469127814946512892E-15 ) ) ;
#64912=AXIS2_PLACEMENT_3D ( 'NONE', #52798, #43131, #7229 ) ;
#64913=CIRCLE ( 'NONE', #31976, 5.000000000000000888 ) ;
#64921=VERTEX_POINT ( 'NONE', #60082 ) ;
#64923=EDGE_LOOP ( 'NONE', ( #36112, #27802, #44373, #49741 ) ) ;
#64924=ADVANCED_FACE ( 'NONE', ( #9512 ), #8886, .T. ) ;
#64926=LINE ( 'NONE', #20048, #1832 ) ;
#64928=CYLINDRICAL_SURFACE ( 'NONE', #11938, 12.18650000000000055 ) ;
#64930=CIRCLE ( 'NONE', #55395, 5.000000000000000888 ) ;
#64932=AXIS2_PLACEMENT_3D ( 'NONE', #41908, #6348, #41574 ) ;
#64934=CYLINDRICAL_SURFACE ( 'NONE', #49207, 12.18650000000000055 ) ;
#64935=CIRCLE ( 'NONE', #33083, 4.999999999999998224 ) ;
#64936=ORIENTED_EDGE ( 'NONE', *, *, #56867, .F. ) ;
#64938=AXIS2_PLACEMENT_3D ( 'NONE', #50946, #10686, #20988 ) ;
#64939=DIRECTION ( 'NONE',  ( 1.000000000000000000, -0.000000000000000000, 0.000000000000000000 ) ) ;
#64942=CIRCLE ( 'NONE', #19305, 4.999999999999999112 ) ;
#64943=EDGE_CURVE ( 'NONE', #6133, #59647, #8910, .T. ) ;
#64944=CIRCLE ( 'NONE', #27797, 5.000000000000001776 ) ;
#64946=CARTESIAN_POINT ( 'NONE',  ( -5.795121526828563852, -1.480313353269908649, 13.41892790137997338 ) ) ;
#64948=ORIENTED_EDGE ( 'NONE', *, *, #28508, .T. ) ;
#64951=DIRECTION ( 'NONE',  ( 0.000000000000000000, -0.8827602140260265573, 0.4698238015817460256 ) ) ;
#64953=B_SPLINE_CURVE_WITH_KNOTS ( 'NONE', 3,
 ( #51537, #36541, #27216, #62447, #47831, #42827, #22567, #52175, #15908, #41507, #56848, #26893, #47509, #5982, #22221, #37521, #32509, #42481, #62780, #17246 ),
 .UNSPECIFIED., .F., .F.,
 ( 4, 2, 2, 2, 2, 2, 2, 2, 2, 4 ),
 ( 0.000000000000000000, 0.001212774353530760669, 0.002425548707061521338, 0.003638323060592281357, 0.004244710237357661800, 0.004851097414123040942, 0.006063871767653796624, 0.007276646121184551438, 0.008489420474715306253, 0.009702194828246061067 ),
 .UNSPECIFIED. ) ;
#64954=ADVANCED_FACE ( 'NONE', ( #4570 ), #29802, .T. ) ;
#64958=DIRECTION ( 'NONE',  ( 0.000000000000000000, 0.9987865678893277366, -0.04924826701374931254 ) ) ;
#64960=EDGE_LOOP ( 'NONE', ( #37676, #52830, #46375, #43751 ) ) ;
#64961=DIRECTION ( 'NONE',  ( 1.000000000000000000, -0.000000000000000000, 0.000000000000000000 ) ) ;
#64962=CARTESIAN_POINT ( 'NONE',  ( -8.806666233050373549, -7.414420935576055527, -9.443457017163492395 ) ) ;
#64963=CARTESIAN_POINT ( 'NONE',  ( -18.36540788822463099, 3.954298550336713181, -11.33046690914046195 ) ) ;
#64964=ORIENTED_EDGE ( 'NONE', *, *, #31128, .F. ) ;
#64965=DIRECTION ( 'NONE',  ( -1.000000000000000000, 0.000000000000000000, 0.000000000000000000 ) ) ;
#64966=CARTESIAN_POINT ( 'NONE',  ( -37.00000000000000711, 12.66641127287626034, 1.457575200925590453 ) ) ;
#64967=ORIENTED_EDGE ( 'NONE', *, *, #29345, .F. ) ;
#64968=ORIENTED_EDGE ( 'NONE', *, *, #35880, .T. ) ;
#64970=CARTESIAN_POINT ( 'NONE',  ( -37.00000000000000711, -0.7536123767499333104, 11.72195762423409704 ) ) ;
#64971=VECTOR ( 'NONE', #65764, 1000.000000000000000 ) ;
#64972=AXIS2_PLACEMENT_3D ( 'NONE', #28578, #64163, #48882 ) ;
#64973=EDGE_LOOP ( 'NONE', ( #45179, #39369, #51530, #1451 ) ) ;
#64974=AXIS2_PLACEMENT_3D ( 'NONE', #61595, #41312, #31662 ) ;
#64975=DIRECTION ( 'NONE',  ( 1.000000000000000000, 0.000000000000000000, 0.000000000000000000 ) ) ;
#64976=DIRECTION ( 'NONE',  ( -1.000000000000000000, 0.000000000000000000, 0.000000000000000000 ) ) ;
#64980=VECTOR ( 'NONE', #36626, 1000.000000000000000 ) ;
#64985=EDGE_CURVE ( 'NONE', #23007, #4893, #34476, .T. ) ;
#64987=EDGE_LOOP ( 'NONE', ( #30026, #46602, #16014, #10537 ) ) ;
#64990=ORIENTED_EDGE ( 'NONE', *, *, #16472, .T. ) ;
#64991=ORIENTED_EDGE ( 'NONE', *, *, #32785, .T. ) ;
#64995=EDGE_CURVE ( 'NONE', #48418, #52930, #14212, .T. ) ;
#64997=DIRECTION ( 'NONE',  ( -1.000000000000000000, -0.000000000000000000, 0.000000000000000000 ) ) ;
#64999=EDGE_LOOP ( 'NONE', ( #10680, #56436, #18356, #46290 ) ) ;
#65000=ORIENTED_EDGE ( 'NONE', *, *, #36157, .F. ) ;
#65002=ORIENTED_EDGE ( 'NONE', *, *, #31916, .F. ) ;
#65003=ADVANCED_FACE ( 'NONE', ( #51442 ), #40788, .T. ) ;
#65006=CIRCLE ( 'NONE', #7688, 12.18649999999999878 ) ;
#65011=DIRECTION ( 'NONE',  ( -1.000000000000000000, 0.000000000000000000, 0.000000000000000000 ) ) ;
#65012=CARTESIAN_POINT ( 'NONE',  ( 26.73057806998188468, -13.02598523147789678, 3.554326270227990303 ) ) ;
#65013=ORIENTED_EDGE ( 'NONE', *, *, #12286, .T. ) ;
#65014=ORIENTED_EDGE ( 'NONE', *, *, #10293, .T. ) ;
#65016=DIRECTION ( 'NONE',  ( 0.000000000000000000, 0.8369827122275325104, 0.5472293298355300761 ) ) ;
#65017=CARTESIAN_POINT ( 'NONE',  ( 37.00000000000000711, 4.705694406421931860E-17, -3.469127814946512892E-15 ) ) ;
#65018=CIRCLE ( 'NONE', #58700, 12.18650000000000055 ) ;
#65019=AXIS2_PLACEMENT_3D ( 'NONE', #39289, #53293, #64241 ) ;
#65021=FACE_OUTER_BOUND ( 'NONE', #25473, .T. ) ;
#65024=CARTESIAN_POINT ( 'NONE',  ( 6.305306969373864590, -9.257074684086198602, -9.828058395331741082 ) ) ;
#65027=DIRECTION ( 'NONE',  ( 0.000000000000000000, 0.01356324068817998940, -0.9999080150203990547 ) ) ;
#65032=DIRECTION ( 'NONE',  ( 0.000000000000000000, 0.8369827122275362852, 0.5472293298355244140 ) ) ;
#65033=ADVANCED_BREP_SHAPE_REPRESENTATION ( '', ( #30113, #24966 ), #7986 ) ;
#65038=ORIENTED_EDGE ( 'NONE', *, *, #49618, .F. ) ;
#65043=CARTESIAN_POINT ( 'NONE',  ( 37.00000000000000711, 4.705694406421931860E-17, -3.469127814946512892E-15 ) ) ;
#65044=CARTESIAN_POINT ( 'NONE',  ( -27.45775109278350712, -13.35262336282553441, -1.989333891161978674 ) ) ;
#65046=VECTOR ( 'NONE', #26973, 1000.000000000000000 ) ;
#65047=LINE ( 'NONE', #19524, #15842 ) ;
#65050=CIRCLE ( 'NONE', #35341, 5.000000000000000000 ) ;
#65051=EDGE_CURVE ( 'NONE', #34193, #3983, #33361, .T. ) ;
#65054=CARTESIAN_POINT ( 'NONE',  ( -35.00000000000000000, 7.110831038798278492, 9.896810808925417646 ) ) ;
#65055=CARTESIAN_POINT ( 'NONE',  ( -8.502077647541781857, 10.07266980514430621, -8.994062260280561105 ) ) ;
#65056=DIRECTION ( 'NONE',  ( -1.000000000000000000, 0.000000000000000000, 0.000000000000000000 ) ) ;
#65057=CARTESIAN_POINT ( 'NONE',  ( 37.00000000000000711, 4.339012074899953220, -10.91536515067649660 ) ) ;
#65059=DIRECTION ( 'NONE',  ( -1.000000000000000000, 0.000000000000000000, 0.000000000000000000 ) ) ;
#65060=EDGE_CURVE ( 'NONE', #53158, #29384, #6803, .T. ) ;
#65062=LINE ( 'NONE', #5897, #1103 ) ;
#65066=CARTESIAN_POINT ( 'NONE',  ( -18.03417828546679047, -5.815239346579785362, -10.49772883765438358 ) ) ;
#65067=AXIS2_PLACEMENT_3D ( 'NONE', #4725, #45258, #24310 ) ;
#65068=VERTEX_POINT ( 'NONE', #35762 ) ;
#65070=LINE ( 'NONE', #23885, #14120 ) ;
#65071=ADVANCED_FACE ( 'NONE', ( #51098 ), #5554, .T. ) ;
#65072=DIRECTION ( 'NONE',  ( -0.000000000000000000, -1.000000000000000000, -0.000000000000000000 ) ) ;
#65073=ORIENTED_EDGE ( 'NONE', *, *, #36858, .T. ) ;
#65074=DIRECTION ( 'NONE',  ( 0.000000000000000000, -0.01356324068817998940, 0.9999080150203990547 ) ) ;
#65075=CARTESIAN_POINT ( 'NONE',  ( 9.575800908719084958, 11.95193887484099093, -1.072919909436247154 ) ) ;
#65076=CARTESIAN_POINT ( 'NONE',  ( 24.66186213270750116, -2.307346164574797687, 13.30714139060018653 ) ) ;
#65077=EDGE_CURVE ( 'NONE', #24451, #24519, #65204, .T. ) ;
#65078=ORIENTED_EDGE ( 'NONE', *, *, #56796, .F. ) ;
#65079=VECTOR ( 'NONE', #6076, 1000.000000000000000 ) ;
#65082=ORIENTED_EDGE ( 'NONE', *, *, #11450, .F. ) ;
#65083=CARTESIAN_POINT ( 'NONE',  ( 4.481592184329596940, -10.18497286202598318, -6.347143897620531661 ) ) ;
#65084=ORIENTED_EDGE ( 'NONE', *, *, #49946, .T. ) ;
#65085=CYLINDRICAL_SURFACE ( 'NONE', #42622, 5.000000000000000888 ) ;
#65086=CARTESIAN_POINT ( 'NONE',  ( -28.41827485489077532, 3.509237424706437292, 11.47541949982830722 ) ) ;
#65088=CARTESIAN_POINT ( 'NONE',  ( -14.29135464769095520, 7.782112657557433977, 11.03126115115966499 ) ) ;
#65089=AXIS2_PLACEMENT_3D ( 'NONE', #40955, #61547, #45604 ) ;
#65090=EDGE_CURVE ( 'NONE', #45080, #47268, #19844, .T. ) ;
#65092=ORIENTED_EDGE ( 'NONE', *, *, #37797, .T. ) ;
#65094=CARTESIAN_POINT ( 'NONE',  ( -35.00000000000000000, 0.000000000000000000, 0.000000000000000000 ) ) ;
#65097=DIRECTION ( 'NONE',  ( 0.000000000000000000, 0.01356324068817992175, -0.9999080150203990547 ) ) ;
#65098=AXIS2_PLACEMENT_3D ( 'NONE', #65459, #23618, #44520 ) ;
#65099=CARTESIAN_POINT ( 'NONE',  ( -18.57917586897355378, 13.44592621184941805, 1.251652577239034558 ) ) ;
#65100=CARTESIAN_POINT ( 'NONE',  ( 24.39670892413253256, -1.088878361238891923, 13.46081842674021090 ) ) ;
#65102=DIRECTION ( 'NONE',  ( 0.000000000000000000, 0.5767582926624911233, 0.8169148498130317515 ) ) ;
#65104=DIRECTION ( 'NONE',  ( -0.000000000000000000, -0.000000000000000000, -1.000000000000000000 ) ) ;
#65105=CIRCLE ( 'NONE', #53456, 12.18650000000000055 ) ;
#65106=AXIS2_PLACEMENT_3D ( 'NONE', #16250, #62437, #36534 ) ;
#65107=ORIENTED_EDGE ( 'NONE', *, *, #45580, .F. ) ;
#65109=VERTEX_POINT ( 'NONE', #5890 ) ;
#65111=CARTESIAN_POINT ( 'NONE',  ( 35.00000000000000000, -11.26103545359853264, 3.340853584269647847 ) ) ;
#65112=LINE ( 'NONE', #8946, #36711 ) ;
#65113=VECTOR ( 'NONE', #35587, 1000.000000000000000 ) ;
#65116=ORIENTED_EDGE ( 'NONE', *, *, #61641, .F. ) ;
#65118=DIRECTION ( 'NONE',  ( 1.000000000000000000, 0.000000000000000000, -0.000000000000000000 ) ) ;
#65119=CARTESIAN_POINT ( 'NONE',  ( -37.00000000000000711, 2.936739658820028520, -11.37311665002360783 ) ) ;
#65121=CARTESIAN_POINT ( 'NONE',  ( 3.459614771489464946, -11.09853614738469396, 4.563167253695070258 ) ) ;
#65122=B_SPLINE_CURVE_WITH_KNOTS ( 'NONE', 3,
 ( #52760, #27466, #28145, #63689, #18168, #59710 ),
 .UNSPECIFIED., .F., .F.,
 ( 4, 2, 4 ),
 ( 0.009913722359341532037, 0.01153912928143344119, 0.01316453620352535034 ),
 .UNSPECIFIED. ) ;
#65123=EDGE_CURVE ( 'NONE', #38116, #40447, #41413, .T. ) ;
#65125=ADVANCED_FACE ( 'NONE', ( #6857 ), #6520, .T. ) ;
#65126=ORIENTED_EDGE ( 'NONE', *, *, #21774, .F. ) ;
#65127=AXIS2_PLACEMENT_3D ( 'NONE', #47858, #2315, #36888 ) ;
#65128=CYLINDRICAL_SURFACE ( 'NONE', #11592, 4.785769192180104881 ) ;
#65130=DIRECTION ( 'NONE',  ( 0.000000000000000000, -0.01356324068817999114, 0.9999080150203989437 ) ) ;
#65131=CARTESIAN_POINT ( 'NONE',  ( -37.00000000000000711, 8.534258022646220354, -8.699265615722891809 ) ) ;
#65132=ADVANCED_FACE ( 'NONE', ( #27127 ), #11491, .T. ) ;
#65133=CARTESIAN_POINT ( 'NONE',  ( 35.00000000000000000, 10.59380114696469732, -7.094637218249395971 ) ) ;
#65134=CARTESIAN_POINT ( 'NONE',  ( -29.60173393771532346, -2.916829795459872088, -13.20259329781003466 ) ) ;
#65135=AXIS2_PLACEMENT_3D ( 'NONE', #27539, #47836, #42833 ) ;
#65136=EDGE_CURVE ( 'NONE', #45350, #15359, #7881, .T. ) ;
#65137=ORIENTED_EDGE ( 'NONE', *, *, #11476, .T. ) ;
#65139=DIRECTION ( 'NONE',  ( -1.000000000000000000, -0.000000000000000000, 0.000000000000000000 ) ) ;
#65141=LINE ( 'NONE', #40866, #23442 ) ;
#65142=FACE_OUTER_BOUND ( 'NONE', #44539, .T. ) ;
#65144=DIRECTION ( 'NONE',  ( 1.000000000000000000, 0.000000000000000000, 0.000000000000000000 ) ) ;
#65146=FACE_OUTER_BOUND ( 'NONE', #56001, .T. ) ;
#65147=EDGE_LOOP ( 'NONE', ( #2726, #50132, #14321, #44183 ) ) ;
#65151=ORIENTED_EDGE ( 'NONE', *, *, #40446, .T. ) ;
#65152=CARTESIAN_POINT ( 'NONE',  ( 0.1900979142430820334, -0.2738684153833554902, 13.49791647769710679 ) ) ;
#65153=LINE ( 'NONE', #33909, #42735 ) ;
#65154=ORIENTED_EDGE ( 'NONE', *, *, #6461, .F. ) ;
#65155=B_SPLINE_CURVE_WITH_KNOTS ( 'NONE', 3,
 ( #50066, #24796, #45076, #65344, #19808, #9809, #50408, #60354, #4854, #25122, #26110, #16462, #41715, #1510, #56023, #30428, #20783, #41055, #21444, #518, #35728, #16117 ),
 .UNSPECIFIED., .F., .F.,
 ( 4, 2, 2, 2, 2, 2, 2, 2, 2, 2, 4 ),
 ( 0.003549775680923942470, 0.004881064640633089174, 0.005546709120487661009, 0.006212353600342233710, 0.007543642560051378246, 0.008209287039905950947, 0.008874931519760523649, 0.01020622047946966905, 0.01153750943917881445, 0.01286879839888795986, 0.01420008735859710700 ),
 .UNSPECIFIED. ) ;
#65156=CARTESIAN_POINT ( 'NONE',  ( -35.00000000000000000, 0.000000000000000000, 0.000000000000000000 ) ) ;
#65157=ORIENTED_EDGE ( 'NONE', *, *, #10656, .T. ) ;
#65158=DIRECTION ( 'NONE',  ( -0.000000000000000000, -0.000000000000000000, -1.000000000000000000 ) ) ;
#65159=VECTOR ( 'NONE', #12872, 1000.000000000000000 ) ;
#65160=CARTESIAN_POINT ( 'NONE',  ( 37.00000000000000711, 8.029056188533806093, 8.573591947375229338 ) ) ;
#65162=EDGE_CURVE ( 'NONE', #62155, #64321, #64164, .T. ) ;
#65163=CARTESIAN_POINT ( 'NONE',  ( 7.266065016736156679, -6.970945981239493605, 9.778723759522906178 ) ) ;
#65165=CIRCLE ( 'NONE', #45005, 5.000000000000000888 ) ;
#65166=ORIENTED_EDGE ( 'NONE', *, *, #12556, .T. ) ;
#65167=DIRECTION ( 'NONE',  ( -1.000000000000000000, 0.000000000000000000, 0.000000000000000000 ) ) ;
#65168=EDGE_CURVE ( 'NONE', #16649, #28605, #21826, .T. ) ;
#65169=ORIENTED_EDGE ( 'NONE', *, *, #2612, .T. ) ;
#65170=LINE ( 'NONE', #4010, #48630 ) ;
#65171=ORIENTED_EDGE ( 'NONE', *, *, #49376, .F. ) ;
#65172=CIRCLE ( 'NONE', #17386, 5.000000000000000000 ) ;
#65176=CARTESIAN_POINT ( 'NONE',  ( -35.00000000000000000, -10.75351884295731253, 4.725891942574718563 ) ) ;
#65177=AXIS2_PLACEMENT_3D ( 'NONE', #28758, #35372, #30395 ) ;
#65179=DIRECTION ( 'NONE',  ( -1.000000000000000000, 0.000000000000000000, -0.000000000000000000 ) ) ;
#65181=ORIENTED_EDGE ( 'NONE', *, *, #44997, .T. ) ;
#65184=VERTEX_POINT ( 'NONE', #11813 ) ;
#65185=FACE_OUTER_BOUND ( 'NONE', #56986, .T. ) ;
#65186=AXIS2_PLACEMENT_3D ( 'NONE', #47455, #1895, #17184 ) ;
#65187=CARTESIAN_POINT ( 'NONE',  ( 37.00000000000000711, -11.80185301892977279, 4.824807283154243898 ) ) ;
#65188=EDGE_CURVE ( 'NONE', #25928, #16089, #32253, .T. ) ;
#65189=VERTEX_POINT ( 'NONE', #62678 ) ;
#65191=DIRECTION ( 'NONE',  ( 0.000000000000000000, -0.6269146997507875074, -0.7790879021242596014 ) ) ;
#65193=ORIENTED_EDGE ( 'NONE', *, *, #64000, .F. ) ;
#65195=ORIENTED_EDGE ( 'NONE', *, *, #21728, .F. ) ;
#65198=CARTESIAN_POINT ( 'NONE',  ( -24.67014067453516901, -8.921734260348005208, 10.13897465123165453 ) ) ;
#65202=CARTESIAN_POINT ( 'NONE',  ( 13.30993466298489913, 10.25874852760247968, -6.229666527591529501 ) ) ;
#65203=ORIENTED_EDGE ( 'NONE', *, *, #26975, .F. ) ;
#65204=CIRCLE ( 'NONE', #39711, 12.18650000000000055 ) ;
#65205=CIRCLE ( 'NONE', #11099, 12.74999999999999822 ) ;
#65207=LINE ( 'NONE', #52865, #57775 ) ;
#65208=CARTESIAN_POINT ( 'NONE',  ( -35.00000000000000000, 0.000000000000000000, 0.000000000000000000 ) ) ;
#65209=DIRECTION ( 'NONE',  ( -1.000000000000000000, 0.000000000000000000, 0.000000000000000000 ) ) ;
#65214=DIRECTION ( 'NONE',  ( 0.000000000000000000, 0.01356324068817999114, -0.9999080150203989437 ) ) ;
#65216=VECTOR ( 'NONE', #58014, 1000.000000000000000 ) ;
#65217=ADVANCED_FACE ( 'NONE', ( #53044 ), #7481, .T. ) ;
#65218=CIRCLE ( 'NONE', #36562, 4.999999999999997335 ) ;
#65219=ORIENTED_EDGE ( 'NONE', *, *, #22706, .F. ) ;
#65220=DIRECTION ( 'NONE',  ( 0.000000000000000000, -0.9937233664769772323, 0.1118654143051511785 ) ) ;
#65222=CARTESIAN_POINT ( 'NONE',  ( 37.00000000000000711, 6.280308599560279426, 9.926225166346956286 ) ) ;
#65223=DIRECTION ( 'NONE',  ( -0.1298914529148032515, 0.000000000000000000, -0.9915282196991074271 ) ) ;
#65224=LINE ( 'NONE', #29632, #39581 ) ;
#65226=CARTESIAN_POINT ( 'NONE',  ( -35.00000000000000000, 6.280308599560139093, 9.926225166347048656 ) ) ;
#65227=ORIENTED_EDGE ( 'NONE', *, *, #2730, .F. ) ;
#65228=EDGE_CURVE ( 'NONE', #52347, #19909, #5803, .T. ) ;
#65229=CIRCLE ( 'NONE', #16405, 12.74999999999999822 ) ;
#65232=CARTESIAN_POINT ( 'NONE',  ( 29.72995639581280969, -7.926718941844264954, 9.022826046292943047 ) ) ;
#65234=AXIS2_PLACEMENT_3D ( 'NONE', #11947, #46241, #26928 ) ;
#65236=VERTEX_POINT ( 'NONE', #28422 ) ;
#65237=CARTESIAN_POINT ( 'NONE',  ( 35.00000000000000000, -9.821084925794620446, -7.215058775251224077 ) ) ;
#65238=FACE_OUTER_BOUND ( 'NONE', #12327, .T. ) ;
#65240=LINE ( 'NONE', #9056, #8889 ) ;
#65241=ORIENTED_EDGE ( 'NONE', *, *, #30663, .T. ) ;
#65243=DIRECTION ( 'NONE',  ( -0.1298914529148032515, 0.000000000000000000, -0.9915282196991074271 ) ) ;
#65245=DIRECTION ( 'NONE',  ( -1.000000000000000000, 0.000000000000000000, 0.000000000000000000 ) ) ;
#65249=EDGE_LOOP ( 'NONE', ( #60641, #16964, #65151, #15925 ) ) ;
#65250=AXIS2_PLACEMENT_3D ( 'NONE', #55990, #30393, #46030 ) ;
#65252=CIRCLE ( 'NONE', #46140, 12.18649999999999878 ) ;
#65253=ORIENTED_EDGE ( 'NONE', *, *, #45596, .T. ) ;
#65254=DIRECTION ( 'NONE',  ( -1.000000000000000000, 0.000000000000000000, 0.000000000000000000 ) ) ;
#65255=CARTESIAN_POINT ( 'NONE',  ( -35.00000000000000000, 0.000000000000000000, 0.000000000000000000 ) ) ;
#65256=ADVANCED_FACE ( 'NONE', ( #59347 ), #48724, .T. ) ;
#65257=DIRECTION ( 'NONE',  ( 0.000000000000000000, 0.01356324068817998940, -0.9999080150203990547 ) ) ;
#65260=DIRECTION ( 'NONE',  ( -1.000000000000000000, 0.000000000000000000, 0.000000000000000000 ) ) ;
#65262=CARTESIAN_POINT ( 'NONE',  ( -37.00000000000000711, -3.805206332242559775, 12.16893194857548899 ) ) ;
#65263=DIRECTION ( 'NONE',  ( 1.000000000000000000, 0.000000000000000000, 0.000000000000000000 ) ) ;
#65264=VERTEX_POINT ( 'NONE', #18486 ) ;
#65265=EDGE_CURVE ( 'NONE', #27835, #35397, #16417, .T. ) ;
#65268=EDGE_LOOP ( 'NONE', ( #40696, #25005, #44155, #45283 ) ) ;
#65269=EDGE_CURVE ( 'NONE', #10311, #17416, #30221, .T. ) ;
#65272=DIRECTION ( 'NONE',  ( -1.000000000000000000, 0.000000000000000000, -0.000000000000000000 ) ) ;
#65273=DIRECTION ( 'NONE',  ( 0.000000000000000000, -0.8827602140260265573, 0.4698238015817460256 ) ) ;
#65274=DIRECTION ( 'NONE',  ( 0.000000000000000000, 0.01356324068817998940, -0.9999080150203990547 ) ) ;
#65276=EDGE_CURVE ( 'NONE', #41059, #43621, #8812, .T. ) ;
#65277=DIRECTION ( 'NONE',  ( 1.000000000000000000, -0.000000000000000000, -0.000000000000000000 ) ) ;
#65278=ORIENTED_EDGE ( 'NONE', *, *, #64119, .F. ) ;
#65280=CARTESIAN_POINT ( 'NONE',  ( 37.00000000000000711, 0.000000000000000000, -1.750000000000000000 ) ) ;
#65281=DIRECTION ( 'NONE',  ( 0.000000000000000000, -0.01356324068817991828, 0.9999080150203990547 ) ) ;
#65284=CIRCLE ( 'NONE', #52548, 12.00000000000000000 ) ;
#65287=CARTESIAN_POINT ( 'NONE',  ( -27.27855387000350262, -10.59660315834921107, 5.631341004100471892 ) ) ;
#65288=CYLINDRICAL_SURFACE ( 'NONE', #4151, 5.000000000000000888 ) ;
#65289=ORIENTED_EDGE ( 'NONE', *, *, #15988, .F. ) ;
#65290=DIRECTION ( 'NONE',  ( 1.000000000000000000, 0.000000000000000000, 0.000000000000000000 ) ) ;
#65291=AXIS2_PLACEMENT_3D ( 'NONE', #40620, #60913, #47195 ) ;
#65293=CARTESIAN_POINT ( 'NONE',  ( 0.2851083653049504285, -0.4107471485392698018, 11.99296822225285730 ) ) ;
#65297=EDGE_LOOP ( 'NONE', ( #62429, #27969, #56138, #12714 ) ) ;
#65299=CARTESIAN_POINT ( 'NONE',  ( -7.489022030332961322, -5.127957880411574187, -10.84914964302385521 ) ) ;
#65302=CARTESIAN_POINT ( 'NONE',  ( 9.383873380784992335, 1.701316094559147230, 13.39399859679633487 ) ) ;
#65303=DIRECTION ( 'NONE',  ( 0.000000000000000000, 0.3218879778915972878, -0.9467777615094571386 ) ) ;
#65305=ADVANCED_FACE ( 'NONE', ( #24101 ), #48407, .T. ) ;
#65306=EDGE_CURVE ( 'NONE', #10842, #42133, #2535, .T. ) ;
#65309=EDGE_CURVE ( 'NONE', #60760, #27227, #47242, .T. ) ;
#65310=CIRCLE ( 'NONE', #35549, 4.999999999999999112 ) ;
#65311=ORIENTED_EDGE ( 'NONE', *, *, #41164, .F. ) ;
#65313=CARTESIAN_POINT ( 'NONE',  ( -36.00000000000000711, 9.196955404009424129, -8.830544224262844466 ) ) ;
#65314=DIRECTION ( 'NONE',  ( -1.000000000000000000, 0.000000000000000000, 0.000000000000000000 ) ) ;
#65317=CARTESIAN_POINT ( 'NONE',  ( -17.58076563216013355, 11.47010079780622682, 3.542952125472129232 ) ) ;
#65318=DIRECTION ( 'NONE',  ( 0.000000000000000000, 0.01356324068817998940, -0.9999080150203990547 ) ) ;
#65323=ORIENTED_EDGE ( 'NONE', *, *, #6188, .F. ) ;
#65324=VERTEX_POINT ( 'NONE', #9126 ) ;
#65327=EDGE_CURVE ( 'NONE', #10194, #44696, #24414, .T. ) ;
#65328=DIRECTION ( 'NONE',  ( 0.000000000000000000, 0.7790879021242527180, -0.6269146997507960561 ) ) ;
#65329=VECTOR ( 'NONE', #54344, 1000.000000000000000 ) ;
#65332=CARTESIAN_POINT ( 'NONE',  ( -35.00000000000000000, -12.09831040184925044, 1.463443770872731919 ) ) ;
#65334=VERTEX_POINT ( 'NONE', #23115 ) ;
#65335=DIRECTION ( 'NONE',  ( 1.000000000000000000, -0.000000000000000000, -0.000000000000000000 ) ) ;
#65337=VERTEX_POINT ( 'NONE', #38404 ) ;
#65338=DIRECTION ( 'NONE',  ( -0.000000000000000000, -0.000000000000000000, -1.000000000000000000 ) ) ;
#65341=B_SPLINE_CURVE_WITH_KNOTS ( 'NONE', 3,
 ( #61138, #60810, #15567, #35832, #15247, #35531, #16239, #56133, #6274, #55827, #945, #62121, #10253, #61441, #21213, #41487, #15885, #36522 ),
 .UNSPECIFIED., .F., .F.,
 ( 4, 2, 2, 2, 2, 2, 2, 2, 4 ),
 ( 1.086801142668811545E-17, 0.002754147681809471920, 0.004131221522714200942, 0.005508295363618930830, 0.006196832284071292739, 0.006885369204523654647, 0.008262443045428381067, 0.009639516886333108353, 0.01101659072723783737 ),
 .UNSPECIFIED. ) ;
#65343=EDGE_CURVE ( 'NONE', #41765, #38476, #32301, .T. ) ;
#65344=CARTESIAN_POINT ( 'NONE',  ( -11.28047536261793304, -6.236380125593958823, -10.25457663355916083 ) ) ;
#65345=FACE_OUTER_BOUND ( 'NONE', #50228, .T. ) ;
#65347=CIRCLE ( 'NONE', #1628, 4.999999999999999112 ) ;
#65349=CARTESIAN_POINT ( 'NONE',  ( -35.00000000000000000, -10.62137734850264614, -5.015831474386418520 ) ) ;
#65350=CARTESIAN_POINT ( 'NONE',  ( -47.00000000000000711, 0.000000000000000000, 0.000000000000000000 ) ) ;
#65352=DIRECTION ( 'NONE',  ( -0.000000000000000000, -1.000000000000000000, -0.000000000000000000 ) ) ;
#65353=CARTESIAN_POINT ( 'NONE',  ( -35.00000000000000000, 6.753013023069858178, -10.14433819232427147 ) ) ;
#65355=CARTESIAN_POINT ( 'NONE',  ( -7.008316857174801129, -1.821497689352610694, -11.86115302356136780 ) ) ;
#65356=DIRECTION ( 'NONE',  ( -1.000000000000000000, -0.000000000000000000, 0.000000000000000000 ) ) ;
#65360=FACE_OUTER_BOUND ( 'NONE', #18048, .T. ) ;
#65362=AXIS2_PLACEMENT_3D ( 'NONE', #24893, #20218, #40495 ) ;
#65366=ORIENTED_EDGE ( 'NONE', *, *, #54628, .T. ) ;
#65370=VERTEX_POINT ( 'NONE', #41020 ) ;
#65371=DIRECTION ( 'NONE',  ( 1.000000000000000000, 0.000000000000000000, 0.000000000000000000 ) ) ;
#65372=CARTESIAN_POINT ( 'NONE',  ( 37.00000000000000711, -4.041347439435937439, -11.02904044024207764 ) ) ;
#65375=DIRECTION ( 'NONE',  ( 0.000000000000000000, -0.01356324068817991828, 0.9999080150203990547 ) ) ;
#65377=DIRECTION ( 'NONE',  ( 1.000000000000000000, 0.000000000000000000, 0.000000000000000000 ) ) ;
#65378=VERTEX_POINT ( 'NONE', #4821 ) ;
#65379=DIRECTION ( 'NONE',  ( 0.000000000000000000, -0.01356324068817991828, 0.9999080150203990547 ) ) ;
#65380=CARTESIAN_POINT ( 'NONE',  ( -37.00000000000000711, 9.908974237959645492, 6.307491713049065751 ) ) ;
#65382=VECTOR ( 'NONE', #25536, 1000.000000000000000 ) ;
#65383=CARTESIAN_POINT ( 'NONE',  ( -47.00000000000000711, 0.000000000000000000, 0.000000000000000000 ) ) ;
#65385=CARTESIAN_POINT ( 'NONE',  ( 35.00000000000000000, 10.49591321039688019, 5.273331777780226659 ) ) ;
#65386=DIRECTION ( 'NONE',  ( -1.000000000000000000, -0.000000000000000000, 0.000000000000000000 ) ) ;
#65387=EDGE_LOOP ( 'NONE', ( #39286, #39956, #6147, #19730 ) ) ;
#65388=VERTEX_POINT ( 'NONE', #14747 ) ;
#65390=VERTEX_POINT ( 'NONE', #45356 ) ;
#65392=LINE ( 'NONE', #5226, #8599 ) ;
#65394=CYLINDRICAL_SURFACE ( 'NONE', #26609, 14.19297241773857188 ) ;
#65395=CARTESIAN_POINT ( 'NONE',  ( -27.22214261968803939, -12.41558776886551740, 5.304269109247355729 ) ) ;
#65396=CARTESIAN_POINT ( 'NONE',  ( 37.00000000000000711, 4.705694406421931860E-17, -3.469127814946512892E-15 ) ) ;
#65397=ORIENTED_EDGE ( 'NONE', *, *, #23413, .F. ) ;
#65398=ORIENTED_EDGE ( 'NONE', *, *, #27265, .T. ) ;
#65399=CARTESIAN_POINT ( 'NONE',  ( -35.00000000000000000, 0.000000000000000000, 0.000000000000000000 ) ) ;
#65401=ORIENTED_EDGE ( 'NONE', *, *, #13297, .T. ) ;
#65403=ORIENTED_EDGE ( 'NONE', *, *, #10166, .T. ) ;
#65404=LINE ( 'NONE', #10875, #9696 ) ;
#65407=DIRECTION ( 'NONE',  ( -0.000000000000000000, -0.000000000000000000, -1.000000000000000000 ) ) ;
#65409=CARTESIAN_POINT ( 'NONE',  ( -14.23194138997495450, 7.940651831586622578, -10.91941811743712876 ) ) ;
#65414=CARTESIAN_POINT ( 'NONE',  ( -18.79799054488956145, 13.49111078119409157, 0.5911816625682176918 ) ) ;
#65415=CARTESIAN_POINT ( 'NONE',  ( 24.20164632272273764, 0.6982551168995920765, 13.48650918581359548 ) ) ;
#65416=DIRECTION ( 'NONE',  ( 0.000000000000000000, -0.4698238015817237656, -0.8827602140260383257 ) ) ;
#65421=EDGE_LOOP ( 'NONE', ( #4998, #53895, #660, #61168 ) ) ;
#65422=CARTESIAN_POINT ( 'NONE',  ( -18.13077481406540414, 6.846344537678046294, -9.858992475546884293 ) ) ;
#65424=VECTOR ( 'NONE', #59992, 1000.000000000000000 ) ;
#65425=EDGE_CURVE ( 'NONE', #51491, #7491, #53600, .T. ) ;
#65427=ORIENTED_EDGE ( 'NONE', *, *, #553, .T. ) ;
#65428=EDGE_CURVE ( 'NONE', #63812, #25246, #8962, .T. ) ;
#65433=EDGE_CURVE ( 'NONE', #64603, #49077, #20649, .T. ) ;
#65434=DIRECTION ( 'NONE',  ( 1.000000000000000000, 0.000000000000000000, 0.000000000000000000 ) ) ;
#65435=VERTEX_POINT ( 'NONE', #40034 ) ;
#65438=CARTESIAN_POINT ( 'NONE',  ( 9.102723003675967206, 3.312403327918474361, 11.53614311619802812 ) ) ;
#65440=EDGE_CURVE ( 'NONE', #13128, #56608, #46139, .T. ) ;
#65441=CARTESIAN_POINT ( 'NONE',  ( 10.75853767213705225, 7.830989516993144051, -10.99661780661415733 ) ) ;
#65443=ORIENTED_EDGE ( 'NONE', *, *, #63398, .T. ) ;
#65444=ADVANCED_FACE ( 'NONE', ( #10761 ), #10114, .T. ) ;
#65448=CARTESIAN_POINT ( 'NONE',  ( -35.00000000000000000, -4.986700593229626222, -10.63508530065527147 ) ) ;
#65450=CARTESIAN_POINT ( 'NONE',  ( 35.00000000000000000, 4.705694406421931860E-17, -3.469127814946512892E-15 ) ) ;
#65451=VERTEX_POINT ( 'NONE', #56672 ) ;
#65452=ORIENTED_EDGE ( 'NONE', *, *, #27050, .F. ) ;
#65454=EDGE_CURVE ( 'NONE', #10789, #13395, #35024, .T. ) ;
#65455=ORIENTED_EDGE ( 'NONE', *, *, #24483, .F. ) ;
#65459=CARTESIAN_POINT ( 'NONE',  ( 35.00000000000000000, -6.036400161834636791, -10.07641281632175634 ) ) ;
#65461=CARTESIAN_POINT ( 'NONE',  ( -35.00000000000000000, 10.80631716521666874, 4.603882218679588689 ) ) ;
#65462=CARTESIAN_POINT ( 'NONE',  ( -19.02967556479664069, -11.99999999999998934, 9.262893081595934602E-16 ) ) ;
#65463=VERTEX_POINT ( 'NONE', #50691 ) ;
#65466=ORIENTED_EDGE ( 'NONE', *, *, #8534, .F. ) ;
#65467=VECTOR ( 'NONE', #23817, 1000.000000000000000 ) ;
#65470=ORIENTED_EDGE ( 'NONE', *, *, #37699, .F. ) ;
#65472=CARTESIAN_POINT ( 'NONE',  ( 35.00000000000000000, 4.705694406421931860E-17, -3.469127814946512892E-15 ) ) ;
#65473=ORIENTED_EDGE ( 'NONE', *, *, #55830, .T. ) ;
#65475=CARTESIAN_POINT ( 'NONE',  ( 3.347841273039249721, -10.61118957148187825, -8.345816669330458737 ) ) ;
#65476=CARTESIAN_POINT ( 'NONE',  ( 17.27839441901508621, 10.52068335315811076, 5.771933972472480967 ) ) ;
#65478=ORIENTED_EDGE ( 'NONE', *, *, #15964, .T. ) ;
#65481=ORIENTED_EDGE ( 'NONE', *, *, #42742, .T. ) ;
#65483=ORIENTED_EDGE ( 'NONE', *, *, #25315, .T. ) ;
#65484=ORIENTED_EDGE ( 'NONE', *, *, #48253, .F. ) ;
#65485=CARTESIAN_POINT ( 'NONE',  ( 37.00000000000000711, -9.196955404009232282, 8.830544224263041642 ) ) ;
#65487=EDGE_CURVE ( 'NONE', #3518, #44848, #50414, .T. ) ;
#65488=CARTESIAN_POINT ( 'NONE',  ( 37.00000000000000711, -12.16893194857552629, -3.805206332242429212 ) ) ;
#65491=DIRECTION ( 'NONE',  ( 0.000000000000000000, -0.01356324068817998940, 0.9999080150203990547 ) ) ;
#65492=ORIENTED_EDGE ( 'NONE', *, *, #28974, .T. ) ;
#65493=CARTESIAN_POINT ( 'NONE',  ( 35.00000000000000000, -7.745827850123079727, -10.12742074351894139 ) ) ;
#65494=DIRECTION ( 'NONE',  ( 0.000000000000000000, 0.01356324068817998940, -0.9999080150203990547 ) ) ;
#65495=EDGE_LOOP ( 'NONE', ( #57386, #57092, #35721, #4597 ) ) ;
#65499=ADVANCED_FACE ( 'NONE', ( #142 ), #20420, .T. ) ;
#65500=ORIENTED_EDGE ( 'NONE', *, *, #33858, .F. ) ;
#65503=ORIENTED_EDGE ( 'NONE', *, *, #46322, .T. ) ;
#65505=CARTESIAN_POINT ( 'NONE',  ( -35.00000000000000000, -11.65150730582933392, -1.488153103997089888 ) ) ;
#65507=CARTESIAN_POINT ( 'NONE',  ( -37.00000000000000711, 12.01765980939845058, -2.021542716731266065 ) ) ;
#65508=CARTESIAN_POINT ( 'NONE',  ( 37.00000000000000711, -0.4353888892049205261, -11.73808581813437968 ) ) ;
#65509=ADVANCED_FACE ( 'NONE', ( #31048 ), #32657, .T. ) ;
#65510=CARTESIAN_POINT ( 'NONE',  ( -19.69476066079020171, -4.201994156881551312, -12.82938989607585789 ) ) ;
#65511=ORIENTED_EDGE ( 'NONE', *, *, #28508, .F. ) ;
#65512=DIRECTION ( 'NONE',  ( 0.000000000000000000, 0.01356324068817992175, -0.9999080150203990547 ) ) ;
#65513=CARTESIAN_POINT ( 'NONE',  ( 35.00000000000000000, -8.029056188533749250, -8.573591947375291511 ) ) ;
#65515=VECTOR ( 'NONE', #8673, 1000.000000000000000 ) ;
#65516=LINE ( 'NONE', #33958, #10451 ) ;
#65519=EDGE_CURVE ( 'NONE', #9279, #7682, #2631, .T. ) ;
#65522=DIRECTION ( 'NONE',  ( 0.000000000000000000, -0.5987040770935736500, 0.8009703041134121904 ) ) ;
#65523=CARTESIAN_POINT ( 'NONE',  ( 36.00000000000000711, 10.02106554660720050, 7.882940143791662635 ) ) ;
#65524=CYLINDRICAL_SURFACE ( 'NONE', #19507, 12.74999999999999822 ) ;
#65528=EDGE_CURVE ( 'NONE', #53824, #36705, #40499, .T. ) ;
#65529=VERTEX_POINT ( 'NONE', #47345 ) ;
#65530=DIRECTION ( 'NONE',  ( 0.000000000000000000, 0.01356324068817992175, -0.9999080150203990547 ) ) ;
#65532=DIRECTION ( 'NONE',  ( 0.000000000000000000, -0.01356324068817999114, 0.9999080150203989437 ) ) ;
#65533=ADVANCED_FACE ( 'NONE', ( #42305 ), #52967, .T. ) ;
#65537=EDGE_LOOP ( 'NONE', ( #49054, #60745, #26183, #48847 ) ) ;
#65543=FACE_OUTER_BOUND ( 'NONE', #9637, .T. ) ;
#65545=ORIENTED_EDGE ( 'NONE', *, *, #63203, .T. ) ;
#65548=DIRECTION ( 'NONE',  ( 0.000000000000000000, 0.8009703041134189627, 0.5987040770935648792 ) ) ;
#65549=DIRECTION ( 'NONE',  ( 0.000000000000000000, 0.01356324068817992175, -0.9999080150203990547 ) ) ;
#65550=ORIENTED_EDGE ( 'NONE', *, *, #54120, .T. ) ;
#65552=ORIENTED_EDGE ( 'NONE', *, *, #59917, .T. ) ;
#65553=DIRECTION ( 'NONE',  ( 1.000000000000000000, 0.000000000000000000, 0.000000000000000000 ) ) ;
#65555=EDGE_LOOP ( 'NONE', ( #48199, #33009, #22472, #11961 ) ) ;
#65556=CIRCLE ( 'NONE', #36910, 5.000000000000001776 ) ;
#65557=CARTESIAN_POINT ( 'NONE',  ( -29.54288940436046929, 0.2973637493423957889, -11.99820176872441024 ) ) ;
#65558=CARTESIAN_POINT ( 'NONE',  ( 12.85578295477420951, -9.379166698650648115, -7.488245662904835065 ) ) ;
#65560=FACE_OUTER_BOUND ( 'NONE', #28035, .T. ) ;
#65561=CYLINDRICAL_SURFACE ( 'NONE', #62294, 4.999999999999999112 ) ;
#65562=ADVANCED_FACE ( 'NONE', ( #26385 ), #52336, .T. ) ;
#65568=CARTESIAN_POINT ( 'NONE',  ( 12.58609921286428879, 13.26567957380986407, -2.535074658557892935 ) ) ;
#65569=ORIENTED_EDGE ( 'NONE', *, *, #18551, .T. ) ;
#65571=ORIENTED_EDGE ( 'NONE', *, *, #24453, .T. ) ;
#65572=LINE ( 'NONE', #34659, #34832 ) ;
#65573=ORIENTED_EDGE ( 'NONE', *, *, #58285, .F. ) ;
#65574=B_SPLINE_CURVE_WITH_KNOTS ( 'NONE', 3,
 ( #26777, #47076, #12447, #32717, #33066, #58032, #57369, #17465, #32077, #27111, #62034, #53372, #11795, #62656, #7819, #2843, #52393, #16485, #47406, #6504, #28102, #6840, #57711, #21810 ),
 .UNSPECIFIED., .F., .F.,
 ( 4, 2, 2, 2, 2, 2, 2, 2, 2, 2, 2, 4 ),
 ( 0.000000000000000000, 0.0005079441056328478201, 0.001015888211265695640, 0.001523832316898543352, 0.002031776422531391280, 0.002539720528164238992, 0.003047664633797086704, 0.004063552845062785163, 0.005079441056328483188, 0.006095329267594181213, 0.007111217478859880106, 0.008127105690125578999 ),
 .UNSPECIFIED. ) ;
#65575=ORIENTED_EDGE ( 'NONE', *, *, #36917, .T. ) ;
#65581=DIRECTION ( 'NONE',  ( 0.000000000000000000, 0.01356324068817998940, -0.9999080150203989437 ) ) ;
#65582=EDGE_CURVE ( 'NONE', #52407, #42299, #28095, .T. ) ;
#65583=DIRECTION ( 'NONE',  ( 0.000000000000000000, -0.01356324068817999114, 0.9999080150203989437 ) ) ;
#65584=ORIENTED_EDGE ( 'NONE', *, *, #65309, .F. ) ;
#65585=DIRECTION ( 'NONE',  ( -1.000000000000000000, 0.000000000000000000, -0.000000000000000000 ) ) ;
#65586=CYLINDRICAL_SURFACE ( 'NONE', #41922, 12.18650000000000055 ) ;
#65589=ORIENTED_EDGE ( 'NONE', *, *, #53702, .T. ) ;
#65590=VECTOR ( 'NONE', #4516, 1000.000000000000000 ) ;
#65592=CARTESIAN_POINT ( 'NONE',  ( -6.597603250208732284, -1.668269591273481067, 13.39685896832295953 ) ) ;
#65595=FACE_OUTER_BOUND ( 'NONE', #40660, .T. ) ;
#65597=CARTESIAN_POINT ( 'NONE',  ( 37.00000000000000711, -8.295159312811920316, -8.927548052240867449 ) ) ;
#65598=DIRECTION ( 'NONE',  ( 1.000000000000000000, 0.000000000000000000, 0.000000000000000000 ) ) ;
#65599=CIRCLE ( 'NONE', #48646, 4.999999999999999112 ) ;
#65600=EDGE_CURVE ( 'NONE', #54679, #39152, #45126, .T. ) ;
#65601=EDGE_CURVE ( 'NONE', #34584, #19083, #56828, .T. ) ;
#65602=DIRECTION ( 'NONE',  ( -1.000000000000000000, 0.000000000000000000, 0.000000000000000000 ) ) ;
#65605=ORIENTED_EDGE ( 'NONE', *, *, #15651, .T. ) ;
#65608=DIRECTION ( 'NONE',  ( 1.000000000000000000, -0.000000000000000000, 0.000000000000000000 ) ) ;
#65609=ORIENTED_EDGE ( 'NONE', *, *, #63879, .T. ) ;
#65610=EDGE_CURVE ( 'NONE', #25109, #56567, #51514, .T. ) ;
#65611=DIRECTION ( 'NONE',  ( 0.5417962735734949131, 0.000000000000000000, -0.8405098440481674205 ) ) ;
#65614=ORIENTED_EDGE ( 'NONE', *, *, #3698, .T. ) ;
#65615=EDGE_LOOP ( 'NONE', ( #33662, #15417, #56341, #30897 ) ) ;
#65619=CARTESIAN_POINT ( 'NONE',  ( -35.00000000000000000, -6.280308599560071592, -9.926225166347094842 ) ) ;
#65620=DIRECTION ( 'NONE',  ( 0.000000000000000000, 0.000000000000000000, -1.000000000000000000 ) ) ;
#65621=CIRCLE ( 'NONE', #36967, 12.74999999999999822 ) ;
#65622=CARTESIAN_POINT ( 'NONE',  ( -18.24374747313077094, 11.99999999999999822, 0.6271958409055273798 ) ) ;
#65623=CARTESIAN_POINT ( 'NONE',  ( 22.88594695219327235, 3.421158645304719137, 11.50198563395281148 ) ) ;
#65624=ORIENTED_EDGE ( 'NONE', *, *, #34099, .F. ) ;
#65628=EDGE_LOOP ( 'NONE', ( #11656, #53846, #12294, #59272 ) ) ;
#65629=VERTEX_POINT ( 'NONE', #48651 ) ;
#65630=CARTESIAN_POINT ( 'NONE',  ( -37.00000000000000711, -12.66641127287624968, -1.457575200925677494 ) ) ;
#65632=VECTOR ( 'NONE', #47531, 1000.000000000000000 ) ;
#65633=CARTESIAN_POINT ( 'NONE',  ( -35.00000000000000000, -11.47758908105692655, -2.497432891016966749 ) ) ;
#65636=DIRECTION ( 'NONE',  ( -0.000000000000000000, -0.000000000000000000, -1.000000000000000000 ) ) ;
#65637=LINE ( 'NONE', #4511, #58610 ) ;
#65639=EDGE_CURVE ( 'NONE', #64188, #65779, #4802, .T. ) ;
#65641=AXIS2_PLACEMENT_3D ( 'NONE', #8163, #28765, #49414 ) ;
#65642=ORIENTED_EDGE ( 'NONE', *, *, #47111, .T. ) ;
#65643=DIRECTION ( 'NONE',  ( -1.000000000000000000, 0.000000000000000000, -0.000000000000000000 ) ) ;
#65645=AXIS2_PLACEMENT_3D ( 'NONE', #17006, #1414, #47606 ) ;
#65647=B_SPLINE_CURVE_WITH_KNOTS ( 'NONE', 3,
 ( #36173, #26540, #51830, #11572, #310, #40521, #30860, #51183, #31527, #10580, #25903, #45853 ),
 .UNSPECIFIED., .F., .F.,
 ( 4, 2, 2, 2, 2, 4 ),
 ( 0.002404377236383827953, 0.003081670566939564634, 0.003758963897495300882, 0.005113550558606773377, 0.006468137219718247607, 0.007822723880829720103 ),
 .UNSPECIFIED. ) ;
#65648=EDGE_CURVE ( 'NONE', #35595, #61175, #32998, .T. ) ;
#65649=CARTESIAN_POINT ( 'NONE',  ( 145.1370849898475797, 3.309064568108273190E-14, 0.000000000000000000 ) ) ;
#65651=AXIS2_PLACEMENT_3D ( 'NONE', #51793, #62092, #47137 ) ;
#65653=CARTESIAN_POINT ( 'NONE',  ( 17.87400702017532339, 6.562307548641454602, 10.06038912854612022 ) ) ;
#65656=CARTESIAN_POINT ( 'NONE',  ( 28.54778262741603712, -12.36770326177027357, 5.424595989953875375 ) ) ;
#65657=ORIENTED_EDGE ( 'NONE', *, *, #11915, .F. ) ;
#65660=EDGE_CURVE ( 'NONE', #11187, #16616, #8737, .T. ) ;
#65662=FACE_OUTER_BOUND ( 'NONE', #22923, .T. ) ;
#65663=ADVANCED_FACE ( 'NONE', ( #53312 ), #33984, .T. ) ;
#65665=DIRECTION ( 'NONE',  ( 0.000000000000000000, -0.4134677391718385997, -0.9105187689796011563 ) ) ;
#65666=DIRECTION ( 'NONE',  ( 0.000000000000000000, -0.01356324068817998940, 0.9999080150203990547 ) ) ;
#65672=CARTESIAN_POINT ( 'NONE',  ( 35.00000000000000000, 8.389074212634284322, -8.839356091080075473 ) ) ;
#65674=AXIS2_PLACEMENT_3D ( 'NONE', #11725, #2093, #56665 ) ;
#65678=CIRCLE ( 'NONE', #29616, 4.999999999999998224 ) ;
#65679=EDGE_LOOP ( 'NONE', ( #57103, #41707, #23753, #55119 ) ) ;
#65683=ORIENTED_EDGE ( 'NONE', *, *, #40224, .F. ) ;
#65684=CIRCLE ( 'NONE', #61337, 4.999999999999999112 ) ;
#65686=CARTESIAN_POINT ( 'NONE',  ( -14.29135464769095520, 7.782112657557433089, -9.134479874907182051 ) ) ;
#65688=AXIS2_PLACEMENT_3D ( 'NONE', #20464, #35731, #56358 ) ;
#65689=DIRECTION ( 'NONE',  ( 0.000000000000000000, 0.9796553971857736576, 0.2006870767258926158 ) ) ;
#65690=VERTEX_POINT ( 'NONE', #6624 ) ;
#65691=DIRECTION ( 'NONE',  ( 1.000000000000000000, 0.000000000000000000, 0.000000000000000000 ) ) ;
#65694=ORIENTED_EDGE ( 'NONE', *, *, #7177, .F. ) ;
#65695=CARTESIAN_POINT ( 'NONE',  ( -37.00000000000000711, 0.000000000000000000, 0.000000000000000000 ) ) ;
#65696=DIRECTION ( 'NONE',  ( 1.000000000000000000, 0.000000000000000000, 0.000000000000000000 ) ) ;
#65697=CARTESIAN_POINT ( 'NONE',  ( -16.05996651011518850, 8.379490699920680186, -10.58476169280406154 ) ) ;
#65700=CARTESIAN_POINT ( 'NONE',  ( -35.00000000000000000, 7.882940143791919319, -10.02106554660700333 ) ) ;
#65703=DIRECTION ( 'NONE',  ( -1.000000000000000000, 0.000000000000000000, 0.000000000000000000 ) ) ;
#65707=VECTOR ( 'NONE', #50167, 1000.000000000000000 ) ;
#65708=DIRECTION ( 'NONE',  ( 1.000000000000000000, 0.000000000000000000, 0.000000000000000000 ) ) ;
#65709=EDGE_LOOP ( 'NONE', ( #39052, #38197, #32544, #16106 ) ) ;
#65710=DIRECTION ( 'NONE',  ( 0.000000000000000000, -0.8369827122275401710, -0.5472293298355184188 ) ) ;
#65711=EDGE_CURVE ( 'NONE', #7123, #35706, #53640, .T. ) ;
#65713=CIRCLE ( 'NONE', #39199, 5.000000000000001776 ) ;
#65714=DIRECTION ( 'NONE',  ( 0.000000000000000000, -1.000000000000000000, 0.000000000000000000 ) ) ;
#65717=DIRECTION ( 'NONE',  ( -1.000000000000000000, -0.000000000000000000, 0.000000000000000000 ) ) ;
#65718=ORIENTED_EDGE ( 'NONE', *, *, #63248, .T. ) ;
#65719=CARTESIAN_POINT ( 'NONE',  ( 22.36482863261543486, -11.96441317219524514, -0.9234811557364158707 ) ) ;
#65722=AXIS2_PLACEMENT_3D ( 'NONE', #52849, #1674, #58505 ) ;
#65724=AXIS2_PLACEMENT_3D ( 'NONE', #41751, #45421, #21480 ) ;
#65726=EDGE_CURVE ( 'NONE', #217, #18633, #14312, .T. ) ;
#65729=ORIENTED_EDGE ( 'NONE', *, *, #9349, .F. ) ;
#65731=FACE_OUTER_BOUND ( 'NONE', #47804, .T. ) ;
#65732=EDGE_CURVE ( 'NONE', #8648, #60414, #12177, .T. ) ;
#65733=LINE ( 'NONE', #25865, #40166 ) ;
#65734=CARTESIAN_POINT ( 'NONE',  ( 10.87033471826838138, 13.40550848972586273, -1.597425313190320662 ) ) ;
#65735=DIRECTION ( 'NONE',  ( -0.000000000000000000, -1.000000000000000000, -0.000000000000000000 ) ) ;
#65736=LINE ( 'NONE', #50160, #36162 ) ;
#65737=CYLINDRICAL_SURFACE ( 'NONE', #519, 12.75000000000000178 ) ;
#65740=EDGE_CURVE ( 'NONE', #50026, #51491, #34949, .T. ) ;
#65741=VERTEX_POINT ( 'NONE', #29985 ) ;
#65742=CARTESIAN_POINT ( 'NONE',  ( -36.00000000000000711, -6.415447294506629206, -11.01837265713080072 ) ) ;
#65743=ORIENTED_EDGE ( 'NONE', *, *, #19881, .T. ) ;
#65744=CYLINDRICAL_SURFACE ( 'NONE', #47704, 5.000000000000000888 ) ;
#65749=ORIENTED_EDGE ( 'NONE', *, *, #57734, .T. ) ;
#65750=FACE_OUTER_BOUND ( 'NONE', #36968, .T. ) ;
#65754=ADVANCED_FACE ( 'NONE', ( #55257 ), #57159, .T. ) ;
#65758=VERTEX_POINT ( 'NONE', #50615 ) ;
#65759=CIRCLE ( 'NONE', #37106, 5.000000000000000888 ) ;
#65760=CARTESIAN_POINT ( 'NONE',  ( -35.00000000000000000, 11.07407352312212723, 3.916263239775389149 ) ) ;
#65761=ORIENTED_EDGE ( 'NONE', *, *, #52223, .F. ) ;
#65762=DIRECTION ( 'NONE',  ( 1.000000000000000000, 0.000000000000000000, 0.000000000000000000 ) ) ;
#65764=DIRECTION ( 'NONE',  ( -0.000000000000000000, -0.000000000000000000, -1.000000000000000000 ) ) ;
#65765=FACE_OUTER_BOUND ( 'NONE', #35066, .T. ) ;
#65766=VECTOR ( 'NONE', #6046, 1000.000000000000000 ) ;
#65767=EDGE_CURVE ( 'NONE', #15829, #38263, #11587, .T. ) ;
#65768=VERTEX_POINT ( 'NONE', #20011 ) ;
#65771=ORIENTED_EDGE ( 'NONE', *, *, #37204, .F. ) ;
#65772=DIRECTION ( 'NONE',  ( 1.000000000000000000, 0.000000000000000000, 0.000000000000000000 ) ) ;
#65773=DIRECTION ( 'NONE',  ( 1.000000000000000000, 0.000000000000000000, 0.000000000000000000 ) ) ;
#65776=DIRECTION ( 'NONE',  ( 1.000000000000000000, 0.000000000000000000, 0.000000000000000000 ) ) ;
#65778=DIRECTION ( 'NONE',  ( -0.000000000000000000, -0.000000000000000000, -1.000000000000000000 ) ) ;
#65779=VERTEX_POINT ( 'NONE', #52174 ) ;
#65780=DIRECTION ( 'NONE',  ( 1.000000000000000000, 0.000000000000000000, 0.000000000000000000 ) ) ;
#65781=VECTOR ( 'NONE', #48192, 1000.000000000000000 ) ;
#65782=ORIENTED_EDGE ( 'NONE', *, *, #30774, .T. ) ;
#65783=CARTESIAN_POINT ( 'NONE',  ( 35.00000000000000000, 4.705694406421931860E-17, -3.469127814946512892E-15 ) ) ;
#65784=DIRECTION ( 'NONE',  ( 0.000000000000000000, 0.5987040770935676548, -0.8009703041134168533 ) ) ;
#65785=ORIENTED_EDGE ( 'NONE', *, *, #11214, .F. ) ;
#65786=DIRECTION ( 'NONE',  ( -0.7738190875236917732, 0.000000000000000000, 0.6334066780386838902 ) ) ;
#65789=CARTESIAN_POINT ( 'NONE',  ( -2.532614230583022152, -11.30437021680553222, 4.026315189028233377 ) ) ;
#65790=EDGE_CURVE ( 'NONE', #36164, #44780, #30273, .T. ) ;
#65791=CARTESIAN_POINT ( 'NONE',  ( 6.633398917601865286, -5.025995922460137599, -12.53510885642684158 ) ) ;
#65792=DIRECTION ( 'NONE',  ( -1.000000000000000000, 0.000000000000000000, -0.000000000000000000 ) ) ;
#65796=CARTESIAN_POINT ( 'NONE',  ( 37.00000000000000711, -3.307597835713332213, -12.31350058095522115 ) ) ;
#65800=ORIENTED_EDGE ( 'NONE', *, *, #13190, .T. ) ;
#65801=ORIENTED_EDGE ( 'NONE', *, *, #53934, .T. ) ;
#65806=AXIS2_PLACEMENT_3D ( 'NONE', #9666, #59914, #39611 ) ;
#65807=DIRECTION ( 'NONE',  ( 0.000000000000000000, -0.8009703041134103030, -0.5987040770935762035 ) ) ;
ENDSEC;
END-ISO-10303-21;
